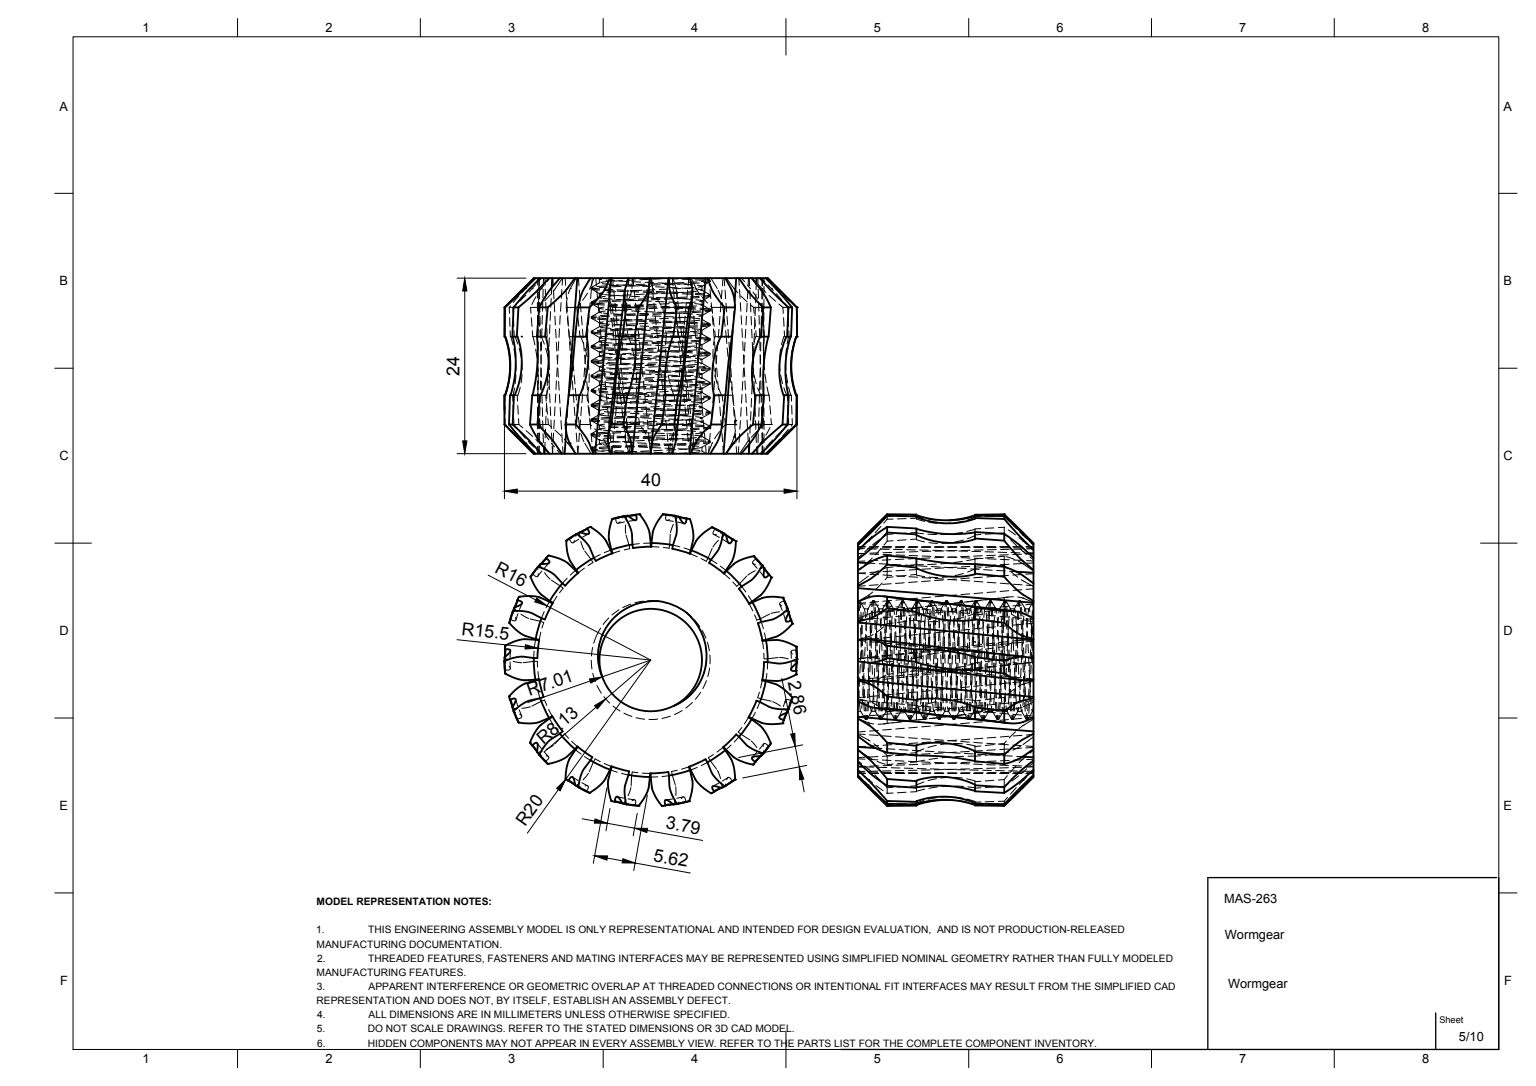
ISO-10303-21;
HEADER;
/* Generated by software containing ST-Developer
 * from STEP Tools, Inc. (www.steptools.com) 
 */

FILE_DESCRIPTION(
/* description */ (''),
/* implementation_level */ '2;1');

FILE_NAME(
/* name */ 'Wormgear.step',
/* time_stamp */ '2026-10-12T15:47:30-07:00',
/* author */ (''),
/* organization */ (''),
/* preprocessor_version */ 'ST-DEVELOPER v20.2',
/* originating_system */ 'Autodesk Translation Framework v15.15.0.0',
/* authorisation */ '');

FILE_SCHEMA (('AUTOMOTIVE_DESIGN { 1 0 10303 214 3 1 1 }'));
ENDSEC;

DATA;
#10=MECHANICAL_DESIGN_GEOMETRIC_PRESENTATION_REPRESENTATION('',(#82),#88483);
#64=SHAPE_REPRESENTATION_RELATIONSHIP('SRR','None',#88520,#73);
#73=ADVANCED_BREP_SHAPE_REPRESENTATION('',(#117),#88474);
#82=STYLED_ITEM('',(#88574),#117);
#117=MANIFOLD_SOLID_BREP('Body1',#12992);
#152=TOROIDAL_SURFACE('',#13586,31.2524414898979,12.0232331490224);
#153=TOROIDAL_SURFACE('',#13587,31.2524414898979,12.0232331490224);
#154=TOROIDAL_SURFACE('',#13588,31.2524414898979,12.0232331490224);
#155=TOROIDAL_SURFACE('',#13589,31.2524414898979,12.0232331490224);
#156=TOROIDAL_SURFACE('',#13590,31.2524414898979,12.0232331490224);
#157=TOROIDAL_SURFACE('',#13591,31.2524414898979,12.0232331490224);
#158=TOROIDAL_SURFACE('',#13592,31.2524414898979,12.0232331490224);
#159=TOROIDAL_SURFACE('',#13593,31.2524414898979,12.0232331490224);
#160=TOROIDAL_SURFACE('',#13594,31.2524414898979,12.0232331490224);
#161=TOROIDAL_SURFACE('',#13595,31.2524414898979,12.0232331490224);
#162=TOROIDAL_SURFACE('',#13596,31.2524414898979,12.0232331490224);
#163=TOROIDAL_SURFACE('',#13597,31.2524414898979,12.0232331490224);
#164=TOROIDAL_SURFACE('',#13598,31.2524414898979,12.0232331490224);
#165=TOROIDAL_SURFACE('',#13599,31.2524414898979,12.0232331490224);
#166=TOROIDAL_SURFACE('',#13600,31.2524414898979,12.0232331490224);
#167=TOROIDAL_SURFACE('',#13601,31.2524414898979,12.0232331490224);
#168=TOROIDAL_SURFACE('',#13602,31.2524414898979,12.0232331490224);
#169=TOROIDAL_SURFACE('',#13603,31.2524414898979,12.0232331490224);
#190=ELLIPSE('',#13431,4.95617711892471,2.63133228090511);
#191=ELLIPSE('',#13435,4.75668688712327,2.27225375309584);
#192=ELLIPSE('',#13437,4.75863627530638,2.27415348140964);
#193=ELLIPSE('',#13440,4.95728877126817,2.63371397588203);
#194=ELLIPSE('',#13442,4.75866828260205,2.27425851275333);
#195=ELLIPSE('',#13445,4.75676106745748,2.27242229825786);
#196=ELLIPSE('',#13449,4.95667352087062,2.63240829794641);
#197=ELLIPSE('',#13451,4.7584190628443,2.27363285019894);
#198=ELLIPSE('',#13454,4.95667835669603,2.63239579497757);
#199=ELLIPSE('',#13456,4.75854812753772,2.27394108049538);
#200=ELLIPSE('',#13459,4.75677100793017,2.27242870543475);
#201=ELLIPSE('',#13461,4.75867193464204,2.27425380136302);
#202=ELLIPSE('',#13464,4.95726759568865,2.6336926662635);
#203=ELLIPSE('',#13468,4.95701438814411,2.63313504607068);
#204=ELLIPSE('',#13470,4.75854681981732,2.2739502765965);
#205=ELLIPSE('',#13473,4.95618501228156,2.63134042899261);
#206=ELLIPSE('',#13475,4.7584142614767,2.27361309014758);
#207=ELLIPSE('',#13478,4.75669159480521,2.2722579746974);
#208=ELLIPSE('',#13480,4.75864115660623,2.27415786894356);
#209=ELLIPSE('',#13483,4.95728232466036,2.63370732110983);
#210=ELLIPSE('',#13487,4.75677068526519,2.27243087287144);
#211=ELLIPSE('',#13489,4.7586448406126,2.27416728394003);
#212=ELLIPSE('',#13492,4.95668328813391,2.63241837237374);
#213=ELLIPSE('',#13494,4.75842436294074,2.27363759998898);
#214=ELLIPSE('',#13497,4.95667013101771,2.63238731158809);
#215=ELLIPSE('',#13499,4.75854743391675,2.27394045782711);
#216=ELLIPSE('',#13502,4.75676675579442,2.2724249104892);
#217=ELLIPSE('',#13504,4.75867738441917,2.27425870334034);
#218=ELLIPSE('',#13507,4.95726880833492,2.63369391317148);
#219=ELLIPSE('',#13511,4.75669596930896,2.27226683434943);
#220=ELLIPSE('',#13516,4.95643307274524,2.6318762393004);
#221=ELLIPSE('',#13520,4.75673549365485,2.27235394216187);
#222=ELLIPSE('',#13524,4.75679029012967,2.27247967692196);
#223=ELLIPSE('',#13528,4.7567393782921,2.272363575723);
#224=ELLIPSE('',#13532,4.75651933654551,2.27183321728508);
#225=ELLIPSE('',#13536,4.75664142700045,2.27213579341419);
#226=ELLIPSE('',#13540,4.75678866048944,2.27247015627199);
#227=ELLIPSE('',#13544,4.75677929568429,2.27246401653084);
#228=ELLIPSE('',#13548,4.7566467644084,2.27215101059843);
#229=ELLIPSE('',#13552,4.75649416981517,2.27179513573923);
#230=ELLIPSE('',#13556,4.75673834040189,2.27235649175302);
#231=ELLIPSE('',#13560,4.7567849310581,2.27247488275134);
#232=ELLIPSE('',#13564,4.75674169310957,2.27236560062855);
#233=ELLIPSE('',#13568,4.75650474573201,2.27182012088408);
#234=ELLIPSE('',#13572,4.75664401077444,2.27213811276921);
#235=ELLIPSE('',#13576,4.75677759115208,2.27246023178278);
#236=ELLIPSE('',#13580,4.95724426884637,2.63364727447111);
#237=ELLIPSE('',#13584,4.95686686267409,2.63282116312156);
#290=CONICAL_SURFACE('',#13250,17.9979895488606,0.785398163397448);
#291=CONICAL_SURFACE('',#13253,17.9979895488606,0.785398163397448);
#292=CONICAL_SURFACE('',#13256,17.9979895488606,0.785398163397448);
#293=CONICAL_SURFACE('',#13259,17.9979895488606,0.785398163397448);
#294=CONICAL_SURFACE('',#13262,17.9979895488606,0.785398163397448);
#295=CONICAL_SURFACE('',#13265,17.9979895488606,0.785398163397448);
#296=CONICAL_SURFACE('',#13268,17.9979895488606,0.785398163397448);
#297=CONICAL_SURFACE('',#13271,17.9979895488606,0.785398163397448);
#298=CONICAL_SURFACE('',#13274,17.9979895488606,0.785398163397448);
#299=CONICAL_SURFACE('',#13277,17.9979895488606,0.785398163397448);
#300=CONICAL_SURFACE('',#13280,17.9979895488606,0.785398163397448);
#301=CONICAL_SURFACE('',#13283,17.9979895488606,0.785398163397448);
#302=CONICAL_SURFACE('',#13286,17.9979895488606,0.785398163397448);
#303=CONICAL_SURFACE('',#13289,17.9979895488606,0.785398163397448);
#304=CONICAL_SURFACE('',#13292,17.9979895488606,0.785398163397448);
#305=CONICAL_SURFACE('',#13295,17.9979895488606,0.785398163397448);
#306=CONICAL_SURFACE('',#13298,17.9979895488606,0.785398163397448);
#307=CONICAL_SURFACE('',#13301,17.9979895488606,0.785398163397448);
#308=CONICAL_SURFACE('',#13304,17.9979895488606,0.785398163397448);
#309=CONICAL_SURFACE('',#13309,17.9979895488606,0.785398163397448);
#310=CONICAL_SURFACE('',#13314,17.9979895488606,0.785398163397448);
#311=CONICAL_SURFACE('',#13319,17.9979895488606,0.785398163397448);
#312=CONICAL_SURFACE('',#13324,17.9979895488606,0.785398163397448);
#313=CONICAL_SURFACE('',#13329,17.9979895488606,0.785398163397448);
#314=CONICAL_SURFACE('',#13334,17.9979895488606,0.785398163397448);
#315=CONICAL_SURFACE('',#13339,17.9979895488606,0.785398163397448);
#316=CONICAL_SURFACE('',#13344,17.9979895488606,0.785398163397448);
#317=CONICAL_SURFACE('',#13349,17.9979895488606,0.785398163397448);
#318=CONICAL_SURFACE('',#13354,17.9979895488606,0.785398163397448);
#319=CONICAL_SURFACE('',#13359,17.9979895488606,0.785398163397448);
#320=CONICAL_SURFACE('',#13364,17.9979895488606,0.785398163397448);
#321=CONICAL_SURFACE('',#13369,17.9979895488606,0.785398163397448);
#322=CONICAL_SURFACE('',#13374,17.9979895488606,0.785398163397448);
#323=CONICAL_SURFACE('',#13379,17.9979895488606,0.785398163397448);
#324=CONICAL_SURFACE('',#13384,17.9979895488606,0.785398163397448);
#325=CONICAL_SURFACE('',#13389,17.9979895488606,0.785398163397448);
#347=FACE_BOUND('',#1491,.T.);
#348=FACE_BOUND('',#1720,.T.);
#440=PLANE('',#13159);
#441=PLANE('',#13196);
#442=PLANE('',#13199);
#443=PLANE('',#13202);
#444=PLANE('',#13205);
#445=PLANE('',#13208);
#446=PLANE('',#13211);
#447=PLANE('',#13214);
#448=PLANE('',#13217);
#449=PLANE('',#13220);
#450=PLANE('',#13223);
#451=PLANE('',#13226);
#452=PLANE('',#13229);
#453=PLANE('',#13232);
#454=PLANE('',#13235);
#455=PLANE('',#13238);
#456=PLANE('',#13241);
#457=PLANE('',#13244);
#458=PLANE('',#13247);
#459=PLANE('',#13394);
#460=PLANE('',#13396);
#461=PLANE('',#13398);
#462=PLANE('',#13400);
#463=PLANE('',#13402);
#464=PLANE('',#13404);
#465=PLANE('',#13406);
#466=PLANE('',#13408);
#467=PLANE('',#13410);
#468=PLANE('',#13412);
#469=PLANE('',#13414);
#470=PLANE('',#13416);
#471=PLANE('',#13418);
#472=PLANE('',#13420);
#473=PLANE('',#13422);
#474=PLANE('',#13424);
#475=PLANE('',#13426);
#476=PLANE('',#13428);
#477=PLANE('',#13430);
#478=PLANE('',#13434);
#479=PLANE('',#13439);
#480=PLANE('',#13444);
#481=PLANE('',#13448);
#482=PLANE('',#13453);
#483=PLANE('',#13458);
#484=PLANE('',#13463);
#485=PLANE('',#13467);
#486=PLANE('',#13472);
#487=PLANE('',#13477);
#488=PLANE('',#13482);
#489=PLANE('',#13486);
#490=PLANE('',#13491);
#491=PLANE('',#13496);
#492=PLANE('',#13501);
#493=PLANE('',#13506);
#494=PLANE('',#13510);
#495=PLANE('',#13514);
#496=PLANE('',#13518);
#497=PLANE('',#13522);
#498=PLANE('',#13526);
#499=PLANE('',#13530);
#500=PLANE('',#13534);
#501=PLANE('',#13538);
#502=PLANE('',#13542);
#503=PLANE('',#13546);
#504=PLANE('',#13550);
#505=PLANE('',#13554);
#506=PLANE('',#13558);
#507=PLANE('',#13562);
#508=PLANE('',#13566);
#509=PLANE('',#13570);
#510=PLANE('',#13574);
#511=PLANE('',#13578);
#512=PLANE('',#13582);
#513=PLANE('',#13680);
#610=B_SPLINE_SURFACE_WITH_KNOTS('',3,3,((#25169,#25170,#25171,#25172,#25173,
#25174,#25175,#25176,#25177,#25178,#25179,#25180,#25181,#25182,#25183,#25184,
#25185,#25186,#25187,#25188,#25189,#25190,#25191,#25192,#25193,#25194,#25195,
#25196,#25197,#25198,#25199,#25200,#25201,#25202,#25203,#25204,#25205,#25206,
#25207,#25208,#25209,#25210,#25211,#25212,#25213,#25214,#25215,#25216,#25217,
#25218,#25219,#25220,#25221,#25222,#25223,#25224,#25225,#25226,#25227,#25228,
#25229,#25230,#25231,#25232,#25233,#25234,#25235,#25236,#25237,#25238,#25239,
#25240,#25241,#25242,#25243,#25244,#25245,#25246,#25247,#25248,#25249,#25250,
#25251,#25252,#25253,#25254,#25255,#25256,#25257,#25258,#25259,#25260,#25261,
#25262,#25263,#25264,#25265,#25266,#25267,#25268,#25269,#25270,#25271,#25272,
#25273,#25274,#25275,#25276,#25277,#25278,#25279,#25280,#25281,#25282,#25283,
#25284,#25285,#25286,#25287,#25288,#25289,#25290,#25291,#25292,#25293,#25294,
#25295,#25296,#25297,#25298,#25299,#25300,#25301,#25302,#25303,#25304,#25305,
#25306,#25307,#25308,#25309,#25310,#25311,#25312,#25313,#25314,#25315,#25316,
#25317,#25318,#25319,#25320,#25321,#25322,#25323,#25324,#25325,#25326,#25327),
(#25328,#25329,#25330,#25331,#25332,#25333,#25334,#25335,#25336,#25337,
#25338,#25339,#25340,#25341,#25342,#25343,#25344,#25345,#25346,#25347,#25348,
#25349,#25350,#25351,#25352,#25353,#25354,#25355,#25356,#25357,#25358,#25359,
#25360,#25361,#25362,#25363,#25364,#25365,#25366,#25367,#25368,#25369,#25370,
#25371,#25372,#25373,#25374,#25375,#25376,#25377,#25378,#25379,#25380,#25381,
#25382,#25383,#25384,#25385,#25386,#25387,#25388,#25389,#25390,#25391,#25392,
#25393,#25394,#25395,#25396,#25397,#25398,#25399,#25400,#25401,#25402,#25403,
#25404,#25405,#25406,#25407,#25408,#25409,#25410,#25411,#25412,#25413,#25414,
#25415,#25416,#25417,#25418,#25419,#25420,#25421,#25422,#25423,#25424,#25425,
#25426,#25427,#25428,#25429,#25430,#25431,#25432,#25433,#25434,#25435,#25436,
#25437,#25438,#25439,#25440,#25441,#25442,#25443,#25444,#25445,#25446,#25447,
#25448,#25449,#25450,#25451,#25452,#25453,#25454,#25455,#25456,#25457,#25458,
#25459,#25460,#25461,#25462,#25463,#25464,#25465,#25466,#25467,#25468,#25469,
#25470,#25471,#25472,#25473,#25474,#25475,#25476,#25477,#25478,#25479,#25480,
#25481,#25482,#25483,#25484,#25485,#25486),(#25487,#25488,#25489,#25490,
#25491,#25492,#25493,#25494,#25495,#25496,#25497,#25498,#25499,#25500,#25501,
#25502,#25503,#25504,#25505,#25506,#25507,#25508,#25509,#25510,#25511,#25512,
#25513,#25514,#25515,#25516,#25517,#25518,#25519,#25520,#25521,#25522,#25523,
#25524,#25525,#25526,#25527,#25528,#25529,#25530,#25531,#25532,#25533,#25534,
#25535,#25536,#25537,#25538,#25539,#25540,#25541,#25542,#25543,#25544,#25545,
#25546,#25547,#25548,#25549,#25550,#25551,#25552,#25553,#25554,#25555,#25556,
#25557,#25558,#25559,#25560,#25561,#25562,#25563,#25564,#25565,#25566,#25567,
#25568,#25569,#25570,#25571,#25572,#25573,#25574,#25575,#25576,#25577,#25578,
#25579,#25580,#25581,#25582,#25583,#25584,#25585,#25586,#25587,#25588,#25589,
#25590,#25591,#25592,#25593,#25594,#25595,#25596,#25597,#25598,#25599,#25600,
#25601,#25602,#25603,#25604,#25605,#25606,#25607,#25608,#25609,#25610,#25611,
#25612,#25613,#25614,#25615,#25616,#25617,#25618,#25619,#25620,#25621,#25622,
#25623,#25624,#25625,#25626,#25627,#25628,#25629,#25630,#25631,#25632,#25633,
#25634,#25635,#25636,#25637,#25638,#25639,#25640,#25641,#25642,#25643,#25644,
#25645),(#25646,#25647,#25648,#25649,#25650,#25651,#25652,#25653,#25654,
#25655,#25656,#25657,#25658,#25659,#25660,#25661,#25662,#25663,#25664,#25665,
#25666,#25667,#25668,#25669,#25670,#25671,#25672,#25673,#25674,#25675,#25676,
#25677,#25678,#25679,#25680,#25681,#25682,#25683,#25684,#25685,#25686,#25687,
#25688,#25689,#25690,#25691,#25692,#25693,#25694,#25695,#25696,#25697,#25698,
#25699,#25700,#25701,#25702,#25703,#25704,#25705,#25706,#25707,#25708,#25709,
#25710,#25711,#25712,#25713,#25714,#25715,#25716,#25717,#25718,#25719,#25720,
#25721,#25722,#25723,#25724,#25725,#25726,#25727,#25728,#25729,#25730,#25731,
#25732,#25733,#25734,#25735,#25736,#25737,#25738,#25739,#25740,#25741,#25742,
#25743,#25744,#25745,#25746,#25747,#25748,#25749,#25750,#25751,#25752,#25753,
#25754,#25755,#25756,#25757,#25758,#25759,#25760,#25761,#25762,#25763,#25764,
#25765,#25766,#25767,#25768,#25769,#25770,#25771,#25772,#25773,#25774,#25775,
#25776,#25777,#25778,#25779,#25780,#25781,#25782,#25783,#25784,#25785,#25786,
#25787,#25788,#25789,#25790,#25791,#25792,#25793,#25794,#25795,#25796,#25797,
#25798,#25799,#25800,#25801,#25802,#25803,#25804)),.UNSPECIFIED.,.F.,.F.,
 .F.,(4,4),(4,1,1,1,1,1,1,1,1,1,1,1,1,1,1,1,1,1,1,1,1,1,1,1,1,1,1,1,1,1,
1,1,1,1,1,1,1,1,1,1,1,1,1,1,1,1,1,1,1,1,1,1,1,1,1,1,1,1,1,1,1,1,1,1,1,1,
1,1,1,1,1,1,1,1,1,1,1,1,1,1,1,1,1,1,1,1,1,1,1,1,1,1,1,1,1,1,1,1,1,1,1,1,
1,1,1,1,1,1,1,1,1,1,1,1,1,1,1,1,1,1,1,1,1,1,1,1,1,1,1,1,1,1,1,1,1,1,1,1,
1,1,1,1,1,1,1,1,1,1,1,1,1,1,1,1,1,1,4),(-8.30696747198589E-5,0.128693006748574),
(11.8548247440635,12.351182148212,12.8474564826858,13.3437308171596,13.8400051516334,
14.3362794861072,14.832553820581,15.3288281550548,15.8251024895286,16.3213768240024,
16.8176511584762,17.31392549295,17.8101998274238,18.3064741618976,18.8027484963714,
19.2990228308452,19.7952971653189,20.2915714997927,20.7878458342665,21.2841201687403,
21.7803945032141,22.2766688376879,22.7729431721617,23.2692175066355,23.7654918411093,
24.2617661755831,24.7580405100569,25.2543148445307,25.7505891790045,26.2468635134783,
26.7431378479521,27.2394121824259,27.7356865168997,28.2319608513735,28.7282351858473,
29.224509520321,29.7207838547948,30.2170581892686,30.7133325237424,31.2096068582162,
31.70588119269,32.2021555271638,32.6984298616376,33.1947041961114,33.6909785305852,
34.187252865059,34.6835271995328,35.1798015340066,35.6760758684804,36.1723502029542,
36.668624537428,37.1648988719018,37.6611732063756,38.1574475408493,38.6537218753231,
39.1499962097969,39.6462705442707,40.1425448787445,40.6388192132183,41.1350935476921,
41.6313678821659,42.1276422166397,42.6239165511135,43.1201908855873,43.6164652200611,
44.1127395545349,44.6090138890087,45.1052882234825,45.6015625579563,46.0978368924301,
46.5941112269039,47.0903855613777,47.5866598958514,48.0829342303252,48.579208564799,
49.0754828992728,49.5717572337466,50.0680315682204,50.5643059026942,51.060580237168,
51.5568545716418,52.0531289061156,52.5494032405894,53.0456775750632,53.541951909537,
54.0382262440108,54.5345005784846,55.0307749129584,55.5270492474322,56.023323581906,
56.5195979163798,57.0158722508535,57.5121465853273,58.0084209198011,58.5046952542749,
59.0009695887487,59.4972439232225,59.9935182576963,60.4897925921701,60.9860669266439,
61.4823412611177,61.9786155955915,62.4748899300653,62.9711642645391,63.4674385990129,
63.9637129334867,64.4599872679605,64.9562616024343,65.452535936908,65.9488102713818,
66.4450846058556,66.9413589403294,67.4376332748032,67.933907609277,68.4301819437508,
68.9264562782246,69.4227306126984,69.9190049471722,70.415279281646,70.9115536161198,
71.4078279505936,71.9041022850674,72.4003766195412,72.896650954015,73.3929252884888,
73.8891996229626,74.3854739574363,74.8817482919101,75.3780226263839,75.8742969608577,
76.3705712953315,76.8668456298053,77.3631199642791,77.8593942987529,78.3556686332267,
78.8519429677005,79.3482173021743,79.8444916366481,80.3407659711219,80.8370403055957,
81.3333146400695,81.8295889745433,82.3258633090171,82.8221376434909,83.3184119779647,
83.8146863124385,84.3109606469122,84.807234981386,85.3035093158598,85.7997836503336,
86.2960579848074,86.7923323192812,87.288606653755,87.7848809882288,88.2811553227026,
88.7774296571764,89.2737039916502),.UNSPECIFIED.);
#611=B_SPLINE_SURFACE_WITH_KNOTS('',3,3,((#26032,#26033,#26034,#26035,#26036,
#26037,#26038,#26039,#26040,#26041,#26042,#26043,#26044,#26045,#26046,#26047,
#26048,#26049,#26050,#26051,#26052,#26053,#26054,#26055,#26056,#26057,#26058,
#26059,#26060,#26061,#26062,#26063,#26064,#26065,#26066,#26067,#26068,#26069,
#26070,#26071,#26072,#26073,#26074,#26075,#26076,#26077,#26078,#26079,#26080,
#26081,#26082,#26083,#26084,#26085,#26086,#26087,#26088,#26089,#26090,#26091,
#26092,#26093,#26094,#26095,#26096,#26097,#26098,#26099,#26100,#26101,#26102,
#26103,#26104,#26105,#26106,#26107,#26108,#26109,#26110,#26111,#26112,#26113,
#26114,#26115,#26116,#26117,#26118,#26119,#26120,#26121,#26122,#26123,#26124,
#26125,#26126,#26127,#26128,#26129,#26130,#26131,#26132,#26133,#26134,#26135,
#26136,#26137,#26138,#26139,#26140,#26141,#26142,#26143,#26144,#26145,#26146,
#26147,#26148,#26149,#26150,#26151,#26152,#26153,#26154,#26155,#26156,#26157,
#26158,#26159,#26160,#26161,#26162,#26163,#26164,#26165,#26166,#26167,#26168,
#26169,#26170,#26171,#26172,#26173,#26174,#26175,#26176,#26177,#26178,#26179,
#26180,#26181,#26182,#26183,#26184,#26185,#26186,#26187,#26188,#26189,#26190),
(#26191,#26192,#26193,#26194,#26195,#26196,#26197,#26198,#26199,#26200,
#26201,#26202,#26203,#26204,#26205,#26206,#26207,#26208,#26209,#26210,#26211,
#26212,#26213,#26214,#26215,#26216,#26217,#26218,#26219,#26220,#26221,#26222,
#26223,#26224,#26225,#26226,#26227,#26228,#26229,#26230,#26231,#26232,#26233,
#26234,#26235,#26236,#26237,#26238,#26239,#26240,#26241,#26242,#26243,#26244,
#26245,#26246,#26247,#26248,#26249,#26250,#26251,#26252,#26253,#26254,#26255,
#26256,#26257,#26258,#26259,#26260,#26261,#26262,#26263,#26264,#26265,#26266,
#26267,#26268,#26269,#26270,#26271,#26272,#26273,#26274,#26275,#26276,#26277,
#26278,#26279,#26280,#26281,#26282,#26283,#26284,#26285,#26286,#26287,#26288,
#26289,#26290,#26291,#26292,#26293,#26294,#26295,#26296,#26297,#26298,#26299,
#26300,#26301,#26302,#26303,#26304,#26305,#26306,#26307,#26308,#26309,#26310,
#26311,#26312,#26313,#26314,#26315,#26316,#26317,#26318,#26319,#26320,#26321,
#26322,#26323,#26324,#26325,#26326,#26327,#26328,#26329,#26330,#26331,#26332,
#26333,#26334,#26335,#26336,#26337,#26338,#26339,#26340,#26341,#26342,#26343,
#26344,#26345,#26346,#26347,#26348,#26349),(#26350,#26351,#26352,#26353,
#26354,#26355,#26356,#26357,#26358,#26359,#26360,#26361,#26362,#26363,#26364,
#26365,#26366,#26367,#26368,#26369,#26370,#26371,#26372,#26373,#26374,#26375,
#26376,#26377,#26378,#26379,#26380,#26381,#26382,#26383,#26384,#26385,#26386,
#26387,#26388,#26389,#26390,#26391,#26392,#26393,#26394,#26395,#26396,#26397,
#26398,#26399,#26400,#26401,#26402,#26403,#26404,#26405,#26406,#26407,#26408,
#26409,#26410,#26411,#26412,#26413,#26414,#26415,#26416,#26417,#26418,#26419,
#26420,#26421,#26422,#26423,#26424,#26425,#26426,#26427,#26428,#26429,#26430,
#26431,#26432,#26433,#26434,#26435,#26436,#26437,#26438,#26439,#26440,#26441,
#26442,#26443,#26444,#26445,#26446,#26447,#26448,#26449,#26450,#26451,#26452,
#26453,#26454,#26455,#26456,#26457,#26458,#26459,#26460,#26461,#26462,#26463,
#26464,#26465,#26466,#26467,#26468,#26469,#26470,#26471,#26472,#26473,#26474,
#26475,#26476,#26477,#26478,#26479,#26480,#26481,#26482,#26483,#26484,#26485,
#26486,#26487,#26488,#26489,#26490,#26491,#26492,#26493,#26494,#26495,#26496,
#26497,#26498,#26499,#26500,#26501,#26502,#26503,#26504,#26505,#26506,#26507,
#26508),(#26509,#26510,#26511,#26512,#26513,#26514,#26515,#26516,#26517,
#26518,#26519,#26520,#26521,#26522,#26523,#26524,#26525,#26526,#26527,#26528,
#26529,#26530,#26531,#26532,#26533,#26534,#26535,#26536,#26537,#26538,#26539,
#26540,#26541,#26542,#26543,#26544,#26545,#26546,#26547,#26548,#26549,#26550,
#26551,#26552,#26553,#26554,#26555,#26556,#26557,#26558,#26559,#26560,#26561,
#26562,#26563,#26564,#26565,#26566,#26567,#26568,#26569,#26570,#26571,#26572,
#26573,#26574,#26575,#26576,#26577,#26578,#26579,#26580,#26581,#26582,#26583,
#26584,#26585,#26586,#26587,#26588,#26589,#26590,#26591,#26592,#26593,#26594,
#26595,#26596,#26597,#26598,#26599,#26600,#26601,#26602,#26603,#26604,#26605,
#26606,#26607,#26608,#26609,#26610,#26611,#26612,#26613,#26614,#26615,#26616,
#26617,#26618,#26619,#26620,#26621,#26622,#26623,#26624,#26625,#26626,#26627,
#26628,#26629,#26630,#26631,#26632,#26633,#26634,#26635,#26636,#26637,#26638,
#26639,#26640,#26641,#26642,#26643,#26644,#26645,#26646,#26647,#26648,#26649,
#26650,#26651,#26652,#26653,#26654,#26655,#26656,#26657,#26658,#26659,#26660,
#26661,#26662,#26663,#26664,#26665,#26666,#26667)),.UNSPECIFIED.,.F.,.F.,
 .F.,(4,4),(4,1,1,1,1,1,1,1,1,1,1,1,1,1,1,1,1,1,1,1,1,1,1,1,1,1,1,1,1,1,
1,1,1,1,1,1,1,1,1,1,1,1,1,1,1,1,1,1,1,1,1,1,1,1,1,1,1,1,1,1,1,1,1,1,1,1,
1,1,1,1,1,1,1,1,1,1,1,1,1,1,1,1,1,1,1,1,1,1,1,1,1,1,1,1,1,1,1,1,1,1,1,1,
1,1,1,1,1,1,1,1,1,1,1,1,1,1,1,1,1,1,1,1,1,1,1,1,1,1,1,1,1,1,1,1,1,1,1,1,
1,1,1,1,1,1,1,1,1,1,1,1,1,1,1,1,1,1,4),(-5.91850316919151E-5,0.128716709650167),
(14.3988535768129,14.8951279112866,15.3914022457604,15.8876765802342,16.383950914708,
16.8802252491818,17.3764995836556,17.8727739181294,18.3690482526032,18.865322587077,
19.3615969215508,19.8578712560246,20.3541455904984,20.8504199249722,21.346694259446,
21.8429685939198,22.3392429283936,22.8355172628674,23.3317915973412,23.828065931815,
24.3243402662887,24.8206146007625,25.3168889352363,25.8131632697101,26.3094376041839,
26.8057119386577,27.3019862731315,27.7982606076053,28.2945349420791,28.7908092765529,
29.2870836110267,29.7833579455005,30.2796322799743,30.7759066144481,31.2721809489219,
31.7684552833957,32.2647296178695,32.7610039523433,33.2572782868171,33.7535526212909,
34.2498269557646,34.7461012902384,35.2423756247122,35.738649959186,36.2349242936598,
36.7311986281336,37.2274729626074,37.7237472970812,38.220021631555,38.7162959660288,
39.2125703005026,39.7088446349764,40.2051189694502,40.701393303924,41.1976676383978,
41.6939419728716,42.1902163073454,42.6864906418191,43.1827649762929,43.6790393107667,
44.1753136452405,44.6715879797143,45.1678623141881,45.6641366486619,46.1604109831357,
46.6566853176095,47.1529596520833,47.6492339865571,48.1455083210309,48.6417826555047,
49.1380569899785,49.6343313244523,50.1306056589261,50.6268799933999,51.1231543278737,
51.6194286623475,52.1157029968213,52.6119773312951,53.1082516657688,53.6045260002426,
54.1008003347164,54.5970746691902,55.093349003664,55.5896233381378,56.0858976726116,
56.5821720070854,57.0784463415592,57.574720676033,58.0709950105068,58.5672693449806,
59.0635436794544,59.5598180139282,60.056092348402,60.5523666828758,61.0486410173496,
61.5449153518233,62.0411896862971,62.5374640207709,63.0337383552447,63.5300126897185,
64.0262870241923,64.5225613586661,65.0188356931399,65.5151100276137,66.0113843620875,
66.5076586965613,67.0039330310351,67.5002073655089,67.9964816999827,68.4927560344565,
68.9890303689303,69.4853047034041,69.9815790378779,70.4778533723517,70.9741277068254,
71.4704020412992,71.966676375773,72.4629507102468,72.9592250447206,73.4554993791944,
73.9517737136682,74.448048048142,74.9443223826158,75.4405967170896,75.9368710515634,
76.4331453860372,76.929419720511,77.4256940549848,77.9219683894586,78.4182427239324,
78.9145170584062,79.41079139288,79.9070657273538,80.4033400618275,80.8996143963013,
81.3958887307751,81.8921630652489,82.3884373997227,82.8847117341965,83.3809860686703,
83.8772604031441,84.3735347376179,84.8698090720917,85.3660834065655,85.8623577410393,
86.3586320755131,86.8549064099869,87.3511807444607,87.8474550789345,88.3437294134083,
88.8400037478821,89.3362780823559,89.8325524168297,90.3288267513034,90.8251010857772,
91.321375420251,91.8177328243995),.UNSPECIFIED.);
#612=B_SPLINE_SURFACE_WITH_KNOTS('',3,3,((#29359,#29360,#29361,#29362),
(#29363,#29364,#29365,#29366),(#29367,#29368,#29369,#29370),(#29371,#29372,
#29373,#29374)),.UNSPECIFIED.,.F.,.F.,.F.,(4,4),(4,4),(-1.00000000738492,
6.33181493099193E-12),(-0.228566601102733,0.828566601102733),
 .UNSPECIFIED.);
#613=B_SPLINE_SURFACE_WITH_KNOTS('',3,3,((#29383,#29384,#29385,#29386),
(#29387,#29388,#29389,#29390),(#29391,#29392,#29393,#29394),(#29395,#29396,
#29397,#29398)),.UNSPECIFIED.,.F.,.F.,.F.,(4,4),(4,4),(-1.00000000738848,
7.85174896767267E-12),(-0.228566601102733,0.828566601102734),
 .UNSPECIFIED.);
#614=B_SPLINE_SURFACE_WITH_KNOTS('',3,3,((#29407,#29408,#29409,#29410),
(#29411,#29412,#29413,#29414),(#29415,#29416,#29417,#29418),(#29419,#29420,
#29421,#29422)),.UNSPECIFIED.,.F.,.F.,.F.,(4,4),(4,4),(-1.00000000739146,
1.55845144401953E-11),(-0.228566601102734,0.828566601102734),
 .UNSPECIFIED.);
#615=B_SPLINE_SURFACE_WITH_KNOTS('',3,3,((#29431,#29432,#29433,#29434),
(#29435,#29436,#29437,#29438),(#29439,#29440,#29441,#29442),(#29443,#29444,
#29445,#29446)),.UNSPECIFIED.,.F.,.F.,.F.,(4,4),(4,4),(-1.00000000737499,
1.10248632487242E-11),(-0.228566601102733,0.828566601102734),
 .UNSPECIFIED.);
#616=B_SPLINE_SURFACE_WITH_KNOTS('',3,3,((#29455,#29456,#29457,#29458),
(#29459,#29460,#29461,#29462),(#29463,#29464,#29465,#29466),(#29467,#29468,
#29469,#29470)),.UNSPECIFIED.,.F.,.F.,.F.,(4,4),(4,4),(-1.00000000737555,
8.62684039186831E-12),(-0.228566601102733,0.828566601102733),
 .UNSPECIFIED.);
#617=B_SPLINE_SURFACE_WITH_KNOTS('',3,3,((#29479,#29480,#29481,#29482),
(#29483,#29484,#29485,#29486),(#29487,#29488,#29489,#29490),(#29491,#29492,
#29493,#29494)),.UNSPECIFIED.,.F.,.F.,.F.,(4,4),(4,4),(-1.00000000738693,
5.72012097454778E-12),(-0.228566601102733,0.828566601102734),
 .UNSPECIFIED.);
#618=B_SPLINE_SURFACE_WITH_KNOTS('',3,3,((#29503,#29504,#29505,#29506),
(#29507,#29508,#29509,#29510),(#29511,#29512,#29513,#29514),(#29515,#29516,
#29517,#29518)),.UNSPECIFIED.,.F.,.F.,.F.,(4,4),(4,4),(-1.00000000738919,
5.62379169111571E-12),(-0.228566601102733,0.828566601102734),
 .UNSPECIFIED.);
#619=B_SPLINE_SURFACE_WITH_KNOTS('',3,3,((#29527,#29528,#29529,#29530),
(#29531,#29532,#29533,#29534),(#29535,#29536,#29537,#29538),(#29539,#29540,
#29541,#29542)),.UNSPECIFIED.,.F.,.F.,.F.,(4,4),(4,4),(-1.00000000739289,
6.50467340161261E-12),(-0.228566601102733,0.828566601102733),
 .UNSPECIFIED.);
#620=B_SPLINE_SURFACE_WITH_KNOTS('',3,3,((#29551,#29552,#29553,#29554),
(#29555,#29556,#29557,#29558),(#29559,#29560,#29561,#29562),(#29563,#29564,
#29565,#29566)),.UNSPECIFIED.,.F.,.F.,.F.,(4,4),(4,4),(-1.00000000739148,
1.40793838710229E-11),(-0.228566601102733,0.828566601102734),
 .UNSPECIFIED.);
#621=B_SPLINE_SURFACE_WITH_KNOTS('',3,3,((#29575,#29576,#29577,#29578),
(#29579,#29580,#29581,#29582),(#29583,#29584,#29585,#29586),(#29587,#29588,
#29589,#29590)),.UNSPECIFIED.,.F.,.F.,.F.,(4,4),(4,4),(-1.00000000738262,
1.82838412051694E-11),(-0.228566601102733,0.828566601102734),
 .UNSPECIFIED.);
#622=B_SPLINE_SURFACE_WITH_KNOTS('',3,3,((#29599,#29600,#29601,#29602),
(#29603,#29604,#29605,#29606),(#29607,#29608,#29609,#29610),(#29611,#29612,
#29613,#29614)),.UNSPECIFIED.,.F.,.F.,.F.,(4,4),(4,4),(-1.00000000737784,
1.02973089179534E-11),(-0.228566601102733,0.828566601102734),
 .UNSPECIFIED.);
#623=B_SPLINE_SURFACE_WITH_KNOTS('',3,3,((#29623,#29624,#29625,#29626),
(#29627,#29628,#29629,#29630),(#29631,#29632,#29633,#29634),(#29635,#29636,
#29637,#29638)),.UNSPECIFIED.,.F.,.F.,.F.,(4,4),(4,4),(-1.00000000738658,
8.03237988227756E-12),(-0.228566601102733,0.828566601102733),
 .UNSPECIFIED.);
#624=B_SPLINE_SURFACE_WITH_KNOTS('',3,3,((#29647,#29648,#29649,#29650),
(#29651,#29652,#29653,#29654),(#29655,#29656,#29657,#29658),(#29659,#29660,
#29661,#29662)),.UNSPECIFIED.,.F.,.F.,.F.,(4,4),(4,4),(-1.00000000738646,
1.53840942326398E-11),(-0.228566601102734,0.828566601102734),
 .UNSPECIFIED.);
#625=B_SPLINE_SURFACE_WITH_KNOTS('',3,3,((#29671,#29672,#29673,#29674),
(#29675,#29676,#29677,#29678),(#29679,#29680,#29681,#29682),(#29683,#29684,
#29685,#29686)),.UNSPECIFIED.,.F.,.F.,.F.,(4,4),(4,4),(-1.00000000737555,
1.43664760969259E-11),(-0.228566601102733,0.828566601102734),
 .UNSPECIFIED.);
#626=B_SPLINE_SURFACE_WITH_KNOTS('',3,3,((#29695,#29696,#29697,#29698),
(#29699,#29700,#29701,#29702),(#29703,#29704,#29705,#29706),(#29707,#29708,
#29709,#29710)),.UNSPECIFIED.,.F.,.F.,.F.,(4,4),(4,4),(-1.00000000738601,
1.73046711715086E-14),(-0.228566601102733,0.828566601102733),
 .UNSPECIFIED.);
#627=B_SPLINE_SURFACE_WITH_KNOTS('',3,3,((#29719,#29720,#29721,#29722),
(#29723,#29724,#29725,#29726),(#29727,#29728,#29729,#29730),(#29731,#29732,
#29733,#29734)),.UNSPECIFIED.,.F.,.F.,.F.,(4,4),(4,4),(-1.00000000738919,
1.07500378715111E-11),(-0.228566601102733,0.828566601102734),
 .UNSPECIFIED.);
#628=B_SPLINE_SURFACE_WITH_KNOTS('',3,3,((#29743,#29744,#29745,#29746),
(#29747,#29748,#29749,#29750),(#29751,#29752,#29753,#29754),(#29755,#29756,
#29757,#29758)),.UNSPECIFIED.,.F.,.F.,.F.,(4,4),(4,4),(-1.00000000739238,
1.18069447204771E-11),(-0.228566601102733,0.828566601102734),
 .UNSPECIFIED.);
#629=B_SPLINE_SURFACE_WITH_KNOTS('',3,3,((#29767,#29768,#29769,#29770),
(#29771,#29772,#29773,#29774),(#29775,#29776,#29777,#29778),(#29779,#29780,
#29781,#29782)),.UNSPECIFIED.,.F.,.F.,.F.,(4,4),(4,4),(-1.00000000739217,
1.4414592214071E-11),(-0.228566601102733,0.828566601102734),
 .UNSPECIFIED.);
#630=B_SPLINE_SURFACE_WITH_KNOTS('',3,3,((#29791,#29792,#29793,#29794),
(#29795,#29796,#29797,#29798),(#29799,#29800,#29801,#29802),(#29803,#29804,
#29805,#29806),(#29807,#29808,#29809,#29810),(#29811,#29812,#29813,#29814),
(#29815,#29816,#29817,#29818)),.UNSPECIFIED.,.F.,.F.,.F.,(4,1,1,1,4),(4,
4),(-5.05014469441185E-14,0.1428571428571,0.28571428571425,0.571428571428551,
1.00000036560903),(-0.228509057368286,0.828509057368286),.UNSPECIFIED.);
#631=B_SPLINE_SURFACE_WITH_KNOTS('',3,3,((#29825,#29826,#29827,#29828),
(#29829,#29830,#29831,#29832),(#29833,#29834,#29835,#29836),(#29837,#29838,
#29839,#29840),(#29841,#29842,#29843,#29844),(#29845,#29846,#29847,#29848)),
 .UNSPECIFIED.,.F.,.F.,.F.,(4,1,1,4),(4,4),(-1.00000000000001,-0.42857142857138,
-0.214285714285645,9.03251141877686E-14),(-0.228509057368286,0.828509057368286),
 .UNSPECIFIED.);
#632=B_SPLINE_SURFACE_WITH_KNOTS('',3,3,((#29851,#29852,#29853,#29854),
(#29855,#29856,#29857,#29858),(#29859,#29860,#29861,#29862),(#29863,#29864,
#29865,#29866)),.UNSPECIFIED.,.F.,.F.,.F.,(4,4),(4,4),(-1.25904053593043E-16,
0.0850880881510745),(-0.100000001340248,0.1),.UNSPECIFIED.);
#633=B_SPLINE_SURFACE_WITH_KNOTS('',3,3,((#29867,#29868,#29869,#29870),
(#29871,#29872,#29873,#29874),(#29875,#29876,#29877,#29878),(#29879,#29880,
#29881,#29882)),.UNSPECIFIED.,.F.,.F.,.F.,(4,4),(4,4),(-1.25904053593043E-16,
0.0850880881510745),(0.5,0.700000001340097),.UNSPECIFIED.);
#634=B_SPLINE_SURFACE_WITH_KNOTS('',3,3,((#29883,#29884,#29885,#29886),
(#29887,#29888,#29889,#29890),(#29891,#29892,#29893,#29894),(#29895,#29896,
#29897,#29898),(#29899,#29900,#29901,#29902),(#29903,#29904,#29905,#29906)),
 .UNSPECIFIED.,.F.,.F.,.F.,(4,1,1,4),(4,4),(-5.14134515353765E-14,0.214285714285675,
0.4285714285714,1.),(-0.228509057368286,0.828509057368286),
 .UNSPECIFIED.);
#635=B_SPLINE_SURFACE_WITH_KNOTS('',3,3,((#29913,#29914,#29915,#29916),
(#29917,#29918,#29919,#29920),(#29921,#29922,#29923,#29924),(#29925,#29926,
#29927,#29928),(#29929,#29930,#29931,#29932),(#29933,#29934,#29935,#29936)),
 .UNSPECIFIED.,.F.,.F.,.F.,(4,1,1,4),(4,4),(-1.00000000000001,-0.428571428571412,
-0.214285714285689,3.45222547669068E-14),(-0.228509057368286,0.828509057368286),
 .UNSPECIFIED.);
#636=B_SPLINE_SURFACE_WITH_KNOTS('',3,3,((#29939,#29940,#29941,#29942),
(#29943,#29944,#29945,#29946),(#29947,#29948,#29949,#29950),(#29951,#29952,
#29953,#29954)),.UNSPECIFIED.,.F.,.F.,.F.,(4,4),(4,4),(-6.55275566865934E-17,
0.0850880881510748),(-0.100000001340248,0.1),.UNSPECIFIED.);
#637=B_SPLINE_SURFACE_WITH_KNOTS('',3,3,((#29955,#29956,#29957,#29958),
(#29959,#29960,#29961,#29962),(#29963,#29964,#29965,#29966),(#29967,#29968,
#29969,#29970)),.UNSPECIFIED.,.F.,.F.,.F.,(4,4),(4,4),(-6.55275566865934E-17,
0.0850880881510748),(0.5,0.700000001340096),.UNSPECIFIED.);
#638=B_SPLINE_SURFACE_WITH_KNOTS('',3,3,((#29971,#29972,#29973,#29974),
(#29975,#29976,#29977,#29978),(#29979,#29980,#29981,#29982),(#29983,#29984,
#29985,#29986),(#29987,#29988,#29989,#29990),(#29991,#29992,#29993,#29994),
(#29995,#29996,#29997,#29998)),.UNSPECIFIED.,.F.,.F.,.F.,(4,1,1,1,4),(4,
4),(-1.49004572061584E-13,0.142857142857015,0.28571428571418,0.571428571428509,
1.),(-0.228509057368286,0.828509057368286),.UNSPECIFIED.);
#639=B_SPLINE_SURFACE_WITH_KNOTS('',3,3,((#30005,#30006,#30007,#30008),
(#30009,#30010,#30011,#30012),(#30013,#30014,#30015,#30016),(#30017,#30018,
#30019,#30020),(#30021,#30022,#30023,#30024),(#30025,#30026,#30027,#30028),
(#30029,#30030,#30031,#30032)),.UNSPECIFIED.,.F.,.F.,.F.,(4,1,1,1,4),(4,
4),(-1.00000000194169,-0.571428572538049,-0.285714286268955,-0.142857143134408,
1.38482423202144E-13),(-0.228509057368286,0.828509057368287),
 .UNSPECIFIED.);
#640=B_SPLINE_SURFACE_WITH_KNOTS('',3,3,((#30035,#30036,#30037,#30038),
(#30039,#30040,#30041,#30042),(#30043,#30044,#30045,#30046),(#30047,#30048,
#30049,#30050)),.UNSPECIFIED.,.F.,.F.,.F.,(4,4),(4,4),(-8.47096787732307E-17,
0.0850880881510746),(-0.100000001340248,0.1),.UNSPECIFIED.);
#641=B_SPLINE_SURFACE_WITH_KNOTS('',3,3,((#30051,#30052,#30053,#30054),
(#30055,#30056,#30057,#30058),(#30059,#30060,#30061,#30062),(#30063,#30064,
#30065,#30066)),.UNSPECIFIED.,.F.,.F.,.F.,(4,4),(4,4),(-8.47096787732307E-17,
0.0850880881510746),(0.5,0.700000001340097),.UNSPECIFIED.);
#642=B_SPLINE_SURFACE_WITH_KNOTS('',3,3,((#30067,#30068,#30069,#30070),
(#30071,#30072,#30073,#30074),(#30075,#30076,#30077,#30078),(#30079,#30080,
#30081,#30082),(#30083,#30084,#30085,#30086),(#30087,#30088,#30089,#30090)),
 .UNSPECIFIED.,.F.,.F.,.F.,(4,1,1,4),(4,4),(-5.51374837743005E-14,0.214285714285672,
0.428571428571398,1.),(-0.228509057368286,0.828509057368286),
 .UNSPECIFIED.);
#643=B_SPLINE_SURFACE_WITH_KNOTS('',3,3,((#30097,#30098,#30099,#30100),
(#30101,#30102,#30103,#30104),(#30105,#30106,#30107,#30108),(#30109,#30110,
#30111,#30112),(#30113,#30114,#30115,#30116),(#30117,#30118,#30119,#30120),
(#30121,#30122,#30123,#30124)),.UNSPECIFIED.,.F.,.F.,.F.,(4,1,1,1,4),(4,
4),(-1.00000000194169,-0.571428572538072,-0.285714286268993,-0.142857143134453,
8.6647533219349E-14),(-0.228509057368286,0.828509057368286),
 .UNSPECIFIED.);
#644=B_SPLINE_SURFACE_WITH_KNOTS('',3,3,((#30127,#30128,#30129,#30130),
(#30131,#30132,#30133,#30134),(#30135,#30136,#30137,#30138),(#30139,#30140,
#30141,#30142)),.UNSPECIFIED.,.F.,.F.,.F.,(4,4),(4,4),(-7.29201002821673E-17,
0.0850880881510746),(-0.100000001340248,0.1),.UNSPECIFIED.);
#645=B_SPLINE_SURFACE_WITH_KNOTS('',3,3,((#30143,#30144,#30145,#30146),
(#30147,#30148,#30149,#30150),(#30151,#30152,#30153,#30154),(#30155,#30156,
#30157,#30158)),.UNSPECIFIED.,.F.,.F.,.F.,(4,4),(4,4),(-7.29201002821673E-17,
0.0850880881510746),(0.5,0.700000001340097),.UNSPECIFIED.);
#646=B_SPLINE_SURFACE_WITH_KNOTS('',3,3,((#30159,#30160,#30161,#30162),
(#30163,#30164,#30165,#30166),(#30167,#30168,#30169,#30170),(#30171,#30172,
#30173,#30174),(#30175,#30176,#30177,#30178),(#30179,#30180,#30181,#30182)),
 .UNSPECIFIED.,.F.,.F.,.F.,(4,1,1,4),(4,4),(-8.88579894424611E-14,0.214285714285645,
0.428571428571379,1.00000036560548),(-0.228509057368286,0.828509057368286),
 .UNSPECIFIED.);
#647=B_SPLINE_SURFACE_WITH_KNOTS('',3,3,((#30189,#30190,#30191,#30192),
(#30193,#30194,#30195,#30196),(#30197,#30198,#30199,#30200),(#30201,#30202,
#30203,#30204),(#30205,#30206,#30207,#30208),(#30209,#30210,#30211,#30212),
(#30213,#30214,#30215,#30216)),.UNSPECIFIED.,.F.,.F.,.F.,(4,1,1,1,4),(4,
4),(-1.00000000194169,-0.571428572538067,-0.285714286268987,-0.142857143134447,
9.29481593602791E-14),(-0.228509057368286,0.828509057368287),
 .UNSPECIFIED.);
#648=B_SPLINE_SURFACE_WITH_KNOTS('',3,3,((#30219,#30220,#30221,#30222),
(#30223,#30224,#30225,#30226),(#30227,#30228,#30229,#30230),(#30231,#30232,
#30233,#30234)),.UNSPECIFIED.,.F.,.F.,.F.,(4,4),(4,4),(-4.15613902556478E-17,
0.0850880881510746),(-0.100000001340247,0.1),.UNSPECIFIED.);
#649=B_SPLINE_SURFACE_WITH_KNOTS('',3,3,((#30235,#30236,#30237,#30238),
(#30239,#30240,#30241,#30242),(#30243,#30244,#30245,#30246),(#30247,#30248,
#30249,#30250)),.UNSPECIFIED.,.F.,.F.,.F.,(4,4),(4,4),(-4.15613902556478E-17,
0.0850880881510746),(0.5,0.700000001340097),.UNSPECIFIED.);
#650=B_SPLINE_SURFACE_WITH_KNOTS('',3,3,((#30251,#30252,#30253,#30254),
(#30255,#30256,#30257,#30258),(#30259,#30260,#30261,#30262),(#30263,#30264,
#30265,#30266),(#30267,#30268,#30269,#30270),(#30271,#30272,#30273,#30274),
(#30275,#30276,#30277,#30278)),.UNSPECIFIED.,.F.,.F.,.F.,(4,1,1,1,4),(4,
4),(-1.61169275568063E-13,0.142857142857005,0.285714285714171,0.571428571428504,
1.00000036560902),(-0.228509057368287,0.828509057368287),.UNSPECIFIED.);
#651=B_SPLINE_SURFACE_WITH_KNOTS('',3,3,((#30285,#30286,#30287,#30288),
(#30289,#30290,#30291,#30292),(#30293,#30294,#30295,#30296),(#30297,#30298,
#30299,#30300),(#30301,#30302,#30303,#30304),(#30305,#30306,#30307,#30308),
(#30309,#30310,#30311,#30312)),.UNSPECIFIED.,.F.,.F.,.F.,(4,1,1,1,4),(4,
4),(-1.00000000194169,-0.571428572538077,-0.285714286269001,-0.142857143134464,
7.42392258779034E-14),(-0.228509057368286,0.828509057368287),
 .UNSPECIFIED.);
#652=B_SPLINE_SURFACE_WITH_KNOTS('',3,3,((#30315,#30316,#30317,#30318),
(#30319,#30320,#30321,#30322),(#30323,#30324,#30325,#30326),(#30327,#30328,
#30329,#30330)),.UNSPECIFIED.,.F.,.F.,.F.,(4,4),(4,4),(-2.07473905953491E-17,
0.0850880881510745),(-0.100000001340248,0.1),.UNSPECIFIED.);
#653=B_SPLINE_SURFACE_WITH_KNOTS('',3,3,((#30331,#30332,#30333,#30334),
(#30335,#30336,#30337,#30338),(#30339,#30340,#30341,#30342),(#30343,#30344,
#30345,#30346)),.UNSPECIFIED.,.F.,.F.,.F.,(4,4),(4,4),(-2.07473905953491E-17,
0.0850880881510745),(0.5,0.700000001340097),.UNSPECIFIED.);
#654=B_SPLINE_SURFACE_WITH_KNOTS('',3,3,((#30347,#30348,#30349,#30350),
(#30351,#30352,#30353,#30354),(#30355,#30356,#30357,#30358),(#30359,#30360,
#30361,#30362),(#30363,#30364,#30365,#30366),(#30367,#30368,#30369,#30370)),
 .UNSPECIFIED.,.F.,.F.,.F.,(4,1,1,4),(4,4),(-5.7507029460608E-14,0.214285714285669,
0.428571428571396,1.),(-0.228509057368286,0.828509057368286),
 .UNSPECIFIED.);
#655=B_SPLINE_SURFACE_WITH_KNOTS('',3,3,((#30377,#30378,#30379,#30380),
(#30381,#30382,#30383,#30384),(#30385,#30386,#30387,#30388),(#30389,#30390,
#30391,#30392),(#30393,#30394,#30395,#30396),(#30397,#30398,#30399,#30400),
(#30401,#30402,#30403,#30404)),.UNSPECIFIED.,.F.,.F.,.F.,(4,1,1,1,4),(4,
4),(-1.00000036560901,-0.571428571428521,-0.285714285714198,-0.142857142857037,
1.24679780388881E-13),(-0.228509057368286,0.828509057368287),
 .UNSPECIFIED.);
#656=B_SPLINE_SURFACE_WITH_KNOTS('',3,3,((#30407,#30408,#30409,#30410),
(#30411,#30412,#30413,#30414),(#30415,#30416,#30417,#30418),(#30419,#30420,
#30421,#30422)),.UNSPECIFIED.,.F.,.F.,.F.,(4,4),(4,4),(-1.07135358020602E-16,
0.0850880881510746),(-0.100000001340247,0.1),.UNSPECIFIED.);
#657=B_SPLINE_SURFACE_WITH_KNOTS('',3,3,((#30423,#30424,#30425,#30426),
(#30427,#30428,#30429,#30430),(#30431,#30432,#30433,#30434),(#30435,#30436,
#30437,#30438)),.UNSPECIFIED.,.F.,.F.,.F.,(4,4),(4,4),(-1.07135358020602E-16,
0.0850880881510746),(0.5,0.700000001340097),.UNSPECIFIED.);
#658=B_SPLINE_SURFACE_WITH_KNOTS('',3,3,((#30439,#30440,#30441,#30442),
(#30443,#30444,#30445,#30446),(#30447,#30448,#30449,#30450),(#30451,#30452,
#30453,#30454),(#30455,#30456,#30457,#30458),(#30459,#30460,#30461,#30462),
(#30463,#30464,#30465,#30466)),.UNSPECIFIED.,.F.,.F.,.F.,(4,1,1,1,4),(4,
4),(-1.32140165738655E-13,0.14285714285703,0.285714285714192,0.571428571428516,
1.),(-0.228509057368287,0.828509057368286),.UNSPECIFIED.);
#659=B_SPLINE_SURFACE_WITH_KNOTS('',3,3,((#30473,#30474,#30475,#30476),
(#30477,#30478,#30479,#30480),(#30481,#30482,#30483,#30484),(#30485,#30486,
#30487,#30488),(#30489,#30490,#30491,#30492),(#30493,#30494,#30495,#30496),
(#30497,#30498,#30499,#30500)),.UNSPECIFIED.,.F.,.F.,.F.,(4,1,1,1,4),(4,
4),(-1.00000000194169,-0.571428572538052,-0.285714286268958,-0.142857143134411,
1.35967626047062E-13),(-0.228509057368286,0.828509057368287),
 .UNSPECIFIED.);
#660=B_SPLINE_SURFACE_WITH_KNOTS('',3,3,((#30503,#30504,#30505,#30506),
(#30507,#30508,#30509,#30510),(#30511,#30512,#30513,#30514),(#30515,#30516,
#30517,#30518)),.UNSPECIFIED.,.F.,.F.,.F.,(4,4),(4,4),(-8.26060906882159E-17,
0.0850880881510746),(-0.100000001340248,0.1),.UNSPECIFIED.);
#661=B_SPLINE_SURFACE_WITH_KNOTS('',3,3,((#30519,#30520,#30521,#30522),
(#30523,#30524,#30525,#30526),(#30527,#30528,#30529,#30530),(#30531,#30532,
#30533,#30534)),.UNSPECIFIED.,.F.,.F.,.F.,(4,4),(4,4),(-8.26060906882159E-17,
0.0850880881510746),(0.5,0.700000001340097),.UNSPECIFIED.);
#662=B_SPLINE_SURFACE_WITH_KNOTS('',3,3,((#30535,#30536,#30537,#30538),
(#30539,#30540,#30541,#30542),(#30543,#30544,#30545,#30546),(#30547,#30548,
#30549,#30550),(#30551,#30552,#30553,#30554),(#30555,#30556,#30557,#30558)),
 .UNSPECIFIED.,.F.,.F.,.F.,(4,1,1,4),(4,4),(-4.84798868997719E-14,0.214285714285676,
0.428571428571401,1.),(-0.228509057368286,0.828509057368286),
 .UNSPECIFIED.);
#663=B_SPLINE_SURFACE_WITH_KNOTS('',3,3,((#30565,#30566,#30567,#30568),
(#30569,#30570,#30571,#30572),(#30573,#30574,#30575,#30576),(#30577,#30578,
#30579,#30580),(#30581,#30582,#30583,#30584),(#30585,#30586,#30587,#30588),
(#30589,#30590,#30591,#30592)),.UNSPECIFIED.,.F.,.F.,.F.,(4,1,1,1,4),(4,
4),(-1.00000000194169,-0.571428572538047,-0.285714286268952,-0.142857143134404,
1.43590337818802E-13),(-0.228509057368286,0.828509057368287),
 .UNSPECIFIED.);
#664=B_SPLINE_SURFACE_WITH_KNOTS('',3,3,((#30595,#30596,#30597,#30598),
(#30599,#30600,#30601,#30602),(#30603,#30604,#30605,#30606),(#30607,#30608,
#30609,#30610)),.UNSPECIFIED.,.F.,.F.,.F.,(4,4),(4,4),(-2.90655708167386E-17,
0.0850880881510745),(-0.100000001340248,0.1),.UNSPECIFIED.);
#665=B_SPLINE_SURFACE_WITH_KNOTS('',3,3,((#30611,#30612,#30613,#30614),
(#30615,#30616,#30617,#30618),(#30619,#30620,#30621,#30622),(#30623,#30624,
#30625,#30626)),.UNSPECIFIED.,.F.,.F.,.F.,(4,4),(4,4),(-2.90655708167386E-17,
0.0850880881510745),(0.5,0.700000001340097),.UNSPECIFIED.);
#666=B_SPLINE_SURFACE_WITH_KNOTS('',3,3,((#30627,#30628,#30629,#30630),
(#30631,#30632,#30633,#30634),(#30635,#30636,#30637,#30638),(#30639,#30640,
#30641,#30642),(#30643,#30644,#30645,#30646),(#30647,#30648,#30649,#30650)),
 .UNSPECIFIED.,.F.,.F.,.F.,(4,1,1,4),(4,4),(-1.28256780196345E-13,0.214285714285614,
0.428571428571356,1.00000036560545),(-0.228509057368286,0.828509057368287),
 .UNSPECIFIED.);
#667=B_SPLINE_SURFACE_WITH_KNOTS('',3,3,((#30657,#30658,#30659,#30660),
(#30661,#30662,#30663,#30664),(#30665,#30666,#30667,#30668),(#30669,#30670,
#30671,#30672),(#30673,#30674,#30675,#30676),(#30677,#30678,#30679,#30680),
(#30681,#30682,#30683,#30684)),.UNSPECIFIED.,.F.,.F.,.F.,(4,1,1,1,4),(4,
4),(-1.00000000194169,-0.571428572538048,-0.285714286268956,-0.142857143134409,
1.3670329409697E-13),(-0.228509057368286,0.828509057368286),
 .UNSPECIFIED.);
#668=B_SPLINE_SURFACE_WITH_KNOTS('',3,3,((#30687,#30688,#30689,#30690),
(#30691,#30692,#30693,#30694),(#30695,#30696,#30697,#30698),(#30699,#30700,
#30701,#30702)),.UNSPECIFIED.,.F.,.F.,.F.,(4,4),(4,4),(-8.38546438727493E-17,
0.0850880881510746),(-0.100000001340248,0.1),.UNSPECIFIED.);
#669=B_SPLINE_SURFACE_WITH_KNOTS('',3,3,((#30703,#30704,#30705,#30706),
(#30707,#30708,#30709,#30710),(#30711,#30712,#30713,#30714),(#30715,#30716,
#30717,#30718)),.UNSPECIFIED.,.F.,.F.,.F.,(4,4),(4,4),(-8.38546438727493E-17,
0.0850880881510746),(0.5,0.700000001340096),.UNSPECIFIED.);
#670=B_SPLINE_SURFACE_WITH_KNOTS('',3,3,((#30719,#30720,#30721,#30722),
(#30723,#30724,#30725,#30726),(#30727,#30728,#30729,#30730),(#30731,#30732,
#30733,#30734),(#30735,#30736,#30737,#30738),(#30739,#30740,#30741,#30742)),
 .UNSPECIFIED.,.F.,.F.,.F.,(4,1,1,4),(4,4),(-8.42716484967992E-14,0.214285714285649,
0.428571428571382,1.),(-0.228509057368286,0.828509057368286),
 .UNSPECIFIED.);
#671=B_SPLINE_SURFACE_WITH_KNOTS('',3,3,((#30749,#30750,#30751,#30752),
(#30753,#30754,#30755,#30756),(#30757,#30758,#30759,#30760),(#30761,#30762,
#30763,#30764),(#30765,#30766,#30767,#30768),(#30769,#30770,#30771,#30772),
(#30773,#30774,#30775,#30776)),.UNSPECIFIED.,.F.,.F.,.F.,(4,1,1,1,4),(4,
4),(-1.00000000000001,-0.571428571428515,-0.285714285714187,-0.142857142857022,
1.42032265556368E-13),(-0.228509057368286,0.828509057368287),
 .UNSPECIFIED.);
#672=B_SPLINE_SURFACE_WITH_KNOTS('',3,3,((#30779,#30780,#30781,#30782),
(#30783,#30784,#30785,#30786),(#30787,#30788,#30789,#30790),(#30791,#30792,
#30793,#30794)),.UNSPECIFIED.,.F.,.F.,.F.,(4,4),(4,4),(-2.97741345382747E-17,
0.0850880881510747),(-0.100000001340248,0.1),.UNSPECIFIED.);
#673=B_SPLINE_SURFACE_WITH_KNOTS('',3,3,((#30795,#30796,#30797,#30798),
(#30799,#30800,#30801,#30802),(#30803,#30804,#30805,#30806),(#30807,#30808,
#30809,#30810)),.UNSPECIFIED.,.F.,.F.,.F.,(4,4),(4,4),(-2.97741345382747E-17,
0.0850880881510747),(0.5,0.700000001340097),.UNSPECIFIED.);
#674=B_SPLINE_SURFACE_WITH_KNOTS('',3,3,((#30811,#30812,#30813,#30814),
(#30815,#30816,#30817,#30818),(#30819,#30820,#30821,#30822),(#30823,#30824,
#30825,#30826),(#30827,#30828,#30829,#30830),(#30831,#30832,#30833,#30834),
(#30835,#30836,#30837,#30838)),.UNSPECIFIED.,.F.,.F.,.F.,(4,1,1,1,4),(4,
4),(-2.83059630199531E-14,0.142857142857119,0.285714285714266,0.57142857142856,
1.),(-0.228509057368285,0.828509057368286),.UNSPECIFIED.);
#675=B_SPLINE_SURFACE_WITH_KNOTS('',3,3,((#30845,#30846,#30847,#30848),
(#30849,#30850,#30851,#30852),(#30853,#30854,#30855,#30856),(#30857,#30858,
#30859,#30860),(#30861,#30862,#30863,#30864),(#30865,#30866,#30867,#30868),
(#30869,#30870,#30871,#30872)),.UNSPECIFIED.,.F.,.F.,.F.,(4,1,1,1,4),(4,
4),(-1.00000000194169,-0.571428572538095,-0.285714286269031,-0.1428571431345,
3.20438120482436E-14),(-0.228509057368286,0.828509057368286),
 .UNSPECIFIED.);
#676=B_SPLINE_SURFACE_WITH_KNOTS('',3,3,((#30875,#30876,#30877,#30878),
(#30879,#30880,#30881,#30882),(#30883,#30884,#30885,#30886),(#30887,#30888,
#30889,#30890)),.UNSPECIFIED.,.F.,.F.,.F.,(4,4),(4,4),(-5.63046512512485E-17,
0.0850880881510746),(-0.100000001340247,0.1),.UNSPECIFIED.);
#677=B_SPLINE_SURFACE_WITH_KNOTS('',3,3,((#30891,#30892,#30893,#30894),
(#30895,#30896,#30897,#30898),(#30899,#30900,#30901,#30902),(#30903,#30904,
#30905,#30906)),.UNSPECIFIED.,.F.,.F.,.F.,(4,4),(4,4),(-5.63046512512485E-17,
0.0850880881510746),(0.5,0.700000001340097),.UNSPECIFIED.);
#678=B_SPLINE_SURFACE_WITH_KNOTS('',3,3,((#30907,#30908,#30909,#30910),
(#30911,#30912,#30913,#30914),(#30915,#30916,#30917,#30918),(#30919,#30920,
#30921,#30922),(#30923,#30924,#30925,#30926),(#30927,#30928,#30929,#30930)),
 .UNSPECIFIED.,.F.,.F.,.F.,(4,1,1,4),(4,4),(-7.28930804605454E-14,0.214285714285657,
0.428571428571387,1.),(-0.228509057368286,0.828509057368286),
 .UNSPECIFIED.);
#679=B_SPLINE_SURFACE_WITH_KNOTS('',3,3,((#30937,#30938,#30939,#30940),
(#30941,#30942,#30943,#30944),(#30945,#30946,#30947,#30948),(#30949,#30950,
#30951,#30952),(#30953,#30954,#30955,#30956),(#30957,#30958,#30959,#30960),
(#30961,#30962,#30963,#30964)),.UNSPECIFIED.,.F.,.F.,.F.,(4,1,1,1,4),(4,
4),(-1.00000000194169,-0.571428572538071,-0.285714286268993,-0.142857143134454,
8.48557335508815E-14),(-0.228509057368286,0.828509057368286),
 .UNSPECIFIED.);
#680=B_SPLINE_SURFACE_WITH_KNOTS('',3,3,((#30967,#30968,#30969,#30970),
(#30971,#30972,#30973,#30974),(#30975,#30976,#30977,#30978),(#30979,#30980,
#30981,#30982)),.UNSPECIFIED.,.F.,.F.,.F.,(4,4),(4,4),(-2.55704448513501E-18,
0.0850880881510746),(-0.100000001340247,0.1),.UNSPECIFIED.);
#681=B_SPLINE_SURFACE_WITH_KNOTS('',3,3,((#30983,#30984,#30985,#30986),
(#30987,#30988,#30989,#30990),(#30991,#30992,#30993,#30994),(#30995,#30996,
#30997,#30998)),.UNSPECIFIED.,.F.,.F.,.F.,(4,4),(4,4),(-2.55704448513501E-18,
0.0850880881510746),(0.5,0.700000001340097),.UNSPECIFIED.);
#682=B_SPLINE_SURFACE_WITH_KNOTS('',3,3,((#30999,#31000,#31001,#31002),
(#31003,#31004,#31005,#31006),(#31007,#31008,#31009,#31010),(#31011,#31012,
#31013,#31014),(#31015,#31016,#31017,#31018),(#31019,#31020,#31021,#31022)),
 .UNSPECIFIED.,.F.,.F.,.F.,(4,1,1,4),(4,4),(-7.99234215486585E-14,0.214285714285652,
0.428571428571384,1.00000036560556),(-0.228509057368286,0.828509057368286),
 .UNSPECIFIED.);
#683=B_SPLINE_SURFACE_WITH_KNOTS('',3,3,((#31029,#31030,#31031,#31032),
(#31033,#31034,#31035,#31036),(#31037,#31038,#31039,#31040),(#31041,#31042,
#31043,#31044),(#31045,#31046,#31047,#31048),(#31049,#31050,#31051,#31052),
(#31053,#31054,#31055,#31056)),.UNSPECIFIED.,.F.,.F.,.F.,(4,1,1,1,4),(4,
4),(-1.00000000194169,-0.571428572538088,-0.28571428626902,-0.142857143134486,
4.79429694563687E-14),(-0.228509057368286,0.828509057368286),
 .UNSPECIFIED.);
#684=B_SPLINE_SURFACE_WITH_KNOTS('',3,3,((#31059,#31060,#31061,#31062),
(#31063,#31064,#31065,#31066),(#31067,#31068,#31069,#31070),(#31071,#31072,
#31073,#31074)),.UNSPECIFIED.,.F.,.F.,.F.,(4,4),(4,4),(-3.9786331981339E-17,
0.0850880881510746),(-0.100000001340247,0.1),.UNSPECIFIED.);
#685=B_SPLINE_SURFACE_WITH_KNOTS('',3,3,((#31075,#31076,#31077,#31078),
(#31079,#31080,#31081,#31082),(#31083,#31084,#31085,#31086),(#31087,#31088,
#31089,#31090)),.UNSPECIFIED.,.F.,.F.,.F.,(4,4),(4,4),(-3.9786331981339E-17,
0.0850880881510746),(0.5,0.700000001340097),.UNSPECIFIED.);
#686=B_SPLINE_SURFACE_WITH_KNOTS('',3,3,((#31091,#31092,#31093,#31094),
(#31095,#31096,#31097,#31098),(#31099,#31100,#31101,#31102),(#31103,#31104,
#31105,#31106),(#31107,#31108,#31109,#31110),(#31111,#31112,#31113,#31114),
(#31115,#31116,#31117,#31118)),.UNSPECIFIED.,.F.,.F.,.F.,(4,1,1,1,4),(4,
4),(-4.11753964257855E-14,0.142857142857108,0.285714285714257,0.571428571428555,
1.00000036560902),(-0.228509057368286,0.828509057368286),.UNSPECIFIED.);
#687=B_SPLINE_SURFACE_WITH_KNOTS('',3,3,((#31125,#31126,#31127,#31128),
(#31129,#31130,#31131,#31132),(#31133,#31134,#31135,#31136),(#31137,#31138,
#31139,#31140),(#31141,#31142,#31143,#31144),(#31145,#31146,#31147,#31148),
(#31149,#31150,#31151,#31152)),.UNSPECIFIED.,.F.,.F.,.F.,(4,1,1,1,4),(4,
4),(-1.00000000000001,-0.571428571428513,-0.285714285714184,-0.14285714285702,
1.44717038445973E-13),(-0.228509057368286,0.828509057368287),
 .UNSPECIFIED.);
#688=B_SPLINE_SURFACE_WITH_KNOTS('',3,3,((#31155,#31156,#31157,#31158),
(#31159,#31160,#31161,#31162),(#31163,#31164,#31165,#31166),(#31167,#31168,
#31169,#31170)),.UNSPECIFIED.,.F.,.F.,.F.,(4,4),(4,4),(-5.86293617278695E-17,
0.0850880881510746),(-0.100000001340248,0.1),.UNSPECIFIED.);
#689=B_SPLINE_SURFACE_WITH_KNOTS('',3,3,((#31171,#31172,#31173,#31174),
(#31175,#31176,#31177,#31178),(#31179,#31180,#31181,#31182),(#31183,#31184,
#31185,#31186)),.UNSPECIFIED.,.F.,.F.,.F.,(4,4),(4,4),(-5.86293617278695E-17,
0.0850880881510746),(0.5,0.700000001340097),.UNSPECIFIED.);
#690=B_SPLINE_SURFACE_WITH_KNOTS('',3,3,((#31187,#31188,#31189,#31190),
(#31191,#31192,#31193,#31194),(#31195,#31196,#31197,#31198),(#31199,#31200,
#31201,#31202),(#31203,#31204,#31205,#31206),(#31207,#31208,#31209,#31210)),
 .UNSPECIFIED.,.F.,.F.,.F.,(4,1,1,4),(4,4),(-9.25699570363353E-14,0.214285714285642,
0.428571428571376,1.),(-0.228509057368286,0.828509057368287),
 .UNSPECIFIED.);
#691=B_SPLINE_SURFACE_WITH_KNOTS('',3,3,((#31217,#31218,#31219,#31220),
(#31221,#31222,#31223,#31224),(#31225,#31226,#31227,#31228),(#31229,#31230,
#31231,#31232),(#31233,#31234,#31235,#31236),(#31237,#31238,#31239,#31240),
(#31241,#31242,#31243,#31244)),.UNSPECIFIED.,.F.,.F.,.F.,(4,1,1,1,4),(4,
4),(-1.00000000194169,-0.571428572538053,-0.285714286268962,-0.142857143134417,
1.28531982146453E-13),(-0.228509057368285,0.828509057368287),
 .UNSPECIFIED.);
#692=B_SPLINE_SURFACE_WITH_KNOTS('',3,3,((#31247,#31248,#31249,#31250),
(#31251,#31252,#31253,#31254),(#31255,#31256,#31257,#31258),(#31259,#31260,
#31261,#31262)),.UNSPECIFIED.,.F.,.F.,.F.,(4,4),(4,4),(-1.09019546950253E-16,
0.0850880881510746),(-0.100000001340248,0.1),.UNSPECIFIED.);
#693=B_SPLINE_SURFACE_WITH_KNOTS('',3,3,((#31263,#31264,#31265,#31266),
(#31267,#31268,#31269,#31270),(#31271,#31272,#31273,#31274),(#31275,#31276,
#31277,#31278)),.UNSPECIFIED.,.F.,.F.,.F.,(4,4),(4,4),(-1.09019546950253E-16,
0.0850880881510746),(0.5,0.700000001340097),.UNSPECIFIED.);
#694=B_SPLINE_SURFACE_WITH_KNOTS('',3,3,((#31279,#31280,#31281,#31282),
(#31283,#31284,#31285,#31286),(#31287,#31288,#31289,#31290),(#31291,#31292,
#31293,#31294),(#31295,#31296,#31297,#31298),(#31299,#31300,#31301,#31302),
(#31303,#31304,#31305,#31306)),.UNSPECIFIED.,.F.,.F.,.F.,(4,1,1,1,4),(4,
4),(-8.76619728054132E-14,0.142857142857068,0.285714285714223,0.571428571428534,
1.),(-0.228509057368286,0.828509057368286),.UNSPECIFIED.);
#695=B_SPLINE_SURFACE_WITH_KNOTS('',3,3,((#31313,#31314,#31315,#31316),
(#31317,#31318,#31319,#31320),(#31321,#31322,#31323,#31324),(#31325,#31326,
#31327,#31328),(#31329,#31330,#31331,#31332),(#31333,#31334,#31335,#31336),
(#31337,#31338,#31339,#31340)),.UNSPECIFIED.,.F.,.F.,.F.,(4,1,1,1,4),(4,
4),(-1.00000000194169,-0.571428572538084,-0.285714286269015,-0.14285714313448,
5.42037452861625E-14),(-0.228509057368285,0.828509057368286),
 .UNSPECIFIED.);
#696=B_SPLINE_SURFACE_WITH_KNOTS('',3,3,((#31343,#31344,#31345,#31346),
(#31347,#31348,#31349,#31350),(#31351,#31352,#31353,#31354),(#31355,#31356,
#31357,#31358)),.UNSPECIFIED.,.F.,.F.,.F.,(4,4),(4,4),(-7.28779245561565E-17,
0.0850880881510746),(-0.100000001340248,0.1),.UNSPECIFIED.);
#697=B_SPLINE_SURFACE_WITH_KNOTS('',3,3,((#31359,#31360,#31361,#31362),
(#31363,#31364,#31365,#31366),(#31367,#31368,#31369,#31370),(#31371,#31372,
#31373,#31374)),.UNSPECIFIED.,.F.,.F.,.F.,(4,4),(4,4),(-7.28779245561565E-17,
0.0850880881510746),(0.5,0.700000001340097),.UNSPECIFIED.);
#698=B_SPLINE_SURFACE_WITH_KNOTS('',3,3,((#31375,#31376,#31377,#31378),
(#31379,#31380,#31381,#31382),(#31383,#31384,#31385,#31386),(#31387,#31388,
#31389,#31390),(#31391,#31392,#31393,#31394),(#31395,#31396,#31397,#31398)),
 .UNSPECIFIED.,.F.,.F.,.F.,(4,1,1,4),(4,4),(-4.97324904964964E-14,0.214285714285675,
0.4285714285714,1.),(-0.228509057368285,0.828509057368286),
 .UNSPECIFIED.);
#699=B_SPLINE_SURFACE_WITH_KNOTS('',3,3,((#31405,#31406,#31407,#31408),
(#31409,#31410,#31411,#31412),(#31413,#31414,#31415,#31416),(#31417,#31418,
#31419,#31420),(#31421,#31422,#31423,#31424),(#31425,#31426,#31427,#31428)),
 .UNSPECIFIED.,.F.,.F.,.F.,(4,1,1,4),(4,4),(-1.0000003656055,-0.428571428571403,
-0.214285714285677,4.91672674796106E-14),(-0.228509057368286,0.828509057368286),
 .UNSPECIFIED.);
#700=B_SPLINE_SURFACE_WITH_KNOTS('',3,3,((#31431,#31432,#31433,#31434),
(#31435,#31436,#31437,#31438),(#31439,#31440,#31441,#31442),(#31443,#31444,
#31445,#31446)),.UNSPECIFIED.,.F.,.F.,.F.,(4,4),(4,4),(-2.90655708167386E-17,
0.0850880881510745),(-0.100000001340247,0.1),.UNSPECIFIED.);
#701=B_SPLINE_SURFACE_WITH_KNOTS('',3,3,((#31447,#31448,#31449,#31450),
(#31451,#31452,#31453,#31454),(#31455,#31456,#31457,#31458),(#31459,#31460,
#31461,#31462)),.UNSPECIFIED.,.F.,.F.,.F.,(4,4),(4,4),(-2.90655708167386E-17,
0.0850880881510745),(0.5,0.700000001340097),.UNSPECIFIED.);
#702=B_SPLINE_SURFACE_WITH_KNOTS('',3,3,((#31463,#31464,#31465,#31466),
(#31467,#31468,#31469,#31470),(#31471,#31472,#31473,#31474),(#31475,#31476,
#31477,#31478)),.UNSPECIFIED.,.F.,.F.,.F.,(4,4),(4,4),(-0.871332876340297,
-0.774999998579001),(-0.3,0.9),.UNSPECIFIED.);
#703=B_SPLINE_SURFACE_WITH_KNOTS('',3,3,((#31494,#31495,#31496,#31497),
(#31498,#31499,#31500,#31501),(#31502,#31503,#31504,#31505),(#31506,#31507,
#31508,#31509)),.UNSPECIFIED.,.F.,.F.,.F.,(4,4),(4,4),(-5.14197626699797E-6,
1.00000003476692),(-0.228566601398621,0.828566601398622),.UNSPECIFIED.);
#704=B_SPLINE_SURFACE_WITH_KNOTS('',3,3,((#31514,#31515,#31516,#31517),
(#31518,#31519,#31520,#31521),(#31522,#31523,#31524,#31525),(#31526,#31527,
#31528,#31529)),.UNSPECIFIED.,.F.,.F.,.F.,(4,4),(4,4),(0.774999998579001,
0.871332876340297),(-0.3,0.9),.UNSPECIFIED.);
#705=B_SPLINE_SURFACE_WITH_KNOTS('',3,3,((#31577,#31578,#31579,#31580),
(#31581,#31582,#31583,#31584),(#31585,#31586,#31587,#31588),(#31589,#31590,
#31591,#31592)),.UNSPECIFIED.,.F.,.F.,.F.,(4,4),(4,4),(0.774999998579001,
0.871332876340298),(-0.3,0.9),.UNSPECIFIED.);
#706=B_SPLINE_SURFACE_WITH_KNOTS('',3,3,((#31612,#31613,#31614,#31615),
(#31616,#31617,#31618,#31619),(#31620,#31621,#31622,#31623),(#31624,#31625,
#31626,#31627)),.UNSPECIFIED.,.F.,.F.,.F.,(4,4),(4,4),(-0.871332876340297,
-0.774999998579),(-0.3,0.9),.UNSPECIFIED.);
#707=B_SPLINE_SURFACE_WITH_KNOTS('',3,3,((#31629,#31630,#31631,#31632),
(#31633,#31634,#31635,#31636),(#31637,#31638,#31639,#31640),(#31641,#31642,
#31643,#31644)),.UNSPECIFIED.,.F.,.F.,.F.,(4,4),(4,4),(-5.14198768541974E-6,
1.00000001443829),(-0.228566601398622,0.828566601398622),.UNSPECIFIED.);
#708=B_SPLINE_SURFACE_WITH_KNOTS('',3,3,((#31645,#31646,#31647,#31648),
(#31649,#31650,#31651,#31652),(#31653,#31654,#31655,#31656),(#31657,#31658,
#31659,#31660)),.UNSPECIFIED.,.F.,.F.,.F.,(4,4),(4,4),(-0.871332876340297,
-0.774999998579),(-0.3,0.9),.UNSPECIFIED.);
#709=B_SPLINE_SURFACE_WITH_KNOTS('',3,3,((#31676,#31677,#31678,#31679),
(#31680,#31681,#31682,#31683),(#31684,#31685,#31686,#31687),(#31688,#31689,
#31690,#31691)),.UNSPECIFIED.,.F.,.F.,.F.,(4,4),(4,4),(0.774999998579,0.871332876340298),
(-0.3,0.9),.UNSPECIFIED.);
#710=B_SPLINE_SURFACE_WITH_KNOTS('',3,3,((#31711,#31712,#31713,#31714),
(#31715,#31716,#31717,#31718),(#31719,#31720,#31721,#31722),(#31723,#31724,
#31725,#31726)),.UNSPECIFIED.,.F.,.F.,.F.,(4,4),(4,4),(-5.14198403323007E-6,
1.00000003476684),(-0.228566601398622,0.828566601398622),.UNSPECIFIED.);
#711=B_SPLINE_SURFACE_WITH_KNOTS('',3,3,((#31817,#31818,#31819,#31820),
(#31821,#31822,#31823,#31824),(#31825,#31826,#31827,#31828),(#31829,#31830,
#31831,#31832)),.UNSPECIFIED.,.F.,.F.,.F.,(4,4),(4,4),(-0.871332876340297,
-0.774999998579),(-0.3,0.9),.UNSPECIFIED.);
#712=B_SPLINE_SURFACE_WITH_KNOTS('',3,3,((#31833,#31834,#31835,#31836),
(#31837,#31838,#31839,#31840),(#31841,#31842,#31843,#31844),(#31845,#31846,
#31847,#31848)),.UNSPECIFIED.,.F.,.F.,.F.,(4,4),(4,4),(-5.14197252954318E-6,
1.00000003476695),(-0.228566601398621,0.828566601398621),.UNSPECIFIED.);
#713=B_SPLINE_SURFACE_WITH_KNOTS('',3,3,((#31853,#31854,#31855,#31856),
(#31857,#31858,#31859,#31860),(#31861,#31862,#31863,#31864),(#31865,#31866,
#31867,#31868)),.UNSPECIFIED.,.F.,.F.,.F.,(4,4),(4,4),(0.774999998579001,
0.871332876340297),(-0.3,0.9),.UNSPECIFIED.);
#714=B_SPLINE_SURFACE_WITH_KNOTS('',3,3,((#31897,#31898,#31899,#31900),
(#31901,#31902,#31903,#31904),(#31905,#31906,#31907,#31908),(#31909,#31910,
#31911,#31912)),.UNSPECIFIED.,.F.,.F.,.F.,(4,4),(4,4),(0.774999998579,0.871332876340298),
(-0.3,0.9),.UNSPECIFIED.);
#715=B_SPLINE_SURFACE_WITH_KNOTS('',3,3,((#31930,#31931,#31932,#31933),
(#31934,#31935,#31936,#31937),(#31938,#31939,#31940,#31941),(#31942,#31943,
#31944,#31945)),.UNSPECIFIED.,.F.,.F.,.F.,(4,4),(4,4),(-0.871332876340297,
-0.774999998579),(-0.3,0.9),.UNSPECIFIED.);
#716=B_SPLINE_SURFACE_WITH_KNOTS('',3,3,((#31946,#31947,#31948,#31949),
(#31950,#31951,#31952,#31953),(#31954,#31955,#31956,#31957),(#31958,#31959,
#31960,#31961)),.UNSPECIFIED.,.F.,.F.,.F.,(4,4),(4,4),(-5.14197203926869E-6,
1.00000003476844),(-0.228566601398621,0.828566601398622),.UNSPECIFIED.);
#717=B_SPLINE_SURFACE_WITH_KNOTS('',3,3,((#31962,#31963,#31964,#31965),
(#31966,#31967,#31968,#31969),(#31970,#31971,#31972,#31973),(#31974,#31975,
#31976,#31977)),.UNSPECIFIED.,.F.,.F.,.F.,(4,4),(4,4),(-0.871332876340297,
-0.774999998579),(-0.3,0.9),.UNSPECIFIED.);
#718=B_SPLINE_SURFACE_WITH_KNOTS('',3,3,((#31991,#31992,#31993,#31994),
(#31995,#31996,#31997,#31998),(#31999,#32000,#32001,#32002),(#32003,#32004,
#32005,#32006)),.UNSPECIFIED.,.F.,.F.,.F.,(4,4),(4,4),(0.774999998579,0.871332876340298),
(-0.3,0.9),.UNSPECIFIED.);
#719=B_SPLINE_SURFACE_WITH_KNOTS('',3,3,((#32024,#32025,#32026,#32027),
(#32028,#32029,#32030,#32031),(#32032,#32033,#32034,#32035),(#32036,#32037,
#32038,#32039)),.UNSPECIFIED.,.F.,.F.,.F.,(4,4),(4,4),(-5.14197986944964E-6,
1.00000003476884),(-0.228566601398622,0.828566601398622),.UNSPECIFIED.);
#720=B_SPLINE_SURFACE_WITH_KNOTS('',3,3,((#32054,#32055,#32056,#32057),
(#32058,#32059,#32060,#32061),(#32062,#32063,#32064,#32065),(#32066,#32067,
#32068,#32069)),.UNSPECIFIED.,.F.,.F.,.F.,(4,4),(4,4),(-0.871332876340297,
-0.774999998579),(-0.3,0.9),.UNSPECIFIED.);
#721=B_SPLINE_SURFACE_WITH_KNOTS('',3,3,((#32070,#32071,#32072,#32073),
(#32074,#32075,#32076,#32077),(#32078,#32079,#32080,#32081),(#32082,#32083,
#32084,#32085)),.UNSPECIFIED.,.F.,.F.,.F.,(4,4),(4,4),(-5.14196888445895E-6,
1.0000000144377),(-0.228566601398621,0.828566601398621),.UNSPECIFIED.);
#722=B_SPLINE_SURFACE_WITH_KNOTS('',3,3,((#32090,#32091,#32092,#32093),
(#32094,#32095,#32096,#32097),(#32098,#32099,#32100,#32101),(#32102,#32103,
#32104,#32105)),.UNSPECIFIED.,.F.,.F.,.F.,(4,4),(4,4),(0.774999998579,0.871332876340297),
(-0.3,0.9),.UNSPECIFIED.);
#723=B_SPLINE_SURFACE_WITH_KNOTS('',3,3,((#32134,#32135,#32136,#32137),
(#32138,#32139,#32140,#32141),(#32142,#32143,#32144,#32145),(#32146,#32147,
#32148,#32149)),.UNSPECIFIED.,.F.,.F.,.F.,(4,4),(4,4),(0.774999998579,0.871332876340298),
(-0.3,0.9),.UNSPECIFIED.);
#724=B_SPLINE_SURFACE_WITH_KNOTS('',3,3,((#32167,#32168,#32169,#32170),
(#32171,#32172,#32173,#32174),(#32175,#32176,#32177,#32178),(#32179,#32180,
#32181,#32182)),.UNSPECIFIED.,.F.,.F.,.F.,(4,4),(4,4),(-0.871332876340297,
-0.774999998579),(-0.3,0.9),.UNSPECIFIED.);
#725=B_SPLINE_SURFACE_WITH_KNOTS('',3,3,((#32183,#32184,#32185,#32186),
(#32187,#32188,#32189,#32190),(#32191,#32192,#32193,#32194),(#32195,#32196,
#32197,#32198)),.UNSPECIFIED.,.F.,.F.,.F.,(4,4),(4,4),(-5.14198304557567E-6,
1.00000001443821),(-0.228566601398622,0.828566601398623),.UNSPECIFIED.);
#726=B_SPLINE_SURFACE_WITH_KNOTS('',3,3,((#32199,#32200,#32201,#32202),
(#32203,#32204,#32205,#32206),(#32207,#32208,#32209,#32210),(#32211,#32212,
#32213,#32214)),.UNSPECIFIED.,.F.,.F.,.F.,(4,4),(4,4),(-0.871332876340297,
-0.774999998579),(-0.3,0.9),.UNSPECIFIED.);
#727=B_SPLINE_SURFACE_WITH_KNOTS('',3,3,((#32228,#32229,#32230,#32231),
(#32232,#32233,#32234,#32235),(#32236,#32237,#32238,#32239),(#32240,#32241,
#32242,#32243)),.UNSPECIFIED.,.F.,.F.,.F.,(4,4),(4,4),(0.774999998579,0.871332876340297),
(-0.3,0.9),.UNSPECIFIED.);
#728=B_SPLINE_SURFACE_WITH_KNOTS('',3,3,((#32261,#32262,#32263,#32264),
(#32265,#32266,#32267,#32268),(#32269,#32270,#32271,#32272),(#32273,#32274,
#32275,#32276)),.UNSPECIFIED.,.F.,.F.,.F.,(4,4),(4,4),(-5.14198393375409E-6,
1.0000000347646),(-0.228566601398622,0.828566601398623),.UNSPECIFIED.);
#729=B_SPLINE_SURFACE_WITH_KNOTS('',3,3,((#32291,#32292,#32293,#32294),
(#32295,#32296,#32297,#32298),(#32299,#32300,#32301,#32302),(#32303,#32304,
#32305,#32306)),.UNSPECIFIED.,.F.,.F.,.F.,(4,4),(4,4),(-0.871332876340297,
-0.774999998579),(-0.3,0.9),.UNSPECIFIED.);
#730=B_SPLINE_SURFACE_WITH_KNOTS('',3,3,((#32307,#32308,#32309,#32310),
(#32311,#32312,#32313,#32314),(#32315,#32316,#32317,#32318),(#32319,#32320,
#32321,#32322)),.UNSPECIFIED.,.F.,.F.,.F.,(4,4),(4,4),(-5.14198745804606E-6,
1.00000001443741),(-0.228566601398622,0.828566601398622),.UNSPECIFIED.);
#731=B_SPLINE_SURFACE_WITH_KNOTS('',3,3,((#32327,#32328,#32329,#32330),
(#32331,#32332,#32333,#32334),(#32335,#32336,#32337,#32338),(#32339,#32340,
#32341,#32342)),.UNSPECIFIED.,.F.,.F.,.F.,(4,4),(4,4),(0.774999998579001,
0.871332876340298),(-0.3,0.900000000000001),.UNSPECIFIED.);
#732=B_SPLINE_SURFACE_WITH_KNOTS('',3,3,((#32371,#32372,#32373,#32374),
(#32375,#32376,#32377,#32378),(#32379,#32380,#32381,#32382),(#32383,#32384,
#32385,#32386)),.UNSPECIFIED.,.F.,.F.,.F.,(4,4),(4,4),(0.774999998579001,
0.871332876340297),(-0.3,0.9),.UNSPECIFIED.);
#733=B_SPLINE_SURFACE_WITH_KNOTS('',3,3,((#32404,#32405,#32406,#32407),
(#32408,#32409,#32410,#32411),(#32412,#32413,#32414,#32415),(#32416,#32417,
#32418,#32419)),.UNSPECIFIED.,.F.,.F.,.F.,(4,4),(4,4),(-0.871332876340297,
-0.774999998579),(-0.3,0.9),.UNSPECIFIED.);
#734=B_SPLINE_SURFACE_WITH_KNOTS('',3,3,((#32420,#32421,#32422,#32423),
(#32424,#32425,#32426,#32427),(#32428,#32429,#32430,#32431),(#32432,#32433,
#32434,#32435)),.UNSPECIFIED.,.F.,.F.,.F.,(4,4),(4,4),(-5.14199177104047E-6,
1.0000000347666),(-0.228566601398622,0.828566601398623),.UNSPECIFIED.);
#735=B_SPLINE_SURFACE_WITH_KNOTS('',3,3,((#32436,#32437,#32438,#32439),
(#32440,#32441,#32442,#32443),(#32444,#32445,#32446,#32447),(#32448,#32449,
#32450,#32451)),.UNSPECIFIED.,.F.,.F.,.F.,(4,4),(4,4),(-0.871332876340297,
-0.774999998579),(-0.3,0.9),.UNSPECIFIED.);
#736=B_SPLINE_SURFACE_WITH_KNOTS('',3,3,((#32465,#32466,#32467,#32468),
(#32469,#32470,#32471,#32472),(#32473,#32474,#32475,#32476),(#32477,#32478,
#32479,#32480)),.UNSPECIFIED.,.F.,.F.,.F.,(4,4),(4,4),(0.774999998579,0.871332876340298),
(-0.3,0.9),.UNSPECIFIED.);
#737=B_SPLINE_SURFACE_WITH_KNOTS('',3,3,((#32498,#32499,#32500,#32501),
(#32502,#32503,#32504,#32505),(#32506,#32507,#32508,#32509),(#32510,#32511,
#32512,#32513)),.UNSPECIFIED.,.F.,.F.,.F.,(4,4),(4,4),(-5.14197888179524E-6,
1.00000003476801),(-0.228566601398622,0.828566601398622),.UNSPECIFIED.);
#738=B_SPLINE_SURFACE_WITH_KNOTS('',3,3,((#32528,#32529,#32530,#32531),
(#32532,#32533,#32534,#32535),(#32536,#32537,#32538,#32539),(#32540,#32541,
#32542,#32543)),.UNSPECIFIED.,.F.,.F.,.F.,(4,4),(4,4),(-0.871332876340297,
-0.774999998579),(-0.3,0.9),.UNSPECIFIED.);
#739=B_SPLINE_SURFACE_WITH_KNOTS('',3,3,((#32544,#32545,#32546,#32547),
(#32548,#32549,#32550,#32551),(#32552,#32553,#32554,#32555),(#32556,#32557,
#32558,#32559)),.UNSPECIFIED.,.F.,.F.,.F.,(4,4),(4,4),(-5.1419737019387E-6,
1.00000001443723),(-0.228566601398621,0.828566601398621),.UNSPECIFIED.);
#740=B_SPLINE_SURFACE_WITH_KNOTS('',3,3,((#32564,#32565,#32566,#32567),
(#32568,#32569,#32570,#32571),(#32572,#32573,#32574,#32575),(#32576,#32577,
#32578,#32579)),.UNSPECIFIED.,.F.,.F.,.F.,(4,4),(4,4),(0.774999998579,0.871332876340297),
(-0.3,0.9),.UNSPECIFIED.);
#741=B_SPLINE_SURFACE_WITH_KNOTS('',3,3,((#32608,#32609,#32610,#32611),
(#32612,#32613,#32614,#32615),(#32616,#32617,#32618,#32619),(#32620,#32621,
#32622,#32623)),.UNSPECIFIED.,.F.,.F.,.F.,(4,4),(4,4),(0.774999998579,0.871332876340297),
(-0.3,0.9),.UNSPECIFIED.);
#742=B_SPLINE_SURFACE_WITH_KNOTS('',3,3,((#32641,#32642,#32643,#32644),
(#32645,#32646,#32647,#32648),(#32649,#32650,#32651,#32652),(#32653,#32654,
#32655,#32656)),.UNSPECIFIED.,.F.,.F.,.F.,(4,4),(4,4),(-0.871332876340297,
-0.774999998579),(-0.3,0.9),.UNSPECIFIED.);
#743=B_SPLINE_SURFACE_WITH_KNOTS('',3,3,((#32657,#32658,#32659,#32660),
(#32661,#32662,#32663,#32664),(#32665,#32666,#32667,#32668),(#32669,#32670,
#32671,#32672)),.UNSPECIFIED.,.F.,.F.,.F.,(4,4),(4,4),(-5.1419868967173E-6,
1.00000003476766),(-0.228566601398622,0.828566601398622),.UNSPECIFIED.);
#744=B_SPLINE_SURFACE_WITH_KNOTS('',3,3,((#32673,#32674,#32675,#32676),
(#32677,#32678,#32679,#32680),(#32681,#32682,#32683,#32684),(#32685,#32686,
#32687,#32688)),.UNSPECIFIED.,.F.,.F.,.F.,(4,4),(4,4),(-0.871332876340297,
-0.774999998579),(-0.3,0.9),.UNSPECIFIED.);
#745=B_SPLINE_SURFACE_WITH_KNOTS('',3,3,((#32702,#32703,#32704,#32705),
(#32706,#32707,#32708,#32709),(#32710,#32711,#32712,#32713),(#32714,#32715,
#32716,#32717)),.UNSPECIFIED.,.F.,.F.,.F.,(4,4),(4,4),(0.774999998579001,
0.871332876340297),(-0.3,0.9),.UNSPECIFIED.);
#746=B_SPLINE_SURFACE_WITH_KNOTS('',3,3,((#32735,#32736,#32737,#32738),
(#32739,#32740,#32741,#32742),(#32743,#32744,#32745,#32746),(#32747,#32748,
#32749,#32750)),.UNSPECIFIED.,.F.,.F.,.F.,(4,4),(4,4),(-5.14197624568169E-6,
1.00000001444045),(-0.228566601398621,0.828566601398622),.UNSPECIFIED.);
#747=B_SPLINE_SURFACE_WITH_KNOTS('',3,3,((#32765,#32766,#32767,#32768),
(#32769,#32770,#32771,#32772),(#32773,#32774,#32775,#32776),(#32777,#32778,
#32779,#32780)),.UNSPECIFIED.,.F.,.F.,.F.,(4,4),(4,4),(-0.871332876340297,
-0.774999998579),(-0.3,0.9),.UNSPECIFIED.);
#748=B_SPLINE_SURFACE_WITH_KNOTS('',3,3,((#32781,#32782,#32783,#32784),
(#32785,#32786,#32787,#32788),(#32789,#32790,#32791,#32792),(#32793,#32794,
#32795,#32796)),.UNSPECIFIED.,.F.,.F.,.F.,(4,4),(4,4),(-5.14197358114643E-6,
1.00000003476771),(-0.228566601398621,0.828566601398622),.UNSPECIFIED.);
#749=B_SPLINE_SURFACE_WITH_KNOTS('',3,3,((#32801,#32802,#32803,#32804),
(#32805,#32806,#32807,#32808),(#32809,#32810,#32811,#32812),(#32813,#32814,
#32815,#32816)),.UNSPECIFIED.,.F.,.F.,.F.,(4,4),(4,4),(0.774999998579,0.871332876340297),
(-0.3,0.9),.UNSPECIFIED.);
#750=B_SPLINE_SURFACE_WITH_KNOTS('',3,3,((#32845,#32846,#32847,#32848),
(#32849,#32850,#32851,#32852),(#32853,#32854,#32855,#32856),(#32857,#32858,
#32859,#32860)),.UNSPECIFIED.,.F.,.F.,.F.,(4,4),(4,4),(0.774999998579,0.871332876340298),
(-0.3,0.9),.UNSPECIFIED.);
#751=B_SPLINE_SURFACE_WITH_KNOTS('',3,3,((#32878,#32879,#32880,#32881),
(#32882,#32883,#32884,#32885),(#32886,#32887,#32888,#32889),(#32890,#32891,
#32892,#32893)),.UNSPECIFIED.,.F.,.F.,.F.,(4,4),(4,4),(-0.871332876340297,
-0.774999998579001),(-0.3,0.9),.UNSPECIFIED.);
#752=B_SPLINE_SURFACE_WITH_KNOTS('',3,3,((#32894,#32895,#32896,#32897),
(#32898,#32899,#32900,#32901),(#32902,#32903,#32904,#32905),(#32906,#32907,
#32908,#32909)),.UNSPECIFIED.,.F.,.F.,.F.,(4,4),(4,4),(-5.14197949286199E-6,
1.00000003476611),(-0.228566601398621,0.828566601398622),.UNSPECIFIED.);
#753=B_SPLINE_SURFACE_WITH_KNOTS('',3,3,((#32910,#32911,#32912,#32913),
(#32914,#32915,#32916,#32917),(#32918,#32919,#32920,#32921),(#32922,#32923,
#32924,#32925)),.UNSPECIFIED.,.F.,.F.,.F.,(4,4),(4,4),(-0.871332876340297,
-0.774999998579),(-0.3,0.9),.UNSPECIFIED.);
#754=B_SPLINE_SURFACE_WITH_KNOTS('',3,3,((#32939,#32940,#32941,#32942),
(#32943,#32944,#32945,#32946),(#32947,#32948,#32949,#32950),(#32951,#32952,
#32953,#32954)),.UNSPECIFIED.,.F.,.F.,.F.,(4,4),(4,4),(0.774999998579,0.871332876340297),
(-0.3,0.9),.UNSPECIFIED.);
#755=B_SPLINE_SURFACE_WITH_KNOTS('',3,3,((#32959,#32960,#32961,#32962),
(#32963,#32964,#32965,#32966),(#32967,#32968,#32969,#32970),(#32971,#32972,
#32973,#32974)),.UNSPECIFIED.,.F.,.F.,.F.,(4,4),(4,4),(-5.14197984813336E-6,
1.00000003476548),(-0.228566601398621,0.828566601398622),.UNSPECIFIED.);
#796=FACE_OUTER_BOUND('',#1462,.T.);
#797=FACE_OUTER_BOUND('',#1463,.T.);
#798=FACE_OUTER_BOUND('',#1464,.T.);
#799=FACE_OUTER_BOUND('',#1465,.T.);
#800=FACE_OUTER_BOUND('',#1466,.T.);
#801=FACE_OUTER_BOUND('',#1467,.T.);
#802=FACE_OUTER_BOUND('',#1468,.T.);
#803=FACE_OUTER_BOUND('',#1469,.T.);
#804=FACE_OUTER_BOUND('',#1470,.T.);
#805=FACE_OUTER_BOUND('',#1471,.T.);
#806=FACE_OUTER_BOUND('',#1472,.T.);
#807=FACE_OUTER_BOUND('',#1473,.T.);
#808=FACE_OUTER_BOUND('',#1474,.T.);
#809=FACE_OUTER_BOUND('',#1475,.T.);
#810=FACE_OUTER_BOUND('',#1476,.T.);
#811=FACE_OUTER_BOUND('',#1477,.T.);
#812=FACE_OUTER_BOUND('',#1478,.T.);
#813=FACE_OUTER_BOUND('',#1479,.T.);
#814=FACE_OUTER_BOUND('',#1480,.T.);
#815=FACE_OUTER_BOUND('',#1481,.T.);
#816=FACE_OUTER_BOUND('',#1482,.T.);
#817=FACE_OUTER_BOUND('',#1483,.T.);
#818=FACE_OUTER_BOUND('',#1484,.T.);
#819=FACE_OUTER_BOUND('',#1485,.T.);
#820=FACE_OUTER_BOUND('',#1486,.T.);
#821=FACE_OUTER_BOUND('',#1487,.T.);
#822=FACE_OUTER_BOUND('',#1488,.T.);
#823=FACE_OUTER_BOUND('',#1489,.T.);
#824=FACE_OUTER_BOUND('',#1490,.T.);
#825=FACE_OUTER_BOUND('',#1492,.T.);
#826=FACE_OUTER_BOUND('',#1493,.T.);
#827=FACE_OUTER_BOUND('',#1494,.T.);
#828=FACE_OUTER_BOUND('',#1495,.T.);
#829=FACE_OUTER_BOUND('',#1496,.T.);
#830=FACE_OUTER_BOUND('',#1497,.T.);
#831=FACE_OUTER_BOUND('',#1498,.T.);
#832=FACE_OUTER_BOUND('',#1499,.T.);
#833=FACE_OUTER_BOUND('',#1500,.T.);
#834=FACE_OUTER_BOUND('',#1501,.T.);
#835=FACE_OUTER_BOUND('',#1502,.T.);
#836=FACE_OUTER_BOUND('',#1503,.T.);
#837=FACE_OUTER_BOUND('',#1504,.T.);
#838=FACE_OUTER_BOUND('',#1505,.T.);
#839=FACE_OUTER_BOUND('',#1506,.T.);
#840=FACE_OUTER_BOUND('',#1507,.T.);
#841=FACE_OUTER_BOUND('',#1508,.T.);
#842=FACE_OUTER_BOUND('',#1509,.T.);
#843=FACE_OUTER_BOUND('',#1510,.T.);
#844=FACE_OUTER_BOUND('',#1511,.T.);
#845=FACE_OUTER_BOUND('',#1512,.T.);
#846=FACE_OUTER_BOUND('',#1513,.T.);
#847=FACE_OUTER_BOUND('',#1514,.T.);
#848=FACE_OUTER_BOUND('',#1515,.T.);
#849=FACE_OUTER_BOUND('',#1516,.T.);
#850=FACE_OUTER_BOUND('',#1517,.T.);
#851=FACE_OUTER_BOUND('',#1518,.T.);
#852=FACE_OUTER_BOUND('',#1519,.T.);
#853=FACE_OUTER_BOUND('',#1520,.T.);
#854=FACE_OUTER_BOUND('',#1521,.T.);
#855=FACE_OUTER_BOUND('',#1522,.T.);
#856=FACE_OUTER_BOUND('',#1523,.T.);
#857=FACE_OUTER_BOUND('',#1524,.T.);
#858=FACE_OUTER_BOUND('',#1525,.T.);
#859=FACE_OUTER_BOUND('',#1526,.T.);
#860=FACE_OUTER_BOUND('',#1527,.T.);
#861=FACE_OUTER_BOUND('',#1528,.T.);
#862=FACE_OUTER_BOUND('',#1529,.T.);
#863=FACE_OUTER_BOUND('',#1530,.T.);
#864=FACE_OUTER_BOUND('',#1531,.T.);
#865=FACE_OUTER_BOUND('',#1532,.T.);
#866=FACE_OUTER_BOUND('',#1533,.T.);
#867=FACE_OUTER_BOUND('',#1534,.T.);
#868=FACE_OUTER_BOUND('',#1535,.T.);
#869=FACE_OUTER_BOUND('',#1536,.T.);
#870=FACE_OUTER_BOUND('',#1537,.T.);
#871=FACE_OUTER_BOUND('',#1538,.T.);
#872=FACE_OUTER_BOUND('',#1539,.T.);
#873=FACE_OUTER_BOUND('',#1540,.T.);
#874=FACE_OUTER_BOUND('',#1541,.T.);
#875=FACE_OUTER_BOUND('',#1542,.T.);
#876=FACE_OUTER_BOUND('',#1543,.T.);
#877=FACE_OUTER_BOUND('',#1544,.T.);
#878=FACE_OUTER_BOUND('',#1545,.T.);
#879=FACE_OUTER_BOUND('',#1546,.T.);
#880=FACE_OUTER_BOUND('',#1547,.T.);
#881=FACE_OUTER_BOUND('',#1548,.T.);
#882=FACE_OUTER_BOUND('',#1549,.T.);
#883=FACE_OUTER_BOUND('',#1550,.T.);
#884=FACE_OUTER_BOUND('',#1551,.T.);
#885=FACE_OUTER_BOUND('',#1552,.T.);
#886=FACE_OUTER_BOUND('',#1553,.T.);
#887=FACE_OUTER_BOUND('',#1554,.T.);
#888=FACE_OUTER_BOUND('',#1555,.T.);
#889=FACE_OUTER_BOUND('',#1556,.T.);
#890=FACE_OUTER_BOUND('',#1557,.T.);
#891=FACE_OUTER_BOUND('',#1558,.T.);
#892=FACE_OUTER_BOUND('',#1559,.T.);
#893=FACE_OUTER_BOUND('',#1560,.T.);
#894=FACE_OUTER_BOUND('',#1561,.T.);
#895=FACE_OUTER_BOUND('',#1562,.T.);
#896=FACE_OUTER_BOUND('',#1563,.T.);
#897=FACE_OUTER_BOUND('',#1564,.T.);
#898=FACE_OUTER_BOUND('',#1565,.T.);
#899=FACE_OUTER_BOUND('',#1566,.T.);
#900=FACE_OUTER_BOUND('',#1567,.T.);
#901=FACE_OUTER_BOUND('',#1568,.T.);
#902=FACE_OUTER_BOUND('',#1569,.T.);
#903=FACE_OUTER_BOUND('',#1570,.T.);
#904=FACE_OUTER_BOUND('',#1571,.T.);
#905=FACE_OUTER_BOUND('',#1572,.T.);
#906=FACE_OUTER_BOUND('',#1573,.T.);
#907=FACE_OUTER_BOUND('',#1574,.T.);
#908=FACE_OUTER_BOUND('',#1575,.T.);
#909=FACE_OUTER_BOUND('',#1576,.T.);
#910=FACE_OUTER_BOUND('',#1577,.T.);
#911=FACE_OUTER_BOUND('',#1578,.T.);
#912=FACE_OUTER_BOUND('',#1579,.T.);
#913=FACE_OUTER_BOUND('',#1580,.T.);
#914=FACE_OUTER_BOUND('',#1581,.T.);
#915=FACE_OUTER_BOUND('',#1582,.T.);
#916=FACE_OUTER_BOUND('',#1583,.T.);
#917=FACE_OUTER_BOUND('',#1584,.T.);
#918=FACE_OUTER_BOUND('',#1585,.T.);
#919=FACE_OUTER_BOUND('',#1586,.T.);
#920=FACE_OUTER_BOUND('',#1587,.T.);
#921=FACE_OUTER_BOUND('',#1588,.T.);
#922=FACE_OUTER_BOUND('',#1589,.T.);
#923=FACE_OUTER_BOUND('',#1590,.T.);
#924=FACE_OUTER_BOUND('',#1591,.T.);
#925=FACE_OUTER_BOUND('',#1592,.T.);
#926=FACE_OUTER_BOUND('',#1593,.T.);
#927=FACE_OUTER_BOUND('',#1594,.T.);
#928=FACE_OUTER_BOUND('',#1595,.T.);
#929=FACE_OUTER_BOUND('',#1596,.T.);
#930=FACE_OUTER_BOUND('',#1597,.T.);
#931=FACE_OUTER_BOUND('',#1598,.T.);
#932=FACE_OUTER_BOUND('',#1599,.T.);
#933=FACE_OUTER_BOUND('',#1600,.T.);
#934=FACE_OUTER_BOUND('',#1601,.T.);
#935=FACE_OUTER_BOUND('',#1602,.T.);
#936=FACE_OUTER_BOUND('',#1603,.T.);
#937=FACE_OUTER_BOUND('',#1604,.T.);
#938=FACE_OUTER_BOUND('',#1605,.T.);
#939=FACE_OUTER_BOUND('',#1606,.T.);
#940=FACE_OUTER_BOUND('',#1607,.T.);
#941=FACE_OUTER_BOUND('',#1608,.T.);
#942=FACE_OUTER_BOUND('',#1609,.T.);
#943=FACE_OUTER_BOUND('',#1610,.T.);
#944=FACE_OUTER_BOUND('',#1611,.T.);
#945=FACE_OUTER_BOUND('',#1612,.T.);
#946=FACE_OUTER_BOUND('',#1613,.T.);
#947=FACE_OUTER_BOUND('',#1614,.T.);
#948=FACE_OUTER_BOUND('',#1615,.T.);
#949=FACE_OUTER_BOUND('',#1616,.T.);
#950=FACE_OUTER_BOUND('',#1617,.T.);
#951=FACE_OUTER_BOUND('',#1618,.T.);
#952=FACE_OUTER_BOUND('',#1619,.T.);
#953=FACE_OUTER_BOUND('',#1620,.T.);
#954=FACE_OUTER_BOUND('',#1621,.T.);
#955=FACE_OUTER_BOUND('',#1622,.T.);
#956=FACE_OUTER_BOUND('',#1623,.T.);
#957=FACE_OUTER_BOUND('',#1624,.T.);
#958=FACE_OUTER_BOUND('',#1625,.T.);
#959=FACE_OUTER_BOUND('',#1626,.T.);
#960=FACE_OUTER_BOUND('',#1627,.T.);
#961=FACE_OUTER_BOUND('',#1628,.T.);
#962=FACE_OUTER_BOUND('',#1629,.T.);
#963=FACE_OUTER_BOUND('',#1630,.T.);
#964=FACE_OUTER_BOUND('',#1631,.T.);
#965=FACE_OUTER_BOUND('',#1632,.T.);
#966=FACE_OUTER_BOUND('',#1633,.T.);
#967=FACE_OUTER_BOUND('',#1634,.T.);
#968=FACE_OUTER_BOUND('',#1635,.T.);
#969=FACE_OUTER_BOUND('',#1636,.T.);
#970=FACE_OUTER_BOUND('',#1637,.T.);
#971=FACE_OUTER_BOUND('',#1638,.T.);
#972=FACE_OUTER_BOUND('',#1639,.T.);
#973=FACE_OUTER_BOUND('',#1640,.T.);
#974=FACE_OUTER_BOUND('',#1641,.T.);
#975=FACE_OUTER_BOUND('',#1642,.T.);
#976=FACE_OUTER_BOUND('',#1643,.T.);
#977=FACE_OUTER_BOUND('',#1644,.T.);
#978=FACE_OUTER_BOUND('',#1645,.T.);
#979=FACE_OUTER_BOUND('',#1646,.T.);
#980=FACE_OUTER_BOUND('',#1647,.T.);
#981=FACE_OUTER_BOUND('',#1648,.T.);
#982=FACE_OUTER_BOUND('',#1649,.T.);
#983=FACE_OUTER_BOUND('',#1650,.T.);
#984=FACE_OUTER_BOUND('',#1651,.T.);
#985=FACE_OUTER_BOUND('',#1652,.T.);
#986=FACE_OUTER_BOUND('',#1653,.T.);
#987=FACE_OUTER_BOUND('',#1654,.T.);
#988=FACE_OUTER_BOUND('',#1655,.T.);
#989=FACE_OUTER_BOUND('',#1656,.T.);
#990=FACE_OUTER_BOUND('',#1657,.T.);
#991=FACE_OUTER_BOUND('',#1658,.T.);
#992=FACE_OUTER_BOUND('',#1659,.T.);
#993=FACE_OUTER_BOUND('',#1660,.T.);
#994=FACE_OUTER_BOUND('',#1661,.T.);
#995=FACE_OUTER_BOUND('',#1662,.T.);
#996=FACE_OUTER_BOUND('',#1663,.T.);
#997=FACE_OUTER_BOUND('',#1664,.T.);
#998=FACE_OUTER_BOUND('',#1665,.T.);
#999=FACE_OUTER_BOUND('',#1666,.T.);
#1000=FACE_OUTER_BOUND('',#1667,.T.);
#1001=FACE_OUTER_BOUND('',#1668,.T.);
#1002=FACE_OUTER_BOUND('',#1669,.T.);
#1003=FACE_OUTER_BOUND('',#1670,.T.);
#1004=FACE_OUTER_BOUND('',#1671,.T.);
#1005=FACE_OUTER_BOUND('',#1672,.T.);
#1006=FACE_OUTER_BOUND('',#1673,.T.);
#1007=FACE_OUTER_BOUND('',#1674,.T.);
#1008=FACE_OUTER_BOUND('',#1675,.T.);
#1009=FACE_OUTER_BOUND('',#1676,.T.);
#1010=FACE_OUTER_BOUND('',#1677,.T.);
#1011=FACE_OUTER_BOUND('',#1678,.T.);
#1012=FACE_OUTER_BOUND('',#1679,.T.);
#1013=FACE_OUTER_BOUND('',#1680,.T.);
#1014=FACE_OUTER_BOUND('',#1681,.T.);
#1015=FACE_OUTER_BOUND('',#1682,.T.);
#1016=FACE_OUTER_BOUND('',#1683,.T.);
#1017=FACE_OUTER_BOUND('',#1684,.T.);
#1018=FACE_OUTER_BOUND('',#1685,.T.);
#1019=FACE_OUTER_BOUND('',#1686,.T.);
#1020=FACE_OUTER_BOUND('',#1687,.T.);
#1021=FACE_OUTER_BOUND('',#1688,.T.);
#1022=FACE_OUTER_BOUND('',#1689,.T.);
#1023=FACE_OUTER_BOUND('',#1690,.T.);
#1024=FACE_OUTER_BOUND('',#1691,.T.);
#1025=FACE_OUTER_BOUND('',#1692,.T.);
#1026=FACE_OUTER_BOUND('',#1693,.T.);
#1027=FACE_OUTER_BOUND('',#1694,.T.);
#1028=FACE_OUTER_BOUND('',#1695,.T.);
#1029=FACE_OUTER_BOUND('',#1696,.T.);
#1030=FACE_OUTER_BOUND('',#1697,.T.);
#1031=FACE_OUTER_BOUND('',#1698,.T.);
#1032=FACE_OUTER_BOUND('',#1699,.T.);
#1033=FACE_OUTER_BOUND('',#1700,.T.);
#1034=FACE_OUTER_BOUND('',#1701,.T.);
#1035=FACE_OUTER_BOUND('',#1702,.T.);
#1036=FACE_OUTER_BOUND('',#1703,.T.);
#1037=FACE_OUTER_BOUND('',#1704,.T.);
#1038=FACE_OUTER_BOUND('',#1705,.T.);
#1039=FACE_OUTER_BOUND('',#1706,.T.);
#1040=FACE_OUTER_BOUND('',#1707,.T.);
#1041=FACE_OUTER_BOUND('',#1708,.T.);
#1042=FACE_OUTER_BOUND('',#1709,.T.);
#1043=FACE_OUTER_BOUND('',#1710,.T.);
#1044=FACE_OUTER_BOUND('',#1711,.T.);
#1045=FACE_OUTER_BOUND('',#1712,.T.);
#1046=FACE_OUTER_BOUND('',#1713,.T.);
#1047=FACE_OUTER_BOUND('',#1714,.T.);
#1048=FACE_OUTER_BOUND('',#1715,.T.);
#1049=FACE_OUTER_BOUND('',#1716,.T.);
#1050=FACE_OUTER_BOUND('',#1717,.T.);
#1051=FACE_OUTER_BOUND('',#1718,.T.);
#1052=FACE_OUTER_BOUND('',#1719,.T.);
#1053=FACE_OUTER_BOUND('',#1721,.T.);
#1054=FACE_OUTER_BOUND('',#1722,.T.);
#1055=FACE_OUTER_BOUND('',#1723,.T.);
#1056=FACE_OUTER_BOUND('',#1724,.T.);
#1057=FACE_OUTER_BOUND('',#1725,.T.);
#1058=FACE_OUTER_BOUND('',#1726,.T.);
#1059=FACE_OUTER_BOUND('',#1727,.T.);
#1060=FACE_OUTER_BOUND('',#1728,.T.);
#1061=FACE_OUTER_BOUND('',#1729,.T.);
#1062=FACE_OUTER_BOUND('',#1730,.T.);
#1063=FACE_OUTER_BOUND('',#1731,.T.);
#1064=FACE_OUTER_BOUND('',#1732,.T.);
#1065=FACE_OUTER_BOUND('',#1733,.T.);
#1066=FACE_OUTER_BOUND('',#1734,.T.);
#1067=FACE_OUTER_BOUND('',#1735,.T.);
#1068=FACE_OUTER_BOUND('',#1736,.T.);
#1069=FACE_OUTER_BOUND('',#1737,.T.);
#1070=FACE_OUTER_BOUND('',#1738,.T.);
#1071=FACE_OUTER_BOUND('',#1739,.T.);
#1072=FACE_OUTER_BOUND('',#1740,.T.);
#1073=FACE_OUTER_BOUND('',#1741,.T.);
#1074=FACE_OUTER_BOUND('',#1742,.T.);
#1075=FACE_OUTER_BOUND('',#1743,.T.);
#1076=FACE_OUTER_BOUND('',#1744,.T.);
#1077=FACE_OUTER_BOUND('',#1745,.T.);
#1078=FACE_OUTER_BOUND('',#1746,.T.);
#1079=FACE_OUTER_BOUND('',#1747,.T.);
#1080=FACE_OUTER_BOUND('',#1748,.T.);
#1081=FACE_OUTER_BOUND('',#1749,.T.);
#1082=FACE_OUTER_BOUND('',#1750,.T.);
#1083=FACE_OUTER_BOUND('',#1751,.T.);
#1084=FACE_OUTER_BOUND('',#1752,.T.);
#1085=FACE_OUTER_BOUND('',#1753,.T.);
#1086=FACE_OUTER_BOUND('',#1754,.T.);
#1087=FACE_OUTER_BOUND('',#1755,.T.);
#1088=FACE_OUTER_BOUND('',#1756,.T.);
#1089=FACE_OUTER_BOUND('',#1757,.T.);
#1090=FACE_OUTER_BOUND('',#1758,.T.);
#1091=FACE_OUTER_BOUND('',#1759,.T.);
#1092=FACE_OUTER_BOUND('',#1760,.T.);
#1093=FACE_OUTER_BOUND('',#1761,.T.);
#1094=FACE_OUTER_BOUND('',#1762,.T.);
#1095=FACE_OUTER_BOUND('',#1763,.T.);
#1096=FACE_OUTER_BOUND('',#1764,.T.);
#1097=FACE_OUTER_BOUND('',#1765,.T.);
#1098=FACE_OUTER_BOUND('',#1766,.T.);
#1099=FACE_OUTER_BOUND('',#1767,.T.);
#1100=FACE_OUTER_BOUND('',#1768,.T.);
#1101=FACE_OUTER_BOUND('',#1769,.T.);
#1102=FACE_OUTER_BOUND('',#1770,.T.);
#1103=FACE_OUTER_BOUND('',#1771,.T.);
#1104=FACE_OUTER_BOUND('',#1772,.T.);
#1105=FACE_OUTER_BOUND('',#1773,.T.);
#1106=FACE_OUTER_BOUND('',#1774,.T.);
#1107=FACE_OUTER_BOUND('',#1775,.T.);
#1108=FACE_OUTER_BOUND('',#1776,.T.);
#1109=FACE_OUTER_BOUND('',#1777,.T.);
#1110=FACE_OUTER_BOUND('',#1778,.T.);
#1111=FACE_OUTER_BOUND('',#1779,.T.);
#1112=FACE_OUTER_BOUND('',#1780,.T.);
#1113=FACE_OUTER_BOUND('',#1781,.T.);
#1462=EDGE_LOOP('',(#8072,#8073,#8074,#8075));
#1463=EDGE_LOOP('',(#8076,#8077,#8078,#8079,#8080,#8081));
#1464=EDGE_LOOP('',(#8082,#8083,#8084,#8085,#8086,#8087));
#1465=EDGE_LOOP('',(#8088,#8089,#8090,#8091,#8092,#8093));
#1466=EDGE_LOOP('',(#8094,#8095,#8096,#8097,#8098,#8099));
#1467=EDGE_LOOP('',(#8100,#8101,#8102,#8103,#8104,#8105));
#1468=EDGE_LOOP('',(#8106,#8107,#8108,#8109,#8110,#8111));
#1469=EDGE_LOOP('',(#8112,#8113,#8114,#8115,#8116,#8117));
#1470=EDGE_LOOP('',(#8118,#8119,#8120,#8121,#8122,#8123));
#1471=EDGE_LOOP('',(#8124,#8125,#8126,#8127,#8128,#8129));
#1472=EDGE_LOOP('',(#8130,#8131,#8132,#8133,#8134,#8135));
#1473=EDGE_LOOP('',(#8136,#8137,#8138,#8139,#8140,#8141));
#1474=EDGE_LOOP('',(#8142,#8143,#8144,#8145));
#1475=EDGE_LOOP('',(#8146,#8147,#8148,#8149,#8150));
#1476=EDGE_LOOP('',(#8151,#8152,#8153,#8154,#8155,#8156));
#1477=EDGE_LOOP('',(#8157,#8158,#8159,#8160,#8161,#8162));
#1478=EDGE_LOOP('',(#8163,#8164,#8165,#8166,#8167,#8168));
#1479=EDGE_LOOP('',(#8169,#8170,#8171,#8172,#8173,#8174));
#1480=EDGE_LOOP('',(#8175,#8176,#8177,#8178,#8179,#8180));
#1481=EDGE_LOOP('',(#8181,#8182,#8183,#8184,#8185));
#1482=EDGE_LOOP('',(#8186,#8187,#8188,#8189,#8190,#8191));
#1483=EDGE_LOOP('',(#8192,#8193,#8194,#8195,#8196));
#1484=EDGE_LOOP('',(#8197,#8198,#8199,#8200,#8201));
#1485=EDGE_LOOP('',(#8202,#8203,#8204,#8205,#8206));
#1486=EDGE_LOOP('',(#8207,#8208,#8209,#8210,#8211,#8212));
#1487=EDGE_LOOP('',(#8213,#8214,#8215,#8216,#8217,#8218));
#1488=EDGE_LOOP('',(#8219,#8220,#8221,#8222,#8223,#8224,#8225,#8226,#8227,
#8228,#8229,#8230,#8231,#8232,#8233,#8234,#8235,#8236,#8237,#8238,#8239,
#8240,#8241,#8242,#8243,#8244,#8245,#8246,#8247,#8248,#8249,#8250,#8251,
#8252,#8253,#8254,#8255,#8256,#8257,#8258,#8259,#8260,#8261,#8262,#8263,
#8264,#8265,#8266,#8267,#8268,#8269));
#1489=EDGE_LOOP('',(#8270,#8271,#8272,#8273,#8274,#8275,#8276,#8277,#8278,
#8279,#8280,#8281,#8282,#8283,#8284,#8285,#8286,#8287,#8288,#8289,#8290,
#8291,#8292,#8293,#8294,#8295,#8296,#8297,#8298,#8299,#8300,#8301,#8302,
#8303,#8304,#8305,#8306,#8307,#8308,#8309,#8310,#8311,#8312,#8313,#8314,
#8315,#8316,#8317,#8318));
#1490=EDGE_LOOP('',(#8319,#8320,#8321,#8322,#8323,#8324,#8325,#8326,#8327,
#8328,#8329,#8330,#8331,#8332,#8333,#8334,#8335,#8336,#8337,#8338,#8339,
#8340,#8341,#8342,#8343,#8344,#8345,#8346,#8347,#8348,#8349,#8350,#8351,
#8352,#8353,#8354,#8355,#8356,#8357,#8358,#8359,#8360,#8361,#8362,#8363,
#8364,#8365,#8366,#8367,#8368,#8369,#8370,#8371,#8372,#8373,#8374,#8375,
#8376,#8377,#8378,#8379,#8380,#8381,#8382,#8383,#8384,#8385,#8386,#8387,
#8388,#8389,#8390));
#1491=EDGE_LOOP('',(#8391,#8392,#8393,#8394));
#1492=EDGE_LOOP('',(#8395,#8396,#8397,#8398));
#1493=EDGE_LOOP('',(#8399,#8400,#8401,#8402));
#1494=EDGE_LOOP('',(#8403,#8404,#8405,#8406));
#1495=EDGE_LOOP('',(#8407,#8408,#8409,#8410));
#1496=EDGE_LOOP('',(#8411,#8412,#8413,#8414));
#1497=EDGE_LOOP('',(#8415,#8416,#8417,#8418));
#1498=EDGE_LOOP('',(#8419,#8420,#8421,#8422));
#1499=EDGE_LOOP('',(#8423,#8424,#8425,#8426));
#1500=EDGE_LOOP('',(#8427,#8428,#8429,#8430));
#1501=EDGE_LOOP('',(#8431,#8432,#8433,#8434));
#1502=EDGE_LOOP('',(#8435,#8436,#8437,#8438));
#1503=EDGE_LOOP('',(#8439,#8440,#8441,#8442));
#1504=EDGE_LOOP('',(#8443,#8444,#8445,#8446));
#1505=EDGE_LOOP('',(#8447,#8448,#8449,#8450));
#1506=EDGE_LOOP('',(#8451,#8452,#8453,#8454));
#1507=EDGE_LOOP('',(#8455,#8456,#8457,#8458));
#1508=EDGE_LOOP('',(#8459,#8460,#8461,#8462));
#1509=EDGE_LOOP('',(#8463,#8464,#8465,#8466));
#1510=EDGE_LOOP('',(#8467,#8468,#8469,#8470,#8471,#8472,#8473,#8474));
#1511=EDGE_LOOP('',(#8475,#8476,#8477,#8478,#8479,#8480,#8481,#8482));
#1512=EDGE_LOOP('',(#8483,#8484,#8485,#8486,#8487,#8488,#8489,#8490));
#1513=EDGE_LOOP('',(#8491,#8492,#8493,#8494,#8495,#8496,#8497,#8498));
#1514=EDGE_LOOP('',(#8499,#8500,#8501,#8502,#8503,#8504,#8505,#8506));
#1515=EDGE_LOOP('',(#8507,#8508,#8509,#8510,#8511,#8512,#8513,#8514));
#1516=EDGE_LOOP('',(#8515,#8516,#8517,#8518,#8519,#8520,#8521,#8522));
#1517=EDGE_LOOP('',(#8523,#8524,#8525,#8526,#8527,#8528,#8529,#8530));
#1518=EDGE_LOOP('',(#8531,#8532,#8533,#8534,#8535,#8536,#8537,#8538));
#1519=EDGE_LOOP('',(#8539,#8540,#8541,#8542,#8543,#8544,#8545,#8546));
#1520=EDGE_LOOP('',(#8547,#8548,#8549,#8550,#8551,#8552,#8553,#8554));
#1521=EDGE_LOOP('',(#8555,#8556,#8557,#8558,#8559,#8560,#8561,#8562));
#1522=EDGE_LOOP('',(#8563,#8564,#8565,#8566,#8567,#8568,#8569,#8570));
#1523=EDGE_LOOP('',(#8571,#8572,#8573,#8574,#8575,#8576,#8577,#8578));
#1524=EDGE_LOOP('',(#8579,#8580,#8581,#8582,#8583,#8584,#8585,#8586));
#1525=EDGE_LOOP('',(#8587,#8588,#8589,#8590,#8591,#8592,#8593,#8594));
#1526=EDGE_LOOP('',(#8595,#8596,#8597,#8598,#8599,#8600,#8601,#8602));
#1527=EDGE_LOOP('',(#8603,#8604,#8605,#8606,#8607,#8608,#8609,#8610));
#1528=EDGE_LOOP('',(#8611,#8612,#8613,#8614,#8615,#8616,#8617,#8618));
#1529=EDGE_LOOP('',(#8619,#8620,#8621,#8622,#8623,#8624,#8625,#8626));
#1530=EDGE_LOOP('',(#8627,#8628,#8629,#8630,#8631,#8632,#8633,#8634));
#1531=EDGE_LOOP('',(#8635,#8636,#8637,#8638,#8639,#8640,#8641,#8642));
#1532=EDGE_LOOP('',(#8643,#8644,#8645,#8646,#8647,#8648,#8649,#8650));
#1533=EDGE_LOOP('',(#8651,#8652,#8653,#8654,#8655,#8656,#8657,#8658));
#1534=EDGE_LOOP('',(#8659,#8660,#8661,#8662,#8663,#8664,#8665,#8666));
#1535=EDGE_LOOP('',(#8667,#8668,#8669,#8670,#8671,#8672,#8673,#8674));
#1536=EDGE_LOOP('',(#8675,#8676,#8677,#8678,#8679,#8680,#8681,#8682));
#1537=EDGE_LOOP('',(#8683,#8684,#8685,#8686,#8687,#8688,#8689,#8690));
#1538=EDGE_LOOP('',(#8691,#8692,#8693,#8694,#8695,#8696,#8697,#8698));
#1539=EDGE_LOOP('',(#8699,#8700,#8701,#8702,#8703,#8704,#8705,#8706));
#1540=EDGE_LOOP('',(#8707,#8708,#8709,#8710,#8711,#8712,#8713,#8714));
#1541=EDGE_LOOP('',(#8715,#8716,#8717,#8718,#8719,#8720,#8721,#8722));
#1542=EDGE_LOOP('',(#8723,#8724,#8725,#8726,#8727,#8728,#8729,#8730));
#1543=EDGE_LOOP('',(#8731,#8732,#8733,#8734,#8735,#8736,#8737,#8738));
#1544=EDGE_LOOP('',(#8739,#8740,#8741,#8742,#8743,#8744,#8745,#8746));
#1545=EDGE_LOOP('',(#8747,#8748,#8749,#8750,#8751,#8752,#8753,#8754));
#1546=EDGE_LOOP('',(#8755,#8756,#8757,#8758));
#1547=EDGE_LOOP('',(#8759,#8760,#8761,#8762));
#1548=EDGE_LOOP('',(#8763,#8764,#8765,#8766));
#1549=EDGE_LOOP('',(#8767,#8768,#8769,#8770));
#1550=EDGE_LOOP('',(#8771,#8772,#8773,#8774));
#1551=EDGE_LOOP('',(#8775,#8776,#8777,#8778));
#1552=EDGE_LOOP('',(#8779,#8780,#8781,#8782));
#1553=EDGE_LOOP('',(#8783,#8784,#8785,#8786));
#1554=EDGE_LOOP('',(#8787,#8788,#8789,#8790));
#1555=EDGE_LOOP('',(#8791,#8792,#8793,#8794));
#1556=EDGE_LOOP('',(#8795,#8796,#8797,#8798));
#1557=EDGE_LOOP('',(#8799,#8800,#8801,#8802));
#1558=EDGE_LOOP('',(#8803,#8804,#8805,#8806));
#1559=EDGE_LOOP('',(#8807,#8808,#8809,#8810));
#1560=EDGE_LOOP('',(#8811,#8812,#8813,#8814));
#1561=EDGE_LOOP('',(#8815,#8816,#8817,#8818));
#1562=EDGE_LOOP('',(#8819,#8820,#8821,#8822));
#1563=EDGE_LOOP('',(#8823,#8824,#8825,#8826));
#1564=EDGE_LOOP('',(#8827,#8828,#8829,#8830));
#1565=EDGE_LOOP('',(#8831,#8832,#8833,#8834));
#1566=EDGE_LOOP('',(#8835,#8836,#8837,#8838));
#1567=EDGE_LOOP('',(#8839,#8840,#8841,#8842));
#1568=EDGE_LOOP('',(#8843,#8844,#8845,#8846));
#1569=EDGE_LOOP('',(#8847,#8848,#8849,#8850));
#1570=EDGE_LOOP('',(#8851,#8852,#8853,#8854));
#1571=EDGE_LOOP('',(#8855,#8856,#8857,#8858));
#1572=EDGE_LOOP('',(#8859,#8860,#8861,#8862));
#1573=EDGE_LOOP('',(#8863,#8864,#8865,#8866));
#1574=EDGE_LOOP('',(#8867,#8868,#8869,#8870));
#1575=EDGE_LOOP('',(#8871,#8872,#8873,#8874));
#1576=EDGE_LOOP('',(#8875,#8876,#8877,#8878));
#1577=EDGE_LOOP('',(#8879,#8880,#8881,#8882));
#1578=EDGE_LOOP('',(#8883,#8884,#8885,#8886));
#1579=EDGE_LOOP('',(#8887,#8888,#8889,#8890));
#1580=EDGE_LOOP('',(#8891,#8892,#8893,#8894));
#1581=EDGE_LOOP('',(#8895,#8896,#8897,#8898));
#1582=EDGE_LOOP('',(#8899,#8900,#8901,#8902));
#1583=EDGE_LOOP('',(#8903,#8904,#8905,#8906));
#1584=EDGE_LOOP('',(#8907,#8908,#8909,#8910));
#1585=EDGE_LOOP('',(#8911,#8912,#8913,#8914));
#1586=EDGE_LOOP('',(#8915,#8916,#8917,#8918));
#1587=EDGE_LOOP('',(#8919,#8920,#8921,#8922));
#1588=EDGE_LOOP('',(#8923,#8924,#8925,#8926));
#1589=EDGE_LOOP('',(#8927,#8928,#8929,#8930));
#1590=EDGE_LOOP('',(#8931,#8932,#8933,#8934));
#1591=EDGE_LOOP('',(#8935,#8936,#8937,#8938));
#1592=EDGE_LOOP('',(#8939,#8940,#8941,#8942));
#1593=EDGE_LOOP('',(#8943,#8944,#8945,#8946));
#1594=EDGE_LOOP('',(#8947,#8948,#8949,#8950));
#1595=EDGE_LOOP('',(#8951,#8952,#8953,#8954));
#1596=EDGE_LOOP('',(#8955,#8956,#8957,#8958));
#1597=EDGE_LOOP('',(#8959,#8960,#8961,#8962));
#1598=EDGE_LOOP('',(#8963,#8964,#8965,#8966));
#1599=EDGE_LOOP('',(#8967,#8968,#8969,#8970));
#1600=EDGE_LOOP('',(#8971,#8972,#8973,#8974));
#1601=EDGE_LOOP('',(#8975,#8976,#8977,#8978));
#1602=EDGE_LOOP('',(#8979,#8980,#8981,#8982));
#1603=EDGE_LOOP('',(#8983,#8984,#8985,#8986));
#1604=EDGE_LOOP('',(#8987,#8988,#8989,#8990));
#1605=EDGE_LOOP('',(#8991,#8992,#8993,#8994));
#1606=EDGE_LOOP('',(#8995,#8996,#8997,#8998));
#1607=EDGE_LOOP('',(#8999,#9000,#9001,#9002));
#1608=EDGE_LOOP('',(#9003,#9004,#9005,#9006));
#1609=EDGE_LOOP('',(#9007,#9008,#9009,#9010));
#1610=EDGE_LOOP('',(#9011,#9012,#9013,#9014));
#1611=EDGE_LOOP('',(#9015,#9016,#9017,#9018));
#1612=EDGE_LOOP('',(#9019,#9020,#9021,#9022));
#1613=EDGE_LOOP('',(#9023,#9024,#9025,#9026));
#1614=EDGE_LOOP('',(#9027,#9028,#9029,#9030));
#1615=EDGE_LOOP('',(#9031,#9032,#9033,#9034));
#1616=EDGE_LOOP('',(#9035,#9036,#9037,#9038));
#1617=EDGE_LOOP('',(#9039,#9040,#9041,#9042));
#1618=EDGE_LOOP('',(#9043,#9044,#9045,#9046));
#1619=EDGE_LOOP('',(#9047,#9048,#9049,#9050));
#1620=EDGE_LOOP('',(#9051,#9052,#9053,#9054));
#1621=EDGE_LOOP('',(#9055,#9056,#9057,#9058));
#1622=EDGE_LOOP('',(#9059,#9060,#9061,#9062));
#1623=EDGE_LOOP('',(#9063,#9064,#9065,#9066));
#1624=EDGE_LOOP('',(#9067,#9068,#9069,#9070));
#1625=EDGE_LOOP('',(#9071,#9072,#9073,#9074));
#1626=EDGE_LOOP('',(#9075,#9076,#9077,#9078));
#1627=EDGE_LOOP('',(#9079,#9080,#9081,#9082));
#1628=EDGE_LOOP('',(#9083,#9084,#9085,#9086));
#1629=EDGE_LOOP('',(#9087,#9088,#9089,#9090));
#1630=EDGE_LOOP('',(#9091,#9092,#9093,#9094));
#1631=EDGE_LOOP('',(#9095,#9096,#9097,#9098));
#1632=EDGE_LOOP('',(#9099,#9100,#9101,#9102));
#1633=EDGE_LOOP('',(#9103,#9104,#9105,#9106));
#1634=EDGE_LOOP('',(#9107,#9108,#9109,#9110));
#1635=EDGE_LOOP('',(#9111,#9112,#9113,#9114));
#1636=EDGE_LOOP('',(#9115,#9116,#9117,#9118,#9119,#9120,#9121,#9122,#9123,
#9124));
#1637=EDGE_LOOP('',(#9125,#9126,#9127,#9128,#9129,#9130,#9131,#9132,#9133,
#9134));
#1638=EDGE_LOOP('',(#9135,#9136,#9137,#9138));
#1639=EDGE_LOOP('',(#9139,#9140,#9141,#9142));
#1640=EDGE_LOOP('',(#9143,#9144,#9145,#9146,#9147,#9148,#9149,#9150,#9151,
#9152));
#1641=EDGE_LOOP('',(#9153,#9154,#9155,#9156,#9157,#9158,#9159,#9160,#9161,
#9162));
#1642=EDGE_LOOP('',(#9163,#9164,#9165,#9166));
#1643=EDGE_LOOP('',(#9167,#9168,#9169,#9170));
#1644=EDGE_LOOP('',(#9171,#9172,#9173,#9174,#9175,#9176,#9177,#9178,#9179,
#9180));
#1645=EDGE_LOOP('',(#9181,#9182,#9183,#9184,#9185,#9186,#9187,#9188,#9189,
#9190));
#1646=EDGE_LOOP('',(#9191,#9192,#9193,#9194));
#1647=EDGE_LOOP('',(#9195,#9196,#9197,#9198));
#1648=EDGE_LOOP('',(#9199,#9200,#9201,#9202,#9203,#9204,#9205,#9206,#9207,
#9208));
#1649=EDGE_LOOP('',(#9209,#9210,#9211,#9212,#9213,#9214,#9215,#9216,#9217,
#9218));
#1650=EDGE_LOOP('',(#9219,#9220,#9221,#9222));
#1651=EDGE_LOOP('',(#9223,#9224,#9225,#9226));
#1652=EDGE_LOOP('',(#9227,#9228,#9229,#9230,#9231,#9232,#9233,#9234,#9235,
#9236));
#1653=EDGE_LOOP('',(#9237,#9238,#9239,#9240,#9241,#9242,#9243,#9244,#9245,
#9246));
#1654=EDGE_LOOP('',(#9247,#9248,#9249,#9250));
#1655=EDGE_LOOP('',(#9251,#9252,#9253,#9254));
#1656=EDGE_LOOP('',(#9255,#9256,#9257,#9258,#9259,#9260,#9261,#9262,#9263,
#9264));
#1657=EDGE_LOOP('',(#9265,#9266,#9267,#9268,#9269,#9270,#9271,#9272,#9273,
#9274));
#1658=EDGE_LOOP('',(#9275,#9276,#9277,#9278));
#1659=EDGE_LOOP('',(#9279,#9280,#9281,#9282));
#1660=EDGE_LOOP('',(#9283,#9284,#9285,#9286,#9287,#9288,#9289,#9290,#9291,
#9292));
#1661=EDGE_LOOP('',(#9293,#9294,#9295,#9296,#9297,#9298,#9299,#9300,#9301,
#9302));
#1662=EDGE_LOOP('',(#9303,#9304,#9305,#9306));
#1663=EDGE_LOOP('',(#9307,#9308,#9309,#9310));
#1664=EDGE_LOOP('',(#9311,#9312,#9313,#9314,#9315,#9316,#9317,#9318,#9319,
#9320));
#1665=EDGE_LOOP('',(#9321,#9322,#9323,#9324,#9325,#9326,#9327,#9328,#9329,
#9330));
#1666=EDGE_LOOP('',(#9331,#9332,#9333,#9334));
#1667=EDGE_LOOP('',(#9335,#9336,#9337,#9338));
#1668=EDGE_LOOP('',(#9339,#9340,#9341,#9342,#9343,#9344,#9345,#9346,#9347,
#9348));
#1669=EDGE_LOOP('',(#9349,#9350,#9351,#9352,#9353,#9354,#9355,#9356,#9357,
#9358));
#1670=EDGE_LOOP('',(#9359,#9360,#9361,#9362));
#1671=EDGE_LOOP('',(#9363,#9364,#9365,#9366));
#1672=EDGE_LOOP('',(#9367,#9368,#9369,#9370,#9371,#9372,#9373,#9374,#9375,
#9376));
#1673=EDGE_LOOP('',(#9377,#9378,#9379,#9380,#9381,#9382,#9383,#9384,#9385,
#9386));
#1674=EDGE_LOOP('',(#9387,#9388,#9389,#9390));
#1675=EDGE_LOOP('',(#9391,#9392,#9393,#9394));
#1676=EDGE_LOOP('',(#9395,#9396,#9397,#9398,#9399,#9400,#9401,#9402,#9403,
#9404));
#1677=EDGE_LOOP('',(#9405,#9406,#9407,#9408,#9409,#9410,#9411,#9412,#9413,
#9414));
#1678=EDGE_LOOP('',(#9415,#9416,#9417,#9418));
#1679=EDGE_LOOP('',(#9419,#9420,#9421,#9422));
#1680=EDGE_LOOP('',(#9423,#9424,#9425,#9426,#9427,#9428,#9429,#9430,#9431,
#9432));
#1681=EDGE_LOOP('',(#9433,#9434,#9435,#9436,#9437,#9438,#9439,#9440,#9441,
#9442));
#1682=EDGE_LOOP('',(#9443,#9444,#9445,#9446));
#1683=EDGE_LOOP('',(#9447,#9448,#9449,#9450));
#1684=EDGE_LOOP('',(#9451,#9452,#9453,#9454,#9455,#9456,#9457,#9458,#9459,
#9460));
#1685=EDGE_LOOP('',(#9461,#9462,#9463,#9464,#9465,#9466,#9467,#9468,#9469,
#9470));
#1686=EDGE_LOOP('',(#9471,#9472,#9473,#9474));
#1687=EDGE_LOOP('',(#9475,#9476,#9477,#9478));
#1688=EDGE_LOOP('',(#9479,#9480,#9481,#9482,#9483,#9484,#9485,#9486,#9487,
#9488));
#1689=EDGE_LOOP('',(#9489,#9490,#9491,#9492,#9493,#9494,#9495,#9496,#9497,
#9498));
#1690=EDGE_LOOP('',(#9499,#9500,#9501,#9502));
#1691=EDGE_LOOP('',(#9503,#9504,#9505,#9506));
#1692=EDGE_LOOP('',(#9507,#9508,#9509,#9510,#9511,#9512,#9513,#9514,#9515,
#9516));
#1693=EDGE_LOOP('',(#9517,#9518,#9519,#9520,#9521,#9522,#9523,#9524,#9525,
#9526));
#1694=EDGE_LOOP('',(#9527,#9528,#9529,#9530));
#1695=EDGE_LOOP('',(#9531,#9532,#9533,#9534));
#1696=EDGE_LOOP('',(#9535,#9536,#9537,#9538,#9539,#9540,#9541,#9542,#9543,
#9544));
#1697=EDGE_LOOP('',(#9545,#9546,#9547,#9548,#9549,#9550,#9551,#9552,#9553,
#9554));
#1698=EDGE_LOOP('',(#9555,#9556,#9557,#9558));
#1699=EDGE_LOOP('',(#9559,#9560,#9561,#9562));
#1700=EDGE_LOOP('',(#9563,#9564,#9565,#9566,#9567,#9568,#9569,#9570,#9571,
#9572));
#1701=EDGE_LOOP('',(#9573,#9574,#9575,#9576,#9577,#9578,#9579,#9580,#9581,
#9582));
#1702=EDGE_LOOP('',(#9583,#9584,#9585,#9586));
#1703=EDGE_LOOP('',(#9587,#9588,#9589,#9590));
#1704=EDGE_LOOP('',(#9591,#9592,#9593,#9594,#9595,#9596,#9597,#9598,#9599,
#9600));
#1705=EDGE_LOOP('',(#9601,#9602,#9603,#9604,#9605,#9606,#9607,#9608,#9609,
#9610));
#1706=EDGE_LOOP('',(#9611,#9612,#9613,#9614));
#1707=EDGE_LOOP('',(#9615,#9616,#9617,#9618));
#1708=EDGE_LOOP('',(#9619,#9620,#9621,#9622,#9623,#9624));
#1709=EDGE_LOOP('',(#9625,#9626,#9627,#9628));
#1710=EDGE_LOOP('',(#9629,#9630,#9631,#9632,#9633,#9634));
#1711=EDGE_LOOP('',(#9635,#9636,#9637,#9638));
#1712=EDGE_LOOP('',(#9639,#9640,#9641,#9642));
#1713=EDGE_LOOP('',(#9643,#9644,#9645,#9646,#9647,#9648));
#1714=EDGE_LOOP('',(#9649,#9650,#9651,#9652,#9653,#9654));
#1715=EDGE_LOOP('',(#9655,#9656,#9657,#9658));
#1716=EDGE_LOOP('',(#9659,#9660,#9661,#9662,#9663,#9664));
#1717=EDGE_LOOP('',(#9665,#9666,#9667,#9668,#9669,#9670));
#1718=EDGE_LOOP('',(#9671,#9672,#9673,#9674));
#1719=EDGE_LOOP('',(#9675,#9676,#9677,#9678,#9679,#9680,#9681,#9682,#9683,
#9684,#9685,#9686,#9687,#9688,#9689,#9690,#9691,#9692,#9693,#9694,#9695,
#9696,#9697,#9698,#9699,#9700,#9701,#9702,#9703,#9704,#9705,#9706,#9707,
#9708,#9709,#9710,#9711,#9712,#9713,#9714,#9715,#9716,#9717,#9718,#9719,
#9720,#9721,#9722,#9723,#9724,#9725,#9726,#9727,#9728,#9729,#9730,#9731,
#9732,#9733,#9734,#9735,#9736,#9737,#9738,#9739,#9740,#9741,#9742,#9743,
#9744,#9745,#9746));
#1720=EDGE_LOOP('',(#9747,#9748,#9749,#9750,#9751));
#1721=EDGE_LOOP('',(#9752,#9753,#9754,#9755));
#1722=EDGE_LOOP('',(#9756,#9757,#9758,#9759,#9760,#9761));
#1723=EDGE_LOOP('',(#9762,#9763,#9764,#9765));
#1724=EDGE_LOOP('',(#9766,#9767,#9768,#9769,#9770,#9771));
#1725=EDGE_LOOP('',(#9772,#9773,#9774,#9775));
#1726=EDGE_LOOP('',(#9776,#9777,#9778,#9779));
#1727=EDGE_LOOP('',(#9780,#9781,#9782,#9783,#9784,#9785));
#1728=EDGE_LOOP('',(#9786,#9787,#9788,#9789,#9790,#9791));
#1729=EDGE_LOOP('',(#9792,#9793,#9794,#9795));
#1730=EDGE_LOOP('',(#9796,#9797,#9798,#9799,#9800,#9801));
#1731=EDGE_LOOP('',(#9802,#9803,#9804,#9805,#9806,#9807));
#1732=EDGE_LOOP('',(#9808,#9809,#9810,#9811));
#1733=EDGE_LOOP('',(#9812,#9813,#9814,#9815));
#1734=EDGE_LOOP('',(#9816,#9817,#9818,#9819,#9820,#9821));
#1735=EDGE_LOOP('',(#9822,#9823,#9824,#9825));
#1736=EDGE_LOOP('',(#9826,#9827,#9828,#9829,#9830,#9831));
#1737=EDGE_LOOP('',(#9832,#9833,#9834,#9835));
#1738=EDGE_LOOP('',(#9836,#9837,#9838,#9839));
#1739=EDGE_LOOP('',(#9840,#9841,#9842,#9843,#9844,#9845));
#1740=EDGE_LOOP('',(#9846,#9847,#9848,#9849,#9850,#9851));
#1741=EDGE_LOOP('',(#9852,#9853,#9854,#9855));
#1742=EDGE_LOOP('',(#9856,#9857,#9858,#9859,#9860,#9861));
#1743=EDGE_LOOP('',(#9862,#9863,#9864,#9865,#9866,#9867));
#1744=EDGE_LOOP('',(#9868,#9869,#9870,#9871));
#1745=EDGE_LOOP('',(#9872,#9873,#9874,#9875));
#1746=EDGE_LOOP('',(#9876,#9877,#9878,#9879,#9880,#9881));
#1747=EDGE_LOOP('',(#9882,#9883,#9884,#9885));
#1748=EDGE_LOOP('',(#9886,#9887,#9888,#9889,#9890,#9891));
#1749=EDGE_LOOP('',(#9892,#9893,#9894,#9895));
#1750=EDGE_LOOP('',(#9896,#9897,#9898,#9899));
#1751=EDGE_LOOP('',(#9900,#9901,#9902,#9903,#9904,#9905));
#1752=EDGE_LOOP('',(#9906,#9907,#9908,#9909,#9910,#9911));
#1753=EDGE_LOOP('',(#9912,#9913,#9914,#9915));
#1754=EDGE_LOOP('',(#9916,#9917,#9918,#9919,#9920,#9921));
#1755=EDGE_LOOP('',(#9922,#9923,#9924,#9925,#9926,#9927));
#1756=EDGE_LOOP('',(#9928,#9929,#9930,#9931));
#1757=EDGE_LOOP('',(#9932,#9933,#9934,#9935));
#1758=EDGE_LOOP('',(#9936,#9937,#9938,#9939,#9940,#9941));
#1759=EDGE_LOOP('',(#9942,#9943,#9944,#9945));
#1760=EDGE_LOOP('',(#9946,#9947,#9948,#9949,#9950,#9951));
#1761=EDGE_LOOP('',(#9952,#9953,#9954,#9955));
#1762=EDGE_LOOP('',(#9956,#9957,#9958,#9959));
#1763=EDGE_LOOP('',(#9960,#9961,#9962,#9963,#9964,#9965));
#1764=EDGE_LOOP('',(#9966,#9967,#9968,#9969,#9970,#9971));
#1765=EDGE_LOOP('',(#9972,#9973,#9974,#9975));
#1766=EDGE_LOOP('',(#9976,#9977,#9978,#9979,#9980,#9981));
#1767=EDGE_LOOP('',(#9982,#9983,#9984,#9985,#9986,#9987));
#1768=EDGE_LOOP('',(#9988,#9989,#9990,#9991));
#1769=EDGE_LOOP('',(#9992,#9993,#9994,#9995));
#1770=EDGE_LOOP('',(#9996,#9997,#9998,#9999,#10000,#10001));
#1771=EDGE_LOOP('',(#10002,#10003,#10004,#10005));
#1772=EDGE_LOOP('',(#10006,#10007,#10008,#10009,#10010,#10011));
#1773=EDGE_LOOP('',(#10012,#10013,#10014,#10015));
#1774=EDGE_LOOP('',(#10016,#10017,#10018,#10019));
#1775=EDGE_LOOP('',(#10020,#10021,#10022,#10023,#10024,#10025));
#1776=EDGE_LOOP('',(#10026,#10027,#10028,#10029,#10030,#10031));
#1777=EDGE_LOOP('',(#10032,#10033,#10034,#10035));
#1778=EDGE_LOOP('',(#10036,#10037,#10038,#10039,#10040,#10041));
#1779=EDGE_LOOP('',(#10042,#10043,#10044,#10045,#10046,#10047));
#1780=EDGE_LOOP('',(#10048,#10049,#10050,#10051));
#1781=EDGE_LOOP('',(#10052,#10053,#10054,#10055));
#2221=CIRCLE('',#13130,8.12525);
#2222=CIRCLE('',#13142,8.12525);
#2223=CIRCLE('',#13144,7.01125);
#2224=CIRCLE('',#13156,7.01125);
#2225=CIRCLE('',#13160,15.9979895488606);
#2226=CIRCLE('',#13161,15.5);
#2227=CIRCLE('',#13162,15.9979895488606);
#2228=CIRCLE('',#13163,15.5);
#2229=CIRCLE('',#13164,15.9979895488606);
#2230=CIRCLE('',#13165,15.5);
#2231=CIRCLE('',#13166,15.9979895488606);
#2232=CIRCLE('',#13167,15.5);
#2233=CIRCLE('',#13168,15.9979895488606);
#2234=CIRCLE('',#13169,15.5);
#2235=CIRCLE('',#13170,15.9979895488606);
#2236=CIRCLE('',#13171,15.5);
#2237=CIRCLE('',#13172,15.9979895488606);
#2238=CIRCLE('',#13173,15.5);
#2239=CIRCLE('',#13174,15.9979895488606);
#2240=CIRCLE('',#13175,15.5);
#2241=CIRCLE('',#13176,15.9979895488606);
#2242=CIRCLE('',#13177,15.5);
#2243=CIRCLE('',#13178,15.9979895488606);
#2244=CIRCLE('',#13179,15.5);
#2245=CIRCLE('',#13180,15.9979895488606);
#2246=CIRCLE('',#13181,15.5);
#2247=CIRCLE('',#13182,15.9979895488606);
#2248=CIRCLE('',#13183,15.5);
#2249=CIRCLE('',#13184,15.9979895488606);
#2250=CIRCLE('',#13185,15.5);
#2251=CIRCLE('',#13186,15.9979895488606);
#2252=CIRCLE('',#13187,15.5);
#2253=CIRCLE('',#13188,15.9979895488606);
#2254=CIRCLE('',#13189,15.5);
#2255=CIRCLE('',#13190,15.9979895488606);
#2256=CIRCLE('',#13191,15.5);
#2257=CIRCLE('',#13192,15.9979895488606);
#2258=CIRCLE('',#13193,15.5);
#2259=CIRCLE('',#13194,15.9979895488606);
#2260=CIRCLE('',#13195,15.5);
#2261=CIRCLE('',#13197,19.9979895488606);
#2262=CIRCLE('',#13198,20.0030144756463);
#2263=CIRCLE('',#13200,19.9979895488606);
#2264=CIRCLE('',#13201,20.0030144756504);
#2265=CIRCLE('',#13203,19.9979895488606);
#2266=CIRCLE('',#13204,20.0030144756628);
#2267=CIRCLE('',#13206,19.9979895488606);
#2268=CIRCLE('',#13207,20.0030144756547);
#2269=CIRCLE('',#13209,19.9979895488606);
#2270=CIRCLE('',#13210,20.0030144756757);
#2271=CIRCLE('',#13212,19.9979895488606);
#2272=CIRCLE('',#13213,20.003014475647);
#2273=CIRCLE('',#13215,19.9979895488606);
#2274=CIRCLE('',#13216,20.0030144756693);
#2275=CIRCLE('',#13218,19.9979895488606);
#2276=CIRCLE('',#13219,20.0030144756498);
#2277=CIRCLE('',#13221,19.9979895488606);
#2278=CIRCLE('',#13222,20.0030144756644);
#2279=CIRCLE('',#13224,19.9979895488606);
#2280=CIRCLE('',#13225,20.0030144756482);
#2281=CIRCLE('',#13227,19.9979895488606);
#2282=CIRCLE('',#13228,20.0030144756504);
#2283=CIRCLE('',#13230,19.9979895488606);
#2284=CIRCLE('',#13231,20.0030144756643);
#2285=CIRCLE('',#13233,19.9979895488606);
#2286=CIRCLE('',#13234,20.0030144756551);
#2287=CIRCLE('',#13236,19.9979895488606);
#2288=CIRCLE('',#13237,20.003014475638);
#2289=CIRCLE('',#13239,19.9979895488606);
#2290=CIRCLE('',#13240,20.0030144756176);
#2291=CIRCLE('',#13242,19.9979895488606);
#2292=CIRCLE('',#13243,20.0030144756693);
#2293=CIRCLE('',#13245,19.9979895488606);
#2294=CIRCLE('',#13246,20.0030144756499);
#2295=CIRCLE('',#13248,19.9979895488606);
#2296=CIRCLE('',#13249,20.0030144756645);
#2297=CIRCLE('',#13251,153.58770900085);
#2298=CIRCLE('',#13252,153.587709001305);
#2299=CIRCLE('',#13254,153.587709000006);
#2300=CIRCLE('',#13255,153.587709000986);
#2301=CIRCLE('',#13257,153.587709000895);
#2302=CIRCLE('',#13258,153.587709000364);
#2303=CIRCLE('',#13260,153.587709000872);
#2304=CIRCLE('',#13261,153.587709001053);
#2305=CIRCLE('',#13263,153.587709000643);
#2306=CIRCLE('',#13264,153.587709000849);
#2307=CIRCLE('',#13266,153.587709004083);
#2308=CIRCLE('',#13267,153.587709001836);
#2309=CIRCLE('',#13269,153.5877090017);
#2310=CIRCLE('',#13270,153.587709001977);
#2311=CIRCLE('',#13272,153.587709000674);
#2312=CIRCLE('',#13273,153.587709000286);
#2313=CIRCLE('',#13275,153.58770900064);
#2314=CIRCLE('',#13276,153.587709001091);
#2315=CIRCLE('',#13278,153.587709000099);
#2316=CIRCLE('',#13279,153.587709001243);
#2317=CIRCLE('',#13281,153.587709001448);
#2318=CIRCLE('',#13282,153.587709000446);
#2319=CIRCLE('',#13284,153.587709000445);
#2320=CIRCLE('',#13285,153.587709000972);
#2321=CIRCLE('',#13287,153.587709000937);
#2322=CIRCLE('',#13288,153.587709001348);
#2323=CIRCLE('',#13290,153.587709001259);
#2324=CIRCLE('',#13291,153.587709000715);
#2325=CIRCLE('',#13293,153.587709001696);
#2326=CIRCLE('',#13294,153.587709001411);
#2327=CIRCLE('',#13296,153.587709001257);
#2328=CIRCLE('',#13297,153.587709000945);
#2329=CIRCLE('',#13299,153.587709001131);
#2330=CIRCLE('',#13300,153.58770900096);
#2331=CIRCLE('',#13302,153.587709000845);
#2332=CIRCLE('',#13303,153.587709000983);
#2333=CIRCLE('',#13305,153.587709001349);
#2334=CIRCLE('',#13306,15.9979895488606);
#2335=CIRCLE('',#13307,153.587709000931);
#2336=CIRCLE('',#13308,19.9979895488606);
#2337=CIRCLE('',#13310,153.587709001089);
#2338=CIRCLE('',#13311,15.9979895488606);
#2339=CIRCLE('',#13312,153.587709001593);
#2340=CIRCLE('',#13313,19.9979895488606);
#2341=CIRCLE('',#13315,153.587709000602);
#2342=CIRCLE('',#13316,15.9979895488606);
#2343=CIRCLE('',#13317,153.587709000574);
#2344=CIRCLE('',#13318,19.9979895488606);
#2345=CIRCLE('',#13320,153.587709001501);
#2346=CIRCLE('',#13321,15.9979895488606);
#2347=CIRCLE('',#13322,153.587709000733);
#2348=CIRCLE('',#13323,19.9979895488606);
#2349=CIRCLE('',#13325,153.587709001334);
#2350=CIRCLE('',#13326,15.9979895488606);
#2351=CIRCLE('',#13327,153.587709000931);
#2352=CIRCLE('',#13328,19.9979895488606);
#2353=CIRCLE('',#13330,153.587709000819);
#2354=CIRCLE('',#13331,15.9979895488606);
#2355=CIRCLE('',#13332,153.587709001092);
#2356=CIRCLE('',#13333,19.9979895488606);
#2357=CIRCLE('',#13335,153.587709000441);
#2358=CIRCLE('',#13336,15.9979895488606);
#2359=CIRCLE('',#13337,153.587709000835);
#2360=CIRCLE('',#13338,19.9979895488606);
#2361=CIRCLE('',#13340,153.587708999976);
#2362=CIRCLE('',#13341,15.9979895488606);
#2363=CIRCLE('',#13342,153.587709002011);
#2364=CIRCLE('',#13343,19.9979895488606);
#2365=CIRCLE('',#13345,153.587709000862);
#2366=CIRCLE('',#13346,15.9979895488606);
#2367=CIRCLE('',#13347,153.587709000429);
#2368=CIRCLE('',#13348,19.9979895488606);
#2369=CIRCLE('',#13350,153.587709000768);
#2370=CIRCLE('',#13351,15.9979895488606);
#2371=CIRCLE('',#13352,153.587709000924);
#2372=CIRCLE('',#13353,19.9979895488606);
#2373=CIRCLE('',#13355,153.587709001594);
#2374=CIRCLE('',#13356,15.9979895488606);
#2375=CIRCLE('',#13357,153.587709001193);
#2376=CIRCLE('',#13358,19.9979895488606);
#2377=CIRCLE('',#13360,153.587708999931);
#2378=CIRCLE('',#13361,15.9979895488606);
#2379=CIRCLE('',#13362,153.587709001467);
#2380=CIRCLE('',#13363,19.9979895488606);
#2381=CIRCLE('',#13365,153.587709001247);
#2382=CIRCLE('',#13366,15.9979895488606);
#2383=CIRCLE('',#13367,153.587709000706);
#2384=CIRCLE('',#13368,19.9979895488606);
#2385=CIRCLE('',#13370,153.587709001118);
#2386=CIRCLE('',#13371,15.9979895488606);
#2387=CIRCLE('',#13372,153.587709000915);
#2388=CIRCLE('',#13373,19.9979895488606);
#2389=CIRCLE('',#13375,153.587709000848);
#2390=CIRCLE('',#13376,15.9979895488606);
#2391=CIRCLE('',#13377,153.587709000911);
#2392=CIRCLE('',#13378,19.9979895488606);
#2393=CIRCLE('',#13380,153.587709000116);
#2394=CIRCLE('',#13381,15.9979895488606);
#2395=CIRCLE('',#13382,153.587709000787);
#2396=CIRCLE('',#13383,19.9979895488606);
#2397=CIRCLE('',#13385,153.587709000229);
#2398=CIRCLE('',#13386,15.9979895488606);
#2399=CIRCLE('',#13387,153.587709001888);
#2400=CIRCLE('',#13388,19.9979895488606);
#2401=CIRCLE('',#13390,153.587709000873);
#2402=CIRCLE('',#13391,15.9979895488606);
#2403=CIRCLE('',#13392,153.587709000422);
#2404=CIRCLE('',#13393,19.9979895488606);
#2405=CIRCLE('',#13395,20.0030144756182);
#2406=CIRCLE('',#13397,20.0030144756451);
#2407=CIRCLE('',#13399,20.0030144756147);
#2408=CIRCLE('',#13401,20.0030144756611);
#2409=CIRCLE('',#13403,20.0030144756232);
#2410=CIRCLE('',#13405,20.0030144756284);
#2411=CIRCLE('',#13407,20.0030144756652);
#2412=CIRCLE('',#13409,20.0030144756486);
#2413=CIRCLE('',#13411,20.0030144756281);
#2414=CIRCLE('',#13413,20.0030144756182);
#2415=CIRCLE('',#13415,20.0030144756466);
#2416=CIRCLE('',#13417,20.003014475679);
#2417=CIRCLE('',#13419,20.0030144756625);
#2418=CIRCLE('',#13421,20.0030144756237);
#2419=CIRCLE('',#13423,20.003014475629);
#2420=CIRCLE('',#13425,20.0030144756642);
#2421=CIRCLE('',#13427,20.0030144756486);
#2422=CIRCLE('',#13429,20.0030144756277);
#2423=CIRCLE('',#13432,20.0030144756662);
#2424=CIRCLE('',#13433,19.9140934904867);
#2425=CIRCLE('',#13436,20.0030144756255);
#2426=CIRCLE('',#13438,19.9140934904867);
#2427=CIRCLE('',#13441,20.0030144756289);
#2428=CIRCLE('',#13443,19.9140934904867);
#2429=CIRCLE('',#13446,20.0030144756142);
#2430=CIRCLE('',#13447,19.9140934904867);
#2431=CIRCLE('',#13450,20.0030144756439);
#2432=CIRCLE('',#13452,19.9140934904867);
#2433=CIRCLE('',#13455,20.0030144756117);
#2434=CIRCLE('',#13457,19.9140934904867);
#2435=CIRCLE('',#13460,20.0030144756195);
#2436=CIRCLE('',#13462,19.9140934904867);
#2437=CIRCLE('',#13465,20.003014475617);
#2438=CIRCLE('',#13466,19.9140934904867);
#2439=CIRCLE('',#13469,20.0030144756512);
#2440=CIRCLE('',#13471,19.9140934904867);
#2441=CIRCLE('',#13474,20.0030144756233);
#2442=CIRCLE('',#13476,19.9140934904867);
#2443=CIRCLE('',#13479,20.0030144756255);
#2444=CIRCLE('',#13481,19.9140934904867);
#2445=CIRCLE('',#13484,20.0030144756289);
#2446=CIRCLE('',#13485,19.9140934904867);
#2447=CIRCLE('',#13488,20.0030144756141);
#2448=CIRCLE('',#13490,19.9140934904867);
#2449=CIRCLE('',#13493,20.0030144756447);
#2450=CIRCLE('',#13495,19.9140934904867);
#2451=CIRCLE('',#13498,20.003014475657);
#2452=CIRCLE('',#13500,19.9140934904867);
#2453=CIRCLE('',#13503,20.0030144756171);
#2454=CIRCLE('',#13505,19.9140934904867);
#2455=CIRCLE('',#13508,20.0030144756463);
#2456=CIRCLE('',#13509,19.9140934904867);
#2457=CIRCLE('',#13512,20.003014475691);
#2458=CIRCLE('',#13513,19.9140934904867);
#2459=CIRCLE('',#13515,19.9140934904867);
#2460=CIRCLE('',#13517,20.0030144756501);
#2461=CIRCLE('',#13519,19.9140934904867);
#2462=CIRCLE('',#13521,20.0030144756426);
#2463=CIRCLE('',#13523,19.9140934904867);
#2464=CIRCLE('',#13525,20.0030144756575);
#2465=CIRCLE('',#13527,19.9140934904867);
#2466=CIRCLE('',#13529,20.0030144756947);
#2467=CIRCLE('',#13531,19.9140934904867);
#2468=CIRCLE('',#13533,20.0030144756567);
#2469=CIRCLE('',#13535,19.9140934904867);
#2470=CIRCLE('',#13537,20.0030144756689);
#2471=CIRCLE('',#13539,19.9140934904867);
#2472=CIRCLE('',#13541,20.0030144756252);
#2473=CIRCLE('',#13543,19.9140934904867);
#2474=CIRCLE('',#13545,20.0030144756634);
#2475=CIRCLE('',#13547,19.9140934904867);
#2476=CIRCLE('',#13549,20.0030144756389);
#2477=CIRCLE('',#13551,19.9140934904867);
#2478=CIRCLE('',#13553,20.0030144756501);
#2479=CIRCLE('',#13555,19.9140934904867);
#2480=CIRCLE('',#13557,20.003014475641);
#2481=CIRCLE('',#13559,19.9140934904867);
#2482=CIRCLE('',#13561,20.0030144756575);
#2483=CIRCLE('',#13563,19.9140934904867);
#2484=CIRCLE('',#13565,20.0030144756939);
#2485=CIRCLE('',#13567,19.9140934904867);
#2486=CIRCLE('',#13569,20.0030144756567);
#2487=CIRCLE('',#13571,19.9140934904867);
#2488=CIRCLE('',#13573,20.00301447567);
#2489=CIRCLE('',#13575,19.9140934904867);
#2490=CIRCLE('',#13577,20.0030144756496);
#2491=CIRCLE('',#13579,19.9140934904867);
#2492=CIRCLE('',#13581,20.0030144756634);
#2493=CIRCLE('',#13583,19.9140934904867);
#2494=CIRCLE('',#13585,20.0030144756377);
#2495=CIRCLE('',#13604,1187.25159941003);
#2496=CIRCLE('',#13605,1187.25159940698);
#2497=CIRCLE('',#13606,1187.25159941794);
#2498=CIRCLE('',#13607,1187.25159940193);
#2499=CIRCLE('',#13608,1187.25159944622);
#2500=CIRCLE('',#13609,1187.2515994077);
#2501=CIRCLE('',#13610,1187.25159945662);
#2502=CIRCLE('',#13611,1187.2515994434);
#2503=CIRCLE('',#13612,1187.25159941087);
#2504=CIRCLE('',#13613,1187.2515994045);
#2505=CIRCLE('',#13614,1187.25365514628);
#2506=CIRCLE('',#13615,1187.25431298417);
#2507=CIRCLE('',#13616,1187.25159941029);
#2508=CIRCLE('',#13617,1187.2515994038);
#2509=CIRCLE('',#13618,1187.25365511458);
#2510=CIRCLE('',#13619,1187.25431295325);
#2511=CIRCLE('',#13620,1187.25159942133);
#2512=CIRCLE('',#13621,1187.25159939926);
#2513=CIRCLE('',#13622,1187.25365512903);
#2514=CIRCLE('',#13623,1187.2543129837);
#2515=CIRCLE('',#13624,1187.2515994291);
#2516=CIRCLE('',#13625,1187.25159943443);
#2517=CIRCLE('',#13626,1187.25365512723);
#2518=CIRCLE('',#13627,1187.25431299336);
#2519=CIRCLE('',#13628,1187.25159941435);
#2520=CIRCLE('',#13629,1187.25159942688);
#2521=CIRCLE('',#13630,1187.25159941979);
#2522=CIRCLE('',#13631,1187.25159941986);
#2523=CIRCLE('',#13632,1187.25159943305);
#2524=CIRCLE('',#13633,1187.2515994192);
#2525=CIRCLE('',#13634,1187.25365512172);
#2526=CIRCLE('',#13635,1187.25431297033);
#2527=CIRCLE('',#13636,1187.2515994132);
#2528=CIRCLE('',#13637,1187.25159939511);
#2529=CIRCLE('',#13638,1187.25365511663);
#2530=CIRCLE('',#13639,1187.25431293833);
#2531=CIRCLE('',#13640,1187.25159941033);
#2532=CIRCLE('',#13641,1187.25159940711);
#2533=CIRCLE('',#13642,1187.25365511087);
#2534=CIRCLE('',#13643,1187.25431299739);
#2535=CIRCLE('',#13644,1187.25159944517);
#2536=CIRCLE('',#13645,1187.25159940862);
#2537=CIRCLE('',#13646,1187.25159943111);
#2538=CIRCLE('',#13647,1187.25159944031);
#2539=CIRCLE('',#13648,1187.25159941049);
#2540=CIRCLE('',#13649,1187.25159940449);
#2541=CIRCLE('',#13650,1187.25365511182);
#2542=CIRCLE('',#13651,1187.25431298523);
#2543=CIRCLE('',#13652,1187.25159941186);
#2544=CIRCLE('',#13653,1187.2515994023);
#2545=CIRCLE('',#13654,1187.2536551145);
#2546=CIRCLE('',#13655,1187.25431297681);
#2547=CIRCLE('',#13656,1187.25159942333);
#2548=CIRCLE('',#13657,1187.25159939856);
#2549=CIRCLE('',#13658,1187.25365512919);
#2550=CIRCLE('',#13659,1187.25431298215);
#2551=CIRCLE('',#13660,1187.2515994291);
#2552=CIRCLE('',#13661,1187.25159943443);
#2553=CIRCLE('',#13662,1187.25159944835);
#2554=CIRCLE('',#13663,1187.25159943896);
#2555=CIRCLE('',#13664,1187.25159941435);
#2556=CIRCLE('',#13665,1187.25159942352);
#2557=CIRCLE('',#13666,1187.25365510695);
#2558=CIRCLE('',#13667,1187.25431298853);
#2559=CIRCLE('',#13668,1187.25159940573);
#2560=CIRCLE('',#13669,1187.25159941578);
#2561=CIRCLE('',#13670,1187.25365512172);
#2562=CIRCLE('',#13671,1187.25431296975);
#2563=CIRCLE('',#13672,1187.25159941323);
#2564=CIRCLE('',#13673,1187.25159939663);
#2565=CIRCLE('',#13674,1187.25159940667);
#2566=CIRCLE('',#13675,1187.25159943706);
#2567=CIRCLE('',#13677,15.5);
#2568=CIRCLE('',#13679,15.5);
#2569=CIRCLE('',#13681,15.5);
#2570=CIRCLE('',#13682,15.5);
#2571=CIRCLE('',#13683,15.5);
#2572=CIRCLE('',#13684,15.5);
#2573=CIRCLE('',#13685,15.5);
#2574=CIRCLE('',#13686,15.5);
#2575=CIRCLE('',#13687,15.5);
#2576=CIRCLE('',#13688,15.5);
#2577=CIRCLE('',#13689,15.5);
#2578=CIRCLE('',#13690,15.5);
#2579=CIRCLE('',#13691,15.5);
#2580=CIRCLE('',#13692,15.5);
#2581=CIRCLE('',#13693,15.5);
#2582=CIRCLE('',#13694,15.5);
#2583=CIRCLE('',#13695,15.5);
#2584=CIRCLE('',#13696,15.5);
#2872=B_SPLINE_CURVE_WITH_KNOTS('',3,(#17360,#17361,#17362,#17363,#17364,
#17365,#17366,#17367),.UNSPECIFIED.,.F.,.F.,(4,1,1,1,1,4),(87.0483584551456,
87.288606653755,87.7848809882288,88.2811553227026,88.7774296571764,89.2737039916502),
 .UNSPECIFIED.);
#2873=B_SPLINE_CURVE_WITH_KNOTS('',3,(#17370,#17371,#17372,#17373,#17374,
#17375,#17376,#17377,#17378),.UNSPECIFIED.,.F.,.F.,(4,1,1,1,1,1,4),(87.0483757384693,
87.3511807444607,87.8474550789345,88.3437294134083,88.8400037478821,89.3362780823559,
89.7970772629679),.UNSPECIFIED.);
#2874=B_SPLINE_CURVE_WITH_KNOTS('',3,(#17384,#17385,#17386,#17387,#17388,
#17389,#17390,#17391,#17392,#17393,#17394,#17395,#17396,#17397,#17398,#17399,
#17400,#17401,#17402,#17403,#17404,#17405,#17406,#17407,#17408,#17409,#17410,
#17411,#17412,#17413,#17414,#17415,#17416,#17417,#17418,#17419,#17420,#17421,
#17422,#17423,#17424,#17425,#17426,#17427,#17428,#17429,#17430,#17431,#17432,
#17433,#17434,#17435,#17436,#17437,#17438,#17439,#17440,#17441,#17442,#17443,
#17444,#17445,#17446,#17447,#17448,#17449,#17450,#17451,#17452,#17453,#17454,
#17455,#17456,#17457,#17458,#17459,#17460,#17461,#17462,#17463,#17464,#17465,
#17466,#17467,#17468,#17469,#17470,#17471,#17472,#17473,#17474,#17475,#17476,
#17477,#17478,#17479,#17480,#17481,#17482,#17483,#17484,#17485,#17486,#17487,
#17488,#17489,#17490,#17491,#17492,#17493,#17494,#17495,#17496,#17497,#17498,
#17499,#17500,#17501,#17502,#17503,#17504,#17505,#17506,#17507,#17508,#17509,
#17510,#17511,#17512,#17513,#17514,#17515,#17516,#17517,#17518,#17519,#17520,
#17521,#17522,#17523,#17524,#17525,#17526,#17527,#17528,#17529,#17530,#17531,
#17532,#17533,#17534,#17535,#17536,#17537,#17538,#17539,#17540,#17541,#17542,
#17543,#17544,#17545,#17546,#17547,#17548,#17549,#17550,#17551,#17552,#17553,
#17554,#17555,#17556,#17557,#17558),.UNSPECIFIED.,.F.,.F.,(4,3,3,3,3,3,
3,3,3,3,3,3,3,3,3,3,3,3,3,3,3,3,3,3,3,3,3,3,3,3,3,3,3,3,3,3,3,3,3,3,3,3,
3,3,3,3,3,3,3,3,3,3,3,3,3,3,3,3,4),(80.7651597880717,80.8370403055957,80.914545344832,
80.9920362923502,81.0695186842698,81.1470072216587,81.2244955439902,81.3020000212182,
81.3333146400695,81.4108196470028,81.4883105620921,81.5657929215612,81.6432814267086,
81.7207697169786,81.7982741626174,81.8295889745433,81.9070940470507,81.9845850279213,
82.0620674531671,82.1395560235961,82.2170443787414,82.2945488882385,82.3258633090171,
82.4033682793892,82.4808591578936,82.5583414808702,82.6358299499321,82.7133182044183,
82.790822614948,82.8221376434909,82.8996427153748,82.9771336953985,83.0546161195796,
83.1321046886325,83.2095930422246,83.2870975499181,83.3184119779647,83.3959170883937,
83.4734081078065,83.5508905720845,83.6283791819793,83.7058675767654,83.7833721259062,
83.8146863124385,83.8921909082518,83.9696814101362,84.0471633556579,84.1246514488292,
84.2021393290257,84.2796433700398,84.3109606469122,84.3884668552791,84.4659589764845,
84.5434425428528,84.6209322471122,84.6984217297766,84.7759273502229,84.807234981386,
84.8230016469244),.UNSPECIFIED.);
#2875=B_SPLINE_CURVE_WITH_KNOTS('',3,(#17559,#17560,#17561,#17562,#17563,
#17564,#17565,#17566),.UNSPECIFIED.,.F.,.F.,(4,1,1,1,1,4),(84.8230016659403,
85.3035093158598,85.7997836503336,86.2960579848074,86.7923323192812,87.0483584551456),
 .UNSPECIFIED.);
#2876=B_SPLINE_CURVE_WITH_KNOTS('',3,(#17568,#17569,#17570,#17571,#17572,
#17573,#17574,#17575,#17576),.UNSPECIFIED.,.F.,.F.,(4,1,1,1,1,1,4),(84.8230016469244,
84.8698090720917,85.3660834065655,85.8623577410393,86.3586320755131,86.8549064099869,
87.0483757384693),.UNSPECIFIED.);
#2877=B_SPLINE_CURVE_WITH_KNOTS('',3,(#17577,#17578,#17579,#17580,#17581,
#17582,#17583,#17584,#17585,#17586,#17587,#17588,#17589,#17590,#17591,#17592,
#17593,#17594,#17595,#17596,#17597,#17598,#17599,#17600,#17601,#17602,#17603,
#17604,#17605,#17606,#17607,#17608,#17609,#17610,#17611,#17612,#17613,#17614,
#17615,#17616,#17617,#17618,#17619,#17620,#17621,#17622,#17623,#17624,#17625,
#17626,#17627,#17628,#17629,#17630,#17631,#17632,#17633,#17634,#17635,#17636,
#17637,#17638,#17639,#17640,#17641,#17642,#17643,#17644,#17645,#17646,#17647,
#17648,#17649,#17650,#17651,#17652,#17653,#17654,#17655,#17656,#17657,#17658,
#17659,#17660,#17661,#17662,#17663,#17664,#17665,#17666,#17667,#17668,#17669,
#17670,#17671,#17672,#17673,#17674,#17675,#17676,#17677,#17678,#17679,#17680,
#17681,#17682,#17683,#17684,#17685,#17686,#17687,#17688,#17689,#17690,#17691,
#17692,#17693,#17694,#17695,#17696,#17697,#17698,#17699,#17700,#17701,#17702,
#17703,#17704,#17705,#17706,#17707,#17708,#17709,#17710,#17711,#17712,#17713,
#17714,#17715,#17716,#17717,#17718,#17719,#17720,#17721,#17722,#17723,#17724,
#17725,#17726,#17727,#17728,#17729,#17730,#17731,#17732,#17733,#17734,#17735,
#17736,#17737,#17738,#17739,#17740,#17741,#17742,#17743,#17744,#17745,#17746,
#17747,#17748),.UNSPECIFIED.,.F.,.F.,(4,3,3,3,3,3,3,3,3,3,3,3,3,3,3,3,3,
3,3,3,3,3,3,3,3,3,3,3,3,3,3,3,3,3,3,3,3,3,3,3,3,3,3,3,3,3,3,3,3,3,3,3,3,
3,3,3,3,4),(80.7651593553048,80.8426649664577,80.8996143963013,80.9771194265575,
81.0546103650544,81.1320927479402,81.2095812763449,81.2870695897373,81.3645740581496,
81.3958887307751,81.4733937598586,81.5508846971797,81.6283670788907,81.7058556061292,
81.7833439183629,81.860848385635,81.8921630652489,81.9696680959697,82.0471590349305,
82.1246414182788,82.2021299471396,82.2796182609839,82.3571227298382,82.3884373997227,
82.4659424292746,82.5434333670696,82.6209157492587,82.6984042769776,82.7758925896912,
82.8533970574419,82.8847117341965,82.962216761565,83.0397076971565,83.1171900771288,
83.1946786026281,83.2721669131255,83.3496713786775,83.3809860686703,83.4584911079066,
83.5359820554258,83.6134644473447,83.6909529847341,83.7684413070656,83.8459457842936,
83.8772604031441,83.9547654100771,84.0322563251666,84.1097386846358,84.1872271897834,
84.2647154800541,84.3422199256925,84.3735347376179,84.4507891948756,84.5280287669538,
84.6052689644067,84.6825047195202,84.7597573289946,84.8230016469244),
 .UNSPECIFIED.);
#2878=B_SPLINE_CURVE_WITH_KNOTS('',3,(#17754,#17755,#17756,#17757,#17758,
#17759,#17760,#17761,#17762,#17763,#17764,#17765),.UNSPECIFIED.,.F.,.F.,
(4,1,1,1,1,1,1,1,1,4),(74.4820139112556,74.8817482919101,75.3780226263839,
75.8742969608577,76.3705712953315,76.8668456298053,77.3631199642791,77.8593942987529,
78.3556686332267,78.5398163045171),.UNSPECIFIED.);
#2879=B_SPLINE_CURVE_WITH_KNOTS('',3,(#17766,#17767,#17768,#17769,#17770,
#17771,#17772,#17773,#17774,#17775,#17776,#17777,#17778,#17779,#17780,#17781,
#17782,#17783,#17784,#17785,#17786,#17787,#17788,#17789,#17790,#17791,#17792,
#17793,#17794,#17795,#17796,#17797,#17798,#17799,#17800,#17801,#17802,#17803,
#17804,#17805,#17806,#17807,#17808,#17809,#17810,#17811,#17812,#17813,#17814,
#17815,#17816,#17817,#17818,#17819,#17820,#17821,#17822,#17823,#17824,#17825,
#17826,#17827,#17828,#17829,#17830,#17831,#17832,#17833,#17834,#17835,#17836,
#17837,#17838,#17839,#17840,#17841,#17842,#17843,#17844,#17845,#17846,#17847,
#17848,#17849,#17850,#17851,#17852,#17853,#17854,#17855,#17856,#17857,#17858,
#17859),.UNSPECIFIED.,.F.,.F.,(4,3,3,3,3,3,3,3,3,3,3,3,3,3,3,3,3,3,3,3,
3,3,3,3,3,3,3,3,3,3,3,4),(78.5398163397448,78.6178479967337,78.6954897638523,
78.7737163657764,78.8519429677005,78.9294479967842,79.0069389341053,79.084421315816,
79.1619098430544,79.2393981552877,79.3169026225599,79.3482173021743,79.4257223328949,
79.5032132718561,79.5806956552048,79.6581841840654,79.735672497909,79.8131769667635,
79.8444916366481,79.9219966662,79.9994876039955,80.0769699861842,80.1544585139031,
80.2319468266171,80.3094512943681,80.3407659711219,80.4182703729319,80.495760433696,
80.5732483850591,80.6507311082695,80.7282234409962,80.7651597880717),
 .UNSPECIFIED.);
#2880=B_SPLINE_CURVE_WITH_KNOTS('',3,(#17861,#17862,#17863,#17864,#17865,
#17866,#17867,#17868,#17869,#17870,#17871,#17872,#17873,#17874,#17875,#17876,
#17877,#17878,#17879,#17880,#17881,#17882,#17883,#17884,#17885,#17886,#17887,
#17888,#17889,#17890,#17891,#17892,#17893,#17894,#17895,#17896,#17897,#17898,
#17899,#17900,#17901,#17902,#17903,#17904,#17905,#17906,#17907,#17908,#17909,
#17910,#17911,#17912,#17913,#17914,#17915,#17916,#17917,#17918,#17919,#17920,
#17921,#17922,#17923,#17924,#17925,#17926,#17927,#17928,#17929,#17930,#17931,
#17932,#17933,#17934,#17935,#17936,#17937,#17938,#17939,#17940,#17941,#17942,
#17943,#17944,#17945,#17946,#17947,#17948,#17949,#17950,#17951,#17952,#17953,
#17954),.UNSPECIFIED.,.F.,.F.,(4,3,3,3,3,3,3,3,3,3,3,3,3,3,3,3,3,3,3,3,
3,3,3,3,3,3,3,3,3,3,3,4),(78.5398163397448,78.6170621768428,78.6943109079355,
78.7715563124194,78.8488208011277,78.9145170584062,78.9920220882176,79.0695130262683,
79.1469954087081,79.2244839366697,79.3019722496216,79.3794767176006,79.41079139288,
79.4882964226991,79.5657873607574,79.6432697432046,79.7207582711736,79.7982465841325,
79.8757510521183,79.9070657273538,79.9845707572399,80.0620616953655,80.139544077881,
80.2170326059175,80.2945209189436,80.3720253869959,80.4033400618275,80.4808443139909,
80.5583386268419,80.6358226274582,80.713310678145,80.7651593553048),
 .UNSPECIFIED.);
#2881=B_SPLINE_CURVE_WITH_KNOTS('',3,(#17955,#17956,#17957,#17958,#17959,
#17960,#17961,#17962,#17963,#17964,#17965,#17966,#17967,#17968,#17969,#17970,
#17971,#17972,#17973,#17974,#17975,#17976,#17977,#17978,#17979,#17980,#17981,
#17982,#17983,#17984,#17985,#17986,#17987,#17988,#17989,#17990,#17991,#17992,
#17993,#17994,#17995,#17996,#17997,#17998,#17999,#18000,#18001,#18002,#18003,
#18004,#18005,#18006,#18007,#18008,#18009,#18010,#18011,#18012,#18013,#18014,
#18015,#18016,#18017,#18018,#18019,#18020,#18021,#18022,#18023,#18024,#18025,
#18026,#18027,#18028,#18029,#18030,#18031,#18032,#18033,#18034,#18035,#18036,
#18037,#18038,#18039,#18040,#18041,#18042,#18043,#18044,#18045,#18046,#18047,
#18048,#18049,#18050,#18051,#18052,#18053,#18054,#18055,#18056,#18057,#18058,
#18059,#18060,#18061,#18062,#18063,#18064,#18065,#18066,#18067,#18068,#18069,
#18070,#18071,#18072,#18073,#18074,#18075,#18076,#18077,#18078,#18079,#18080,
#18081,#18082,#18083,#18084,#18085,#18086,#18087,#18088,#18089,#18090,#18091,
#18092,#18093,#18094,#18095,#18096,#18097,#18098,#18099,#18100,#18101,#18102,
#18103,#18104,#18105,#18106,#18107,#18108,#18109,#18110,#18111,#18112,#18113,
#18114,#18115,#18116,#18117,#18118,#18119,#18120,#18121,#18122,#18123,#18124,
#18125,#18126),.UNSPECIFIED.,.F.,.F.,(4,3,3,3,3,3,3,3,3,3,3,3,3,3,3,3,3,
3,3,3,3,3,3,3,3,3,3,3,3,3,3,3,3,3,3,3,3,3,3,3,3,3,3,3,3,3,3,3,3,3,3,3,3,
3,3,3,3,4),(74.4819991062224,74.5594972817628,74.6369837912023,74.7144748782765,
74.7919626281567,74.8694696203011,74.9443223826158,75.0218274124397,75.0993183505029,
75.1768007329554,75.2542892609294,75.3317775738933,75.4092820418842,75.4405967170896,
75.5181017469132,75.5955926849761,75.6730750674282,75.7505635954018,75.8280519083655,
75.9055563763561,75.9368710515634,76.0143760813873,76.0918670194505,76.1693494019029,
76.2468379298769,76.3243262428409,76.4018307108318,76.4331453860372,76.5106504158612,
76.5881413539246,76.6656237363772,76.7431122643514,76.8206005773155,76.8981050453065,
76.929419720511,77.0069247503333,77.0844156883949,77.1618980708456,77.239386598818,
77.3168749117803,77.3943793797696,77.4256940549848,77.5031990848125,77.5806900228796,
77.658172405336,77.7356609333137,77.8131492462817,77.8906537142763,77.9219683894586,
77.9994734192743,78.0769643573295,78.1544467397738,78.2319352677398,78.3094235806959,
78.3869280486788,78.4182427239324,78.4997461276738,78.5398163396564),
 .UNSPECIFIED.);
#2882=B_SPLINE_CURVE_WITH_KNOTS('',3,(#18132,#18133,#18134,#18135,#18136,
#18137,#18138,#18139,#18140,#18141,#18142,#18143,#18144,#18145,#18146,#18147,
#18148,#18149,#18150,#18151,#18152,#18153,#18154,#18155,#18156,#18157,#18158,
#18159,#18160,#18161,#18162,#18163,#18164,#18165,#18166,#18167,#18168,#18169,
#18170,#18171,#18172,#18173,#18174,#18175,#18176,#18177,#18178,#18179,#18180,
#18181,#18182,#18183,#18184,#18185,#18186,#18187,#18188,#18189,#18190,#18191,
#18192,#18193,#18194,#18195,#18196,#18197,#18198,#18199,#18200,#18201,#18202,
#18203,#18204,#18205,#18206,#18207,#18208,#18209,#18210,#18211,#18212,#18213,
#18214,#18215,#18216,#18217,#18218,#18219,#18220,#18221,#18222,#18223,#18224,
#18225,#18226,#18227,#18228,#18229,#18230,#18231,#18232,#18233,#18234,#18235,
#18236,#18237,#18238,#18239,#18240,#18241,#18242,#18243,#18244,#18245,#18246,
#18247,#18248,#18249,#18250,#18251,#18252,#18253,#18254,#18255,#18256,#18257,
#18258,#18259,#18260,#18261,#18262,#18263,#18264,#18265,#18266,#18267,#18268,
#18269,#18270,#18271,#18272,#18273,#18274,#18275,#18276,#18277,#18278,#18279,
#18280,#18281,#18282,#18283,#18284,#18285,#18286,#18287,#18288,#18289,#18290,
#18291,#18292,#18293,#18294,#18295,#18296,#18297,#18298,#18299,#18300,#18301,
#18302,#18303),.UNSPECIFIED.,.F.,.F.,(4,3,3,3,3,3,3,3,3,3,3,3,3,3,3,3,3,
3,3,3,3,3,3,3,3,3,3,3,3,3,3,3,3,3,3,3,3,3,3,3,3,3,3,3,3,3,3,3,3,3,3,3,3,
3,3,3,3,4),(68.198801431243,68.2762891932681,68.3537963258945,68.4301819437508,
68.5076869735746,68.5851779116379,68.6626602940891,68.740148822063,68.8176371350266,
68.8951416030175,68.9264562782246,69.0039613080483,69.0814522461114,69.1589346285636,
69.2364231565373,69.3139114695007,69.3914159374917,69.4227306126984,69.500235642522,
69.5777265805855,69.6552089630386,69.7326974910125,69.8101858039759,69.8876902719668,
69.9190049471722,69.9965099769959,70.0740009150587,70.1514832975117,70.2289718254855,
70.306460138449,70.38396460644,70.415279281646,70.4927843114698,70.5702752495332,
70.6477576319852,70.7252461599591,70.8027344729236,70.8802389409149,70.9115536161198,
70.9890586459435,71.0665495840061,71.1440319664588,71.2215204944324,71.2990088073963,
71.3765132753868,71.4078279505936,71.4853329804172,71.5628239184807,71.6403063009341,
71.7177948289081,71.7952831418719,71.872787609863,71.9041022850674,71.9814641664295,
72.0588148259056,72.1361550941926,72.213498904701,72.2566310325652),
 .UNSPECIFIED.);
#2883=B_SPLINE_CURVE_WITH_KNOTS('',3,(#18304,#18305,#18306,#18307,#18308,
#18309,#18310,#18311,#18312),.UNSPECIFIED.,.F.,.F.,(4,1,1,1,1,1,4),(72.2566310562343,
72.4003766195412,72.896650954015,73.3929252884888,73.8891996229626,74.3854739574363,
74.4820139112556),.UNSPECIFIED.);
#2884=B_SPLINE_CURVE_WITH_KNOTS('',3,(#18314,#18315,#18316,#18317,#18318,
#18319,#18320,#18321,#18322,#18323,#18324,#18325,#18326,#18327,#18328,#18329,
#18330,#18331,#18332,#18333,#18334,#18335,#18336,#18337,#18338,#18339,#18340,
#18341,#18342,#18343,#18344,#18345,#18346,#18347,#18348,#18349,#18350,#18351,
#18352,#18353,#18354,#18355,#18356,#18357,#18358,#18359,#18360,#18361,#18362,
#18363,#18364,#18365,#18366,#18367,#18368,#18369,#18370,#18371,#18372,#18373,
#18374,#18375,#18376,#18377,#18378,#18379,#18380,#18381,#18382,#18383,#18384,
#18385,#18386,#18387,#18388,#18389,#18390,#18391,#18392,#18393,#18394,#18395,
#18396,#18397,#18398,#18399,#18400,#18401,#18402,#18403,#18404,#18405,#18406,
#18407,#18408,#18409,#18410),.UNSPECIFIED.,.F.,.F.,(4,3,3,3,3,3,3,3,3,3,
3,3,3,3,3,3,3,3,3,3,3,3,3,3,3,3,3,3,3,3,3,3,4),(72.2566310326268,72.3358367452908,
72.4150680313353,72.4629507102468,72.5404557400706,72.6179466781338,72.695429060586,
72.7729175885598,72.8504059015235,72.927910369514,72.9592250447206,73.0367300745445,
73.1142210126076,73.1917033950602,73.269191923034,73.3466802359978,73.4241847039887,
73.4554993791944,73.5330044090182,73.6104953470813,73.6879777295337,73.7654662575075,
73.8429545704714,73.9204590384622,73.9517737136682,74.029278743492,74.1067696815552,
74.1842520640075,74.2617405919814,74.3392289049453,74.4167333729361,74.448048048142,
74.4819991062224),.UNSPECIFIED.);
#2885=B_SPLINE_CURVE_WITH_KNOTS('',3,(#18411,#18412,#18413,#18414,#18415,
#18416,#18417,#18418,#18419,#18420,#18421,#18422,#18423,#18424,#18425,#18426,
#18427,#18428,#18429,#18430,#18431,#18432,#18433,#18434,#18435,#18436,#18437,
#18438,#18439,#18440,#18441,#18442,#18443,#18444,#18445,#18446,#18447,#18448,
#18449,#18450,#18451,#18452,#18453,#18454,#18455,#18456,#18457,#18458,#18459,
#18460,#18461,#18462,#18463,#18464,#18465,#18466,#18467,#18468,#18469,#18470,
#18471,#18472,#18473,#18474,#18475,#18476,#18477,#18478,#18479,#18480,#18481,
#18482,#18483,#18484,#18485,#18486,#18487,#18488,#18489,#18490,#18491,#18492,
#18493,#18494,#18495,#18496,#18497,#18498,#18499,#18500,#18501,#18502,#18503,
#18504,#18505,#18506,#18507,#18508,#18509,#18510,#18511,#18512,#18513,#18514,
#18515,#18516,#18517,#18518,#18519,#18520,#18521,#18522,#18523,#18524,#18525,
#18526,#18527,#18528,#18529,#18530,#18531,#18532,#18533,#18534,#18535,#18536,
#18537,#18538,#18539,#18540,#18541,#18542,#18543,#18544,#18545,#18546,#18547,
#18548,#18549,#18550,#18551,#18552,#18553,#18554,#18555,#18556,#18557,#18558,
#18559,#18560,#18561,#18562,#18563,#18564,#18565,#18566,#18567,#18568,#18569,
#18570,#18571,#18572,#18573,#18574,#18575,#18576,#18577,#18578,#18579,#18580,
#18581,#18582),.UNSPECIFIED.,.F.,.F.,(4,3,3,3,3,3,3,3,3,3,3,3,3,3,3,3,3,
3,3,3,3,3,3,3,3,3,3,3,3,3,3,3,3,3,3,3,3,3,3,3,3,3,3,3,3,3,3,3,3,3,3,3,3,
3,3,3,3,4),(68.198812002236,68.2763021152483,68.3537898515224,68.4312957656329,
68.4927560344565,68.5702610642803,68.6477520023434,68.7252343847957,68.8027229127696,
68.8802112257334,68.9577156937242,68.9890303689303,69.0665353987541,69.1440263368171,
69.2215087192695,69.2989972472433,69.3764855602071,69.4539900281979,69.4853047034041,
69.5628097332279,69.640300671291,69.7177830537434,69.7952715817172,69.8727598946811,
69.9502643626719,69.9815790378779,70.0590840677017,70.1365750057647,70.214057388217,
70.2915459161909,70.3690342291547,70.4465386971454,70.4778533723517,70.5553584021755,
70.6328493402385,70.7103317226907,70.7878202506645,70.8653085636282,70.942813031619,
70.9741277068254,71.0516327366491,71.1291236747122,71.2066060571644,71.2840945851382,
71.361582898102,71.4390873660927,71.4704020412992,71.547907071123,71.6253980091863,
71.7028803916382,71.780368919612,71.8578572325758,71.9353617005666,71.966676375773,
72.0445687492081,72.122444909863,72.2003138435325,72.2566310325652),
 .UNSPECIFIED.);
#2886=B_SPLINE_CURVE_WITH_KNOTS('',3,(#18588,#18589,#18590,#18591,#18592,
#18593,#18594,#18595,#18596,#18597,#18598,#18599,#18600,#18601,#18602,#18603,
#18604,#18605,#18606,#18607,#18608,#18609,#18610,#18611,#18612,#18613,#18614,
#18615,#18616,#18617,#18618,#18619,#18620,#18621,#18622,#18623,#18624,#18625,
#18626,#18627,#18628,#18629,#18630,#18631,#18632,#18633,#18634,#18635,#18636,
#18637,#18638,#18639,#18640,#18641,#18642,#18643,#18644,#18645,#18646,#18647,
#18648,#18649,#18650,#18651,#18652,#18653,#18654,#18655,#18656,#18657,#18658,
#18659,#18660,#18661,#18662,#18663,#18664,#18665,#18666,#18667,#18668,#18669,
#18670,#18671,#18672,#18673,#18674,#18675,#18676,#18677,#18678,#18679,#18680,
#18681,#18682,#18683,#18684,#18685,#18686,#18687,#18688,#18689,#18690,#18691,
#18692,#18693,#18694,#18695,#18696,#18697,#18698,#18699,#18700,#18701,#18702,
#18703,#18704,#18705,#18706,#18707,#18708,#18709,#18710,#18711,#18712,#18713,
#18714,#18715,#18716,#18717,#18718,#18719,#18720,#18721,#18722,#18723,#18724,
#18725,#18726,#18727,#18728,#18729,#18730,#18731,#18732,#18733,#18734,#18735,
#18736,#18737,#18738,#18739,#18740,#18741,#18742,#18743,#18744,#18745,#18746,
#18747,#18748,#18749,#18750,#18751,#18752,#18753,#18754,#18755,#18756,#18757,
#18758,#18759,#18760,#18761,#18762),.UNSPECIFIED.,.F.,.F.,(4,3,3,3,3,3,
3,3,3,3,3,3,3,3,3,3,3,3,3,3,3,3,3,3,3,3,3,3,3,3,3,3,3,3,3,3,3,3,3,3,3,3,
3,3,3,3,3,3,3,3,3,3,3,3,3,3,3,3,4),(61.9156047763896,61.9786155955915,62.0561206254154,
62.1336115634786,62.2110939459307,62.2885824739047,62.3660707868687,62.4435752548594,
62.4748899300653,62.552394959889,62.6298858979524,62.7073682804045,62.7848568083784,
62.862345121342,62.9398495893327,62.9711642645391,63.0486692943629,63.126160232426,
63.2036426148776,63.2811311428513,63.3586194558156,63.4361239238064,63.4674385990129,
63.5449436288367,63.6224345668995,63.6999169493516,63.7774054773254,63.8548937902894,
63.9323982582801,63.9637129334867,64.0412179633103,64.1187089013731,64.1961912838254,
64.2736798117994,64.3511681247633,64.4286725927539,64.4599872679605,64.5374922977843,
64.614983235847,64.6924656183003,64.7699541462741,64.8474424592383,64.924946927229,
64.9562616024343,65.0337666322583,65.1112575703216,65.188739952774,65.266228480748,
65.3437167937126,65.4212212617037,65.452535936908,65.5300409667316,65.6075319047948,
65.6850142872465,65.7625028152201,65.8399911281846,65.9174955961746,65.9488102713818,
65.9734457253856),.UNSPECIFIED.);
#2887=B_SPLINE_CURVE_WITH_KNOTS('',3,(#18763,#18764,#18765,#18766,#18767,
#18768,#18769,#18770,#18771,#18772,#18773,#18774,#18775,#18776,#18777,#18778,
#18779,#18780,#18781,#18782,#18783,#18784,#18785,#18786,#18787,#18788,#18789,
#18790,#18791,#18792,#18793,#18794,#18795,#18796,#18797,#18798,#18799,#18800,
#18801,#18802,#18803,#18804,#18805,#18806,#18807,#18808,#18809,#18810,#18811,
#18812,#18813,#18814,#18815,#18816,#18817,#18818,#18819,#18820,#18821,#18822,
#18823,#18824,#18825,#18826,#18827,#18828,#18829,#18830,#18831,#18832,#18833,
#18834,#18835,#18836,#18837,#18838,#18839,#18840,#18841,#18842,#18843,#18844,
#18845,#18846,#18847,#18848,#18849,#18850,#18851,#18852,#18853,#18854,#18855,
#18856),.UNSPECIFIED.,.F.,.F.,(4,3,3,3,3,3,3,3,3,3,3,3,3,3,3,3,3,3,3,3,
3,3,3,3,3,3,3,3,3,3,3,4),(65.9734457254986,66.0507928770444,66.1281258638911,
66.2073655493822,66.2846965630064,66.364890584431,66.4450846058556,66.5225896356792,
66.6000805737422,66.6775629561948,66.7550514841686,66.8325397971324,66.910044265123,
66.9413589403294,67.0188639701531,67.0963549082163,67.173837290669,67.2513258186429,
67.3288141316065,67.4063185995973,67.4376332748032,67.5151383046269,67.5926292426899,
67.6701116251421,67.7476001531158,67.8250884660794,67.9025929340702,67.933907609277,
68.0114130956238,68.0889034409014,68.1663881412969,68.198801431243),
 .UNSPECIFIED.);
#2888=B_SPLINE_CURVE_WITH_KNOTS('',3,(#18858,#18859,#18860,#18861,#18862,
#18863,#18864,#18865,#18866,#18867,#18868,#18869,#18870,#18871,#18872,#18873,
#18874,#18875,#18876,#18877,#18878,#18879,#18880,#18881,#18882,#18883,#18884,
#18885,#18886,#18887,#18888,#18889,#18890,#18891,#18892,#18893,#18894,#18895,
#18896,#18897,#18898,#18899,#18900,#18901,#18902,#18903,#18904,#18905,#18906,
#18907,#18908,#18909,#18910,#18911,#18912,#18913,#18914,#18915,#18916,#18917,
#18918,#18919,#18920,#18921,#18922,#18923,#18924,#18925,#18926,#18927,#18928,
#18929,#18930,#18931,#18932,#18933,#18934,#18935,#18936,#18937,#18938,#18939,
#18940,#18941,#18942,#18943,#18944,#18945,#18946,#18947,#18948,#18949,#18950,
#18951,#18952,#18953,#18954),.UNSPECIFIED.,.F.,.F.,(4,3,3,3,3,3,3,3,3,3,
3,3,3,3,3,3,3,3,3,3,3,3,3,3,3,3,3,3,3,3,3,3,4),(65.9734457253856,66.0113843620875,
66.0888893919113,66.1663803299744,66.2438627124269,66.3213512404007,66.3988395533646,
66.4763440213554,66.5076586965613,66.5851637263852,66.6626546644483,66.7401370469007,
66.8176255748745,66.8951138878385,66.9726183558293,67.0039330310351,67.0814380608589,
67.1589289989221,67.2364113813744,67.3138999093482,67.3913882223121,67.4688926903028,
67.5002073655089,67.5777123953327,67.6552033333958,67.7326857158482,67.810174243822,
67.8876625567858,67.9651670247766,67.9964816999827,68.0739860168883,68.1514785081145,
68.198812002236),.UNSPECIFIED.);
#2889=B_SPLINE_CURVE_WITH_KNOTS('',3,(#18955,#18956,#18957,#18958,#18959,
#18960,#18961,#18962,#18963,#18964,#18965,#18966),.UNSPECIFIED.,.F.,.F.,
(4,1,1,1,1,1,1,1,1,4),(61.915593798429,62.0411896862971,62.5374640207709,
63.0337383552447,63.5300126897185,64.0262870241923,64.5225613586661,65.0188356931399,
65.5151100276137,65.973445690953),.UNSPECIFIED.);
#2890=B_SPLINE_CURVE_WITH_KNOTS('',3,(#18972,#18973,#18974,#18975,#18976,
#18977,#18978,#18979,#18980,#18981,#18982,#18983,#18984,#18985,#18986,#18987,
#18988,#18989,#18990,#18991,#18992,#18993,#18994,#18995,#18996,#18997,#18998,
#18999,#19000,#19001,#19002,#19003,#19004,#19005,#19006,#19007,#19008,#19009,
#19010,#19011,#19012,#19013,#19014,#19015,#19016,#19017,#19018,#19019,#19020,
#19021,#19022,#19023,#19024,#19025,#19026,#19027,#19028,#19029,#19030,#19031,
#19032,#19033,#19034,#19035,#19036,#19037,#19038,#19039,#19040,#19041,#19042,
#19043,#19044,#19045,#19046,#19047,#19048,#19049,#19050,#19051,#19052,#19053,
#19054,#19055,#19056,#19057,#19058,#19059,#19060,#19061,#19062,#19063,#19064,
#19065,#19066,#19067,#19068,#19069,#19070,#19071,#19072,#19073,#19074,#19075,
#19076,#19077,#19078,#19079,#19080,#19081,#19082,#19083,#19084,#19085,#19086,
#19087,#19088,#19089,#19090,#19091,#19092,#19093,#19094,#19095,#19096,#19097,
#19098,#19099,#19100,#19101,#19102,#19103,#19104,#19105,#19106,#19107,#19108,
#19109,#19110,#19111,#19112,#19113,#19114,#19115,#19116,#19117,#19118,#19119,
#19120,#19121,#19122,#19123,#19124,#19125,#19126,#19127,#19128,#19129,#19130,
#19131,#19132,#19133,#19134,#19135,#19136,#19137,#19138,#19139,#19140,#19141,
#19142,#19143),.UNSPECIFIED.,.F.,.F.,(4,3,3,3,3,3,3,3,3,3,3,3,3,3,3,3,3,
3,3,3,3,3,3,3,3,3,3,3,3,3,3,3,3,3,3,3,3,3,3,3,3,3,3,3,3,3,3,3,3,3,3,3,3,
3,3,3,3,4),(55.6324502817996,55.7099375026088,55.7882840224331,55.8657718222351,
55.9445477020706,56.023323581906,56.1008286117298,56.1783195497928,56.2558019322451,
56.3332904602189,56.4107787731827,56.4882832411734,56.5195979163798,56.5971029462036,
56.6745938842667,56.752076266719,56.8295647946928,56.9070531076567,56.9845575756474,
57.0158722508535,57.0933772806773,57.1708682187403,57.2483506011926,57.3258391291664,
57.4033274421302,57.4808319101209,57.5121465853273,57.5896516151511,57.6671425532142,
57.7446249356666,57.8221134636404,57.8996017766043,57.9771062445951,58.0084209198011,
58.0859259496249,58.1634168876881,58.2408992701405,58.3183877981143,58.3958761110781,
58.4733805790688,58.5046952542749,58.5822002840987,58.6596912221618,58.7371736046139,
58.8146621325877,58.8921504455517,58.9696549135425,59.0009695887487,59.0784746185724,
59.1559655566355,59.2334479390883,59.3109364670621,59.3884247800259,59.4659292480167,
59.4972439232225,59.5767649286567,59.6562642201875,59.6902604181339),
 .UNSPECIFIED.);
#2891=B_SPLINE_CURVE_WITH_KNOTS('',3,(#19144,#19145,#19146,#19147,#19148,
#19149,#19150,#19151,#19152,#19153,#19154,#19155,#19156,#19157,#19158,#19159,
#19160,#19161,#19162,#19163,#19164,#19165,#19166,#19167,#19168,#19169,#19170,
#19171,#19172,#19173,#19174,#19175,#19176,#19177,#19178,#19179,#19180,#19181,
#19182,#19183,#19184,#19185,#19186,#19187,#19188,#19189,#19190,#19191,#19192,
#19193,#19194,#19195,#19196,#19197,#19198,#19199,#19200,#19201,#19202,#19203,
#19204,#19205,#19206,#19207,#19208,#19209,#19210,#19211,#19212,#19213,#19214,
#19215,#19216,#19217,#19218,#19219,#19220,#19221,#19222,#19223,#19224,#19225,
#19226,#19227,#19228,#19229,#19230,#19231,#19232,#19233,#19234,#19235,#19236,
#19237),.UNSPECIFIED.,.F.,.F.,(4,3,3,3,3,3,3,3,3,3,3,3,3,3,3,3,3,3,3,3,
3,3,3,3,3,3,3,3,3,3,3,4),(59.690260418206,59.7679892440258,59.8457171883824,
59.9234656380215,59.9935182576963,60.0710232875201,60.1485142255832,60.2259966080357,
60.3034851360095,60.3809734489736,60.4584779169643,60.4897925921701,60.5672976219939,
60.6447885600572,60.7222709425095,60.7997594704833,60.8772477834472,60.954752251438,
60.9860669266439,61.0635719564677,61.1410628945307,61.2185452769831,61.296033804957,
61.3735221179207,61.4510265859116,61.4823412611177,61.5598457164873,61.6373358615963,
61.714824493991,61.7923078312911,61.8698020429645,61.9156047763896),
 .UNSPECIFIED.);
#2892=B_SPLINE_CURVE_WITH_KNOTS('',3,(#19239,#19240,#19241,#19242,#19243,
#19244,#19245,#19246),.UNSPECIFIED.,.F.,.F.,(4,1,1,1,1,4),(59.690260418206,
60.056092348402,60.5523666828758,61.0486410173496,61.5449153518233,61.915593798429),
 .UNSPECIFIED.);
#2893=B_SPLINE_CURVE_WITH_KNOTS('',3,(#19247,#19248,#19249,#19250,#19251,
#19252,#19253,#19254,#19255,#19256,#19257,#19258,#19259,#19260,#19261,#19262,
#19263,#19264,#19265,#19266,#19267,#19268,#19269,#19270,#19271,#19272,#19273,
#19274,#19275,#19276,#19277,#19278,#19279,#19280,#19281,#19282,#19283,#19284,
#19285,#19286,#19287,#19288,#19289,#19290,#19291,#19292,#19293,#19294,#19295,
#19296,#19297,#19298,#19299,#19300,#19301,#19302,#19303,#19304,#19305,#19306,
#19307,#19308,#19309,#19310,#19311,#19312,#19313,#19314,#19315,#19316,#19317,
#19318,#19319,#19320,#19321,#19322,#19323,#19324,#19325,#19326,#19327,#19328,
#19329,#19330,#19331,#19332,#19333,#19334,#19335,#19336,#19337,#19338,#19339,
#19340,#19341,#19342,#19343,#19344,#19345,#19346,#19347,#19348,#19349,#19350,
#19351,#19352,#19353,#19354,#19355,#19356,#19357,#19358,#19359,#19360,#19361,
#19362,#19363,#19364,#19365,#19366,#19367,#19368,#19369,#19370,#19371,#19372,
#19373,#19374,#19375,#19376,#19377,#19378,#19379,#19380,#19381,#19382,#19383,
#19384,#19385,#19386,#19387,#19388,#19389,#19390,#19391,#19392,#19393,#19394,
#19395,#19396,#19397,#19398,#19399,#19400,#19401,#19402,#19403,#19404,#19405,
#19406,#19407,#19408,#19409,#19410,#19411,#19412,#19413,#19414,#19415,#19416,
#19417,#19418),.UNSPECIFIED.,.F.,.F.,(4,3,3,3,3,3,3,3,3,3,3,3,3,3,3,3,3,
3,3,3,3,3,3,3,3,3,3,3,3,3,3,3,3,3,3,3,3,3,3,3,3,3,3,3,3,3,3,3,3,3,3,3,3,
3,3,3,3,4),(55.6324449452842,55.7099415050222,55.7874270322703,55.8649174558887,
55.9424051781908,56.0199114266392,56.0858976726116,56.1634027024354,56.2408936404985,
56.3183760229507,56.3958645509246,56.4733528638884,56.5508573318792,56.5821720070854,
56.6596770369092,56.7371679749723,56.8146503574246,56.8921388853984,56.9696271983623,
57.0471316663531,57.0784463415592,57.155951371383,57.2334423094461,57.3109246918983,
57.3884132198722,57.465901532836,57.5434060008268,57.574720676033,57.6522257058568,
57.7297166439199,57.8071990263723,57.8846875543461,57.96217586731,58.0396803353008,
58.0709950105068,58.1485000403306,58.2259909783937,58.3034733608458,58.3809618888196,
58.4584502017835,58.5359546697743,58.5672693449806,58.6447743748043,58.7222653128674,
58.7997476953199,58.8772362232938,58.9547245362576,59.0322290042483,59.0635436794544,
59.1410487092782,59.2185396473415,59.2960220297936,59.3735105577675,59.4509988707312,
59.528503338722,59.5598180139282,59.6410306749168,59.6902604165018),
 .UNSPECIFIED.);
#2894=B_SPLINE_CURVE_WITH_KNOTS('',3,(#19424,#19425,#19426,#19427,#19428,
#19429,#19430,#19431,#19432,#19433,#19434,#19435),.UNSPECIFIED.,.F.,.F.,
(4,1,1,1,1,1,1,1,1,4),(49.3492407452519,49.5717572337466,50.0680315682204,
50.5643059026942,51.060580237168,51.5568545716418,52.0531289061156,52.5494032405894,
53.0456775750632,53.4070751110264),.UNSPECIFIED.);
#2895=B_SPLINE_CURVE_WITH_KNOTS('',3,(#19436,#19437,#19438,#19439,#19440,
#19441,#19442,#19443,#19444,#19445,#19446,#19447,#19448,#19449,#19450,#19451,
#19452,#19453,#19454,#19455,#19456,#19457,#19458,#19459,#19460,#19461,#19462,
#19463,#19464,#19465,#19466,#19467,#19468,#19469,#19470,#19471,#19472,#19473,
#19474,#19475,#19476,#19477,#19478,#19479,#19480,#19481,#19482,#19483,#19484,
#19485,#19486,#19487,#19488,#19489,#19490,#19491,#19492,#19493,#19494,#19495,
#19496,#19497,#19498,#19499,#19500,#19501,#19502,#19503,#19504,#19505,#19506,
#19507,#19508,#19509,#19510,#19511,#19512,#19513,#19514,#19515,#19516,#19517,
#19518,#19519,#19520,#19521,#19522,#19523,#19524,#19525,#19526,#19527,#19528,
#19529,#19530,#19531,#19532),.UNSPECIFIED.,.F.,.F.,(4,3,3,3,3,3,3,3,3,3,
3,3,3,3,3,3,3,3,3,3,3,3,3,3,3,3,3,3,3,3,3,3,4),(53.40707511313,53.488147551321,
53.541951909537,53.6194569393608,53.6969478774239,53.7744302598764,53.8519187878503,
53.929407100814,54.0069115688048,54.0382262440108,54.1157312738346,54.1932222118976,
54.2707045943503,54.348193122324,54.425681435288,54.5031859032787,54.5345005784846,
54.6120056083084,54.6894965463715,54.7669789288238,54.8444674567977,54.9219557697616,
54.9994602377522,55.0307749129584,55.1082799427822,55.1857708808453,55.2632532632976,
55.3407417912714,55.4182301042351,55.4957345722259,55.5270492474322,55.6045536371399,
55.6324502817996),.UNSPECIFIED.);
#2896=B_SPLINE_CURVE_WITH_KNOTS('',3,(#19534,#19535,#19536,#19537,#19538,
#19539,#19540,#19541,#19542,#19543,#19544,#19545,#19546,#19547,#19548,#19549,
#19550,#19551,#19552,#19553,#19554,#19555,#19556,#19557,#19558,#19559,#19560,
#19561,#19562,#19563,#19564,#19565,#19566,#19567,#19568,#19569,#19570,#19571,
#19572,#19573,#19574,#19575,#19576,#19577,#19578,#19579,#19580,#19581,#19582,
#19583,#19584,#19585,#19586,#19587,#19588,#19589,#19590,#19591,#19592,#19593,
#19594,#19595,#19596,#19597,#19598,#19599,#19600,#19601,#19602,#19603,#19604,
#19605,#19606,#19607,#19608,#19609,#19610,#19611,#19612,#19613,#19614,#19615,
#19616,#19617,#19618,#19619,#19620,#19621,#19622,#19623,#19624,#19625,#19626,
#19627,#19628,#19629,#19630),.UNSPECIFIED.,.F.,.F.,(4,3,3,3,3,3,3,3,3,3,
3,3,3,3,3,3,3,3,3,3,3,3,3,3,3,3,3,3,3,3,3,3,4),(53.4070751110957,53.4864712424076,
53.5658927786533,53.6045260002426,53.6820310300664,53.7595219681295,53.8370043505816,
53.9144928785553,53.9919811915191,54.0694856595099,54.1008003347164,54.1783053645402,
54.2557963026032,54.3332786850558,54.4107672130297,54.4882555259938,54.5657599939845,
54.5970746691902,54.6745796990139,54.7520706370771,54.8295530195294,54.9070415475032,
54.9845298604671,55.0620343284579,55.093349003664,55.1708540334878,55.2483449715509,
55.3258273540031,55.403315881977,55.4808041949409,55.5583086629317,55.5896233381378,
55.6324449452842),.UNSPECIFIED.);
#2897=B_SPLINE_CURVE_WITH_KNOTS('',3,(#19631,#19632,#19633,#19634,#19635,
#19636,#19637,#19638,#19639,#19640,#19641,#19642,#19643,#19644,#19645,#19646,
#19647,#19648,#19649,#19650,#19651,#19652,#19653,#19654,#19655,#19656,#19657,
#19658,#19659,#19660,#19661,#19662,#19663,#19664,#19665,#19666,#19667,#19668,
#19669,#19670,#19671,#19672,#19673,#19674,#19675,#19676,#19677,#19678,#19679,
#19680,#19681,#19682,#19683,#19684,#19685,#19686,#19687,#19688,#19689,#19690,
#19691,#19692,#19693,#19694,#19695,#19696,#19697,#19698,#19699,#19700,#19701,
#19702,#19703,#19704,#19705,#19706,#19707,#19708,#19709,#19710,#19711,#19712,
#19713,#19714,#19715,#19716,#19717,#19718,#19719,#19720,#19721,#19722,#19723,
#19724,#19725,#19726,#19727,#19728,#19729,#19730,#19731,#19732,#19733,#19734,
#19735,#19736,#19737,#19738,#19739,#19740,#19741,#19742,#19743,#19744,#19745,
#19746,#19747,#19748,#19749,#19750,#19751,#19752,#19753,#19754,#19755,#19756,
#19757,#19758,#19759,#19760,#19761,#19762,#19763,#19764,#19765,#19766,#19767,
#19768,#19769,#19770,#19771,#19772,#19773,#19774,#19775,#19776,#19777,#19778,
#19779,#19780,#19781,#19782,#19783,#19784,#19785,#19786,#19787,#19788,#19789,
#19790,#19791,#19792,#19793,#19794,#19795,#19796,#19797,#19798,#19799,#19800,
#19801,#19802),.UNSPECIFIED.,.F.,.F.,(4,3,3,3,3,3,3,3,3,3,3,3,3,3,3,3,3,
3,3,3,3,3,3,3,3,3,3,3,3,3,3,3,3,3,3,3,3,3,3,3,3,3,3,3,3,3,3,3,3,3,3,3,3,
3,3,3,3,4),(49.3492546709687,49.4267442304708,49.5042320490615,49.581737396915,
49.6343313244523,49.7118363542761,49.7893272923391,49.8668096747915,49.9442982027653,
50.0217865157291,50.0992909837199,50.1306056589261,50.2081106887499,50.285601626813,
50.3630840092653,50.4405725372391,50.5180608502029,50.5955653181937,50.6268799933999,
50.7043850232237,50.7818759612868,50.8593583437391,50.9368468717129,51.0143351846768,
51.0918396526675,51.1231543278737,51.2006593576975,51.2781502957606,51.3556326782129,
51.4331212061867,51.5106095191505,51.5881139871414,51.6194286623475,51.6969336921713,
51.7744246302345,51.8519070126868,51.9293955406606,52.0068838536244,52.0843883216152,
52.1157029968213,52.1932080266451,52.2706989647081,52.3481813471605,52.4256698751343,
52.5031581880983,52.580662656089,52.6119773312951,52.6894823611189,52.7669732991819,
52.8444556816342,52.9219442096081,52.9994325225718,53.0769369905626,53.1082516657688,
53.1860463074653,53.2638247514645,53.3415977600619,53.4070751110264),
 .UNSPECIFIED.);
#2898=B_SPLINE_CURVE_WITH_KNOTS('',3,(#19808,#19809,#19810,#19811,#19812,
#19813,#19814,#19815,#19816,#19817,#19818,#19819,#19820,#19821,#19822,#19823,
#19824,#19825,#19826,#19827,#19828,#19829,#19830,#19831,#19832,#19833,#19834,
#19835,#19836,#19837,#19838,#19839,#19840,#19841,#19842,#19843,#19844,#19845,
#19846,#19847,#19848,#19849,#19850,#19851,#19852,#19853,#19854,#19855,#19856,
#19857,#19858,#19859,#19860,#19861,#19862,#19863,#19864,#19865,#19866,#19867,
#19868,#19869,#19870,#19871,#19872,#19873,#19874,#19875,#19876,#19877,#19878,
#19879,#19880,#19881,#19882,#19883,#19884,#19885,#19886,#19887,#19888,#19889,
#19890,#19891,#19892,#19893,#19894,#19895,#19896,#19897,#19898,#19899,#19900,
#19901,#19902,#19903,#19904,#19905,#19906,#19907,#19908,#19909,#19910,#19911,
#19912,#19913,#19914,#19915,#19916,#19917,#19918,#19919,#19920,#19921,#19922,
#19923,#19924,#19925,#19926,#19927,#19928,#19929,#19930,#19931,#19932,#19933,
#19934,#19935,#19936,#19937,#19938,#19939,#19940,#19941,#19942,#19943,#19944,
#19945,#19946,#19947,#19948,#19949,#19950,#19951,#19952,#19953,#19954,#19955,
#19956,#19957,#19958,#19959,#19960,#19961,#19962,#19963,#19964,#19965,#19966,
#19967,#19968,#19969,#19970,#19971,#19972,#19973,#19974,#19975,#19976,#19977,
#19978,#19979,#19980,#19981,#19982),.UNSPECIFIED.,.F.,.F.,(4,3,3,3,3,3,
3,3,3,3,3,3,3,3,3,3,3,3,3,3,3,3,3,3,3,3,3,3,3,3,3,3,3,3,3,3,3,3,3,3,3,3,
3,3,3,3,3,3,3,3,3,3,3,3,3,3,3,3,4),(43.0660500108131,43.1201908855873,43.1976959154111,
43.2751868534745,43.3526692359268,43.4301577639007,43.5076460768648,43.5851505448554,
43.6164652200611,43.6939702498849,43.7714611879481,43.8489435704003,43.9264320983741,
44.0039204113377,44.0814248793284,44.1127395545349,44.1902445843586,44.2677355224217,
44.3452179048738,44.4227064328476,44.5001947458119,44.5776992138026,44.6090138890087,
44.6865189188325,44.7640098568957,44.841492239348,44.9189807673218,44.9964690802853,
45.0739735482761,45.1052882234825,45.1827932533063,45.2602841913696,45.337766573823,
45.4152551017967,45.4927434147604,45.5702478827512,45.6015625579563,45.6790675877801,
45.7565585258428,45.8340409082948,45.9115294362686,45.9890177492321,46.0665222172227,
46.0978368924301,46.175341922254,46.252832860317,46.3303152427694,46.4078037707431,
46.4852920837064,46.5627965516972,46.5941112269039,46.6716162567278,46.7491071947912,
46.8265895772435,46.9040781052176,46.9815664181814,47.0590708861724,47.0903855613777,
47.1238898038468),.UNSPECIFIED.);
#2899=B_SPLINE_CURVE_WITH_KNOTS('',3,(#19983,#19984,#19985,#19986,#19987,
#19988,#19989,#19990),.UNSPECIFIED.,.F.,.F.,(4,1,1,1,1,4),(47.1238898363668,
47.5866598958514,48.0829342303252,48.579208564799,49.0754828992728,49.3492407452519),
 .UNSPECIFIED.);
#2900=B_SPLINE_CURVE_WITH_KNOTS('',3,(#19992,#19993,#19994,#19995,#19996,
#19997,#19998,#19999,#20000,#20001,#20002,#20003,#20004,#20005,#20006,#20007,
#20008,#20009,#20010,#20011,#20012,#20013,#20014,#20015,#20016,#20017,#20018,
#20019,#20020,#20021,#20022,#20023,#20024,#20025,#20026,#20027,#20028,#20029,
#20030,#20031,#20032,#20033,#20034,#20035,#20036,#20037,#20038,#20039,#20040,
#20041,#20042,#20043,#20044,#20045,#20046,#20047,#20048,#20049,#20050,#20051,
#20052,#20053,#20054,#20055,#20056,#20057,#20058,#20059,#20060,#20061,#20062,
#20063,#20064,#20065,#20066,#20067,#20068,#20069,#20070,#20071,#20072,#20073,
#20074,#20075,#20076,#20077,#20078,#20079,#20080,#20081,#20082,#20083,#20084,
#20085,#20086,#20087,#20088),.UNSPECIFIED.,.F.,.F.,(4,3,3,3,3,3,3,3,3,3,
3,3,3,3,3,3,3,3,3,3,3,3,3,3,3,3,3,3,3,3,3,3,4),(47.1238898038468,47.1529596520833,
47.2304646819071,47.3079556199699,47.3854380024221,47.462926530396,47.5404148433597,
47.6179193113505,47.6492339865571,47.7267390163809,47.8042299544441,47.8817123368962,
47.95920086487,48.0366891778341,48.1141936458248,48.1455083210309,48.2230133508547,
48.3005042889178,48.3779866713703,48.4554751993441,48.5329635123081,48.6104679802988,
48.6417826555047,48.7192876853285,48.7967786233916,48.8742610058439,48.9517495338177,
49.0292378467816,49.1067423147723,49.1380569899785,49.2155613837407,49.2930547509972,
49.3492546709687),.UNSPECIFIED.);
#2901=B_SPLINE_CURVE_WITH_KNOTS('',3,(#20089,#20090,#20091,#20092,#20093,
#20094,#20095,#20096,#20097,#20098,#20099,#20100),.UNSPECIFIED.,.F.,.F.,
(4,1,1,1,1,1,1,1,1,4),(43.0660378051096,43.1827649762929,43.6790393107667,
44.1753136452405,44.6715879797143,45.1678623141881,45.6641366486619,46.1604109831357,
46.6566853176095,47.1238897738335),.UNSPECIFIED.);
#2902=B_SPLINE_CURVE_WITH_KNOTS('',3,(#20106,#20107,#20108,#20109,#20110,
#20111,#20112,#20113,#20114,#20115,#20116,#20117),.UNSPECIFIED.,.F.,.F.,
(4,1,1,1,1,1,1,1,1,4),(36.7829030456445,37.1648988719018,37.6611732063756,
38.1574475408493,38.6537218753231,39.1499962097969,39.6462705442707,40.1425448787445,
40.6388192132183,40.8407044662609),.UNSPECIFIED.);
#2903=B_SPLINE_CURVE_WITH_KNOTS('',3,(#20118,#20119,#20120,#20121,#20122,
#20123,#20124,#20125,#20126,#20127,#20128,#20129,#20130,#20131,#20132,#20133,
#20134,#20135,#20136,#20137,#20138,#20139,#20140,#20141,#20142,#20143,#20144,
#20145,#20146,#20147,#20148,#20149,#20150,#20151,#20152,#20153,#20154,#20155,
#20156,#20157,#20158,#20159,#20160,#20161,#20162,#20163,#20164,#20165,#20166,
#20167,#20168,#20169,#20170,#20171,#20172,#20173,#20174,#20175,#20176,#20177,
#20178,#20179,#20180,#20181,#20182,#20183,#20184,#20185,#20186,#20187,#20188,
#20189,#20190,#20191,#20192,#20193,#20194,#20195,#20196,#20197,#20198,#20199,
#20200,#20201,#20202,#20203,#20204,#20205,#20206,#20207,#20208,#20209,#20210,
#20211),.UNSPECIFIED.,.F.,.F.,(4,3,3,3,3,3,3,3,3,3,3,3,3,3,3,3,3,3,3,3,
3,3,3,3,3,3,3,3,3,3,3,4),(40.8407044966673,40.9185261972124,40.9963482049705,
41.0741901903445,41.1350935476921,41.212598577516,41.2900895155792,41.3675718980314,
41.4450604260052,41.5225487389693,41.6000532069602,41.6313678821659,41.7088729119896,
41.7863638500527,41.8638462325043,41.9413347604782,42.0188230734419,42.0963275414328,
42.1276422166397,42.2051472464636,42.2826381845264,42.3601205669791,42.4376090949529,
42.5150974079168,42.5926018759076,42.6239165511135,42.701421064934,42.7789112992601,
42.8564006396014,42.9338846178947,43.0113808235583,43.0660500108131),
 .UNSPECIFIED.);
#2904=B_SPLINE_CURVE_WITH_KNOTS('',3,(#20213,#20214,#20215,#20216,#20217,
#20218,#20219,#20220),.UNSPECIFIED.,.F.,.F.,(4,1,1,1,1,4),(40.8407044966673,
41.1976676383978,41.6939419728716,42.1902163073454,42.6864906418191,43.0660378051096),
 .UNSPECIFIED.);
#2905=B_SPLINE_CURVE_WITH_KNOTS('',3,(#20221,#20222,#20223,#20224,#20225,
#20226,#20227,#20228,#20229,#20230,#20231,#20232,#20233,#20234,#20235,#20236,
#20237,#20238,#20239,#20240,#20241,#20242,#20243,#20244,#20245,#20246,#20247,
#20248,#20249,#20250,#20251,#20252,#20253,#20254,#20255,#20256,#20257,#20258,
#20259,#20260,#20261,#20262,#20263,#20264,#20265,#20266,#20267,#20268,#20269,
#20270,#20271,#20272,#20273,#20274,#20275,#20276,#20277,#20278,#20279,#20280,
#20281,#20282,#20283,#20284,#20285,#20286,#20287,#20288,#20289,#20290,#20291,
#20292,#20293,#20294,#20295,#20296,#20297,#20298,#20299,#20300,#20301,#20302,
#20303,#20304,#20305,#20306,#20307,#20308,#20309,#20310,#20311,#20312,#20313,
#20314,#20315,#20316,#20317,#20318,#20319,#20320,#20321,#20322,#20323,#20324,
#20325,#20326,#20327,#20328,#20329,#20330,#20331,#20332,#20333,#20334,#20335,
#20336,#20337,#20338,#20339,#20340,#20341,#20342,#20343,#20344,#20345,#20346,
#20347,#20348,#20349,#20350,#20351,#20352,#20353,#20354,#20355,#20356,#20357,
#20358,#20359,#20360,#20361,#20362,#20363,#20364,#20365,#20366,#20367,#20368,
#20369,#20370,#20371,#20372,#20373,#20374,#20375,#20376,#20377,#20378,#20379,
#20380,#20381,#20382,#20383,#20384,#20385,#20386,#20387,#20388,#20389,#20390,
#20391,#20392),.UNSPECIFIED.,.F.,.F.,(4,3,3,3,3,3,3,3,3,3,3,3,3,3,3,3,3,
3,3,3,3,3,3,3,3,3,3,3,3,3,3,3,3,3,3,3,3,3,3,3,3,3,3,3,3,3,3,3,3,3,3,3,3,
3,3,3,3,4),(36.7828905111531,36.8603855276508,36.9378701451936,37.0153599781323,
37.0928477456159,37.1703533678302,37.2274729626074,37.3049779924312,37.3824689304943,
37.4599513129466,37.5374398409205,37.6149281538843,37.6924326218751,37.7237472970812,
37.801252326905,37.8787432649681,37.9562256474204,38.0337141753942,38.111202488358,
38.1887069563488,38.220021631555,38.2975266613788,38.3750175994419,38.4524999818942,
38.529988509868,38.6074768228319,38.6849812908227,38.7162959660288,38.7938009958526,
38.8712919339157,38.9487743163681,39.0262628443419,39.1037511573058,39.1812556252966,
39.2125703005026,39.2900753303264,39.3675662683894,39.4450486508418,39.5225371788156,
39.6000254917794,39.6775299597702,39.7088446349764,39.7863496648002,39.8638406028632,
39.9413229853155,40.0188115132893,40.0962998262532,40.173804294244,40.2051189694502,
40.282623999274,40.3601149373372,40.4375973197892,40.5150858477629,40.592574160727,
40.6700786287177,40.701393303924,40.7823288599563,40.8407044942733),
 .UNSPECIFIED.);
#2906=B_SPLINE_CURVE_WITH_KNOTS('',3,(#20398,#20399,#20400,#20401,#20402,
#20403,#20404,#20405,#20406,#20407,#20408,#20409,#20410,#20411,#20412,#20413,
#20414,#20415,#20416,#20417,#20418,#20419,#20420,#20421,#20422,#20423,#20424,
#20425,#20426,#20427,#20428,#20429,#20430,#20431,#20432,#20433,#20434,#20435,
#20436,#20437,#20438,#20439,#20440,#20441,#20442,#20443,#20444,#20445,#20446,
#20447,#20448,#20449,#20450,#20451,#20452,#20453,#20454,#20455,#20456,#20457,
#20458,#20459,#20460,#20461,#20462,#20463,#20464,#20465,#20466,#20467,#20468,
#20469,#20470,#20471,#20472,#20473,#20474,#20475,#20476,#20477,#20478,#20479,
#20480,#20481,#20482,#20483,#20484,#20485,#20486,#20487,#20488,#20489,#20490,
#20491,#20492,#20493,#20494,#20495,#20496,#20497,#20498,#20499,#20500,#20501,
#20502,#20503,#20504,#20505,#20506,#20507,#20508,#20509,#20510,#20511,#20512,
#20513,#20514,#20515,#20516,#20517,#20518,#20519,#20520,#20521,#20522,#20523,
#20524,#20525,#20526,#20527,#20528,#20529,#20530,#20531,#20532,#20533,#20534,
#20535,#20536,#20537,#20538,#20539,#20540,#20541,#20542,#20543,#20544,#20545,
#20546,#20547,#20548,#20549,#20550,#20551,#20552,#20553,#20554,#20555,#20556,
#20557,#20558,#20559,#20560,#20561,#20562,#20563,#20564,#20565,#20566,#20567,
#20568,#20569),.UNSPECIFIED.,.F.,.F.,(4,3,3,3,3,3,3,3,3,3,3,3,3,3,3,3,3,
3,3,3,3,3,3,3,3,3,3,3,3,3,3,3,3,3,3,3,3,3,3,3,3,3,3,3,3,3,3,3,3,3,3,3,3,
3,3,3,3,4),(30.4996866134875,30.5771743679583,30.6546800900358,30.7133325237424,
30.7908375535663,30.8683284916292,30.9458108740808,31.0232994020546,31.1007877150188,
31.1782921830093,31.2096068582162,31.2871118880399,31.364602826103,31.4420852085554,
31.5195737365294,31.5970620494926,31.6745665174833,31.70588119269,31.7833862225136,
31.8608771605768,31.9383595430285,32.0158480710025,32.0933363839657,32.1708408519566,
32.2021555271638,32.2796605569876,32.3571514950511,32.4346338775035,32.5121224054774,
32.589610718441,32.6671151864316,32.6984298616376,32.7759348914614,32.8534258295247,
32.9309082119769,33.0083967399509,33.0858850529152,33.1633895209059,33.1947041961114,
33.2722092259351,33.3497001639985,33.4271825464495,33.5046710744235,33.5821593873876,
33.6596638553783,33.6909785305852,33.7684835604093,33.8459744984727,33.9234568809248,
34.0009454088985,34.078433721862,34.155938189853,34.187252865059,34.2645317736749,
34.341800711369,34.4190593754722,34.4963250242707,34.5575191894877),
 .UNSPECIFIED.);
#2907=B_SPLINE_CURVE_WITH_KNOTS('',3,(#20570,#20571,#20572,#20573,#20574,
#20575,#20576,#20577,#20578),.UNSPECIFIED.,.F.,.F.,(4,1,1,1,1,1,4),(34.5575191995802,
34.6835271995328,35.1798015340066,35.6760758684804,36.1723502029542,36.668624537428,
36.7829030456445),.UNSPECIFIED.);
#2908=B_SPLINE_CURVE_WITH_KNOTS('',3,(#20580,#20581,#20582,#20583,#20584,
#20585,#20586,#20587,#20588,#20589,#20590,#20591,#20592,#20593,#20594,#20595,
#20596,#20597,#20598,#20599,#20600,#20601,#20602,#20603,#20604,#20605,#20606,
#20607,#20608,#20609,#20610,#20611,#20612,#20613,#20614,#20615,#20616,#20617,
#20618,#20619,#20620,#20621,#20622,#20623,#20624,#20625,#20626,#20627,#20628,
#20629,#20630,#20631,#20632,#20633,#20634,#20635,#20636,#20637,#20638,#20639,
#20640,#20641,#20642,#20643,#20644,#20645,#20646,#20647,#20648,#20649,#20650,
#20651,#20652,#20653,#20654,#20655,#20656,#20657,#20658,#20659,#20660,#20661,
#20662,#20663,#20664,#20665,#20666,#20667,#20668,#20669,#20670,#20671,#20672,
#20673,#20674,#20675,#20676),.UNSPECIFIED.,.F.,.F.,(4,3,3,3,3,3,3,3,3,3,
3,3,3,3,3,3,3,3,3,3,3,3,3,3,3,3,3,3,3,3,3,3,4),(34.5575191941331,34.6371161377194,
34.7167383160435,34.7461012902384,34.8236063200621,34.9010972581253,34.9785796405779,
35.0560681685518,35.1335564815155,35.2110609495063,35.2423756247122,35.319880654536,
35.3973715925991,35.4748539750512,35.5523425030251,35.6298308159892,35.7073352839799,
35.738649959186,35.8161549890098,35.8936459270729,35.9711283095253,36.0486168374991,
36.1261051504629,36.2036096184536,36.2349242936598,36.3124293234836,36.3899202615467,
36.4674026439991,36.5448911719729,36.6223794849368,36.6998839529276,36.7311986281336,
36.7828905111531),.UNSPECIFIED.);
#2909=B_SPLINE_CURVE_WITH_KNOTS('',3,(#20677,#20678,#20679,#20680,#20681,
#20682,#20683,#20684,#20685,#20686,#20687,#20688),.UNSPECIFIED.,.F.,.F.,
(4,1,1,1,1,1,1,1,1,4),(30.4997008468882,30.7759066144481,31.2721809489219,
31.7684552833957,32.2647296178695,32.7610039523433,33.2572782868171,33.7535526212909,
34.2498269557646,34.5575191894877),.UNSPECIFIED.);
#2910=B_SPLINE_CURVE_WITH_KNOTS('',3,(#20694,#20695,#20696,#20697,#20698,
#20699,#20700,#20701,#20702,#20703,#20704,#20705,#20706),.UNSPECIFIED.,
 .F.,.F.,(4,1,1,1,1,1,1,1,1,1,4),(24.2164925491897,24.2617661755831,24.7580405100569,
25.2543148445307,25.7505891790045,26.2468635134783,26.7431378479521,27.2394121824259,
27.7356865168997,28.2319608513735,28.2743338823081),.UNSPECIFIED.);
#2911=B_SPLINE_CURVE_WITH_KNOTS('',3,(#20707,#20708,#20709,#20710,#20711,
#20712,#20713,#20714,#20715,#20716,#20717,#20718,#20719,#20720,#20721,#20722,
#20723,#20724,#20725,#20726,#20727,#20728,#20729,#20730,#20731,#20732,#20733,
#20734,#20735,#20736,#20737,#20738,#20739,#20740,#20741,#20742,#20743,#20744,
#20745,#20746,#20747,#20748,#20749,#20750,#20751,#20752,#20753,#20754,#20755,
#20756,#20757,#20758,#20759,#20760,#20761,#20762,#20763,#20764,#20765,#20766,
#20767,#20768,#20769,#20770,#20771,#20772,#20773,#20774,#20775,#20776,#20777,
#20778,#20779,#20780,#20781,#20782,#20783,#20784,#20785,#20786,#20787,#20788,
#20789,#20790,#20791,#20792,#20793,#20794,#20795,#20796,#20797,#20798,#20799,
#20800),.UNSPECIFIED.,.F.,.F.,(4,3,3,3,3,3,3,3,3,3,3,3,3,3,3,3,3,3,3,3,
3,3,3,3,3,3,3,3,3,3,3,4),(28.2743338823081,28.3516005304913,28.4288535310633,
28.5061092838686,28.5833615214816,28.6606328802227,28.7282351858473,28.805740215671,
28.8832311537342,28.9607135361864,29.0382020641603,29.1156903771241,29.1931948451148,
29.224509520321,29.3020145501449,29.379505488208,29.4569878706601,29.5344763986339,
29.6119647115976,29.6894691795883,29.7207838547948,29.7982888846186,29.8757798226816,
29.9532622051341,30.0307507331081,30.1082390460719,30.1857435140626,30.2170581892686,
30.2945642729969,30.3720550819576,30.4495420149547,30.4996866134875),
 .UNSPECIFIED.);
#2912=B_SPLINE_CURVE_WITH_KNOTS('',3,(#20802,#20803,#20804,#20805,#20806,
#20807,#20808,#20809,#20810),.UNSPECIFIED.,.F.,.F.,(4,1,1,1,1,1,4),(28.2743338823081,
28.2945349420791,28.7908092765529,29.2870836110267,29.7833579455005,30.2796322799743,
30.4997008468882),.UNSPECIFIED.);
#2913=B_SPLINE_CURVE_WITH_KNOTS('',3,(#20811,#20812,#20813,#20814,#20815,
#20816,#20817,#20818,#20819,#20820,#20821,#20822,#20823,#20824,#20825,#20826,
#20827,#20828,#20829,#20830,#20831,#20832,#20833,#20834,#20835,#20836,#20837,
#20838,#20839,#20840,#20841,#20842,#20843,#20844,#20845,#20846,#20847,#20848,
#20849,#20850,#20851,#20852,#20853,#20854,#20855,#20856,#20857,#20858,#20859,
#20860,#20861,#20862,#20863,#20864,#20865,#20866,#20867,#20868,#20869,#20870,
#20871,#20872,#20873,#20874,#20875,#20876,#20877,#20878,#20879,#20880,#20881,
#20882,#20883,#20884,#20885,#20886,#20887,#20888,#20889,#20890,#20891,#20892,
#20893,#20894,#20895,#20896,#20897,#20898,#20899,#20900,#20901,#20902,#20903,
#20904,#20905,#20906,#20907,#20908,#20909,#20910,#20911,#20912,#20913,#20914,
#20915,#20916,#20917,#20918,#20919,#20920,#20921,#20922,#20923,#20924,#20925,
#20926,#20927,#20928,#20929,#20930,#20931,#20932,#20933,#20934,#20935,#20936,
#20937,#20938,#20939,#20940,#20941,#20942,#20943,#20944,#20945,#20946,#20947,
#20948,#20949,#20950,#20951,#20952,#20953,#20954,#20955,#20956,#20957,#20958,
#20959,#20960,#20961,#20962,#20963,#20964,#20965,#20966,#20967,#20968,#20969,
#20970,#20971,#20972,#20973,#20974,#20975,#20976,#20977,#20978,#20979,#20980,
#20981,#20982,#20983,#20984,#20985),.UNSPECIFIED.,.F.,.F.,(4,3,3,3,3,3,
3,3,3,3,3,3,3,3,3,3,3,3,3,3,3,3,3,3,3,3,3,3,3,3,3,3,3,3,3,3,3,3,3,3,3,3,
3,3,3,3,3,3,3,3,3,3,3,3,3,3,3,3,4),(24.2164906146016,24.293995059513,24.3243402662887,
24.4018452953929,24.4793362327265,24.5568186144429,24.6343071416759,24.7117954538968,
24.7892999211475,24.8206146007625,24.8981196310086,24.9756105694992,25.0530929523823,
25.1305814807896,25.2080697941879,25.285574262611,25.3168889352363,25.3943939648685,
25.4718849027378,25.5493672849951,25.6268558127727,25.7043441255404,25.7818485933357,
25.8131632697101,25.8906682995953,25.9681592377207,26.0456416202358,26.1231301482722,
26.2006184612982,26.2781229293511,26.3094376041839,26.3869426340027,26.4644335720607,
26.5419159545076,26.6194044824769,26.6968927954367,26.7743972634227,26.8057119386577,
26.8832169684698,26.9607079065205,27.0381902889601,27.1156788169219,27.1931671298729,
27.2706715978511,27.3019862731315,27.3794913029673,27.4569822410422,27.5344646235078,
27.6119531514941,27.6894414644704,27.7669459324735,27.7982606076053,27.8756329726693,
27.952990826376,28.033326590359,28.1106815343842,28.1880375066588,28.2654085791595,
28.2743338823081),.UNSPECIFIED.);
#2914=B_SPLINE_CURVE_WITH_KNOTS('',3,(#20991,#20992,#20993,#20994,#20995,
#20996,#20997,#20998,#20999),.UNSPECIFIED.,.F.,.F.,(4,1,1,1,1,1,4),(15.7079632679489,
15.8876765802342,16.383950914708,16.8802252491818,17.3764995836556,17.8727739181294,
17.9333400728794),.UNSPECIFIED.);
#2915=B_SPLINE_CURVE_WITH_KNOTS('',3,(#21001,#21002,#21003,#21004,#21005,
#21006),.UNSPECIFIED.,.F.,.F.,(4,1,1,4),(14.3988535768129,14.8951279112866,
15.3914022457604,15.7079632679489),.UNSPECIFIED.);
#2916=B_SPLINE_CURVE_WITH_KNOTS('',3,(#21010,#21011,#21012,#21013,#21014,
#21015,#21016,#21017,#21018,#21019,#21020,#21021,#21022,#21023,#21024,#21025,
#21026,#21027,#21028,#21029,#21030,#21031,#21032,#21033,#21034,#21035,#21036,
#21037,#21038,#21039,#21040,#21041,#21042,#21043,#21044,#21045,#21046,#21047,
#21048,#21049,#21050,#21051,#21052,#21053,#21054,#21055,#21056,#21057,#21058,
#21059,#21060,#21061,#21062,#21063,#21064,#21065,#21066,#21067,#21068,#21069,
#21070,#21071,#21072,#21073,#21074,#21075,#21076,#21077,#21078,#21079,#21080,
#21081,#21082,#21083,#21084,#21085),.UNSPECIFIED.,.F.,.F.,(4,3,3,3,3,3,
3,3,3,3,3,3,3,3,3,3,3,3,3,3,3,3,3,3,3,4),(13.8754803054952,13.9527915991825,
14.0300891179163,14.1073893679387,14.1846856665792,14.2620014441097,14.3362794861072,
14.4137829478898,14.4912723246912,14.5687531577414,14.6462401656036,14.7237269782611,
14.801229985091,14.832553820581,14.9100553301433,14.987542692496,15.0650214555568,
15.142506326132,15.2199909664686,15.2974917626711,15.3288281550548,15.4060793552377,
15.4833212986073,15.5605530255635,15.6377935536614,15.7079632679489),
 .UNSPECIFIED.);
#2917=B_SPLINE_CURVE_WITH_KNOTS('',3,(#21086,#21087,#21088,#21089,#21090,
#21091,#21092,#21093,#21094,#21095,#21096,#21097,#21098,#21099,#21100,#21101,
#21102,#21103,#21104,#21105,#21106,#21107,#21108,#21109,#21110,#21111,#21112,
#21113,#21114,#21115,#21116,#21117,#21118,#21119,#21120,#21121,#21122,#21123,
#21124,#21125,#21126,#21127,#21128,#21129,#21130,#21131,#21132,#21133,#21134,
#21135,#21136,#21137,#21138,#21139,#21140,#21141,#21142,#21143,#21144,#21145,
#21146,#21147,#21148,#21149,#21150,#21151,#21152,#21153,#21154,#21155,#21156,
#21157,#21158,#21159,#21160,#21161,#21162,#21163,#21164,#21165,#21166,#21167,
#21168,#21169,#21170,#21171,#21172,#21173,#21174,#21175,#21176,#21177,#21178,
#21179,#21180,#21181,#21182),.UNSPECIFIED.,.F.,.F.,(4,3,3,3,3,3,3,3,3,3,
3,3,3,3,3,3,3,3,3,3,3,3,3,3,3,3,3,3,3,3,3,3,4),(15.7079632680288,15.7896238438224,
15.8251024895286,15.9026051904092,15.9800937703955,16.0575737733851,16.1350599078411,
16.2125458235925,16.2900479042311,16.3213768240024,16.3988830078092,16.4763751134108,
16.5538586731209,16.6313483840178,16.7088378809863,16.7863435270014,16.8176511584762,
16.895155760811,16.9726462668389,17.0501282141283,17.1276163055372,17.2051041819359,
17.2826082161604,17.31392549295,17.3914306039829,17.4689216237793,17.5464040882215,
17.6238926979533,17.7013810923885,17.7788856409009,17.8101998274238,17.8877048528018,
17.9333380487234),.UNSPECIFIED.);
#2918=B_SPLINE_CURVE_WITH_KNOTS('',3,(#21188,#21189,#21190,#21191,#21192,
#21193,#21194,#21195),.UNSPECIFIED.,.F.,.F.,(4,2,2,4),(-0.24984933934325,
-0.173343887030935,-0.120986450366014,-5.83022767437317E-5),
 .UNSPECIFIED.);
#2919=B_SPLINE_CURVE_WITH_KNOTS('',3,(#21198,#21199,#21200,#21201,#21202,
#21203,#21204,#21205,#21206,#21207,#21208,#21209,#21210,#21211,#21212,#21213,
#21214,#21215,#21216,#21217,#21218,#21219,#21220,#21221,#21222,#21223,#21224,
#21225,#21226,#21227,#21228,#21229,#21230,#21231,#21232,#21233,#21234,#21235,
#21236,#21237,#21238,#21239,#21240,#21241,#21242,#21243,#21244,#21245,#21246,
#21247,#21248,#21249,#21250,#21251,#21252,#21253,#21254,#21255,#21256,#21257,
#21258,#21259,#21260,#21261,#21262,#21263,#21264,#21265,#21266,#21267,#21268,
#21269,#21270,#21271,#21272,#21273,#21274,#21275,#21276,#21277,#21278,#21279,
#21280,#21281,#21282,#21283,#21284,#21285),.UNSPECIFIED.,.F.,.F.,(4,3,3,
3,3,3,3,3,3,3,3,3,3,3,3,3,3,3,3,3,3,3,3,3,3,3,3,3,3,4),(-75.398223608073,
-75.318009037967,-75.2378091726219,-75.1576065863558,-75.0774076436808,
-74.9971894012001,-74.937424505543,-74.8570105508218,-74.7766116468169,
-74.69274627788,-74.6123498096441,-74.5319524963766,-74.4515392340459,-74.4411501710692,
-74.3607382418802,-74.2803414302624,-74.1964750318456,-74.1160807873363,
-74.0356857342678,-73.9552747701957,-73.9448758365954,-73.8644565163834,
-73.7840522023662,-73.700189527305,-73.6197876282239,-73.539384899434,-73.4589662739223,
-73.4486015021216,-73.3682988747528,-73.3238177496334),.UNSPECIFIED.);
#2920=B_SPLINE_CURVE_WITH_KNOTS('',3,(#21290,#21291,#21292,#21293,#21294,
#21295,#21296,#21297,#21298,#21299,#21300,#21301,#21302,#21303,#21304,#21305,
#21306,#21307,#21308,#21309,#21310,#21311,#21312,#21313,#21314,#21315,#21316,
#21317,#21318,#21319,#21320,#21321,#21322,#21323,#21324,#21325,#21326,#21327,
#21328,#21329,#21330,#21331,#21332,#21333,#21334,#21335,#21336,#21337,#21338,
#21339,#21340,#21341,#21342,#21343,#21344,#21345,#21346,#21347,#21348,#21349,
#21350,#21351,#21352,#21353,#21354,#21355,#21356,#21357,#21358,#21359,#21360,
#21361,#21362,#21363,#21364,#21365,#21366,#21367,#21368,#21369,#21370,#21371,
#21372,#21373,#21374,#21375,#21376,#21377,#21378,#21379,#21380,#21381,#21382,
#21383,#21384,#21385,#21386,#21387,#21388,#21389,#21390,#21391,#21392,#21393,
#21394,#21395,#21396,#21397,#21398,#21399,#21400,#21401,#21402,#21403,#21404,
#21405,#21406,#21407,#21408,#21409,#21410,#21411,#21412,#21413,#21414,#21415,
#21416,#21417,#21418,#21419,#21420,#21421,#21422,#21423,#21424,#21425,#21426,
#21427,#21428,#21429,#21430,#21431,#21432,#21433,#21434,#21435,#21436,#21437,
#21438,#21439,#21440,#21441,#21442,#21443),.UNSPECIFIED.,.F.,.F.,(4,2,2,
2,2,2,2,2,2,2,2,2,2,2,2,2,2,2,2,2,2,2,2,2,2,2,2,2,2,2,2,2,2,2,2,2,2,2,2,
2,2,2,2,2,2,2,2,2,2,2,2,2,2,2,2,2,2,2,2,2,2,2,2,2,2,2,2,2,2,2,2,2,2,2,2,
2,4),(-4.6604807148913,-4.61334475694576,-4.55984181574834,-4.53242377612221,
-4.5107875949951,-4.42356313296582,-4.35683282385191,-4.29437188688845,
-4.20601588083401,-4.17280892017205,-4.11426280773656,-4.04896992918726,
-3.99267617112123,-3.91273796752958,-3.86163756290624,-3.82680962834829,
-3.77698350095406,-3.70606384614301,-3.64832213371534,-3.53312480790826,
-3.50975322979048,-3.4763685978861,-3.41697863169213,-3.351940989318,-3.29570890247222,
-3.21866506262813,-3.16591823667992,-3.13061402538623,-3.06420103444955,
-3.02019411022275,-2.95843573977559,-2.83467487239128,-2.78861356788968,
-2.7491478137684,-2.668206714305,-2.60791226229094,-2.49096078734472,-2.45512420992431,
-2.42379811483375,-2.40623558811782,-2.34983856552957,-2.27766018523853,
-2.22111731642953,-2.15489946542858,-2.09929972861543,-2.06675245307284,
-1.98003559810137,-1.91589221954151,-1.85163962848125,-1.76974127329886,
-1.73549093138055,-1.67210578483828,-1.57986492237622,-1.52261465929151,
-1.45413293650151,-1.39911962377229,-1.36454975712187,-1.31406964444337,
-1.23315151866149,-1.17747412332377,-1.11354560615875,-1.05123048084556,
-1.01671421042371,-0.966982982709164,-0.883978144907126,-0.826699521657825,
-0.758975125168801,-0.704205029792625,-0.670313095416478,-0.646154031014603,
-0.534877130256036,-0.483215096994178,-0.419123134283916,-0.357410058846901,
-0.328069350014561,-0.290289649212232,-0.24984933934325),.UNSPECIFIED.);
#2921=B_SPLINE_CURVE_WITH_KNOTS('',3,(#21445,#21446,#21447,#21448,#21449,
#21450,#21451,#21452,#21453,#21454,#21455,#21456,#21457,#21458,#21459,#21460),
 .UNSPECIFIED.,.F.,.F.,(4,3,3,3,3,4),(-73.3238177496334,-73.2435365115161,
-73.1632507410983,-73.0829664079746,-73.0026647607017,-72.9680938357794),
 .UNSPECIFIED.);
#2922=B_SPLINE_CURVE_WITH_KNOTS('',3,(#21461,#21462,#21463,#21464,#21465,
#21466,#21467,#21468,#21469,#21470,#21471,#21472,#21473,#21474,#21475,#21476,
#21477),.UNSPECIFIED.,.F.,.F.,(4,2,1,1,1,1,1,1,1,1,1,1,1,4),(-72.9680938331862,
-72.9523271676478,-72.456052833174,-71.9597784987002,-71.4635041642264,
-70.9672298297526,-70.4709554952788,-69.974681160805,-69.4784068263312,
-68.9821324918575,-68.4858581573837,-67.9895838229099,-67.4933094884361,
-67.0406615200402),.UNSPECIFIED.);
#2923=B_SPLINE_CURVE_WITH_KNOTS('',3,(#21483,#21484,#21485,#21486,#21487,
#21488,#21489,#21490,#21491,#21492,#21493,#21494,#21495,#21496,#21497,#21498),
 .UNSPECIFIED.,.F.,.F.,(4,1,1,1,1,1,1,1,1,1,1,1,1,4),(64.4966950710674,
64.5156634815933,65.0119378160671,65.5082121505409,66.0044864850147,66.5007608194885,
66.9970351539623,67.4933094884361,67.9895838229099,68.4858581573837,68.9821324918575,
69.4784068263313,69.9746811608051,70.4241480285323),.UNSPECIFIED.);
#2924=B_SPLINE_CURVE_WITH_KNOTS('',3,(#21499,#21500,#21501,#21502,#21503,
#21504,#21505,#21506,#21507,#21508,#21509,#21510),.UNSPECIFIED.,.F.,.F.,
(4,2,2,2,2,4),(-4.91020706723789,-4.88001929369499,-4.84959643912597,-4.74176696137822,
-4.68911415734267,-4.6604807148913),.UNSPECIFIED.);
#2925=B_SPLINE_CURVE_WITH_KNOTS('',3,(#21512,#21513,#21514,#21515,#21516),
 .UNSPECIFIED.,.F.,.F.,(4,1,4),(-67.0406615200402,-66.9970351539623,-66.6849085260066),
 .UNSPECIFIED.);
#2926=B_SPLINE_CURVE_WITH_KNOTS('',3,(#21517,#21518,#21519,#21520,#21521,
#21522,#21523,#21524,#21525,#21526,#21527,#21528,#21529,#21530,#21531,#21532,
#21533,#21534,#21535,#21536,#21537,#21538,#21539,#21540,#21541,#21542,#21543,
#21544,#21545,#21546,#21547,#21548,#21549,#21550,#21551,#21552,#21553,#21554,
#21555,#21556,#21557,#21558,#21559,#21560,#21561,#21562,#21563,#21564,#21565,
#21566,#21567,#21568,#21569,#21570,#21571,#21572,#21573,#21574,#21575,#21576,
#21577,#21578,#21579,#21580,#21581,#21582,#21583,#21584,#21585,#21586,#21587,
#21588,#21589,#21590,#21591,#21592,#21593,#21594,#21595,#21596,#21597,#21598,
#21599,#21600,#21601,#21602,#21603,#21604,#21605,#21606,#21607,#21608,#21609,
#21610,#21611,#21612,#21613,#21614,#21615,#21616,#21617,#21618,#21619,#21620,
#21621,#21622,#21623,#21624,#21625,#21626,#21627,#21628,#21629,#21630,#21631,
#21632,#21633,#21634,#21635,#21636,#21637,#21638,#21639,#21640,#21641,#21642,
#21643,#21644,#21645,#21646,#21647,#21648,#21649,#21650,#21651,#21652,#21653,
#21654,#21655,#21656,#21657,#21658,#21659,#21660,#21661,#21662,#21663,#21664,
#21665,#21666,#21667,#21668,#21669,#21670,#21671,#21672,#21673,#21674,#21675,
#21676,#21677,#21678,#21679,#21680,#21681,#21682,#21683,#21684,#21685,#21686,
#21687,#21688,#21689,#21690,#21691,#21692,#21693,#21694,#21695,#21696,#21697,
#21698,#21699,#21700,#21701,#21702,#21703,#21704,#21705,#21706,#21707,#21708,
#21709,#21710,#21711,#21712,#21713,#21714,#21715,#21716,#21717,#21718,#21719,
#21720,#21721,#21722,#21723,#21724,#21725,#21726,#21727,#21728,#21729,#21730,
#21731,#21732,#21733,#21734,#21735,#21736,#21737,#21738,#21739,#21740,#21741,
#21742,#21743,#21744,#21745,#21746,#21747,#21748,#21749,#21750,#21751,#21752,
#21753,#21754,#21755,#21756,#21757,#21758,#21759,#21760,#21761,#21762,#21763,
#21764,#21765,#21766,#21767,#21768,#21769),.UNSPECIFIED.,.F.,.F.,(4,3,3,
3,3,3,3,3,3,3,3,3,3,3,3,3,3,3,3,3,3,3,3,3,3,3,3,3,3,3,3,3,3,3,3,3,3,3,3,
3,3,3,3,3,3,3,3,3,3,3,3,3,3,3,3,3,3,3,3,3,3,3,3,3,3,3,3,3,3,3,3,3,3,3,3,
3,3,3,3,3,3,3,3,3,4),(-66.6849085260066,-66.6022141450956,-66.5194935653768,
-66.5007608194885,-66.4203452380402,-66.3399447147115,-66.2560801572873,
-66.175682114948,-66.0952832498526,-66.0148684756778,-66.0044864850147,
-65.9240709033037,-65.8436703797093,-65.7598058224172,-65.6794077798094,
-65.599008914445,-65.5185941400035,-65.5082121505409,-65.4277965688989,
-65.3473960453742,-65.2635314880474,-65.1831334455096,-65.1027345802153,
-65.0223198058429,-65.0119378160671,-64.9315222344323,-64.8511217109148,
-64.7672571535845,-64.6868591110544,-64.6064602457679,-64.5260454714036,
-64.5156634815933,-64.4352478999337,-64.3548473763912,-64.2709828190733,
-64.1905847765176,-64.1101859112055,-64.0297711368156,-64.0193891471195,
-63.9389735654804,-63.8585730419587,-63.7747084846305,-63.6943104420959,
-63.6139115768051,-63.5334968024362,-63.5231148126457,-63.4426992309946,
-63.3622987074607,-63.2784341501385,-63.1980361075916,-63.1176372422883,
-63.0372224679071,-63.0268404781719,-62.9464248965263,-62.8660243729978,
-62.7821598156729,-62.7017617731316,-62.6213629078341,-62.5409481334585,
-62.5305661436981,-62.4501505620507,-62.3697500385205,-62.2858854811964,
-62.2054874386533,-62.125088573354,-62.0446737989765,-62.0342918092243,
-61.953876227577,-61.873475704047,-61.7896111467229,-61.7092131041798,-61.6288142388805,
-61.5483994645032,-61.5380174747505,-61.4576018931038,-61.3772013695742,
-61.2933368122498,-61.2129387697073,-61.1325399044087,-61.0521251300321,
-61.0417431402768,-60.9613264014195,-60.8809260071003,-60.8005299808948,
-60.7574681838464),.UNSPECIFIED.);
#2927=B_SPLINE_CURVE_WITH_KNOTS('',3,(#21775,#21776,#21777,#21778,#21779,
#21780,#21781,#21782,#21783,#21784,#21785,#21786,#21787,#21788,#21789,#21790,
#21791,#21792,#21793,#21794,#21795,#21796,#21797,#21798,#21799,#21800,#21801,
#21802,#21803,#21804,#21805,#21806,#21807,#21808,#21809,#21810,#21811,#21812,
#21813,#21814,#21815,#21816,#21817,#21818,#21819,#21820,#21821,#21822,#21823,
#21824,#21825,#21826,#21827,#21828,#21829,#21830,#21831,#21832,#21833,#21834,
#21835,#21836,#21837,#21838,#21839,#21840,#21841,#21842,#21843,#21844,#21845,
#21846,#21847,#21848,#21849,#21850,#21851,#21852,#21853,#21854,#21855,#21856,
#21857,#21858,#21859,#21860,#21861,#21862,#21863,#21864,#21865,#21866,#21867,
#21868,#21869,#21870,#21871,#21872,#21873,#21874,#21875,#21876,#21877,#21878,
#21879,#21880,#21881,#21882,#21883,#21884,#21885,#21886,#21887,#21888,#21889,
#21890,#21891,#21892,#21893,#21894,#21895,#21896,#21897,#21898,#21899,#21900,
#21901,#21902,#21903,#21904,#21905,#21906,#21907,#21908,#21909,#21910,#21911,
#21912,#21913,#21914,#21915,#21916,#21917,#21918,#21919,#21920,#21921,#21922,
#21923,#21924,#21925,#21926,#21927,#21928,#21929,#21930,#21931,#21932,#21933,
#21934,#21935,#21936,#21937,#21938,#21939,#21940,#21941,#21942,#21943,#21944,
#21945,#21946,#21947,#21948,#21949,#21950,#21951,#21952,#21953,#21954,#21955,
#21956,#21957,#21958,#21959,#21960,#21961,#21962,#21963,#21964,#21965,#21966,
#21967,#21968,#21969,#21970,#21971,#21972,#21973,#21974,#21975,#21976,#21977,
#21978,#21979,#21980,#21981,#21982,#21983,#21984,#21985,#21986,#21987,#21988,
#21989,#21990,#21991,#21992,#21993,#21994,#21995,#21996,#21997,#21998,#21999,
#22000,#22001,#22002,#22003,#22004,#22005,#22006,#22007,#22008,#22009,#22010,
#22011,#22012,#22013,#22014,#22015,#22016,#22017,#22018,#22019,#22020,#22021,
#22022,#22023,#22024,#22025,#22026,#22027),.UNSPECIFIED.,.F.,.F.,(4,3,3,
3,3,3,3,3,3,3,3,3,3,3,3,3,3,3,3,3,3,3,3,3,3,3,3,3,3,3,3,3,3,3,3,3,3,3,3,
3,3,3,3,3,3,3,3,3,3,3,3,3,3,3,3,3,3,3,3,3,3,3,3,3,3,3,3,3,3,3,3,3,3,3,3,
3,3,3,3,3,3,3,3,3,4),(58.2135306995125,58.2939232292864,58.3743217990603,
58.4547200449574,58.5351349677853,58.5603714679078,58.6407870495549,58.7211875730847,
58.8050521304089,58.8854501729518,58.9658490382507,59.0462638126277,59.0566458023816,
59.1370613840286,59.2174619075586,59.3013264648828,59.3817245074256,59.4621233727246,
59.5425381471016,59.5529201368554,59.6333357185025,59.7137362420324,59.7976007993566,
59.8779988418995,59.9583977071986,60.0388124815757,60.0491944713292,60.1296100529762,
60.210010576506,60.2938751338303,60.374273176373,60.4546720416721,60.5350868160491,
60.545468805803,60.6258843874502,60.7062849109802,60.7901494683044,60.8705475108473,
60.9509463761467,61.0313611505239,61.0417431402768,61.1221587219237,61.2025592454535,
61.2864238027778,61.3668218453204,61.4472207106195,61.5276354849965,61.5380174747506,
61.6184330563977,61.6988335799276,61.7826981372518,61.8630961797946,61.9434950450938,
62.023909819471,62.0342918092243,62.1147073908717,62.195107914402,62.278972471726,
62.3593705142691,62.4397693795688,62.5201841539462,62.5305661436981,62.6109817253437,
62.6913822488721,62.7752468061971,62.8556448487385,62.9360437140362,63.0164584884119,
63.0268404781719,63.107256059823,63.187656583357,63.2715211406792,63.351919183226,
63.4323180485291,63.5127328229102,63.5231148126457,63.6035303942844,63.683930917806,
63.7677954751344,63.8481935176689,63.9285923829598,64.0090071573289,64.0193891471195,
64.1039532538953,64.1409627629319),.UNSPECIFIED.);
#2928=B_SPLINE_CURVE_WITH_KNOTS('',3,(#22028,#22029,#22030,#22031),
 .UNSPECIFIED.,.F.,.F.,(4,4),(64.1409627629319,64.4966950710674),
 .UNSPECIFIED.);
#2929=B_SPLINE_CURVE_WITH_KNOTS('',3,(#22033,#22034,#22035,#22036,#22037,
#22038,#22039,#22040,#22041,#22042,#22043,#22044,#22045,#22046,#22047,#22048),
 .UNSPECIFIED.,.F.,.F.,(4,3,3,3,3,4),(-60.7574681838464,-60.6770705117027,
-60.5966545091061,-60.545468805803,-60.4616324956271,-60.401723218827),
 .UNSPECIFIED.);
#2930=B_SPLINE_CURVE_WITH_KNOTS('',3,(#22049,#22050,#22051,#22052,#22053,
#22054,#22055,#22056,#22057,#22058,#22059,#22060,#22061,#22062,#22063,#22064),
 .UNSPECIFIED.,.F.,.F.,(4,1,1,1,1,1,1,1,1,1,1,1,1,4),(-60.401723218827,
-60.0491944713291,-59.5529201368554,-59.0566458023816,-58.5603714679078,
-58.064097133434,-57.5678227989602,-57.0715484644864,-56.5752741300126,
-56.0789997955388,-55.582725461065,-55.0864511265912,-54.5901767921174,
-54.4742514652626),.UNSPECIFIED.);
#2931=B_SPLINE_CURVE_WITH_KNOTS('',3,(#22070,#22071,#22072,#22073,#22074,
#22075,#22076,#22077,#22078,#22079,#22080,#22081,#22082,#22083,#22084,#22085),
 .UNSPECIFIED.,.F.,.F.,(4,1,1,1,1,1,1,1,1,1,1,1,1,4),(51.9303121562591,
52.1088051197484,52.6050794542222,53.101353788696,53.5976281231698,54.0939024576436,
54.5901767921174,55.0864511265912,55.582725461065,56.0789997955388,56.5752741300126,
57.0715484644864,57.5678227989602,57.8577774557523),.UNSPECIFIED.);
#2932=B_SPLINE_CURVE_WITH_KNOTS('',3,(#22086,#22087,#22088,#22089,#22090,
#22091,#22092,#22093,#22094,#22095,#22096,#22097,#22098,#22099,#22100,#22101),
 .UNSPECIFIED.,.F.,.F.,(4,3,3,3,3,4),(57.8577774557523,57.9399575861014,
58.0221642585411,58.064097133434,58.1445144829838,58.2135306995125),
 .UNSPECIFIED.);
#2933=B_SPLINE_CURVE_WITH_KNOTS('',3,(#22103,#22104,#22105,#22106),
 .UNSPECIFIED.,.F.,.F.,(4,4),(-54.4742514652626,-54.118537942137),
 .UNSPECIFIED.);
#2934=B_SPLINE_CURVE_WITH_KNOTS('',3,(#22107,#22108,#22109,#22110,#22111,
#22112,#22113,#22114,#22115,#22116,#22117,#22118,#22119,#22120,#22121,#22122,
#22123,#22124,#22125,#22126,#22127,#22128,#22129,#22130,#22131,#22132,#22133,
#22134,#22135,#22136,#22137,#22138,#22139,#22140,#22141,#22142,#22143,#22144,
#22145,#22146,#22147,#22148,#22149,#22150,#22151,#22152,#22153,#22154,#22155,
#22156,#22157,#22158,#22159,#22160,#22161,#22162,#22163,#22164,#22165,#22166,
#22167,#22168,#22169,#22170,#22171,#22172,#22173,#22174,#22175,#22176,#22177,
#22178,#22179,#22180,#22181,#22182,#22183,#22184,#22185,#22186,#22187,#22188,
#22189,#22190,#22191,#22192,#22193,#22194,#22195,#22196,#22197,#22198,#22199,
#22200,#22201,#22202,#22203,#22204,#22205,#22206,#22207,#22208,#22209,#22210,
#22211,#22212,#22213,#22214,#22215,#22216,#22217,#22218,#22219,#22220,#22221,
#22222,#22223,#22224,#22225,#22226,#22227,#22228,#22229,#22230,#22231,#22232,
#22233,#22234,#22235,#22236,#22237,#22238,#22239,#22240,#22241,#22242,#22243,
#22244,#22245,#22246,#22247,#22248,#22249,#22250,#22251,#22252,#22253,#22254,
#22255,#22256,#22257,#22258,#22259,#22260,#22261,#22262,#22263,#22264,#22265,
#22266,#22267,#22268,#22269,#22270,#22271,#22272,#22273,#22274,#22275,#22276,
#22277,#22278,#22279,#22280,#22281,#22282,#22283,#22284,#22285,#22286,#22287,
#22288,#22289,#22290,#22291,#22292,#22293,#22294,#22295,#22296,#22297,#22298,
#22299,#22300,#22301,#22302,#22303,#22304,#22305,#22306,#22307,#22308,#22309,
#22310,#22311,#22312,#22313,#22314,#22315,#22316,#22317,#22318,#22319,#22320,
#22321,#22322,#22323,#22324,#22325,#22326,#22327,#22328,#22329,#22330,#22331,
#22332,#22333,#22334,#22335,#22336,#22337,#22338,#22339,#22340,#22341,#22342,
#22343,#22344,#22345,#22346,#22347,#22348,#22349,#22350,#22351,#22352,#22353,
#22354,#22355,#22356,#22357,#22358,#22359),.UNSPECIFIED.,.F.,.F.,(4,3,3,
3,3,3,3,3,3,3,3,3,3,3,3,3,3,3,3,3,3,3,3,3,3,3,3,3,3,3,3,3,3,3,3,3,3,3,3,
3,3,3,3,3,3,3,3,3,3,3,3,3,3,3,3,3,3,3,3,3,3,3,3,3,3,3,3,3,3,3,3,3,3,3,3,
3,3,3,3,3,3,3,3,3,4),(-54.1185379116474,-54.0939024576436,-54.0134868759983,
-53.9330863524702,-53.8492217951451,-53.768823752604,-53.6884248873065,
-53.6080101129313,-53.5976281231698,-53.517212541522,-53.4368120179915,
-53.3529474606676,-53.2725494181242,-53.1921505528245,-53.1117357784469,
-53.101353788696,-53.0209382070492,-52.9405376835194,-52.8566731261951,
-52.7762750836525,-52.6958762183537,-52.6154614439767,-52.6050794542222,
-52.5246638725751,-52.4442633490453,-52.3603987917211,-52.2800007491782,
-52.199601883879,-52.1191871095019,-52.1088051197484,-52.0283895381012,
-51.9479890145712,-51.864124457247,-51.7837264147041,-51.7033275494047,
-51.6229127750274,-51.6125307852746,-51.5321152036277,-51.451714680098,
-51.3678501227737,-51.2874520802311,-51.2070532149321,-51.1266384405552,
-51.1162564508009,-51.0358408691537,-50.9554403456238,-50.8715757882996,
-50.7911777457567,-50.7107788804575,-50.6303641060803,-50.6199821163271,
-50.53956653468,-50.45916601115,-50.3753014538258,-50.294903411283,-50.2145045459838,
-50.1340897716066,-50.1237077818533,-50.0432922002063,-49.9628916766764,
-49.8790271193522,-49.7986290768094,-49.7182302115103,-49.6378154371333,
-49.6274334473795,-49.5470178657324,-49.4666173422025,-49.3827527848783,
-49.3023547423355,-49.2219558770364,-49.1415411026592,-49.1311591129057,
-49.0507435312586,-48.9703430077288,-48.8864784504046,-48.8060804078618,
-48.7256815425627,-48.6452667681856,-48.6348847784319,-48.5544697200655,
-48.4740699157614,-48.3936710920797,-48.3132774925887,-48.232871672302,
-48.1911042754973),.UNSPECIFIED.);
#2935=B_SPLINE_CURVE_WITH_KNOTS('',3,(#22365,#22366,#22367,#22368,#22369,
#22370,#22371,#22372,#22373,#22374,#22375,#22376,#22377,#22378,#22379,#22380,
#22381,#22382,#22383,#22384,#22385,#22386,#22387,#22388,#22389,#22390,#22391,
#22392,#22393,#22394,#22395,#22396,#22397,#22398,#22399,#22400,#22401,#22402,
#22403,#22404,#22405,#22406,#22407,#22408,#22409,#22410,#22411,#22412,#22413,
#22414,#22415,#22416,#22417,#22418,#22419,#22420,#22421,#22422,#22423,#22424,
#22425,#22426,#22427,#22428,#22429,#22430,#22431,#22432,#22433,#22434,#22435,
#22436,#22437,#22438,#22439,#22440,#22441,#22442,#22443,#22444,#22445,#22446,
#22447,#22448,#22449,#22450,#22451,#22452,#22453,#22454,#22455,#22456,#22457,
#22458,#22459,#22460,#22461,#22462,#22463,#22464,#22465,#22466,#22467,#22468,
#22469,#22470,#22471,#22472,#22473,#22474,#22475,#22476,#22477,#22478,#22479,
#22480,#22481,#22482,#22483,#22484,#22485,#22486,#22487,#22488,#22489,#22490,
#22491,#22492,#22493,#22494,#22495,#22496,#22497,#22498,#22499,#22500,#22501,
#22502,#22503,#22504,#22505,#22506,#22507,#22508,#22509,#22510,#22511,#22512,
#22513,#22514,#22515,#22516,#22517,#22518,#22519,#22520,#22521,#22522,#22523,
#22524,#22525,#22526,#22527,#22528,#22529,#22530,#22531,#22532,#22533,#22534,
#22535,#22536,#22537,#22538,#22539,#22540,#22541,#22542,#22543,#22544,#22545,
#22546,#22547,#22548,#22549,#22550,#22551,#22552,#22553,#22554,#22555,#22556,
#22557,#22558,#22559,#22560,#22561,#22562,#22563,#22564,#22565,#22566,#22567,
#22568,#22569,#22570,#22571,#22572,#22573,#22574,#22575,#22576,#22577,#22578,
#22579,#22580,#22581,#22582,#22583,#22584,#22585,#22586,#22587,#22588,#22589,
#22590,#22591,#22592,#22593,#22594,#22595,#22596,#22597,#22598,#22599,#22600,
#22601,#22602,#22603,#22604,#22605,#22606,#22607,#22608,#22609,#22610,#22611,
#22612,#22613,#22614,#22615,#22616,#22617),.UNSPECIFIED.,.F.,.F.,(4,3,3,
3,3,3,3,3,3,3,3,3,3,3,3,3,3,3,3,3,3,3,3,3,3,3,3,3,3,3,3,3,3,3,3,3,3,3,3,
3,3,3,3,3,3,3,3,3,3,3,3,3,3,3,3,3,3,3,3,3,3,3,3,3,3,3,3,3,3,3,3,3,3,3,3,
3,3,3,3,3,3,3,3,3,4),(45.647142400955,45.6572387715891,45.7376543532363,
45.8180548767661,45.9019194340903,45.9823174766332,46.0627163419325,46.1431311163099,
46.1535131060629,46.2339286877099,46.3143292112395,46.3981937685638,46.4785918111067,
46.5589906764063,46.6394054507831,46.6497874405367,46.7302030221839,46.8106035457137,
46.8944681030379,46.9748661455806,47.0552650108795,47.135679785257,47.1460617750105,
47.2264773566577,47.3068778801874,47.3907424375117,47.4711404800545,47.5515393453538,
47.6319541197311,47.6423361094843,47.7227516911314,47.8031522146613,47.8870167719855,
47.9674148145283,48.0478136798277,48.1282284542052,48.1386104439581,48.2190260256053,
48.2994265491352,48.3832911064594,48.4636891490023,48.5440880143019,48.6245027886792,
48.6348847784319,48.7153003600789,48.7957008836091,48.8795654409332,48.959963483476,
49.0403623487745,49.1207771231514,49.1311591129057,49.2115746945528,49.2919752180826,
49.3758397754068,49.4562378179496,49.5366366832484,49.6170514576258,49.6274334473795,
49.7078490290264,49.7882495525564,49.8721141098806,49.9525121524234,50.0329110177216,
50.113325792099,50.1237077818533,50.2041233635004,50.2845238870303,50.3683884443545,
50.4487864868975,50.5291853521968,50.6096001265737,50.6199821163271,50.7003976979744,
50.7807982215041,50.8646627788283,50.9450608213712,51.0254596866705,51.1058744610481,
51.1162564508009,51.1964454262238,51.2766186167369,51.3567929105404,51.4369628388392,
51.5171506432341,51.5745921433062),.UNSPECIFIED.);
#2936=B_SPLINE_CURVE_WITH_KNOTS('',3,(#22618,#22619,#22620,#22621,#22622),
 .UNSPECIFIED.,.F.,.F.,(4,1,4),(51.5745921485727,51.6125307852747,51.9303121562591),
 .UNSPECIFIED.);
#2937=B_SPLINE_CURVE_WITH_KNOTS('',3,(#22624,#22625,#22626,#22627,#22628,
#22629,#22630,#22631,#22632,#22633,#22634,#22635,#22636,#22637,#22638,#22639),
 .UNSPECIFIED.,.F.,.F.,(4,3,3,3,3,4),(-48.1911042754973,-48.1386104439581,
-48.0579420042558,-47.9772908992282,-47.8966451486634,-47.8353526044678),
 .UNSPECIFIED.);
#2938=B_SPLINE_CURVE_WITH_KNOTS('',3,(#22640,#22641,#22642,#22643,#22644,
#22645,#22646,#22647,#22648,#22649,#22650,#22651,#22652,#22653,#22654,#22655),
 .UNSPECIFIED.,.F.,.F.,(4,1,1,1,1,1,1,1,1,1,1,1,1,4),(-47.8353525749775,
-47.6423361094843,-47.1460617750105,-46.6497874405367,-46.1535131060629,
-45.6572387715891,-45.1609644371153,-44.6646901026415,-44.1684157681677,
-43.6721414336939,-43.1758670992201,-42.6795927647463,-42.1833184302725,
-41.9079142575377),.UNSPECIFIED.);
#2939=B_SPLINE_CURVE_WITH_KNOTS('',3,(#22661,#22662,#22663,#22664,#22665,
#22666,#22667,#22668,#22669,#22670,#22671,#22672,#22673,#22674,#22675,#22676,
#22677,#22678,#22679,#22680,#22681,#22682,#22683,#22684,#22685,#22686,#22687,
#22688,#22689,#22690,#22691,#22692,#22693,#22694,#22695,#22696,#22697,#22698,
#22699,#22700,#22701,#22702,#22703,#22704,#22705,#22706,#22707,#22708,#22709,
#22710,#22711,#22712,#22713,#22714,#22715,#22716,#22717,#22718,#22719,#22720,
#22721,#22722,#22723,#22724,#22725,#22726,#22727,#22728,#22729,#22730,#22731,
#22732,#22733,#22734,#22735,#22736,#22737,#22738,#22739,#22740,#22741,#22742,
#22743,#22744,#22745,#22746,#22747,#22748,#22749,#22750,#22751,#22752,#22753,
#22754,#22755,#22756,#22757,#22758,#22759,#22760,#22761,#22762,#22763,#22764,
#22765,#22766,#22767,#22768,#22769,#22770,#22771,#22772,#22773,#22774,#22775,
#22776,#22777,#22778,#22779,#22780,#22781,#22782,#22783,#22784,#22785,#22786,
#22787,#22788,#22789,#22790,#22791,#22792,#22793,#22794,#22795,#22796),
 .UNSPECIFIED.,.F.,.F.,(4,2,2,2,2,2,2,2,2,2,2,2,2,2,2,2,2,2,2,2,2,2,2,2,
2,2,2,2,2,2,2,2,2,2,2,2,2,2,2,2,2,2,2,2,2,2,2,2,2,2,2,2,2,2,2,2,2,2,2,2,
2,2,2,2,2,2,2,4),(-4.16125843062839,-4.1108086605335,-4.05416447052261,
-3.98749224892683,-3.93335266536444,-3.90089760007793,-3.81396261840104,
-3.75034504100606,-3.68650609084296,-3.60473171151153,-3.57003366441495,
-3.50441512059131,-3.41364754281864,-3.35686392893218,-3.28964848409738,
-3.23537623700149,-3.20235008820308,-3.17963213204777,-3.05593950076319,
-2.99418126756799,-2.95018762802497,-2.88372166014699,-2.84839584138017,
-2.79557554860951,-2.71865311166099,-2.66243250284885,-2.59742866299811,
-2.53793459965514,-2.50453156308288,-2.48112530574869,-2.36122344306523,
-2.30092403435905,-2.21995596297141,-2.18052956626483,-2.13434766972314,
-2.01080383157267,-1.94908345957558,-1.83812709929393,-1.80245275651468,
-1.74842312898728,-1.67350706895093,-1.6173100370115,-1.55240221556747,
-1.49258544298174,-1.45911175717965,-1.43557908690942,-1.31490300923238,
-1.25386188550675,-1.16989048405493,-1.13360923308017,-1.08140683606103,
-0.96871936538971,-0.909129093310782,-0.831008023402229,-0.791565263964351,
-0.75438182047145,-0.695006080529864,-0.621258347948833,-0.56218228778284,
-0.486096455137806,-0.442681649268167,-0.404944314135633,-0.343370842314088,
-0.277218096883528,-0.225297486579145,-0.119533728146101,-0.0878835127706171,
-0.000106117481471679),.UNSPECIFIED.);
#2940=B_SPLINE_CURVE_WITH_KNOTS('',3,(#22797,#22798,#22799,#22800,#22801,
#22802,#22803,#22804,#22805,#22806,#22807,#22808,#22809,#22810,#22811,#22812),
 .UNSPECIFIED.,.F.,.F.,(4,3,3,3,3,4),(45.2914068413931,45.3715871243321,
45.4517702421806,45.5319511477599,45.6121488851322,45.647142400955),
 .UNSPECIFIED.);
#2941=B_SPLINE_CURVE_WITH_KNOTS('',3,(#22814,#22815,#22816,#22817,#22818),
 .UNSPECIFIED.,.F.,.F.,(4,1,4),(-41.9079142575377,-41.6870440957988,-41.5521673127012),
 .UNSPECIFIED.);
#2942=B_SPLINE_CURVE_WITH_KNOTS('',3,(#22819,#22820,#22821,#22822,#22823,
#22824,#22825,#22826,#22827,#22828,#22829,#22830,#22831,#22832,#22833,#22834,
#22835,#22836,#22837,#22838,#22839,#22840,#22841,#22842,#22843,#22844,#22845,
#22846,#22847,#22848,#22849,#22850,#22851,#22852,#22853,#22854,#22855,#22856,
#22857,#22858,#22859,#22860,#22861,#22862,#22863,#22864,#22865,#22866,#22867,
#22868,#22869,#22870,#22871,#22872,#22873,#22874,#22875,#22876,#22877,#22878,
#22879,#22880,#22881,#22882,#22883,#22884,#22885,#22886,#22887,#22888,#22889,
#22890,#22891,#22892,#22893,#22894,#22895,#22896,#22897,#22898,#22899,#22900,
#22901,#22902,#22903,#22904,#22905,#22906,#22907,#22908,#22909,#22910,#22911,
#22912,#22913,#22914,#22915,#22916,#22917,#22918,#22919,#22920,#22921,#22922,
#22923,#22924,#22925,#22926,#22927,#22928,#22929,#22930,#22931,#22932,#22933,
#22934,#22935,#22936,#22937,#22938,#22939,#22940,#22941,#22942,#22943,#22944,
#22945,#22946,#22947,#22948,#22949,#22950,#22951,#22952,#22953,#22954,#22955,
#22956,#22957,#22958,#22959,#22960,#22961,#22962,#22963,#22964,#22965,#22966,
#22967,#22968,#22969,#22970,#22971,#22972,#22973,#22974,#22975,#22976,#22977,
#22978,#22979,#22980,#22981,#22982,#22983,#22984,#22985,#22986,#22987,#22988,
#22989,#22990,#22991,#22992,#22993,#22994,#22995,#22996,#22997,#22998,#22999,
#23000,#23001,#23002,#23003,#23004,#23005,#23006,#23007,#23008,#23009,#23010,
#23011,#23012,#23013,#23014,#23015,#23016,#23017,#23018,#23019,#23020,#23021,
#23022,#23023,#23024,#23025,#23026,#23027,#23028,#23029,#23030,#23031,#23032,
#23033,#23034,#23035,#23036,#23037,#23038,#23039,#23040,#23041,#23042,#23043,
#23044,#23045,#23046,#23047,#23048,#23049,#23050,#23051,#23052,#23053,#23054,
#23055,#23056,#23057,#23058,#23059,#23060,#23061,#23062,#23063,#23064,#23065,
#23066,#23067,#23068,#23069,#23070,#23071),.UNSPECIFIED.,.F.,.F.,(4,3,3,
3,3,3,3,3,3,3,3,3,3,3,3,3,3,3,3,3,3,3,3,3,3,3,3,3,3,3,3,3,3,3,3,3,3,3,3,
3,3,3,3,3,3,3,3,3,3,3,3,3,3,3,3,3,3,3,3,3,3,3,3,3,3,3,3,3,3,3,3,3,3,3,3,
3,3,3,3,3,3,3,3,3,4),(-41.5521672972882,-41.4719671688436,-41.3917628968607,
-41.3115604309128,-41.2313396225703,-41.190769761325,-41.1103541796779,
-41.0299536561481,-40.9460890988238,-40.865691056281,-40.7852921909818,
-40.7048774166049,-40.6944954268512,-40.6140798452041,-40.533679321674,
-40.4498147643498,-40.369416721807,-40.2890178565077,-40.2086030821303,
-40.1982210923774,-40.1178055107303,-40.0374049872004,-39.9535404298762,
-39.8731423873333,-39.7927435220346,-39.7123287476571,-39.7019467579036,
-39.6215311762567,-39.5411306527269,-39.4572660954026,-39.3768680528599,
-39.2964691875608,-39.2160544131837,-39.2056724234298,-39.1252568417827,
-39.0448563182525,-38.9609917609284,-38.8805937183855,-38.8001948530866,
-38.7197800787096,-38.709398088956,-38.6289825073088,-38.5485819837791,
-38.4647174264549,-38.3843193839121,-38.3039205186132,-38.2235057442359,
-38.2131237544822,-38.1327081728352,-38.0523076493057,-37.9684430919814,
-37.8880450494384,-37.8076461841394,-37.7272314097624,-37.7168494200084,
-37.6364338383614,-37.5560333148318,-37.4721687575075,-37.3917707149647,
-37.311371849666,-37.2309570752894,-37.2205750855346,-37.1401595038874,
-37.0597589803572,-36.9758944230331,-36.8954963804905,-36.815097515191,
-36.7346827408139,-36.7243007510608,-36.6438851694137,-36.5634846458835,
-36.4796200885594,-36.3992220460168,-36.3188231807168,-36.2384084063399,
-36.228026416587,-36.1476108349403,-36.0672103114103,-35.983345754086,-35.9029477115432,
-35.8225488462444,-35.7421340718673,-35.7317520821132,-35.6515438818655,
-35.6247062080056),.UNSPECIFIED.);
#2943=B_SPLINE_CURVE_WITH_KNOTS('',3,(#23076,#23077,#23078,#23079,#23080,
#23081,#23082,#23083,#23084,#23085,#23086,#23087,#23088,#23089,#23090,#23091,
#23092,#23093,#23094,#23095,#23096,#23097,#23098,#23099,#23100,#23101,#23102,
#23103,#23104,#23105,#23106,#23107,#23108,#23109,#23110,#23111,#23112,#23113,
#23114,#23115,#23116,#23117,#23118,#23119,#23120,#23121,#23122,#23123,#23124,
#23125,#23126,#23127,#23128,#23129,#23130,#23131,#23132,#23133,#23134,#23135,
#23136,#23137,#23138,#23139,#23140,#23141,#23142,#23143,#23144,#23145,#23146,
#23147,#23148,#23149,#23150,#23151,#23152,#23153,#23154,#23155,#23156,#23157,
#23158,#23159,#23160,#23161,#23162,#23163,#23164,#23165,#23166,#23167,#23168,
#23169,#23170,#23171,#23172,#23173,#23174,#23175,#23176,#23177,#23178,#23179,
#23180,#23181,#23182,#23183,#23184,#23185,#23186,#23187,#23188,#23189,#23190,
#23191,#23192,#23193,#23194,#23195,#23196,#23197,#23198,#23199,#23200,#23201,
#23202,#23203,#23204,#23205,#23206,#23207,#23208,#23209,#23210,#23211,#23212,
#23213,#23214,#23215,#23216,#23217,#23218,#23219,#23220,#23221,#23222,#23223,
#23224,#23225,#23226,#23227),.UNSPECIFIED.,.F.,.F.,(4,2,2,2,2,2,2,2,2,2,
2,2,2,2,2,2,2,2,2,2,2,2,2,2,2,2,2,2,2,2,2,2,2,2,2,2,2,2,2,2,2,2,2,2,2,2,
2,2,2,2,2,2,2,2,2,2,2,2,2,2,2,2,2,2,2,2,2,2,2,2,2,2,2,2,2,4),(-8.57214567350776,
-8.5266526945173,-8.47967990369863,-8.45352593416885,-8.41269080105662,
-8.32357750766793,-8.26675918760088,-8.17541753599182,-8.11128974902864,
-8.07734762921564,-7.99492171986943,-7.93051510561155,-7.867438884642,-7.78085350584145,
-7.74794241748207,-7.68271771847744,-7.62071885661382,-7.59482270420592,
-7.53820554178689,-7.41727315483455,-7.38527882315083,-7.30251478290774,
-7.23574075296484,-7.17329952166471,-7.08490414212474,-7.05168861272035,
-6.99309313453794,-6.92780991550629,-6.87151711115175,-6.79163488564728,
-6.74049863515228,-6.70565835006123,-6.65581906752867,-6.58489709551557,
-6.52715000382637,-6.41197745733838,-6.38859477706288,-6.35520388857515,
-6.29576392880009,-6.23073825351169,-6.17451102941036,-6.09734748834294,
-6.0446691883285,-6.00938343143802,-5.96661625394913,-5.89148028632875,
-5.8326462101903,-5.75898501190176,-5.69985734716562,-5.66274231957707,
-5.6232229887053,-5.54517646139644,-5.48560457797253,-5.37305407574671,
-5.32076994023303,-5.28450800708924,-5.20050925348284,-5.13946077987214,
-5.01875985988877,-4.99523565647675,-4.96176632701582,-4.90196426199717,
-4.83704884082245,-4.7808499002071,-4.70579620245074,-4.65185471080323,
-4.61620534622512,-4.56149675036933,-4.49267357885504,-4.46599248140042,
-4.41096987361156,-4.38049219746669,-4.29791625040967,-4.2646669972504,
-4.19899215883652,-4.16125843062839),.UNSPECIFIED.);
#2944=B_SPLINE_CURVE_WITH_KNOTS('',3,(#23229,#23230,#23231,#23232,#23233,
#23234,#23235,#23236,#23237,#23238,#23239,#23240,#23241,#23242,#23243,#23244),
 .UNSPECIFIED.,.F.,.F.,(4,3,3,3,3,4),(-35.6247062080056,-35.5445172087638,
-35.4643253594168,-35.3841357287812,-35.3039293308426,-35.2689819950581),
 .UNSPECIFIED.);
#2945=B_SPLINE_CURVE_WITH_KNOTS('',3,(#23245,#23246,#23247,#23248,#23249,
#23250,#23251,#23252,#23253,#23254,#23255,#23256,#23257,#23258,#23259,#23260),
 .UNSPECIFIED.,.F.,.F.,(4,1,1,1,1,1,1,1,1,1,1,1,1,4),(-35.2689819901086,
-35.2354777476394,-34.7392034131656,-34.2429290786918,-33.746654744218,
-33.2503804097442,-32.7541060752704,-32.2578317407966,-31.7615574063229,
-31.2652830718491,-30.7690087373753,-30.2727344029015,-29.7764600684277,
-29.3415541759224),.UNSPECIFIED.);
#2946=B_SPLINE_CURVE_WITH_KNOTS('',3,(#23266,#23267,#23268,#23269,#23270,
#23271,#23272,#23273,#23274,#23275,#23276,#23277,#23278,#23279,#23280,#23281,
#23282,#23283,#23284,#23285,#23286,#23287,#23288,#23289,#23290,#23291,#23292,
#23293,#23294,#23295,#23296,#23297,#23298,#23299,#23300,#23301,#23302,#23303,
#23304,#23305,#23306,#23307,#23308,#23309,#23310,#23311,#23312,#23313,#23314,
#23315,#23316,#23317,#23318,#23319,#23320,#23321,#23322,#23323,#23324,#23325,
#23326,#23327,#23328,#23329,#23330,#23331,#23332,#23333,#23334,#23335,#23336,
#23337,#23338,#23339,#23340,#23341,#23342,#23343,#23344,#23345,#23346,#23347,
#23348,#23349,#23350,#23351,#23352,#23353,#23354,#23355,#23356,#23357,#23358,
#23359,#23360,#23361,#23362,#23363,#23364,#23365,#23366,#23367,#23368,#23369,
#23370,#23371,#23372,#23373,#23374,#23375,#23376,#23377,#23378,#23379,#23380,
#23381,#23382,#23383,#23384,#23385,#23386,#23387,#23388,#23389,#23390,#23391,
#23392,#23393,#23394,#23395,#23396,#23397,#23398,#23399,#23400,#23401,#23402,
#23403,#23404,#23405,#23406,#23407,#23408,#23409,#23410,#23411,#23412,#23413,
#23414,#23415,#23416,#23417,#23418,#23419,#23420,#23421,#23422,#23423,#23424,
#23425,#23426,#23427,#23428,#23429,#23430,#23431,#23432,#23433,#23434,#23435,
#23436,#23437,#23438,#23439,#23440,#23441,#23442,#23443,#23444,#23445,#23446,
#23447,#23448,#23449,#23450,#23451,#23452,#23453,#23454,#23455,#23456,#23457,
#23458,#23459,#23460,#23461,#23462,#23463,#23464,#23465,#23466,#23467,#23468,
#23469,#23470,#23471,#23472,#23473,#23474,#23475,#23476,#23477,#23478,#23479,
#23480,#23481,#23482,#23483,#23484,#23485,#23486,#23487,#23488,#23489,#23490,
#23491,#23492,#23493,#23494,#23495,#23496,#23497,#23498,#23499,#23500,#23501,
#23502,#23503,#23504,#23505,#23506,#23507,#23508,#23509,#23510,#23511,#23512,
#23513,#23514,#23515,#23516,#23517,#23518),.UNSPECIFIED.,.F.,.F.,(4,3,3,
3,3,3,3,3,3,3,3,3,3,3,3,3,3,3,3,3,3,3,3,3,3,3,3,3,3,3,3,3,3,3,3,3,3,3,3,
3,3,3,3,3,3,3,3,3,3,3,3,3,3,3,3,3,3,3,3,3,3,3,3,3,3,3,3,3,3,3,3,3,3,3,3,
3,3,3,3,3,3,3,3,3,4),(26.7975893262247,26.7988140615849,26.8792296432319,
26.9596301667617,27.043494724086,27.1238927666289,27.2042916319276,27.2847064063046,
27.2950883960587,27.3755039777059,27.4559045012358,27.53976905856,27.6201671011028,
27.700565966402,27.7809807407789,27.7913627305325,27.8717783121796,27.9521788357092,
28.0360433930335,28.1164414355764,28.1968403008755,28.2772550752525,28.2876370650063,
28.3680526466533,28.448453170183,28.5323177275073,28.61271577005,28.6931146353489,
28.7735294097261,28.7839113994801,28.8643269811273,28.9447275046572,29.0285920619814,
29.1089901045244,29.1893889698233,29.2698037442009,29.2801857339539,29.360601315601,
29.4410018391309,29.5248663964551,29.6052644389978,29.6856633042968,29.7660780786739,
29.7764600684277,29.8568756500748,29.9372761736052,30.0211407309293,30.1015387734722,
30.1819376387715,30.262352413149,30.2727344029015,30.3531499845486,30.4335505080785,
30.5174150654027,30.5978131079454,30.6782119732445,30.7586267476212,30.7690087373753,
30.8494243190225,30.929824842553,31.013689399877,31.0940874424199,31.1744863077184,
31.2549010820954,31.2652830718491,31.3456986534964,31.4260991770262,31.5099637343504,
31.5903617768931,31.6707606421923,31.7511754165694,31.7615574063229,31.8419729879701,
31.9223735115007,32.0062380688247,32.0866361113677,32.1670349766674,32.2474497510447,
32.2578317407967,32.3380614960746,32.4182755973972,32.4984913520439,32.5787024990809,
32.6589326269847,32.72503622265),.UNSPECIFIED.);
#2947=B_SPLINE_CURVE_WITH_KNOTS('',3,(#23519,#23520,#23521,#23522,#23523,
#23524,#23525,#23526,#23527,#23528,#23529,#23530),.UNSPECIFIED.,.F.,.F.,
(4,2,2,2,2,4),(-8.82186319664549,-8.79141945747857,-8.74049362082466,-8.66687908944385,
-8.61461409729926,-8.57214567350776),.UNSPECIFIED.);
#2948=B_SPLINE_CURVE_WITH_KNOTS('',3,(#23532,#23533,#23534,#23535,#23536),
 .UNSPECIFIED.,.F.,.F.,(4,1,4),(-29.3415541759224,-29.2801857339539,-28.985796682929),
 .UNSPECIFIED.);
#2949=B_SPLINE_CURVE_WITH_KNOTS('',3,(#23537,#23538,#23539,#23540,#23541,
#23542,#23543,#23544,#23545,#23546,#23547,#23548,#23549,#23550,#23551,#23552,
#23553,#23554,#23555,#23556,#23557,#23558,#23559,#23560,#23561,#23562,#23563,
#23564,#23565,#23566,#23567,#23568,#23569,#23570,#23571,#23572,#23573,#23574,
#23575,#23576,#23577,#23578,#23579,#23580,#23581,#23582,#23583,#23584,#23585,
#23586,#23587,#23588,#23589,#23590,#23591,#23592,#23593,#23594,#23595,#23596,
#23597,#23598,#23599,#23600,#23601,#23602,#23603,#23604,#23605,#23606,#23607,
#23608,#23609,#23610,#23611,#23612,#23613,#23614,#23615,#23616,#23617,#23618,
#23619,#23620,#23621,#23622,#23623,#23624,#23625,#23626,#23627,#23628,#23629,
#23630,#23631,#23632,#23633,#23634,#23635,#23636,#23637,#23638,#23639,#23640,
#23641,#23642,#23643,#23644,#23645,#23646,#23647,#23648,#23649,#23650,#23651,
#23652,#23653,#23654,#23655,#23656,#23657,#23658,#23659,#23660,#23661,#23662,
#23663,#23664,#23665,#23666,#23667,#23668,#23669,#23670,#23671,#23672,#23673,
#23674),.UNSPECIFIED.,.F.,.F.,(4,2,2,2,2,2,2,2,2,2,2,2,2,2,2,2,2,2,2,2,
2,2,2,2,2,2,2,2,2,2,2,2,2,2,2,2,2,2,2,2,2,2,2,2,2,2,2,2,2,2,2,2,2,2,2,2,
2,2,2,2,2,2,2,2,2,2,2,2,4),(-8.82172059392306,-8.71505368676722,-8.68624371205641,
-8.65611514691957,-8.54557674370032,-8.49338883640374,-8.40158893096534,
-8.35665083111386,-8.32980663957806,-8.28691118496182,-8.21003328989268,
-8.15075738237388,-8.07570115263926,-8.01696196782507,-7.97995546412746,
-7.94025100202579,-7.86237138033921,-7.80284299793858,-7.73325471975515,
-7.6705356287488,-7.63244458781466,-7.58491672932839,-7.51108418160777,
-7.45258680549647,-7.37981951316885,-7.32053733326194,-7.28338074337444,
-7.2439083516446,-7.16581840375805,-7.10623786727216,-6.99361175932215,
-6.94138128277694,-6.90510911230878,-6.82112971419231,-6.76008840114547,
-6.63941157246137,-6.61588393384177,-6.58241383775098,-6.52780156363633,
-6.46035964173157,-6.40351868950041,-6.31168471996753,-6.24706609050832,
-6.2124428079742,-6.12588788695974,-6.06419368677298,-5.94075834738571,
-5.89452728609497,-5.85512965052663,-5.77413146740684,-5.71382525966102,
-5.59389389757059,-5.57049885079202,-5.53710218161794,-5.47763050823255,
-5.41261884996788,-5.35639726446858,-5.28316424821052,-5.22801481061597,
-5.19202016590582,-5.08111441265303,-5.01923283027586,-4.9515521806941,
-4.86795926594443,-4.85351588792323,-4.81890838662932,-4.7323315443045,
-4.6706319387406,-4.660704216232),.UNSPECIFIED.);
#2950=B_SPLINE_CURVE_WITH_KNOTS('',3,(#23680,#23681,#23682,#23683,#23684,
#23685,#23686,#23687,#23688,#23689,#23690,#23691,#23692,#23693,#23694,#23695,
#23696,#23697,#23698,#23699,#23700,#23701,#23702,#23703,#23704,#23705,#23706,
#23707,#23708,#23709,#23710,#23711,#23712,#23713,#23714,#23715,#23716,#23717,
#23718,#23719,#23720,#23721,#23722,#23723,#23724,#23725,#23726,#23727,#23728,
#23729,#23730,#23731,#23732,#23733,#23734,#23735,#23736,#23737,#23738,#23739,
#23740,#23741,#23742,#23743,#23744,#23745,#23746,#23747,#23748,#23749,#23750,
#23751,#23752,#23753,#23754,#23755,#23756,#23757,#23758,#23759,#23760,#23761,
#23762,#23763,#23764,#23765,#23766,#23767,#23768,#23769,#23770,#23771,#23772,
#23773,#23774,#23775,#23776,#23777,#23778,#23779,#23780,#23781,#23782,#23783,
#23784,#23785,#23786,#23787,#23788,#23789,#23790,#23791,#23792,#23793,#23794,
#23795,#23796,#23797,#23798,#23799,#23800,#23801,#23802,#23803,#23804,#23805,
#23806,#23807,#23808,#23809,#23810,#23811),.UNSPECIFIED.,.F.,.F.,(4,2,2,
2,2,2,2,2,2,2,2,2,2,2,2,2,2,2,2,2,2,2,2,2,2,2,2,2,2,2,2,2,2,2,2,2,2,2,2,
2,2,2,2,2,2,2,2,2,2,2,2,2,2,2,2,2,2,2,2,2,2,2,2,2,2,4),(-4.16138304547812,
-4.10880352144696,-4.04805008561075,-3.96523095703559,-3.92757479253391,
-3.87734452415319,-3.7613557865919,-3.70123826662044,-3.62100074986933,
-3.58082982128405,-3.53586596392477,-3.40982075028046,-3.34742356816844,
-3.23988682517842,-3.20580322670447,-3.15728421195415,-3.07244360287468,
-3.01596606526195,-2.94994473558394,-2.89376227702972,-2.8609918600829,
-2.83875677645363,-2.713177381296,-2.65091225920373,-2.54277365518383,-2.50846622597842,
-2.4591702484774,-2.37584352543414,-2.31943100330132,-2.25366876917332,
-2.1966509079333,-2.16373525390199,-2.07714140578139,-2.01407762942821,
-1.94966166227699,-1.86723904862984,-1.83330977350635,-1.76858209765694,
-1.67797231069848,-1.62119634461225,-1.55401342392953,-1.49980315704946,
-1.4668438961061,-1.44425152277379,-1.32007145222321,-1.25818624235187,
-1.14729443100237,-1.11131094387604,-1.05620309810477,-0.982935406714329,
-0.926724669947922,-0.861764380026687,-0.802118393454944,-0.768681882116029,
-0.745216402820036,-0.624295447520146,-0.563199493245989,-0.479013994167103,
-0.442911235281126,-0.415516240580332,-0.362141659965845,-0.286147608388949,
-0.233496139249837,-0.125746681025646,-0.0941040473628391,-0.000106119371468615),
 .UNSPECIFIED.);
#2951=B_SPLINE_CURVE_WITH_KNOTS('',3,(#23812,#23813,#23814,#23815,#23816,
#23817,#23818,#23819,#23820,#23821,#23822,#23823,#23824,#23825,#23826,#23827),
 .UNSPECIFIED.,.F.,.F.,(4,3,3,3,3,4),(26.4418509198543,26.522072587646,
26.6022987878389,26.6825236672068,26.7627664191034,26.7975893262247),
 .UNSPECIFIED.);
#2952=B_SPLINE_CURVE_WITH_KNOTS('',3,(#23828,#23829,#23830,#23831,#23832,
#23833,#23834,#23835,#23836,#23837,#23838,#23839,#23840,#23841,#23842,#23843,
#23844,#23845,#23846,#23847,#23848,#23849,#23850,#23851,#23852,#23853,#23854,
#23855,#23856,#23857,#23858,#23859,#23860,#23861,#23862,#23863,#23864,#23865,
#23866,#23867,#23868,#23869,#23870,#23871,#23872,#23873,#23874,#23875,#23876,
#23877,#23878,#23879,#23880,#23881,#23882,#23883,#23884,#23885,#23886,#23887,
#23888,#23889,#23890,#23891,#23892,#23893,#23894,#23895,#23896,#23897,#23898,
#23899,#23900,#23901,#23902,#23903,#23904,#23905,#23906,#23907,#23908,#23909,
#23910,#23911,#23912,#23913,#23914,#23915,#23916,#23917,#23918,#23919,#23920,
#23921,#23922,#23923,#23924,#23925,#23926,#23927,#23928,#23929,#23930,#23931,
#23932,#23933,#23934,#23935,#23936,#23937,#23938,#23939,#23940,#23941,#23942,
#23943,#23944,#23945,#23946,#23947,#23948,#23949,#23950,#23951,#23952,#23953,
#23954,#23955,#23956,#23957,#23958,#23959,#23960,#23961,#23962,#23963,#23964,
#23965,#23966,#23967,#23968,#23969,#23970,#23971,#23972,#23973,#23974,#23975),
 .UNSPECIFIED.,.F.,.F.,(4,2,2,2,2,2,2,2,2,2,2,2,2,2,2,2,2,2,2,2,2,2,2,2,
2,2,2,2,2,2,2,2,2,2,2,2,2,2,2,2,2,2,2,2,2,2,2,2,2,2,2,2,2,2,2,2,2,2,2,2,
2,2,2,2,2,2,2,2,2,2,2,2,2,4),(-4.660704216232,-4.54717480836569,-4.52439802262577,
-4.49134032769968,-4.41095770906608,-4.33846805041116,-4.28202925163412,
-4.21615621482939,-4.15950699887394,-4.12665741613199,-4.08257226621711,
-3.98859124966383,-3.931639734452,-3.8637717708191,-3.8088144078729,-3.77453866438938,
-3.72535087666706,-3.64181968159527,-3.58539993883686,-3.51960524249073,
-3.46269887573972,-3.42980362476136,-3.38554825092803,-3.29191886988205,
-3.23498348594814,-3.16718122252458,-3.11225612445079,-3.07810177585851,
-3.02933756822755,-2.94497659794237,-2.88851973318813,-2.82258247217076,
-2.76612709165884,-2.73330995681478,-2.66158730669186,-2.59494606351099,
-2.53791946566919,-2.46976809087832,-2.41473488817004,-2.37996583558301,
-2.32907305363151,-2.24874533318724,-2.1924410454408,-2.12710903943484,
-2.06868969505259,-2.0355088158653,-1.9472743563323,-1.88471530185778,-1.8181228971323,
-1.73537908631784,-1.70329384084289,-1.58051101535088,-1.52975767095848,
-1.44746322211503,-1.3730957337222,-1.34052211829442,-1.25387596864685,
-1.19030967730142,-1.12641693492717,-1.04155617290932,-1.00816851100997,
-0.875070668338063,-0.820273992003613,-0.793332950341518,-0.722356942616175,
-0.67273142763783,-0.637974179999183,-0.587120874394874,-0.506724252010099,
-0.453316858963204,-0.390466277726096,-0.328215731381091,-0.296710621679306,
-0.249923280266006),.UNSPECIFIED.);
#2953=B_SPLINE_CURVE_WITH_KNOTS('',3,(#23980,#23981,#23982,#23983,#23984,
#23985,#23986,#23987,#23988,#23989,#23990,#23991,#23992,#23993,#23994,#23995,
#23996,#23997,#23998,#23999,#24000,#24001,#24002,#24003,#24004,#24005,#24006,
#24007,#24008,#24009,#24010,#24011,#24012,#24013,#24014,#24015,#24016,#24017,
#24018,#24019,#24020,#24021,#24022,#24023,#24024,#24025,#24026,#24027,#24028,
#24029,#24030,#24031,#24032,#24033,#24034,#24035,#24036,#24037,#24038,#24039,
#24040,#24041,#24042,#24043,#24044,#24045,#24046,#24047,#24048,#24049,#24050,
#24051,#24052,#24053,#24054,#24055,#24056,#24057,#24058,#24059,#24060,#24061,
#24062,#24063,#24064,#24065,#24066,#24067,#24068,#24069,#24070,#24071,#24072,
#24073,#24074,#24075,#24076,#24077,#24078,#24079,#24080,#24081,#24082,#24083,
#24084,#24085,#24086,#24087,#24088,#24089,#24090,#24091,#24092,#24093,#24094,
#24095,#24096,#24097,#24098,#24099,#24100,#24101,#24102,#24103,#24104,#24105,
#24106,#24107,#24108,#24109,#24110,#24111,#24112,#24113,#24114,#24115,#24116,
#24117,#24118,#24119,#24120,#24121,#24122,#24123,#24124,#24125,#24126,#24127),
 .UNSPECIFIED.,.F.,.F.,(4,2,2,2,2,2,2,2,2,2,2,2,2,2,2,2,2,2,2,2,2,2,2,2,
2,2,2,2,2,2,2,2,2,2,2,2,2,2,2,2,2,2,2,2,2,2,2,2,2,2,2,2,2,2,2,2,2,2,2,2,
2,2,2,2,2,2,2,2,2,2,2,2,2,4),(-8.57207326543173,-8.52540157720413,-8.48258196231714,
-8.45354508349237,-8.40816043619921,-8.32814767430087,-8.27172870728119,
-8.18823972312311,-8.13903307648575,-8.104751464036,-7.99668303756801,-7.93440105020989,
-7.80876681606068,-7.78654819712475,-7.75378653899148,-7.69977967941424,
-7.63269438177325,-7.57594519780263,-7.48580263904452,-7.42151370133059,
-7.38811004137267,-7.30325416509756,-7.23938405597625,-7.17580111269242,
-7.08904419035894,-7.05652048815099,-7.00189634746641,-6.9353791069696,
-6.8787756658092,-6.79136222217601,-6.72539664972693,-6.69233904816397,
-6.60740205800124,-6.54309020535531,-6.47865734322217,-6.39324180946986,
-6.37786536766714,-6.34521886813112,-6.26251897439032,-6.19636468789063,
-6.13350594686396,-6.04579945998549,-6.01266771602776,-5.95830159661692,
-5.89103040409763,-5.83423267327737,-5.74321587174528,-5.68184083926186,
-5.64992581521011,-5.56715567188756,-5.50022934259423,-5.43789336089576,
-5.34936433787834,-5.31612168526708,-5.26166689922114,-5.19433972773177,
-5.13752754186971,-5.04624537886821,-4.98104132260954,-4.94632315303402,
-4.86456245237656,-4.80073608887504,-4.73710628141658,-4.65010069051738,
-4.61767551275871,-4.55556568905253,-4.49267278742941,-4.46668244678827,
-4.41110587693669,-4.34647792101919,-4.28573190276621,-4.25204675379642,
-4.22813653827197,-4.16138304547812),.UNSPECIFIED.);
#2954=B_SPLINE_CURVE_WITH_KNOTS('',3,(#24129,#24130,#24131,#24132,#24133,
#24134,#24135,#24136),.UNSPECIFIED.,.F.,.F.,(4,2,2,4),(-0.249923280266006,
-0.171457320855668,-0.119217469302637,-0.000106124780310168),
 .UNSPECIFIED.);
#2955=B_SPLINE_CURVE_WITH_KNOTS('',3,(#24137,#24138,#24139,#24140,#24141,
#24142,#24143,#24144,#24145,#24146,#24147,#24148,#24149,#24150,#24151,#24152,
#24153,#24154,#24155,#24156,#24157,#24158,#24159,#24160,#24161,#24162,#24163,
#24164,#24165,#24166,#24167,#24168,#24169,#24170,#24171,#24172,#24173,#24174,
#24175,#24176,#24177,#24178,#24179,#24180,#24181,#24182,#24183,#24184,#24185,
#24186,#24187,#24188,#24189,#24190,#24191,#24192,#24193,#24194,#24195,#24196,
#24197,#24198,#24199,#24200,#24201,#24202,#24203,#24204,#24205,#24206,#24207,
#24208,#24209,#24210,#24211,#24212,#24213,#24214,#24215,#24216,#24217,#24218,
#24219,#24220,#24221,#24222,#24223,#24224,#24225,#24226,#24227,#24228,#24229,
#24230,#24231,#24232,#24233,#24234,#24235,#24236,#24237,#24238,#24239,#24240,
#24241,#24242,#24243,#24244,#24245,#24246,#24247,#24248,#24249,#24250,#24251,
#24252,#24253,#24254,#24255,#24256,#24257,#24258,#24259,#24260,#24261,#24262,
#24263,#24264,#24265,#24266,#24267,#24268,#24269,#24270,#24271,#24272,#24273,
#24274,#24275,#24276,#24277,#24278,#24279,#24280,#24281,#24282,#24283,#24284,
#24285,#24286,#24287,#24288,#24289,#24290,#24291,#24292,#24293,#24294,#24295,
#24296,#24297,#24298,#24299,#24300,#24301,#24302,#24303,#24304,#24305,#24306,
#24307,#24308,#24309,#24310,#24311,#24312,#24313,#24314,#24315,#24316,#24317,
#24318,#24319,#24320,#24321,#24322,#24323,#24324,#24325,#24326,#24327,#24328,
#24329,#24330,#24331,#24332,#24333,#24334,#24335,#24336,#24337,#24338,#24339,
#24340,#24341,#24342,#24343,#24344,#24345,#24346,#24347,#24348,#24349,#24350,
#24351,#24352,#24353,#24354,#24355,#24356,#24357,#24358,#24359,#24360,#24361,
#24362,#24363,#24364,#24365,#24366,#24367,#24368,#24369,#24370,#24371,#24372,
#24373,#24374,#24375,#24376,#24377,#24378,#24379,#24380,#24381,#24382,#24383,
#24384,#24385,#24386,#24387,#24388,#24389),.UNSPECIFIED.,.F.,.F.,(4,3,3,
3,3,3,3,3,3,3,3,3,3,3,3,3,3,3,3,3,3,3,3,3,3,3,3,3,3,3,3,3,3,3,3,3,3,3,3,
3,3,3,3,3,3,3,3,3,3,3,3,3,3,3,3,3,3,3,3,3,3,3,3,3,3,3,3,3,3,3,3,3,3,3,3,
3,3,3,3,3,3,3,3,3,4),(-16.4194260685698,-16.3770530376352,-16.2966374559875,
-16.2162369324569,-16.132372375133,-16.0519743325897,-15.9715754672898,
-15.8911606929121,-15.8807787031614,-15.8003631215144,-15.7199625979849,
-15.6360980406606,-15.555699998118,-15.4753011328189,-15.394886358442,-15.3845043686876,
-15.3040887870402,-15.2236882635099,-15.1398237061858,-15.0594256636427,
-14.9790267983431,-14.8986120239656,-14.8882300342138,-14.8078144525681,
-14.7274139290397,-14.6435493717148,-14.5631513291734,-14.4827524638757,
-14.4023376895001,-14.39195569974,-14.311540118089,-14.2311395945552,-14.147275037233,
-14.0668769946863,-13.9864781293833,-13.9060633550023,-13.8956813652663,
-13.8152657836274,-13.7348652601058,-13.6510007027774,-13.5706026602428,
-13.4902037949517,-13.4097890205825,-13.3994070307925,-13.3189914491325,
-13.2385909255897,-13.154726368272,-13.0743283257164,-12.9939294604045,
-12.913514686015,-12.9031326963187,-12.8227171146844,-12.7423165911674,
-12.6584520338368,-12.5780539913066,-12.4976551260199,-12.417240351655,
-12.4068583618449,-12.3264427802026,-12.2460422566776,-12.162177699351,
-12.0817796568132,-12.0013807915192,-11.9209660171472,-11.9105840273711,
-11.8301684456594,-11.7497679220645,-11.6659033647727,-11.585505322165,
-11.5051064568015,-11.4246916823607,-11.4143096928973,-11.3338941114529,
-11.2534935881266,-11.1696290307009,-11.0892309883605,-11.0088321232625,
-10.9284173490835,-10.9180353584235,-10.8376204161101,-10.7572207940968,
-10.676823409421,-10.5964311048214,-10.5160291436,-10.4919945899008),
 .UNSPECIFIED.);
#2956=B_SPLINE_CURVE_WITH_KNOTS('',3,(#24395,#24396,#24397,#24398,#24399),
 .UNSPECIFIED.,.F.,.F.,(4,1,4),(-4.20879728873375,-3.97019467579036,-3.85305545639561),
 .UNSPECIFIED.);
#2957=B_SPLINE_CURVE_WITH_KNOTS('',3,(#24401,#24402,#24403,#24404,#24405,
#24406,#24407,#24408,#24409,#24410,#24411,#24412,#24413,#24414,#24415,#24416,
#24417,#24418,#24419,#24420,#24421,#24422,#24423,#24424,#24425,#24426,#24427,
#24428,#24429,#24430,#24431,#24432,#24433,#24434,#24435,#24436,#24437,#24438,
#24439,#24440,#24441,#24442,#24443,#24444,#24445,#24446,#24447,#24448,#24449,
#24450,#24451,#24452,#24453,#24454,#24455,#24456,#24457,#24458,#24459,#24460,
#24461,#24462,#24463,#24464,#24465,#24466,#24467,#24468,#24469,#24470,#24471,
#24472,#24473,#24474,#24475,#24476,#24477,#24478,#24479,#24480,#24481,#24482,
#24483,#24484,#24485,#24486,#24487,#24488,#24489,#24490,#24491,#24492,#24493,
#24494,#24495,#24496,#24497,#24498,#24499,#24500,#24501,#24502,#24503,#24504,
#24505,#24506,#24507,#24508,#24509,#24510,#24511,#24512,#24513,#24514,#24515,
#24516,#24517,#24518,#24519,#24520,#24521,#24522,#24523,#24524,#24525,#24526,
#24527,#24528,#24529,#24530,#24531,#24532,#24533,#24534,#24535,#24536,#24537,
#24538,#24539,#24540,#24541,#24542,#24543,#24544,#24545,#24546,#24547,#24548,
#24549,#24550,#24551,#24552,#24553,#24554,#24555,#24556,#24557,#24558,#24559,
#24560),.UNSPECIFIED.,.F.,.F.,(4,3,3,3,3,3,3,3,3,3,3,3,3,3,3,3,3,3,3,3,
3,3,3,3,3,3,3,3,3,3,3,3,3,3,3,3,3,3,3,3,3,3,3,3,3,3,3,3,3,3,3,3,3,4),(-3.85305545421067,
-3.77291964238566,-3.69278153984504,-3.61264712623592,-3.53249330145913,
-3.47392034131656,-3.39350856937354,-3.31311185551211,-3.22924539334477,
-3.14885109862192,-3.06845594440698,-2.98804480902414,-2.97764600684277,
-2.89723194483455,-2.81683297413262,-2.73296764869171,-2.65257121471742,
-2.5721739704636,-2.4917608250185,-2.48137167236897,-2.40093647695799,-2.32051622613262,
-2.23666150407326,-2.15624377821962,-2.07582532646403,-1.99539121234268,
-1.98509733789518,-1.90474324759607,-1.82440447274427,-1.74050910541355,
-1.66017244479229,-1.57983458393119,-1.4994799427304,-1.48882300342138,
-1.40826740291856,-1.32772640753817,-1.24393197289052,-1.16339467572715,
-1.08285756497712,-1.00230674301718,-0.99254866894759,-0.912388322686476,
-0.832243389392974,-0.748251125663179,-0.668105491870725,-0.587956937046544,
-0.507788147193865,-0.496274334473794,-0.415365456522927,-0.334472363569503,
-0.250854272677127,-0.169974037999006,-0.0849870189995029,0.),
 .UNSPECIFIED.);
#2958=B_SPLINE_CURVE_WITH_KNOTS('',3,(#24563,#24564,#24565,#24566,#24567,
#24568,#24569,#24570,#24571,#24572,#24573,#24574,#24575,#24576,#24577,#24578,
#24579,#24580,#24581,#24582,#24583,#24584,#24585,#24586,#24587,#24588,#24589,
#24590,#24591,#24592,#24593,#24594,#24595,#24596,#24597,#24598,#24599,#24600,
#24601,#24602,#24603,#24604,#24605,#24606,#24607,#24608,#24609,#24610,#24611,
#24612,#24613,#24614,#24615,#24616,#24617,#24618,#24619,#24620,#24621,#24622,
#24623,#24624,#24625,#24626,#24627,#24628,#24629,#24630,#24631,#24632,#24633,
#24634,#24635,#24636,#24637,#24638,#24639,#24640,#24641,#24642,#24643,#24644,
#24645,#24646,#24647,#24648,#24649,#24650,#24651,#24652,#24653,#24654,#24655,
#24656,#24657,#24658,#24659,#24660,#24661,#24662,#24663,#24664,#24665,#24666,
#24667,#24668,#24669,#24670,#24671,#24672,#24673,#24674,#24675,#24676,#24677,
#24678,#24679,#24680,#24681,#24682,#24683,#24684,#24685,#24686,#24687,#24688,
#24689,#24690,#24691,#24692,#24693,#24694,#24695,#24696,#24697,#24698,#24699,
#24700),.UNSPECIFIED.,.F.,.F.,(4,2,2,2,2,2,2,2,2,2,2,2,2,2,2,2,2,2,2,2,
2,2,2,2,2,2,2,2,2,2,2,2,2,2,2,2,2,2,2,2,2,2,2,2,2,2,2,2,2,2,2,2,2,2,2,2,
2,2,2,2,2,2,2,2,2,2,2,2,4),(-8.32193337931491,-8.19665781353201,-8.1427529639967,
-8.02220072731463,-7.99255198247967,-7.94385232850661,-7.87303717104052,
-7.82270695671389,-7.69679462639956,-7.67463489572474,-7.6419389575693,
-7.58786118762996,-7.52072419252838,-7.46394288169517,-7.37415689321913,
-7.30823185140564,-7.27385373582285,-7.19183114545146,-7.12772906426362,
-7.06306346937112,-6.97762663172909,-6.94495075490186,-6.88928089675609,
-6.8230946558089,-6.76657808334903,-6.69760602277879,-6.63903708717948,
-6.60207759364124,-6.56362835461421,-6.48500962592191,-6.42528878653741,
-6.35583897708348,-6.2928149402416,-6.25464003254163,-6.20734561495133,
-6.13334845796692,-6.07480848589869,-6.01432373401582,-5.9465127727114,
-5.90709862009578,-5.86436758857633,-5.77267610384581,-5.74681023095454,
-5.69007100024129,-5.56944863910889,-5.53738516985327,-5.45463390315573,
-5.38799611725067,-5.32546887649081,-5.23719453118219,-5.20400494179616,
-5.14958925729567,-5.08228560596609,-5.02547738868342,-4.9343210120028,
-4.87303275504826,-4.84110725070179,-4.7583339931184,-4.69142205281254,
-4.62907103673601,-4.54055340354179,-4.50731238809251,-4.44858947671009,
-4.38334647012783,-4.32706453012634,-4.24752462083681,-4.19620040999603,
-4.16130608063852,-4.16130056038158),.UNSPECIFIED.);
#2959=B_SPLINE_CURVE_WITH_KNOTS('',3,(#24703,#24704,#24705,#24706,#24707,
#24708,#24709,#24710,#24711,#24712,#24713,#24714,#24715,#24716,#24717,#24718,
#24719,#24720,#24721,#24722,#24723,#24724,#24725,#24726,#24727,#24728,#24729,
#24730,#24731,#24732,#24733,#24734,#24735,#24736,#24737,#24738,#24739,#24740,
#24741,#24742,#24743,#24744,#24745,#24746,#24747,#24748,#24749,#24750,#24751,
#24752,#24753,#24754,#24755,#24756,#24757,#24758,#24759,#24760,#24761,#24762,
#24763,#24764,#24765,#24766,#24767,#24768,#24769,#24770,#24771,#24772,#24773,
#24774,#24775,#24776,#24777,#24778,#24779,#24780,#24781,#24782,#24783,#24784,
#24785,#24786,#24787,#24788,#24789,#24790,#24791,#24792,#24793,#24794,#24795,
#24796,#24797,#24798,#24799,#24800,#24801,#24802,#24803,#24804,#24805,#24806,
#24807,#24808,#24809,#24810,#24811,#24812,#24813,#24814,#24815,#24816,#24817,
#24818,#24819,#24820,#24821,#24822,#24823,#24824,#24825,#24826,#24827,#24828,
#24829,#24830,#24831,#24832,#24833,#24834),.UNSPECIFIED.,.F.,.F.,(4,2,2,
2,2,2,2,2,2,2,2,2,2,2,2,2,2,2,2,2,2,2,2,2,2,2,2,2,2,2,2,2,2,2,2,2,2,2,2,
2,2,2,2,2,2,2,2,2,2,2,2,2,2,2,2,2,2,2,2,2,2,2,2,2,2,4),(-4.16130056038158,
-4.14695393791753,-4.06352973478219,-3.99548150715283,-3.93379535980784,
-3.84727841182617,-3.81262648858228,-3.74894939215065,-3.65595505377096,
-3.59905127916525,-3.53137331181627,-3.47652887803669,-3.44260623387991,
-3.41827850791444,-3.30037702990747,-3.23990795474275,-3.15825244353961,
-3.11950337566717,-3.07200793984769,-2.95226383378267,-2.89199586497062,
-2.81115409710204,-2.77160112118748,-2.72564150774563,-2.60165031294345,
-2.5398150447074,-2.44638631193077,-2.41429831063311,-2.35007478735879,
-2.26329695406303,-2.20672615451093,-2.14033861576261,-2.08531481131674,
-2.05272994009653,-1.96611697937537,-1.90191556761914,-1.83736857855361,
-1.75492110859993,-1.72110895505862,-1.70636375952528,-1.62121747498458,
-1.55519381364485,-1.49224145259603,-1.40074251949297,-1.36878041841618,
-1.30285834918699,-1.21855005778575,-1.162097566399,-1.0961716147161,-1.03968999970123,
-1.00686929024496,-0.962893811918559,-0.868682850224344,-0.811720046912751,
-0.743809316271993,-0.688833908848399,-0.654481905197044,-0.605029867622139,
-0.522007255792696,-0.469543740804877,-0.407196423362226,-0.343212260589455,
-0.312139103092669,-0.206243036740045,-0.149073400185228,-0.000110996093532989),
 .UNSPECIFIED.);
#2960=B_SPLINE_CURVE_WITH_KNOTS('',3,(#24835,#24836,#24837,#24838,#24839,
#24840,#24841,#24842,#24843,#24844,#24845,#24846),.UNSPECIFIED.,.F.,.F.,
(4,2,2,2,2,4),(-8.82178672303514,-8.79444566643878,-8.74517120012775,-8.67475029100605,
-8.62305989272208,-8.57207326543173),.UNSPECIFIED.);
#2961=B_SPLINE_CURVE_WITH_KNOTS('',3,(#24848,#24849,#24850,#24851,#24852,
#24853,#24854,#24855,#24856,#24857,#24858,#24859,#24860,#24861,#24862,#24863),
 .UNSPECIFIED.,.F.,.F.,(4,3,3,3,3,4),(-10.4919945899008,-10.4217610239497,
-10.3408897465942,-10.2600358481682,-10.1791909548845,-10.1362407613903),
 .UNSPECIFIED.);
#2962=B_SPLINE_CURVE_WITH_KNOTS('',3,(#24864,#24865,#24866,#24867,#24868,
#24869,#24870,#24871,#24872,#24873,#24874,#24875,#24876,#24877,#24878,#24879),
 .UNSPECIFIED.,.F.,.F.,(4,1,1,1,1,1,1,1,1,1,1,1,1,4),(-10.1362407381615,
-9.92548668947589,-9.4292123550021,-8.9329380205283,-8.43666368605451,-7.94038935158072,
-7.44411501710692,-6.94784068263312,-6.45156634815933,-5.95529201368554,
-5.45901767921174,-4.96274334473795,-4.46646901026415,-4.20879728873375),
 .UNSPECIFIED.);
#2963=B_SPLINE_CURVE_WITH_KNOTS('',3,(#24882,#24883,#24884,#24885,#24886,
#24887,#24888,#24889,#24890,#24891,#24892,#24893,#24894,#24895,#24896,#24897,
#24898,#24899,#24900,#24901,#24902,#24903,#24904,#24905,#24906,#24907,#24908,
#24909,#24910,#24911,#24912,#24913,#24914,#24915,#24916,#24917,#24918,#24919,
#24920,#24921,#24922,#24923,#24924,#24925,#24926,#24927,#24928,#24929,#24930,
#24931,#24932,#24933,#24934,#24935,#24936,#24937,#24938,#24939,#24940,#24941,
#24942,#24943,#24944,#24945,#24946,#24947,#24948,#24949,#24950,#24951,#24952,
#24953,#24954,#24955,#24956,#24957,#24958,#24959,#24960,#24961,#24962,#24963,
#24964,#24965,#24966,#24967,#24968,#24969,#24970,#24971,#24972,#24973,#24974,
#24975,#24976,#24977,#24978,#24979,#24980,#24981,#24982,#24983,#24984,#24985,
#24986,#24987,#24988,#24989,#24990,#24991,#24992,#24993,#24994,#24995,#24996,
#24997,#24998,#24999,#25000,#25001,#25002,#25003,#25004,#25005,#25006,#25007,
#25008,#25009,#25010,#25011,#25012,#25013,#25014,#25015,#25016,#25017,#25018,
#25019,#25020,#25021,#25022,#25023,#25024,#25025,#25026,#25027,#25028,#25029,
#25030,#25031,#25032,#25033,#25034,#25035,#25036,#25037,#25038,#25039,#25040,
#25041,#25042,#25043,#25044,#25045,#25046,#25047,#25048,#25049,#25050,#25051,
#25052,#25053),.UNSPECIFIED.,.F.,.F.,(4,3,3,3,3,3,3,3,3,3,3,3,3,3,3,3,3,
3,3,3,3,3,3,3,3,3,3,3,3,3,3,3,3,3,3,3,3,3,3,3,3,3,3,3,3,3,3,3,3,3,3,3,3,
3,3,3,3,4),(17.9333380487234,18.0108233197382,18.0883135892053,18.1658013598437,
18.2433074384587,18.3064741618976,18.3839791341702,18.4614700138817,18.538952337374,
18.6164408059227,18.6939290593022,18.7714334678537,18.8027484963714,18.8802535677613,
18.9577445479216,19.0352269728638,19.1127155435947,19.1902038993907,19.2677084100512,
19.2990228308452,19.3765278382868,19.454018753699,19.5315011133061,19.6089896183162,
19.6864779082904,19.7639823534002,19.7952971653189,19.8728022043913,19.9502931518055,
20.027775543681,20.1052640811144,20.1827524035413,20.2602568809398,20.2915714997927,
20.369076527175,20.4465674627749,20.5240498427505,20.6015383682459,20.6790266787349,
20.7565311442723,20.7878458342665,20.8653508638495,20.9428418016642,21.0203241838615,
21.097812711572,21.1753010242683,21.2528054919869,21.2841201687403,21.3616251994293,
21.4391161383701,21.51659852171,21.5940870505792,21.6715753644414,21.7490798333289,
21.7803945032141,21.8595346027181,21.9386551930325,21.9911485717322),
 .UNSPECIFIED.);
#2964=B_SPLINE_CURVE_WITH_KNOTS('',3,(#25054,#25055,#25056,#25057,#25058,
#25059,#25060,#25061),.UNSPECIFIED.,.F.,.F.,(4,1,1,1,1,4),(21.9911485751285,
22.2766688376879,22.7729431721617,23.2692175066355,23.7654918411093,24.2164925491897),
 .UNSPECIFIED.);
#2965=B_SPLINE_CURVE_WITH_KNOTS('',3,(#25063,#25064,#25065,#25066,#25067,
#25068,#25069,#25070,#25071,#25072,#25073,#25074,#25075,#25076,#25077,#25078,
#25079,#25080,#25081,#25082,#25083,#25084,#25085,#25086,#25087,#25088,#25089,
#25090,#25091,#25092,#25093,#25094,#25095,#25096,#25097,#25098,#25099,#25100,
#25101,#25102,#25103,#25104,#25105,#25106,#25107,#25108,#25109,#25110,#25111,
#25112,#25113,#25114,#25115,#25116,#25117,#25118,#25119,#25120,#25121,#25122,
#25123,#25124,#25125,#25126,#25127,#25128,#25129,#25130,#25131,#25132,#25133,
#25134,#25135,#25136,#25137,#25138,#25139,#25140,#25141,#25142,#25143,#25144,
#25145,#25146,#25147,#25148,#25149,#25150,#25151,#25152,#25153,#25154,#25155,
#25156),.UNSPECIFIED.,.F.,.F.,(4,3,3,3,3,3,3,3,3,3,3,3,3,3,3,3,3,3,3,3,
3,3,3,3,3,3,3,3,3,3,3,4),(21.9911485751285,22.0685137227498,22.14588444626,
22.2232545020621,22.3006419241412,22.3392429283936,22.416747967466,22.4942389148803,
22.571721306756,22.6492098441894,22.7266981666165,22.804202644015,22.8355172628674,
22.9130222902497,22.9905132258493,23.0679956058247,23.1454841313203,23.2229724418092,
23.3004769073466,23.3317915973412,23.4092966269243,23.486787564739,23.5642699469356,
23.641758474646,23.7192467873425,23.7967512550612,23.828065931815,23.9055702049626,
23.9833003073723,24.0607857874918,24.1386382010467,24.2164906146016),
 .UNSPECIFIED.);
#2966=B_SPLINE_CURVE_WITH_KNOTS('',3,(#25157,#25158,#25159,#25160,#25161,
#25162,#25163,#25164,#25165,#25166,#25167,#25168),.UNSPECIFIED.,.F.,.F.,
(4,1,1,1,1,1,1,1,1,4),(17.9333400728794,18.3690482526032,18.865322587077,
19.3615969215508,19.8578712560246,20.3541455904984,20.8504199249722,21.346694259446,
21.8429685939198,21.9911485487957),.UNSPECIFIED.);
#2967=B_SPLINE_CURVE_WITH_KNOTS('',3,(#25805,#25806,#25807,#25808,#25809,
#25810,#25811,#25812,#25813,#25814,#25815,#25816,#25817,#25818,#25819,#25820,
#25821,#25822,#25823,#25824,#25825,#25826,#25827,#25828,#25829,#25830,#25831,
#25832,#25833,#25834,#25835,#25836,#25837,#25838,#25839,#25840,#25841,#25842,
#25843,#25844,#25845,#25846,#25847,#25848,#25849,#25850,#25851,#25852,#25853,
#25854,#25855,#25856,#25857,#25858,#25859,#25860,#25861,#25862,#25863,#25864,
#25865,#25866,#25867,#25868,#25869,#25870,#25871,#25872,#25873,#25874,#25875,
#25876,#25877,#25878,#25879,#25880,#25881,#25882,#25883,#25884,#25885,#25886,
#25887,#25888,#25889,#25890,#25891,#25892,#25893,#25894,#25895,#25896,#25897,
#25898,#25899,#25900,#25901,#25902,#25903,#25904,#25905,#25906,#25907,#25908,
#25909,#25910,#25911,#25912,#25913),.UNSPECIFIED.,.F.,.F.,(4,3,3,3,3,3,
3,3,3,3,3,3,3,3,3,3,3,3,3,3,3,3,3,3,3,3,3,3,3,3,3,3,3,3,3,3,4),(0.,0.0625573555055976,
0.125878327368043,0.18909072172842,0.251393671417134,0.304922771869898,
0.312525381797511,0.319603549735867,0.381466347527152,0.398722998462767,
0.460761132960107,0.522788946210543,0.584119984043925,0.609251897050035,
0.616406215049582,0.623860834291625,0.684593333574402,0.744931857036463,
0.784341213415679,0.847163709339813,0.909986205263948,0.918319049054216,
0.97788433880908,1.03729699480677,1.09693860144022,1.15658020807367,1.18303706385244,
1.19757756249814,1.20796090274694,1.26646558172373,1.3247313868406,1.36823505430382,
1.37738657121944,1.43493464047012,1.49171401465407,1.51467421871742,1.53973642054055),
 .UNSPECIFIED.);
#2968=B_SPLINE_CURVE_WITH_KNOTS('',3,(#25914,#25915,#25916,#25917,#25918,
#25919,#25920,#25921,#25922,#25923,#25924,#25925,#25926,#25927,#25928,#25929,
#25930,#25931,#25932,#25933,#25934,#25935,#25936,#25937,#25938,#25939,#25940,
#25941,#25942,#25943,#25944,#25945,#25946,#25947,#25948,#25949,#25950,#25951,
#25952,#25953,#25954,#25955,#25956,#25957,#25958,#25959,#25960,#25961,#25962,
#25963,#25964,#25965,#25966,#25967,#25968,#25969,#25970,#25971,#25972,#25973,
#25974,#25975,#25976,#25977,#25978,#25979,#25980,#25981,#25982,#25983,#25984,
#25985,#25986,#25987,#25988,#25989,#25990,#25991,#25992,#25993,#25994,#25995,
#25996,#25997,#25998,#25999,#26000,#26001,#26002,#26003,#26004,#26005,#26006,
#26007,#26008,#26009,#26010,#26011,#26012,#26013,#26014,#26015,#26016,#26017,
#26018,#26019,#26020,#26021,#26022,#26023,#26024,#26025,#26026,#26027,#26028,
#26029,#26030,#26031),.UNSPECIFIED.,.F.,.F.,(4,3,3,3,3,3,3,3,3,3,3,3,3,
3,3,3,3,3,3,3,3,3,3,3,3,3,3,3,3,3,3,3,3,3,3,3,3,3,3,4),(0.,0.0558770828944057,
0.113141002024866,0.170836081600947,0.226512310746881,0.254350425319848,
0.268269482606332,0.277344944194597,0.282188539892815,0.341010793961021,
0.356700869327603,0.414900143477246,0.473727786287952,0.532755410441651,
0.550847767022388,0.561747769745167,0.570285683041986,0.630075869297723,
0.690421239086179,0.726872796438621,0.786792026171573,0.847034073674744,
0.85453090427754,0.863944001987961,0.925525636112025,0.986994127643801,
1.04863233306401,1.11027053848422,1.15749615432221,1.16513297885951,1.22688035244015,
1.28927963589503,1.32015168917181,1.33465273393439,1.34439171958657,1.35395106897205,
1.4172068923124,1.4805171829652,1.50616871736932,1.53495510956274),
 .UNSPECIFIED.);
#2969=B_SPLINE_CURVE_WITH_KNOTS('',3,(#26668,#26669,#26670,#26671,#26672,
#26673,#26674,#26675,#26676,#26677,#26678,#26679,#26680,#26681,#26682,#26683,
#26684,#26685,#26686,#26687,#26688,#26689,#26690,#26691,#26692,#26693,#26694,
#26695,#26696,#26697,#26698,#26699,#26700,#26701,#26702,#26703,#26704,#26705,
#26706,#26707,#26708,#26709,#26710,#26711,#26712,#26713,#26714,#26715,#26716,
#26717,#26718,#26719,#26720,#26721,#26722,#26723,#26724,#26725,#26726,#26727,
#26728,#26729,#26730,#26731,#26732,#26733,#26734,#26735,#26736,#26737,#26738,
#26739,#26740,#26741,#26742,#26743,#26744,#26745,#26746,#26747,#26748,#26749,
#26750,#26751,#26752,#26753,#26754,#26755,#26756,#26757,#26758,#26759,#26760,
#26761,#26762,#26763,#26764,#26765,#26766,#26767,#26768,#26769,#26770,#26771,
#26772,#26773),.UNSPECIFIED.,.F.,.F.,(4,3,3,3,3,3,3,3,3,3,3,3,3,3,3,3,3,
3,3,3,3,3,3,3,3,3,3,3,3,3,3,3,3,3,3,4),(0.,0.0558602583733117,0.113102874179053,
0.170787757446949,0.228459514024139,0.275917418730984,0.284810036819283,
0.343644920942749,0.35670086932759,0.414962508627316,0.47376239878265,0.532768485616126,
0.557903354456782,0.567232860585173,0.62699085349851,0.687333251691766,
0.726872796438614,0.78679202603564,0.847034072316043,0.85453090427055,0.861553469994431,
0.923732737116866,0.985191220366593,1.04773087942538,1.11027053848417,1.15749615445995,
1.16513297888962,1.22688035264506,1.2892796358153,1.32015168909275,1.34459345495989,
1.35352159663707,1.41677518013709,1.48008662244226,1.50616871736924,1.53495770636289),
 .UNSPECIFIED.);
#2970=B_SPLINE_CURVE_WITH_KNOTS('',3,(#26775,#26776,#26777,#26778),
 .UNSPECIFIED.,.F.,.F.,(4,4),(-0.000938309331961322,0.),.UNSPECIFIED.);
#2971=B_SPLINE_CURVE_WITH_KNOTS('',3,(#26779,#26780,#26781,#26782,#26783,
#26784,#26785,#26786,#26787,#26788,#26789,#26790,#26791,#26792,#26793,#26794,
#26795,#26796,#26797,#26798,#26799,#26800,#26801,#26802,#26803,#26804,#26805,
#26806,#26807,#26808,#26809,#26810,#26811,#26812,#26813,#26814,#26815,#26816,
#26817,#26818,#26819,#26820,#26821,#26822,#26823,#26824,#26825,#26826,#26827,
#26828,#26829,#26830,#26831,#26832,#26833,#26834,#26835,#26836,#26837,#26838,
#26839,#26840,#26841,#26842,#26843,#26844,#26845,#26846,#26847,#26848,#26849,
#26850,#26851,#26852,#26853,#26854,#26855,#26856,#26857,#26858,#26859,#26860,
#26861,#26862,#26863,#26864,#26865,#26866,#26867,#26868,#26869,#26870,#26871,
#26872,#26873,#26874,#26875,#26876,#26877,#26878,#26879,#26880,#26881,#26882,
#26883,#26884,#26885,#26886,#26887,#26888,#26889,#26890,#26891,#26892,#26893),
 .UNSPECIFIED.,.F.,.F.,(4,3,3,3,3,3,3,3,3,3,3,3,3,3,3,3,3,3,3,3,3,3,3,3,
3,3,3,3,3,3,3,3,3,3,3,3,3,3,4),(8.32765479367532E-15,0.0625573555448621,
0.125878327380841,0.189090721668103,0.251393670961933,0.304922771867042,
0.312525381935688,0.319603549767331,0.38146634752137,0.398722998462751,
0.460761132980128,0.522788946141237,0.584119984199227,0.609251897024497,
0.616406215120755,0.623860834300335,0.684593333606756,0.744931857050254,
0.784341213415659,0.845068255831707,0.884007249861946,0.901043059750176,
0.912236715472706,0.920839905576931,0.980342222581217,1.03974346201836,
1.09825254793676,1.15658020807362,1.18303706386245,1.1975775625098,1.20796090260796,
1.26646558135057,1.32473138703364,1.36823505438423,1.37738657107583,1.43493464029449,
1.49171401425249,1.51467421871737,1.53973642054051),.UNSPECIFIED.);
#2972=B_SPLINE_CURVE_WITH_KNOTS('',3,(#27208,#27209,#27210,#27211,#27212,
#27213,#27214,#27215),.UNSPECIFIED.,.F.,.F.,(4,2,2,4),(9.38674526974159E-7,
0.197912071307587,0.244750653263811,0.283675624189322),.UNSPECIFIED.);
#2973=B_SPLINE_CURVE_WITH_KNOTS('',3,(#27217,#27218,#27219,#27220,#27221,
#27222,#27223,#27224,#27225,#27226),.UNSPECIFIED.,.F.,.F.,(4,2,2,2,4),(0.,
0.00238154318238252,0.00529193749553023,0.0121953093380869,0.0169288782364552),
 .UNSPECIFIED.);
#2974=B_SPLINE_CURVE_WITH_KNOTS('',3,(#27235,#27236,#27237,#27238,#27239,
#27240,#27241,#27242),.UNSPECIFIED.,.F.,.F.,(4,2,2,4),(9.39134819485715E-7,
0.313007067364836,0.466067686181722,0.641395236280365),.UNSPECIFIED.);
#2975=B_SPLINE_CURVE_WITH_KNOTS('',3,(#27244,#27245,#27246,#27247,#27248,
#27249,#27250,#27251,#27252,#27253),.UNSPECIFIED.,.F.,.F.,(4,2,2,2,4),(0.,
0.00238340067887078,0.00529624616302871,0.0122051825225569,0.0169424867765656),
 .UNSPECIFIED.);
#2976=B_SPLINE_CURVE_WITH_KNOTS('',3,(#27262,#27263,#27264,#27265,#27266,
#27267,#27268,#27269),.UNSPECIFIED.,.F.,.F.,(4,2,2,4),(9.38674282470181E-7,
0.197987316009641,0.244851770135215,0.28379594641037),.UNSPECIFIED.);
#2977=B_SPLINE_CURVE_WITH_KNOTS('',3,(#27271,#27272,#27273,#27274,#27275,
#27276,#27277,#27278),.UNSPECIFIED.,.F.,.F.,(4,2,2,4),(0.,0.0047633736137187,
0.00902722460288498,0.0150831942940084),.UNSPECIFIED.);
#2978=B_SPLINE_CURVE_WITH_KNOTS('',3,(#27287,#27288,#27289,#27290,#27291,
#27292,#27293,#27294),.UNSPECIFIED.,.F.,.F.,(4,2,2,4),(9.39136670358377E-7,
0.313011184875832,0.466084249009382,0.641473613344403),.UNSPECIFIED.);
#2979=B_SPLINE_CURVE_WITH_KNOTS('',3,(#27296,#27297,#27298,#27299,#27300,
#27301,#27302,#27303,#27304,#27305),.UNSPECIFIED.,.F.,.F.,(4,2,2,2,4),(0.,
0.00237357460738177,0.0052734579858211,0.0121529658906331,0.0168705147066673),
 .UNSPECIFIED.);
#2980=B_SPLINE_CURVE_WITH_KNOTS('',3,(#27314,#27315,#27316,#27317,#27318,
#27319,#27320,#27321),.UNSPECIFIED.,.F.,.F.,(4,2,2,4),(9.39136720441153E-7,
0.313011292240562,0.466084402983163,0.641474389410526),.UNSPECIFIED.);
#2981=B_SPLINE_CURVE_WITH_KNOTS('',3,(#27323,#27324,#27325,#27326,#27327,
#27328,#27329,#27330,#27331,#27332),.UNSPECIFIED.,.F.,.F.,(4,2,2,2,4),(0.,
0.0023782900743644,0.00528439250760633,0.0121780205899161,0.0169050485394452),
 .UNSPECIFIED.);
#2982=B_SPLINE_CURVE_WITH_KNOTS('',3,(#27341,#27342,#27343,#27344,#27345,
#27346,#27347,#27348),.UNSPECIFIED.,.F.,.F.,(4,2,2,4),(9.38674284612347E-7,
0.197985480739605,0.244849302967186,0.283793010207111),.UNSPECIFIED.);
#2983=B_SPLINE_CURVE_WITH_KNOTS('',3,(#27350,#27351,#27352,#27353,#27354,
#27355,#27356,#27357,#27358,#27359),.UNSPECIFIED.,.F.,.F.,(4,2,2,2,4),(0.,
0.00238320602712813,0.00529579462832576,0.0122041478366525,0.016941060634997),
 .UNSPECIFIED.);
#2984=B_SPLINE_CURVE_WITH_KNOTS('',3,(#27368,#27369,#27370,#27371,#27372,
#27373,#27374,#27375),.UNSPECIFIED.,.F.,.F.,(4,2,2,4),(9.39134818369318E-7,
0.31300706365764,0.466067681436598,0.641395213194101),.UNSPECIFIED.);
#2985=B_SPLINE_CURVE_WITH_KNOTS('',3,(#27377,#27378,#27379,#27380,#27381,
#27382,#27383,#27384),.UNSPECIFIED.,.F.,.F.,(4,2,2,4),(0.,0.00476388970796606,
0.00902830722597645,0.0150851135700706),.UNSPECIFIED.);
#2986=B_SPLINE_CURVE_WITH_KNOTS('',3,(#27393,#27394,#27395,#27396,#27397,
#27398,#27399,#27400),.UNSPECIFIED.,.F.,.F.,(4,2,2,4),(9.39135631813739E-7,
0.313008884693273,0.466070291990264,0.641408534042971),.UNSPECIFIED.);
#2987=B_SPLINE_CURVE_WITH_KNOTS('',3,(#27402,#27403,#27404,#27405,#27406,
#27407,#27408,#27409,#27410,#27411),.UNSPECIFIED.,.F.,.F.,(4,2,2,2,4),(0.,
0.0023785439095033,0.00528498118810588,0.0121793694890388,0.0169069077752386),
 .UNSPECIFIED.);
#2988=B_SPLINE_CURVE_WITH_KNOTS('',3,(#27420,#27421,#27422,#27423,#27424,
#27425,#27426,#27427),.UNSPECIFIED.,.F.,.F.,(4,2,2,4),(9.39138223560896E-7,
0.313014634420147,0.466099866256976,0.641546846663167),.UNSPECIFIED.);
#2989=B_SPLINE_CURVE_WITH_KNOTS('',3,(#27429,#27430,#27431,#27432,#27433,
#27434,#27435,#27436,#27437,#27438),.UNSPECIFIED.,.F.,.F.,(4,2,2,2,4),(0.,
0.00237319534257096,0.0052725786320786,0.0121509510394241,0.0168677375635532),
 .UNSPECIFIED.);
#2990=B_SPLINE_CURVE_WITH_KNOTS('',3,(#27447,#27448,#27449,#27450,#27451,
#27452,#27453,#27454),.UNSPECIFIED.,.F.,.F.,(4,2,2,4),(9.38674527823462E-7,
0.197912070601848,0.244750652620493,0.283675623600454),.UNSPECIFIED.);
#2991=B_SPLINE_CURVE_WITH_KNOTS('',3,(#27456,#27457,#27458,#27459,#27460,
#27461,#27462,#27463,#27464,#27465),.UNSPECIFIED.,.F.,.F.,(4,2,2,2,4),(0.,
0.00238154317971207,0.00529193748943623,0.012195309323669,0.0169288782166237),
 .UNSPECIFIED.);
#2992=B_SPLINE_CURVE_WITH_KNOTS('',3,(#27474,#27475,#27476,#27477,#27478,
#27479,#27480,#27481),.UNSPECIFIED.,.F.,.F.,(4,2,2,4),(9.3913481761243E-7,
0.31300706664949,0.466067685923882,0.641395236588582),.UNSPECIFIED.);
#2993=B_SPLINE_CURVE_WITH_KNOTS('',3,(#27483,#27484,#27485,#27486,#27487,
#27488,#27489,#27490),.UNSPECIFIED.,.F.,.F.,(4,2,2,4),(0.,0.00476393585611593,
0.00902840402447764,0.0150852851575008),.UNSPECIFIED.);
#2994=B_SPLINE_CURVE_WITH_KNOTS('',3,(#27499,#27500,#27501,#27502,#27503,
#27504,#27505,#27506),.UNSPECIFIED.,.F.,.F.,(4,2,2,4),(9.38674282697379E-7,
0.197987318201236,0.24485177211621,0.283795948207931),.UNSPECIFIED.);
#2995=B_SPLINE_CURVE_WITH_KNOTS('',3,(#27508,#27509,#27510,#27511,#27512,
#27513,#27514,#27515,#27516,#27517),.UNSPECIFIED.,.F.,.F.,(4,2,2,2,4),(0.,
0.0023816918039995,0.00529228222519305,0.0121960992691896,0.0169299670267326),
 .UNSPECIFIED.);
#2996=B_SPLINE_CURVE_WITH_KNOTS('',3,(#27526,#27527,#27528,#27529,#27530,
#27531,#27532,#27533),.UNSPECIFIED.,.F.,.F.,(4,2,2,4),(9.39136669948809E-7,
0.313011185099831,0.466084249090031,0.641473613246853),.UNSPECIFIED.);
#2997=B_SPLINE_CURVE_WITH_KNOTS('',3,(#27535,#27536,#27537,#27538,#27539,
#27540,#27541,#27542,#27543,#27544),.UNSPECIFIED.,.F.,.F.,(4,2,2,2,4),(0.,
0.00237357460648197,0.00527345798380301,0.0121529658846397,0.016870514699817),
 .UNSPECIFIED.);
#2998=B_SPLINE_CURVE_WITH_KNOTS('',3,(#27553,#27554,#27555,#27556,#27557,
#27558,#27559,#27560),.UNSPECIFIED.,.F.,.F.,(4,2,2,4),(9.39136719522134E-7,
0.313011292197314,0.466084402967806,0.641474389430124),.UNSPECIFIED.);
#2999=B_SPLINE_CURVE_WITH_KNOTS('',3,(#27562,#27563,#27564,#27565,#27566,
#27567,#27568,#27569,#27570,#27571),.UNSPECIFIED.,.F.,.F.,(4,2,2,2,4),(0.,
0.00237829007741614,0.00528439251454885,0.0121780206098593,0.0169050485629513),
 .UNSPECIFIED.);
#3000=B_SPLINE_CURVE_WITH_KNOTS('',3,(#27580,#27581,#27582,#27583,#27584,
#27585,#27586,#27587),.UNSPECIFIED.,.F.,.F.,(4,2,2,4),(9.38674290583485E-7,
0.197985478708047,0.244849301132532,0.283793008543649),.UNSPECIFIED.);
#3001=B_SPLINE_CURVE_WITH_KNOTS('',3,(#27589,#27590,#27591,#27592,#27593,
#27594,#27595,#27596,#27597,#27598),.UNSPECIFIED.,.F.,.F.,(4,2,2,2,4),(0.,
0.00238320602681499,0.00529579462760504,0.0122041478355376,0.0169410606327885),
 .UNSPECIFIED.);
#3002=B_SPLINE_CURVE_WITH_KNOTS('',3,(#27607,#27608,#27609,#27610,#27611,
#27612,#27613,#27614),.UNSPECIFIED.,.F.,.F.,(4,2,2,4),(9.39134818485942E-7,
0.313007063639476,0.466067681430211,0.641395213202689),.UNSPECIFIED.);
#3003=B_SPLINE_CURVE_WITH_KNOTS('',3,(#27616,#27617,#27618,#27619,#27620,
#27621,#27622,#27623,#27624,#27625),.UNSPECIFIED.,.F.,.F.,(4,2,2,2,4),(0.,
0.00288584394666921,0.00676564596185734,0.0194599953243108,0.045988200349411),
 .UNSPECIFIED.);
#3004=B_SPLINE_CURVE_WITH_KNOTS('',3,(#27634,#27635,#27636,#27637,#27638,
#27639,#27640,#27641),.UNSPECIFIED.,.F.,.F.,(4,2,2,4),(9.39138223334931E-7,
0.31301463434841,0.466099866231014,0.641546846692122),.UNSPECIFIED.);
#3005=B_SPLINE_CURVE_WITH_KNOTS('',3,(#27643,#27644,#27645,#27646,#27647,
#27648,#27649,#27650,#27651,#27652),.UNSPECIFIED.,.F.,.F.,(4,2,2,2,4),(0.,
0.00288578889265372,0.00676552602658123,0.0194588364051688,0.0459849509963726),
 .UNSPECIFIED.);
#3006=B_SPLINE_CURVE_WITH_KNOTS('',3,(#27661,#27662,#27663,#27664,#27665,
#27666,#27667,#27668),.UNSPECIFIED.,.F.,.F.,(4,2,2,4),(9.38674512203643E-7,
0.197915707554863,0.244755539870822,0.283681439071384),.UNSPECIFIED.);
#3007=B_SPLINE_CURVE_WITH_KNOTS('',3,(#27670,#27671,#27672,#27673,#27674,
#27675,#27676,#27677,#27678,#27679),.UNSPECIFIED.,.F.,.F.,(4,2,2,2,4),(0.,
0.00288581812123732,0.00676558988611721,0.0194594510099433,0.0459866741536432),
 .UNSPECIFIED.);
#3008=B_SPLINE_CURVE_WITH_KNOTS('',3,(#27692,#27693,#27694,#27695,#27696,
#27697,#27698,#27699),.UNSPECIFIED.,.F.,.F.,(4,2,2,4),(9.3913745254888E-7,
0.313012920882138,0.466097404509773,0.641534556152897),.UNSPECIFIED.);
#3009=B_SPLINE_CURVE_WITH_KNOTS('',3,(#27703,#27704,#27705,#27706,#27707,
#27708,#27709,#27710,#27711,#27712),.UNSPECIFIED.,.F.,.F.,(4,2,2,2,4),(0.,
0.00288577255855134,0.00676549015491415,0.0194584932984043,0.0459839884509012),
 .UNSPECIFIED.);
#3010=B_SPLINE_CURVE_WITH_KNOTS('',3,(#27725,#27726,#27727,#27728,#27729,
#27730,#27731,#27732,#27733,#27734),.UNSPECIFIED.,.F.,.F.,(4,2,2,2,4),(9.38676322936076E-7,
0.190216558583583,0.359875507174653,0.441533870949612,0.507581347070439),
 .UNSPECIFIED.);
#3011=B_SPLINE_CURVE_WITH_KNOTS('',3,(#27738,#27739,#27740,#27741,#27742,
#27743,#27744,#27745),.UNSPECIFIED.,.F.,.F.,(4,2,2,4),(0.,0.00476287317060948,
0.0090261747394427,0.0150813329561307),.UNSPECIFIED.);
#3012=B_SPLINE_CURVE_WITH_KNOTS('',3,(#27758,#27759,#27760,#27761,#27762,
#27763,#27764,#27765,#27766,#27767),.UNSPECIFIED.,.F.,.F.,(4,2,2,2,4),(9.38676132424859E-7,
0.190216675552138,0.359875382199115,0.441534255569763,0.507580281805651),
 .UNSPECIFIED.);
#3013=B_SPLINE_CURVE_WITH_KNOTS('',3,(#27771,#27772,#27773,#27774,#27775,
#27776,#27777,#27778,#27779,#27780),.UNSPECIFIED.,.F.,.F.,(4,2,2,2,4),(0.,
0.00288584518508398,0.00676564864347784,0.0194600214082376,0.0459882734084581),
 .UNSPECIFIED.);
#3014=B_SPLINE_CURVE_WITH_KNOTS('',3,(#27793,#27794,#27795,#27796,#27797,
#27798,#27799,#27800),.UNSPECIFIED.,.F.,.F.,(4,2,2,4),(9.38674377615734E-7,
0.19795837352917,0.244812875199329,0.283749664140645),.UNSPECIFIED.);
#3015=B_SPLINE_CURVE_WITH_KNOTS('',3,(#27804,#27805,#27806,#27807,#27808,
#27809,#27810,#27811),.UNSPECIFIED.,.F.,.F.,(4,2,2,4),(0.,0.00476368678937328,
0.00902788155483768,0.0150843589237395),.UNSPECIFIED.);
#3016=B_SPLINE_CURVE_WITH_KNOTS('',3,(#27824,#27825,#27826,#27827,#27828,
#27829,#27830,#27831,#27832,#27833),.UNSPECIFIED.,.F.,.F.,(4,2,2,2,4),(9.38677117360782E-7,
0.190216058945539,0.359865342787696,0.44150491422111,0.507545138629862),
 .UNSPECIFIED.);
#3017=B_SPLINE_CURVE_WITH_KNOTS('',3,(#27837,#27838,#27839,#27840,#27841,
#27842,#27843,#27844,#27845,#27846),.UNSPECIFIED.,.F.,.F.,(4,2,2,2,4),(0.,
0.00288580557302315,0.00676556252532466,0.0194591867332428,0.0459859327527602),
 .UNSPECIFIED.);
#3018=B_SPLINE_CURVE_WITH_KNOTS('',3,(#27859,#27860,#27861,#27862,#27863,
#27864,#27865,#27866,#27867,#27868),.UNSPECIFIED.,.F.,.F.,(4,2,2,2,4),(9.38676644870429E-7,
0.190216354160521,0.359865058426445,0.441505964266297,0.507542572156931),
 .UNSPECIFIED.);
#3019=B_SPLINE_CURVE_WITH_KNOTS('',3,(#27872,#27873,#27874,#27875,#27876,
#27877,#27878,#27879,#27880,#27881),.UNSPECIFIED.,.F.,.F.,(4,2,2,2,4),(0.,
0.00288580454690941,0.00676556028459874,0.0194591651238233,0.0459858721133107),
 .UNSPECIFIED.);
#3020=B_SPLINE_CURVE_WITH_KNOTS('',3,(#27894,#27895,#27896,#27897,#27898,
#27899,#27900,#27901,#27902,#27903),.UNSPECIFIED.,.F.,.F.,(4,2,2,2,4),(9.38676160620083E-7,
0.19021666331625,0.359875396536414,0.441534218705211,0.507580398815235),
 .UNSPECIFIED.);
#3021=B_SPLINE_CURVE_WITH_KNOTS('',3,(#27907,#27908,#27909,#27910,#27911,
#27912,#27913,#27914),.UNSPECIFIED.,.F.,.F.,(4,2,2,4),(0.,0.00476366682174163,
0.00902783959238785,0.0150842843350958),.UNSPECIFIED.);
#3022=B_SPLINE_CURVE_WITH_KNOTS('',3,(#27927,#27928,#27929,#27930,#27931,
#27932,#27933,#27934),.UNSPECIFIED.,.F.,.F.,(4,2,2,4),(9.38674218968633E-7,
0.198006053174433,0.24487695114834,0.283825910095945),.UNSPECIFIED.);
#3023=B_SPLINE_CURVE_WITH_KNOTS('',3,(#27938,#27939,#27940,#27941,#27942,
#27943,#27944,#27945,#27946,#27947),.UNSPECIFIED.,.F.,.F.,(4,2,2,2,4),(0.,
0.00288584520885465,0.00676564869365475,0.0194600220037921,0.0459882752473628),
 .UNSPECIFIED.);
#3024=B_SPLINE_CURVE_WITH_KNOTS('',3,(#27960,#27961,#27962,#27963,#27964,
#27965,#27966,#27967,#27968,#27969),.UNSPECIFIED.,.F.,.F.,(4,2,2,2,4),(9.38676621047222E-7,
0.190216370014355,0.35986504387141,0.4415060225351,0.507542435940933),
 .UNSPECIFIED.);
#3025=B_SPLINE_CURVE_WITH_KNOTS('',3,(#27973,#27974,#27975,#27976,#27977,
#27978,#27979,#27980,#27981,#27982),.UNSPECIFIED.,.F.,.F.,(4,2,2,2,4),(0.,
0.00288582767659631,0.00676561067367699,0.0194596521031919,0.0459872376775252),
 .UNSPECIFIED.);
#3026=B_SPLINE_CURVE_WITH_KNOTS('',3,(#27995,#27996,#27997,#27998,#27999,
#28000,#28001,#28002,#28003,#28004),.UNSPECIFIED.,.F.,.F.,(4,2,2,2,4),(9.38677156228019E-7,
0.190216034794342,0.359865371222063,0.44150484321002,0.507545363962411),
 .UNSPECIFIED.);
#3027=B_SPLINE_CURVE_WITH_KNOTS('',3,(#28008,#28009,#28010,#28011,#28012,
#28013,#28014,#28015,#28016,#28017),.UNSPECIFIED.,.F.,.F.,(4,2,2,2,4),(0.,
0.00288577255842772,0.00676549015463377,0.0194584932973895,0.0459839884562596),
 .UNSPECIFIED.);
#3028=B_SPLINE_CURVE_WITH_KNOTS('',3,(#28030,#28031,#28032,#28033,#28034,
#28035,#28036,#28037,#28038,#28039),.UNSPECIFIED.,.F.,.F.,(4,2,2,2,4),(9.38676323177046E-7,
0.190216558327547,0.359875507149927,0.441533871021912,0.507581347237268),
 .UNSPECIFIED.);
#3029=B_SPLINE_CURVE_WITH_KNOTS('',3,(#28043,#28044,#28045,#28046,#28047,
#28048,#28049,#28050),.UNSPECIFIED.,.F.,.F.,(4,2,2,4),(0.,0.00476287319732046,
0.00902617482142203,0.0150813331688102),.UNSPECIFIED.);
#3030=B_SPLINE_CURVE_WITH_KNOTS('',3,(#28063,#28064,#28065,#28066,#28067,
#28068,#28069,#28070),.UNSPECIFIED.,.F.,.F.,(4,2,2,4),(9.38674206481295E-7,
0.198010313344894,0.244882676520894,0.28383272291311),.UNSPECIFIED.);
#3031=B_SPLINE_CURVE_WITH_KNOTS('',3,(#28074,#28075,#28076,#28077,#28078,
#28079,#28080,#28081,#28082,#28083),.UNSPECIFIED.,.F.,.F.,(4,2,2,2,4),(0.,
0.00288584517738443,0.00676564862539164,0.0194600213508031,0.0459882734381834),
 .UNSPECIFIED.);
#3032=B_SPLINE_CURVE_WITH_KNOTS('',3,(#28096,#28097,#28098,#28099,#28100,
#28101,#28102,#28103,#28104,#28105),.UNSPECIFIED.,.F.,.F.,(4,2,2,2,4),(9.38676310254617E-7,
0.190216568196222,0.359875496482002,0.441533899642992,0.507581258743622),
 .UNSPECIFIED.);
#3033=B_SPLINE_CURVE_WITH_KNOTS('',3,(#28109,#28110,#28111,#28112,#28113,
#28114,#28115,#28116),.UNSPECIFIED.,.F.,.F.,(4,2,2,4),(0.,0.00476368668604745,
0.0090278812393193,0.0150843581077754),.UNSPECIFIED.);
#3034=B_SPLINE_CURVE_WITH_KNOTS('',3,(#28129,#28130,#28131,#28132,#28133,
#28134,#28135,#28136,#28137,#28138),.UNSPECIFIED.,.F.,.F.,(4,2,2,2,4),(9.38677117179183E-7,
0.190216058846508,0.359865342778253,0.44150491424923,0.507545138694429),
 .UNSPECIFIED.);
#3035=B_SPLINE_CURVE_WITH_KNOTS('',3,(#28142,#28143,#28144,#28145,#28146,
#28147,#28148,#28149,#28150,#28151),.UNSPECIFIED.,.F.,.F.,(4,2,2,2,4),(0.,
0.0028858055760958,0.00676556253253746,0.0194591867562179,0.0459859327383561),
 .UNSPECIFIED.);
#3036=B_SPLINE_CURVE_WITH_KNOTS('',3,(#28164,#28165,#28166,#28167,#28168,
#28169,#28170,#28171,#28172,#28173),.UNSPECIFIED.,.F.,.F.,(4,2,2,2,4),(9.38676644713873E-7,
0.190216354185753,0.359865058428838,0.441505964259139,0.507542572138923),
 .UNSPECIFIED.);
#3037=B_SPLINE_CURVE_WITH_KNOTS('',3,(#28177,#28178,#28179,#28180,#28181,
#28182,#28183,#28184,#28185,#28186),.UNSPECIFIED.,.F.,.F.,(4,2,2,2,4),(0.,
0.00288580454917283,0.00676556028991565,0.0194591651405655,0.045985872109436),
 .UNSPECIFIED.);
#3038=B_SPLINE_CURVE_WITH_KNOTS('',3,(#28199,#28200,#28201,#28202,#28203,
#28204,#28205,#28206,#28207,#28208),.UNSPECIFIED.,.F.,.F.,(4,2,2,2,4),(9.38676160335773E-7,
0.190216663193983,0.35987539652473,0.441534218739778,0.507580398893346),
 .UNSPECIFIED.);
#3039=B_SPLINE_CURVE_WITH_KNOTS('',3,(#28212,#28213,#28214,#28215,#28216,
#28217,#28218,#28219),.UNSPECIFIED.,.F.,.F.,(4,2,2,4),(0.,0.00476366691827938,
0.00902783988845374,0.0150842851027805),.UNSPECIFIED.);
#3040=B_SPLINE_CURVE_WITH_KNOTS('',3,(#28232,#28233,#28234,#28235,#28236,
#28237,#28238,#28239),.UNSPECIFIED.,.F.,.F.,(4,2,2,4),(9.39134874106605E-7,
0.313007195011186,0.466067869529335,0.641396175473332),.UNSPECIFIED.);
#3041=B_SPLINE_CURVE_WITH_KNOTS('',3,(#28243,#28244,#28245,#28246,#28247,
#28248,#28249,#28250,#28251,#28252),.UNSPECIFIED.,.F.,.F.,(4,2,2,2,4),(0.,
0.00288584520947008,0.00676564869509268,0.019460022008105,0.0459882752517017),
 .UNSPECIFIED.);
#3042=B_SPLINE_CURVE_WITH_KNOTS('',3,(#28265,#28266,#28267,#28268,#28269,
#28270,#28271,#28272),.UNSPECIFIED.,.F.,.F.,(4,2,2,4),(9.39136080394831E-7,
0.313009874980368,0.466082370050846,0.641464116445783),.UNSPECIFIED.);
#3043=B_SPLINE_CURVE_WITH_KNOTS('',3,(#28276,#28277,#28278,#28279,#28280,
#28281,#28282,#28283),.UNSPECIFIED.,.F.,.F.,(4,2,2,4),(0.,0.0047629124728381,
0.00902625721222522,0.0150814792303183),.UNSPECIFIED.);
#3044=B_SPLINE_CURVE_WITH_KNOTS('',3,(#28400,#28401,#28402,#28403,#28404,
#28405),.UNSPECIFIED.,.F.,.F.,(4,2,4),(-0.00983438259802202,-0.00492102107344964,
0.),.UNSPECIFIED.);
#3045=B_SPLINE_CURVE_WITH_KNOTS('',3,(#28432,#28433,#28434,#28435,#28436,
#28437),.UNSPECIFIED.,.F.,.F.,(4,2,4),(-0.00983535924918913,-0.00492266478240658,
0.),.UNSPECIFIED.);
#3046=B_SPLINE_CURVE_WITH_KNOTS('',3,(#28473,#28474,#28475,#28476,#28477,
#28478),.UNSPECIFIED.,.F.,.F.,(4,2,4),(-0.00983535878889612,-0.00492266422265586,
0.),.UNSPECIFIED.);
#3047=B_SPLINE_CURVE_WITH_KNOTS('',3,(#28514,#28515,#28516,#28517,#28518,
#28519),.UNSPECIFIED.,.F.,.F.,(4,2,4),(-0.0098353587479088,-0.00492266417261958,
0.),.UNSPECIFIED.);
#3048=B_SPLINE_CURVE_WITH_KNOTS('',3,(#28564,#28565,#28566,#28567,#28568,
#28569),.UNSPECIFIED.,.F.,.F.,(4,2,4),(-0.00983437497489847,-0.00492101512779726,
0.),.UNSPECIFIED.);
#3049=B_SPLINE_CURVE_WITH_KNOTS('',3,(#28578,#28579,#28580,#28581,#28582,
#28583),.UNSPECIFIED.,.F.,.F.,(4,2,4),(-0.0098343785393361,-0.00492101790414255,
0.),.UNSPECIFIED.);
#3050=B_SPLINE_CURVE_WITH_KNOTS('',3,(#28588,#28589,#28590,#28591,#28592,
#28593),.UNSPECIFIED.,.F.,.F.,(4,2,4),(-0.00983438488091109,-0.00492102285998894,
0.),.UNSPECIFIED.);
#3051=B_SPLINE_CURVE_WITH_KNOTS('',3,(#28602,#28603,#28604,#28605,#28606,
#28607),.UNSPECIFIED.,.F.,.F.,(4,2,4),(-0.00983535969514932,-0.00492266532538871,
0.),.UNSPECIFIED.);
#3052=B_SPLINE_CURVE_WITH_KNOTS('',3,(#28616,#28617,#28618,#28619,#28620,
#28621),.UNSPECIFIED.,.F.,.F.,(4,2,4),(-0.00983437480440195,-0.00492101499529718,
0.),.UNSPECIFIED.);
#3053=B_SPLINE_CURVE_WITH_KNOTS('',3,(#28630,#28631,#28632,#28633,#28634,
#28635),.UNSPECIFIED.,.F.,.F.,(4,2,4),(-0.00983535897005503,-0.00492266444295711,
0.),.UNSPECIFIED.);
#3054=B_SPLINE_CURVE_WITH_KNOTS('',3,(#28644,#28645,#28646,#28647,#28648,
#28649),.UNSPECIFIED.,.F.,.F.,(4,2,4),(-0.00983438028091156,-0.00492101926303028,
0.),.UNSPECIFIED.);
#3055=B_SPLINE_CURVE_WITH_KNOTS('',3,(#28658,#28659,#28660,#28661,#28662,
#28663),.UNSPECIFIED.,.F.,.F.,(4,2,4),(-0.00983438042371488,-0.00492101937453644,
0.),.UNSPECIFIED.);
#3056=B_SPLINE_CURVE_WITH_KNOTS('',3,(#28672,#28673,#28674,#28675,#28676,
#28677),.UNSPECIFIED.,.F.,.F.,(4,2,4),(-0.00983535898766203,-0.00492266446437622,
0.),.UNSPECIFIED.);
#3057=B_SPLINE_CURVE_WITH_KNOTS('',3,(#28686,#28687,#28688,#28689,#28690,
#28691),.UNSPECIFIED.,.F.,.F.,(4,2,4),(-0.00983437480033418,-0.00492101499217869,
0.),.UNSPECIFIED.);
#3058=B_SPLINE_CURVE_WITH_KNOTS('',3,(#28700,#28701,#28702,#28703,#28704,
#28705),.UNSPECIFIED.,.F.,.F.,(4,2,4),(-0.00983437721979582,-0.00492101687559478,
0.),.UNSPECIFIED.);
#3059=B_SPLINE_CURVE_WITH_KNOTS('',3,(#28714,#28715,#28716,#28717,#28718,
#28719),.UNSPECIFIED.,.F.,.F.,(4,2,4),(-0.00983438488112925,-0.00492102286014865,
0.),.UNSPECIFIED.);
#3060=B_SPLINE_CURVE_WITH_KNOTS('',3,(#28728,#28729,#28730,#28731,#28732,
#28733),.UNSPECIFIED.,.F.,.F.,(4,2,4),(-0.00983535969514463,-0.0049226653253664,
0.),.UNSPECIFIED.);
#3061=B_SPLINE_CURVE_WITH_KNOTS('',3,(#28742,#28743,#28744,#28745,#28746,
#28747),.UNSPECIFIED.,.F.,.F.,(4,2,4),(-0.00983437480384014,-0.00492101499504691,
0.),.UNSPECIFIED.);
#3062=B_SPLINE_CURVE_WITH_KNOTS('',3,(#28756,#28757,#28758,#28759,#28760,
#28761),.UNSPECIFIED.,.F.,.F.,(4,2,4),(-0.00983535896995666,-0.00492266444279139,
0.),.UNSPECIFIED.);
#3063=B_SPLINE_CURVE_WITH_KNOTS('',3,(#28770,#28771,#28772,#28773,#28774,
#28775),.UNSPECIFIED.,.F.,.F.,(4,2,4),(-0.00983438028095572,-0.00492101926308378,
0.),.UNSPECIFIED.);
#3064=B_SPLINE_CURVE_WITH_KNOTS('',3,(#28784,#28785,#28786,#28787,#28788,
#28789),.UNSPECIFIED.,.F.,.F.,(4,2,4),(-0.00983438042362209,-0.00492101937455925,
0.),.UNSPECIFIED.);
#3065=B_SPLINE_CURVE_WITH_KNOTS('',3,(#28798,#28799,#28800,#28801,#28802,
#28803),.UNSPECIFIED.,.F.,.F.,(4,2,4),(-0.00983535898790276,-0.00492266446462651,
0.),.UNSPECIFIED.);
#3066=B_SPLINE_CURVE_WITH_KNOTS('',3,(#28812,#28813,#28814,#28815,#28816,
#28817),.UNSPECIFIED.,.F.,.F.,(4,2,4),(-0.00983437479993856,-0.00492101499183855,
0.),.UNSPECIFIED.);
#3067=B_SPLINE_CURVE_WITH_KNOTS('',3,(#28826,#28827,#28828,#28829,#28830,
#28831),.UNSPECIFIED.,.F.,.F.,(4,2,4),(-0.00983535966014206,-0.00492266528281923,
0.),.UNSPECIFIED.);
#3068=B_SPLINE_CURVE_WITH_KNOTS('',3,(#28838,#28839,#28840,#28841,#28842,
#28843,#28844,#28845,#28846,#28847,#28848,#28849,#28850,#28851),
 .UNSPECIFIED.,.F.,.F.,(4,2,2,2,2,2,4),(-0.82600395443711,-0.625773509086572,
-0.500319880314509,-0.4128988677948,-0.323416359045162,-0.187269988974532,
-3.37805815843223E-6),.UNSPECIFIED.);
#3069=B_SPLINE_CURVE_WITH_KNOTS('',3,(#28852,#28853,#28854,#28855,#28856,
#28857,#28858,#28859,#28860,#28861,#28862,#28863,#28864,#28865),
 .UNSPECIFIED.,.F.,.F.,(4,2,2,2,2,2,4),(-0.826003693746637,-0.62577441198849,
-0.500320233133826,-0.41289872345655,-0.323415723219816,-0.187268878424026,
-3.38098086435097E-6),.UNSPECIFIED.);
#3070=B_SPLINE_CURVE_WITH_KNOTS('',3,(#28867,#28868,#28869,#28870,#28871,
#28872,#28873,#28874,#28875,#28876,#28877,#28878,#28879,#28880),
 .UNSPECIFIED.,.F.,.F.,(4,2,2,2,2,2,4),(-0.826160973205696,-0.625505733497847,
-0.500256557879679,-0.412982835097184,-0.323646851595676,-0.187689432402941,
-2.22228171383796E-6),.UNSPECIFIED.);
#3071=B_SPLINE_CURVE_WITH_KNOTS('',3,(#28881,#28882,#28883,#28884,#28885,
#28886,#28887,#28888,#28889,#28890,#28891,#28892,#28893,#28894),
 .UNSPECIFIED.,.F.,.F.,(4,2,2,2,2,2,4),(-0.826160921263055,-0.625505869063133,
-0.500256603642305,-0.412982806908025,-0.323646750043836,-0.187689250732374,
-2.2228099030522E-6),.UNSPECIFIED.);
#3072=B_SPLINE_CURVE_WITH_KNOTS('',3,(#28896,#28897,#28898,#28899,#28900,
#28901,#28902,#28903,#28904,#28905,#28906,#28907,#28908,#28909),
 .UNSPECIFIED.,.F.,.F.,(4,2,2,2,2,2,4),(-0.826002804744842,-0.625777498404662,
-0.500321440270458,-0.412898231168244,-0.323413550926482,-0.187265084649461,
-3.39095613572205E-6),.UNSPECIFIED.);
#3073=B_SPLINE_CURVE_WITH_KNOTS('',3,(#28910,#28911,#28912,#28913,#28914,
#28915,#28916,#28917,#28918,#28919,#28920,#28921,#28922,#28923),
 .UNSPECIFIED.,.F.,.F.,(4,2,2,2,2,2,4),(-0.826160850959899,-0.625506052002871,
-0.50025666536275,-0.412982768750562,-0.323646612808788,-0.187689005398769,
-2.22350912481821E-6),.UNSPECIFIED.);
#3074=B_SPLINE_CURVE_WITH_KNOTS('',3,(#28925,#28926,#28927,#28928,#28929,
#28930,#28931,#28932,#28933,#28934,#28935,#28936,#28937,#28938),
 .UNSPECIFIED.,.F.,.F.,(4,2,2,2,2,2,4),(-0.826160879595006,-0.625505976987524,
-0.500256640008355,-0.412982784285415,-0.32364666890615,-0.18768910580297,
-2.22321262101263E-6),.UNSPECIFIED.);
#3075=B_SPLINE_CURVE_WITH_KNOTS('',3,(#28939,#28940,#28941,#28942,#28943,
#28944,#28945,#28946,#28947,#28948,#28949,#28950,#28951,#28952),
 .UNSPECIFIED.,.F.,.F.,(4,2,2,2,2,2,4),(-0.826160915626209,-0.625505883254,
-0.500256608389856,-0.412982803848779,-0.323646739244151,-0.187689231547272,
-2.22285427832525E-6),.UNSPECIFIED.);
#3076=B_SPLINE_CURVE_WITH_KNOTS('',3,(#28954,#28955,#28956,#28957,#28958,
#28959,#28960,#28961,#28962,#28963,#28964,#28965,#28966,#28967),
 .UNSPECIFIED.,.F.,.F.,(4,2,2,2,2,2,4),(-0.826003429306002,-0.625775328896998,
-0.500320591576485,-0.412898577035401,-0.32341507769936,-0.187267750996852,
-3.38394675953995E-6),.UNSPECIFIED.);
#3077=B_SPLINE_CURVE_WITH_KNOTS('',3,(#28968,#28969,#28970,#28971,#28972,
#28973,#28974,#28975,#28976,#28977,#28978,#28979,#28980,#28981),
 .UNSPECIFIED.,.F.,.F.,(4,2,2,2,2,2,4),(-0.826161221320018,-0.625505089589237,
-0.500256340926373,-0.412982969745037,-0.323647335030655,-0.187690296613032,
-2.21982746541616E-6),.UNSPECIFIED.);
#3078=B_SPLINE_CURVE_WITH_KNOTS('',3,(#28983,#28984,#28985,#28986,#28987,
#28988,#28989,#28990,#28991,#28992,#28993,#28994,#28995,#28996),
 .UNSPECIFIED.,.F.,.F.,(4,2,2,2,2,2,4),(-0.826003445592927,-0.625775272398046,
-0.500320569485795,-0.412898586055166,-0.323415117474739,-0.187267820464824,
-3.38376405458033E-6),.UNSPECIFIED.);
#3079=B_SPLINE_CURVE_WITH_KNOTS('',3,(#28997,#28998,#28999,#29000,#29001,
#29002,#29003,#29004,#29005,#29006,#29007,#29008,#29009,#29010),
 .UNSPECIFIED.,.F.,.F.,(4,2,2,2,2,2,4),(-0.826161044059661,-0.625505549780422,
-0.500256495972241,-0.412982873540227,-0.323646989578432,-0.187689678966569,
-2.22158898431419E-6),.UNSPECIFIED.);
#3080=B_SPLINE_CURVE_WITH_KNOTS('',3,(#29012,#29013,#29014,#29015,#29016,
#29017,#29018,#29019,#29020,#29021,#29022,#29023,#29024,#29025),
 .UNSPECIFIED.,.F.,.F.,(4,2,2,2,2,2,4),(-0.826160881882724,-0.62550597104126,
-0.500256638003748,-0.412982785530703,-0.323646673376656,-0.187689113795201,
-2.22318986310915E-6),.UNSPECIFIED.);
#3081=B_SPLINE_CURVE_WITH_KNOTS('',3,(#29026,#29027,#29028,#29029,#29030,
#29031,#29032,#29033,#29034,#29035,#29036,#29037,#29038,#29039),
 .UNSPECIFIED.,.F.,.F.,(4,2,2,2,2,2,4),(-0.826160858333095,-0.625506032805967,
-0.50025665888393,-0.412982772750447,-0.323646627202582,-0.187689031129653,
-2.22343578162597E-6),.UNSPECIFIED.);
#3082=B_SPLINE_CURVE_WITH_KNOTS('',3,(#29041,#29042,#29043,#29044,#29045,
#29046,#29047,#29048,#29049,#29050,#29051,#29052,#29053,#29054),
 .UNSPECIFIED.,.F.,.F.,(4,2,2,2,2,2,4),(-0.82600280426376,-0.625777500099417,
-0.500321440937581,-0.412898230912546,-0.323413549762581,-0.187265082618854,
-3.3909615432171E-6),.UNSPECIFIED.);
#3083=B_SPLINE_CURVE_WITH_KNOTS('',3,(#29055,#29056,#29057,#29058,#29059,
#29060,#29061,#29062,#29063,#29064,#29065,#29066,#29067,#29068),
 .UNSPECIFIED.,.F.,.F.,(4,2,2,2,2,2,4),(-0.826160856252331,-0.625506037746287,
-0.500256660510859,-0.412982771619331,-0.323646623338634,-0.187689024343634,
-2.22344480128072E-6),.UNSPECIFIED.);
#3084=B_SPLINE_CURVE_WITH_KNOTS('',3,(#29070,#29071,#29072,#29073,#29074,
#29075,#29076,#29077,#29078,#29079,#29080,#29081,#29082,#29083),
 .UNSPECIFIED.,.F.,.F.,(4,2,2,2,2,2,4),(-0.826003080122764,-0.625776541178574,
-0.500321065714738,-0.412898383680039,-0.323414224480335,-0.187266260903283,
-3.3878648413558E-6),.UNSPECIFIED.);
#3085=B_SPLINE_CURVE_WITH_KNOTS('',3,(#29084,#29085,#29086,#29087,#29088,
#29089,#29090,#29091,#29092,#29093,#29094,#29095,#29096,#29097),
 .UNSPECIFIED.,.F.,.F.,(4,2,2,2,2,2,4),(-0.826161034493358,-0.625505574643043,
-0.500256504354302,-0.412982868350074,-0.323646970925289,-0.187689645618028,
-2.2216840828131E-6),.UNSPECIFIED.);
#3086=B_SPLINE_CURVE_WITH_KNOTS('',3,(#29099,#29100,#29101,#29102,#29103,
#29104,#29105,#29106,#29107,#29108,#29109,#29110,#29111,#29112),
 .UNSPECIFIED.,.F.,.F.,(4,2,2,2,2,2,4),(-0.826003954437199,-0.62577350908337,
-0.500319880312736,-0.412898867793276,-0.32341635904328,-0.187269988970896,
-3.37805815897863E-6),.UNSPECIFIED.);
#3087=B_SPLINE_CURVE_WITH_KNOTS('',3,(#29113,#29114,#29115,#29116,#29117,
#29118,#29119,#29120,#29121,#29122,#29123,#29124,#29125,#29126),
 .UNSPECIFIED.,.F.,.F.,(4,2,2,2,2,2,4),(-0.826161235539218,-0.62550505270487,
-0.500256328505594,-0.412982977460568,-0.323647362721577,-0.187690346125095,
-2.21968621033823E-6),.UNSPECIFIED.);
#3088=B_SPLINE_CURVE_WITH_KNOTS('',3,(#29128,#29129,#29130,#29131,#29132,
#29133,#29134,#29135,#29136,#29137,#29138,#29139,#29140,#29141),
 .UNSPECIFIED.,.F.,.F.,(4,2,2,2,2,2,4),(-0.826160973205453,-0.625505733506315,
-0.500256557884447,-0.412982835101311,-0.323646851600755,-0.187689432412604,
-2.22228171405919E-6),.UNSPECIFIED.);
#3089=B_SPLINE_CURVE_WITH_KNOTS('',3,(#29142,#29143,#29144,#29145,#29146,
#29147,#29148,#29149,#29150,#29151,#29152,#29153,#29154,#29155),
 .UNSPECIFIED.,.F.,.F.,(4,2,2,2,2,2,4),(-0.826160921263198,-0.625505869052163,
-0.500256603636118,-0.412982806902687,-0.32364675003728,-0.187689250719983,
-2.222809903634E-6),.UNSPECIFIED.);
#3090=B_SPLINE_CURVE_WITH_KNOTS('',3,(#29157,#29158,#29159,#29160,#29161,
#29162,#29163,#29164,#29165,#29166,#29167,#29168,#29169,#29170),
 .UNSPECIFIED.,.F.,.F.,(4,2,2,2,2,2,4),(-0.826002804744918,-0.625777498402643,
-0.500321440269319,-0.412898231167257,-0.323413550925271,-0.187265084647106,
-3.39095613619537E-6),.UNSPECIFIED.);
#3091=B_SPLINE_CURVE_WITH_KNOTS('',3,(#29171,#29172,#29173,#29174,#29175,
#29176,#29177,#29178,#29179,#29180,#29181,#29182,#29183,#29184),
 .UNSPECIFIED.,.F.,.F.,(4,2,2,2,2,2,4),(-0.826160850943245,-0.625506051581447,
-0.500256665182958,-0.412982768745325,-0.32364661298202,-0.187689005830614,
-2.22349760923232E-6),.UNSPECIFIED.);
#3092=B_SPLINE_CURVE_WITH_KNOTS('',3,(#29186,#29187,#29188,#29189,#29190,
#29191,#29192,#29193,#29194,#29195,#29196,#29197,#29198,#29199),
 .UNSPECIFIED.,.F.,.F.,(4,2,2,2,2,2,4),(-0.826160879595277,-0.625505977003457,
-0.500256640017278,-0.412982784293015,-0.32364666891538,-0.187689105820326,
-2.22321261846373E-6),.UNSPECIFIED.);
#3093=B_SPLINE_CURVE_WITH_KNOTS('',3,(#29200,#29201,#29202,#29203,#29204,
#29205,#29206,#29207,#29208,#29209,#29210,#29211,#29212,#29213),
 .UNSPECIFIED.,.F.,.F.,(4,2,2,2,2,2,4),(-0.826160915642974,-0.625505883674515,
-0.500256608569079,-0.41298280385346,-0.323646739070228,-0.187689231114119,
-2.2228657925752E-6),.UNSPECIFIED.);
#3094=B_SPLINE_CURVE_WITH_KNOTS('',3,(#29215,#29216,#29217,#29218,#29219,
#29220,#29221,#29222,#29223,#29224,#29225,#29226,#29227,#29228),
 .UNSPECIFIED.,.F.,.F.,(4,2,2,2,2,2,4),(-0.826003429305969,-0.62577532888724,
-0.500320591570943,-0.412898577030623,-0.323415077693532,-0.187267750985861,
-3.38394675763227E-6),.UNSPECIFIED.);
#3095=B_SPLINE_CURVE_WITH_KNOTS('',3,(#29229,#29230,#29231,#29232,#29233,
#29234,#29235,#29236,#29237,#29238,#29239,#29240,#29241,#29242),
 .UNSPECIFIED.,.F.,.F.,(4,2,2,2,2,2,4),(-0.826161221319965,-0.62550508958843,
-0.500256340925903,-0.412982969744594,-0.323647335030077,-0.187690296611956,
-2.21982746525486E-6),.UNSPECIFIED.);
#3096=B_SPLINE_CURVE_WITH_KNOTS('',3,(#29244,#29245,#29246,#29247,#29248,
#29249,#29250,#29251,#29252,#29253,#29254,#29255,#29256,#29257),
 .UNSPECIFIED.,.F.,.F.,(4,2,2,2,2,2,4),(-0.826003445593229,-0.625775272394187,
-0.500320569483619,-0.41289858605328,-0.323415117472456,-0.187267820460476,
-3.38376405419045E-6),.UNSPECIFIED.);
#3097=B_SPLINE_CURVE_WITH_KNOTS('',3,(#29258,#29259,#29260,#29261,#29262,
#29263,#29264,#29265,#29266,#29267,#29268,#29269,#29270,#29271),
 .UNSPECIFIED.,.F.,.F.,(4,2,2,2,2,2,4),(-0.826161044059727,-0.625505549788039,
-0.500256495976546,-0.412982873543913,-0.32364698958292,-0.187689678975083,
-2.22158898273768E-6),.UNSPECIFIED.);
#3098=B_SPLINE_CURVE_WITH_KNOTS('',3,(#29273,#29274,#29275,#29276,#29277,
#29278,#29279,#29280,#29281,#29282,#29283,#29284,#29285,#29286),
 .UNSPECIFIED.,.F.,.F.,(4,2,2,2,2,2,4),(-0.826160881882804,-0.625505971051268,
-0.500256638009421,-0.412982785535515,-0.32364667338246,-0.187689113806309,
-2.2231898652661E-6),.UNSPECIFIED.);
#3099=B_SPLINE_CURVE_WITH_KNOTS('',3,(#29287,#29288,#29289,#29290,#29291,
#29292,#29293,#29294,#29295,#29296,#29297,#29298,#29299,#29300),
 .UNSPECIFIED.,.F.,.F.,(4,2,2,2,2,2,4),(-0.82616085833322,-0.625506032808248,
-0.500256658885217,-0.412982772751494,-0.323646627203788,-0.187689031131961,
-2.22343578221399E-6),.UNSPECIFIED.);
#3100=B_SPLINE_CURVE_WITH_KNOTS('',3,(#29302,#29303,#29304,#29305,#29306,
#29307,#29308,#29309,#29310,#29311,#29312,#29313,#29314,#29315),
 .UNSPECIFIED.,.F.,.F.,(4,2,2,2,2,2,4),(-0.826002804263561,-0.625777500092833,
-0.500321440933868,-0.412898230909481,-0.32341354975897,-0.187265082612001,
-3.39096154339912E-6),.UNSPECIFIED.);
#3101=B_SPLINE_CURVE_WITH_KNOTS('',3,(#29316,#29317,#29318,#29319,#29320,
#29321,#29322,#29323,#29324,#29325,#29326,#29327,#29328,#29329),
 .UNSPECIFIED.,.F.,.F.,(4,2,2,2,2,2,4),(-0.826002824122889,-0.625777431019925,
-0.500321413899708,-0.412898241904804,-0.323413598347589,-0.187265167461547,
-3.39073857045983E-6),.UNSPECIFIED.);
#3102=B_SPLINE_CURVE_WITH_KNOTS('',3,(#29331,#29332,#29333,#29334,#29335,
#29336,#29337,#29338,#29339,#29340,#29341,#29342,#29343,#29344),
 .UNSPECIFIED.,.F.,.F.,(4,2,2,2,2,2,4),(-0.826160968685895,-0.625505745254935,
-0.500256561845671,-0.412982832646704,-0.323646842781018,-0.187689416644658,
-2.22232665636257E-6),.UNSPECIFIED.);
#3103=B_SPLINE_CURVE_WITH_KNOTS('',3,(#29345,#29346,#29347,#29348,#29349,
#29350,#29351,#29352,#29353,#29354,#29355,#29356,#29357,#29358),
 .UNSPECIFIED.,.F.,.F.,(4,2,2,2,2,2,4),(-0.826003230622126,-0.625776018447498,
-0.500320861233349,-0.412898467008696,-0.323414592324213,-0.18726690330586,
-3.38617589407379E-6),.UNSPECIFIED.);
#3104=B_SPLINE_CURVE_WITH_KNOTS('',3,(#29375,#29376,#29377,#29378),
 .UNSPECIFIED.,.F.,.F.,(4,4),(-0.228509057368285,0.828509057368286),
 .UNSPECIFIED.);
#3105=B_SPLINE_CURVE_WITH_KNOTS('',3,(#29379,#29380,#29381,#29382),
 .UNSPECIFIED.,.F.,.F.,(4,4),(-0.228566601102733,0.828566601102733),
 .UNSPECIFIED.);
#3106=B_SPLINE_CURVE_WITH_KNOTS('',3,(#29399,#29400,#29401,#29402),
 .UNSPECIFIED.,.F.,.F.,(4,4),(-0.228509057368286,0.828509057368286),
 .UNSPECIFIED.);
#3107=B_SPLINE_CURVE_WITH_KNOTS('',3,(#29403,#29404,#29405,#29406),
 .UNSPECIFIED.,.F.,.F.,(4,4),(-0.228566601102733,0.828566601102733),
 .UNSPECIFIED.);
#3108=B_SPLINE_CURVE_WITH_KNOTS('',3,(#29423,#29424,#29425,#29426),
 .UNSPECIFIED.,.F.,.F.,(4,4),(-0.228509057368285,0.828509057368286),
 .UNSPECIFIED.);
#3109=B_SPLINE_CURVE_WITH_KNOTS('',3,(#29427,#29428,#29429,#29430),
 .UNSPECIFIED.,.F.,.F.,(4,4),(-0.228566601102733,0.828566601102733),
 .UNSPECIFIED.);
#3110=B_SPLINE_CURVE_WITH_KNOTS('',3,(#29447,#29448,#29449,#29450),
 .UNSPECIFIED.,.F.,.F.,(4,4),(-0.228509057368286,0.828509057368286),
 .UNSPECIFIED.);
#3111=B_SPLINE_CURVE_WITH_KNOTS('',3,(#29451,#29452,#29453,#29454),
 .UNSPECIFIED.,.F.,.F.,(4,4),(-0.228566601102733,0.828566601102733),
 .UNSPECIFIED.);
#3112=B_SPLINE_CURVE_WITH_KNOTS('',3,(#29471,#29472,#29473,#29474),
 .UNSPECIFIED.,.F.,.F.,(4,4),(-0.228509057368286,0.828509057368286),
 .UNSPECIFIED.);
#3113=B_SPLINE_CURVE_WITH_KNOTS('',3,(#29475,#29476,#29477,#29478),
 .UNSPECIFIED.,.F.,.F.,(4,4),(-0.228566601102733,0.828566601102733),
 .UNSPECIFIED.);
#3114=B_SPLINE_CURVE_WITH_KNOTS('',3,(#29495,#29496,#29497,#29498),
 .UNSPECIFIED.,.F.,.F.,(4,4),(-0.228509057368285,0.828509057368286),
 .UNSPECIFIED.);
#3115=B_SPLINE_CURVE_WITH_KNOTS('',3,(#29499,#29500,#29501,#29502),
 .UNSPECIFIED.,.F.,.F.,(4,4),(-0.228566601102733,0.828566601102733),
 .UNSPECIFIED.);
#3116=B_SPLINE_CURVE_WITH_KNOTS('',3,(#29519,#29520,#29521,#29522),
 .UNSPECIFIED.,.F.,.F.,(4,4),(-0.228509057368285,0.828509057368286),
 .UNSPECIFIED.);
#3117=B_SPLINE_CURVE_WITH_KNOTS('',3,(#29523,#29524,#29525,#29526),
 .UNSPECIFIED.,.F.,.F.,(4,4),(-0.228566601102733,0.828566601102733),
 .UNSPECIFIED.);
#3118=B_SPLINE_CURVE_WITH_KNOTS('',3,(#29543,#29544,#29545,#29546),
 .UNSPECIFIED.,.F.,.F.,(4,4),(-0.228509057368286,0.828509057368286),
 .UNSPECIFIED.);
#3119=B_SPLINE_CURVE_WITH_KNOTS('',3,(#29547,#29548,#29549,#29550),
 .UNSPECIFIED.,.F.,.F.,(4,4),(-0.228566601102733,0.828566601102733),
 .UNSPECIFIED.);
#3120=B_SPLINE_CURVE_WITH_KNOTS('',3,(#29567,#29568,#29569,#29570),
 .UNSPECIFIED.,.F.,.F.,(4,4),(-0.228509057368285,0.828509057368286),
 .UNSPECIFIED.);
#3121=B_SPLINE_CURVE_WITH_KNOTS('',3,(#29571,#29572,#29573,#29574),
 .UNSPECIFIED.,.F.,.F.,(4,4),(-0.228566601102733,0.828566601102733),
 .UNSPECIFIED.);
#3122=B_SPLINE_CURVE_WITH_KNOTS('',3,(#29591,#29592,#29593,#29594),
 .UNSPECIFIED.,.F.,.F.,(4,4),(-0.228509057368285,0.828509057368286),
 .UNSPECIFIED.);
#3123=B_SPLINE_CURVE_WITH_KNOTS('',3,(#29595,#29596,#29597,#29598),
 .UNSPECIFIED.,.F.,.F.,(4,4),(-0.228566601102733,0.828566601102733),
 .UNSPECIFIED.);
#3124=B_SPLINE_CURVE_WITH_KNOTS('',3,(#29615,#29616,#29617,#29618),
 .UNSPECIFIED.,.F.,.F.,(4,4),(-0.228509057368286,0.828509057368286),
 .UNSPECIFIED.);
#3125=B_SPLINE_CURVE_WITH_KNOTS('',3,(#29619,#29620,#29621,#29622),
 .UNSPECIFIED.,.F.,.F.,(4,4),(-0.228566601102733,0.828566601102733),
 .UNSPECIFIED.);
#3126=B_SPLINE_CURVE_WITH_KNOTS('',3,(#29639,#29640,#29641,#29642),
 .UNSPECIFIED.,.F.,.F.,(4,4),(-0.228509057368285,0.828509057368286),
 .UNSPECIFIED.);
#3127=B_SPLINE_CURVE_WITH_KNOTS('',3,(#29643,#29644,#29645,#29646),
 .UNSPECIFIED.,.F.,.F.,(4,4),(-0.228566601102733,0.828566601102733),
 .UNSPECIFIED.);
#3128=B_SPLINE_CURVE_WITH_KNOTS('',3,(#29663,#29664,#29665,#29666),
 .UNSPECIFIED.,.F.,.F.,(4,4),(-0.228509057368285,0.828509057368286),
 .UNSPECIFIED.);
#3129=B_SPLINE_CURVE_WITH_KNOTS('',3,(#29667,#29668,#29669,#29670),
 .UNSPECIFIED.,.F.,.F.,(4,4),(-0.228566601102734,0.828566601102734),
 .UNSPECIFIED.);
#3130=B_SPLINE_CURVE_WITH_KNOTS('',3,(#29687,#29688,#29689,#29690),
 .UNSPECIFIED.,.F.,.F.,(4,4),(-0.228509057368285,0.828509057368286),
 .UNSPECIFIED.);
#3131=B_SPLINE_CURVE_WITH_KNOTS('',3,(#29691,#29692,#29693,#29694),
 .UNSPECIFIED.,.F.,.F.,(4,4),(-0.228566601102733,0.828566601102733),
 .UNSPECIFIED.);
#3132=B_SPLINE_CURVE_WITH_KNOTS('',3,(#29711,#29712,#29713,#29714),
 .UNSPECIFIED.,.F.,.F.,(4,4),(-0.228509057368285,0.828509057368286),
 .UNSPECIFIED.);
#3133=B_SPLINE_CURVE_WITH_KNOTS('',3,(#29715,#29716,#29717,#29718),
 .UNSPECIFIED.,.F.,.F.,(4,4),(-0.228566601102733,0.828566601102733),
 .UNSPECIFIED.);
#3134=B_SPLINE_CURVE_WITH_KNOTS('',3,(#29735,#29736,#29737,#29738),
 .UNSPECIFIED.,.F.,.F.,(4,4),(-0.228509057368285,0.828509057368286),
 .UNSPECIFIED.);
#3135=B_SPLINE_CURVE_WITH_KNOTS('',3,(#29739,#29740,#29741,#29742),
 .UNSPECIFIED.,.F.,.F.,(4,4),(-0.228566601102733,0.828566601102733),
 .UNSPECIFIED.);
#3136=B_SPLINE_CURVE_WITH_KNOTS('',3,(#29759,#29760,#29761,#29762),
 .UNSPECIFIED.,.F.,.F.,(4,4),(-0.228509057368285,0.828509057368286),
 .UNSPECIFIED.);
#3137=B_SPLINE_CURVE_WITH_KNOTS('',3,(#29763,#29764,#29765,#29766),
 .UNSPECIFIED.,.F.,.F.,(4,4),(-0.228566601102733,0.828566601102733),
 .UNSPECIFIED.);
#3138=B_SPLINE_CURVE_WITH_KNOTS('',3,(#29783,#29784,#29785,#29786),
 .UNSPECIFIED.,.F.,.F.,(4,4),(-0.228509057368285,0.828509057368286),
 .UNSPECIFIED.);
#3139=B_SPLINE_CURVE_WITH_KNOTS('',3,(#29787,#29788,#29789,#29790),
 .UNSPECIFIED.,.F.,.F.,(4,4),(-0.228566601102733,0.828566601102733),
 .UNSPECIFIED.);
#3140=B_SPLINE_CURVE_WITH_KNOTS('',3,(#29819,#29820,#29821,#29822),
 .UNSPECIFIED.,.F.,.F.,(4,4),(-0.228509057368286,0.828509057368286),
 .UNSPECIFIED.);
#3141=B_SPLINE_CURVE_WITH_KNOTS('',3,(#29907,#29908,#29909,#29910),
 .UNSPECIFIED.,.F.,.F.,(4,4),(-0.228509057368286,0.828509057368286),
 .UNSPECIFIED.);
#3142=B_SPLINE_CURVE_WITH_KNOTS('',3,(#29999,#30000,#30001,#30002),
 .UNSPECIFIED.,.F.,.F.,(4,4),(-0.228509057368285,0.828509057368286),
 .UNSPECIFIED.);
#3143=B_SPLINE_CURVE_WITH_KNOTS('',3,(#30091,#30092,#30093,#30094),
 .UNSPECIFIED.,.F.,.F.,(4,4),(-0.228509057368286,0.828509057368286),
 .UNSPECIFIED.);
#3144=B_SPLINE_CURVE_WITH_KNOTS('',3,(#30183,#30184,#30185,#30186),
 .UNSPECIFIED.,.F.,.F.,(4,4),(-0.228509057368286,0.828509057368286),
 .UNSPECIFIED.);
#3145=B_SPLINE_CURVE_WITH_KNOTS('',3,(#30279,#30280,#30281,#30282),
 .UNSPECIFIED.,.F.,.F.,(4,4),(-0.228509057368287,0.828509057368287),
 .UNSPECIFIED.);
#3146=B_SPLINE_CURVE_WITH_KNOTS('',3,(#30371,#30372,#30373,#30374),
 .UNSPECIFIED.,.F.,.F.,(4,4),(-0.228509057368286,0.828509057368286),
 .UNSPECIFIED.);
#3147=B_SPLINE_CURVE_WITH_KNOTS('',3,(#30467,#30468,#30469,#30470),
 .UNSPECIFIED.,.F.,.F.,(4,4),(-0.228509057368286,0.828509057368286),
 .UNSPECIFIED.);
#3148=B_SPLINE_CURVE_WITH_KNOTS('',3,(#30559,#30560,#30561,#30562),
 .UNSPECIFIED.,.F.,.F.,(4,4),(-0.228509057368286,0.828509057368286),
 .UNSPECIFIED.);
#3149=B_SPLINE_CURVE_WITH_KNOTS('',3,(#30651,#30652,#30653,#30654),
 .UNSPECIFIED.,.F.,.F.,(4,4),(-0.228509057368286,0.828509057368287),
 .UNSPECIFIED.);
#3150=B_SPLINE_CURVE_WITH_KNOTS('',3,(#30743,#30744,#30745,#30746),
 .UNSPECIFIED.,.F.,.F.,(4,4),(-0.228509057368286,0.828509057368286),
 .UNSPECIFIED.);
#3151=B_SPLINE_CURVE_WITH_KNOTS('',3,(#30839,#30840,#30841,#30842),
 .UNSPECIFIED.,.F.,.F.,(4,4),(-0.228509057368285,0.828509057368286),
 .UNSPECIFIED.);
#3152=B_SPLINE_CURVE_WITH_KNOTS('',3,(#30931,#30932,#30933,#30934),
 .UNSPECIFIED.,.F.,.F.,(4,4),(-0.228509057368286,0.828509057368286),
 .UNSPECIFIED.);
#3153=B_SPLINE_CURVE_WITH_KNOTS('',3,(#31023,#31024,#31025,#31026),
 .UNSPECIFIED.,.F.,.F.,(4,4),(-0.228509057368286,0.828509057368286),
 .UNSPECIFIED.);
#3154=B_SPLINE_CURVE_WITH_KNOTS('',3,(#31119,#31120,#31121,#31122),
 .UNSPECIFIED.,.F.,.F.,(4,4),(-0.228509057368286,0.828509057368286),
 .UNSPECIFIED.);
#3155=B_SPLINE_CURVE_WITH_KNOTS('',3,(#31211,#31212,#31213,#31214),
 .UNSPECIFIED.,.F.,.F.,(4,4),(-0.228509057368286,0.828509057368287),
 .UNSPECIFIED.);
#3156=B_SPLINE_CURVE_WITH_KNOTS('',3,(#31307,#31308,#31309,#31310),
 .UNSPECIFIED.,.F.,.F.,(4,4),(-0.228509057368286,0.828509057368286),
 .UNSPECIFIED.);
#3157=B_SPLINE_CURVE_WITH_KNOTS('',3,(#31399,#31400,#31401,#31402),
 .UNSPECIFIED.,.F.,.F.,(4,4),(-0.228509057368285,0.828509057368286),
 .UNSPECIFIED.);
#3158=B_SPLINE_CURVE_WITH_KNOTS('',3,(#31481,#31482,#31483,#31484,#31485,
#31486,#31487,#31488,#31489,#31490,#31491,#31492,#31493),.UNSPECIFIED.,
 .F.,.F.,(4,3,3,3,4),(-0.301665508889116,0.,0.301549467956627,0.603098935913254,
0.904721008425295),.UNSPECIFIED.);
#3159=B_SPLINE_CURVE_WITH_KNOTS('',3,(#31510,#31511,#31512,#31513),
 .UNSPECIFIED.,.F.,.F.,(4,4),(-0.228566601102733,0.828566601102733),
 .UNSPECIFIED.);
#3160=B_SPLINE_CURVE_WITH_KNOTS('',3,(#31531,#31532,#31533,#31534,#31535,
#31536,#31537,#31538,#31539,#31540,#31541,#31542,#31543),.UNSPECIFIED.,
 .F.,.F.,(4,3,3,3,4),(-0.301622072512042,0.,0.301549467956626,0.603098935913254,
0.90476444480237),.UNSPECIFIED.);
#3161=B_SPLINE_CURVE_WITH_KNOTS('',3,(#31548,#31549,#31550,#31551,#31552,
#31553,#31554,#31555,#31556,#31557,#31558,#31559,#31560),.UNSPECIFIED.,
 .F.,.F.,(4,3,3,3,4),(-0.301622072512042,0.,0.301549467956627,0.603098935913254,
0.904764444802371),.UNSPECIFIED.);
#3162=B_SPLINE_CURVE_WITH_KNOTS('',3,(#31563,#31564,#31565,#31566,#31567,
#31568,#31569,#31570,#31571,#31572,#31573,#31574,#31575),.UNSPECIFIED.,
 .F.,.F.,(4,3,3,3,4),(-0.301665508889117,0.,0.301549467956628,0.603098935913255,
0.904721008425297),.UNSPECIFIED.);
#3163=B_SPLINE_CURVE_WITH_KNOTS('',3,(#31594,#31595,#31596,#31597,#31598,
#31599,#31600,#31601,#31602,#31603,#31604,#31605,#31606),.UNSPECIFIED.,
 .F.,.F.,(4,3,3,3,4),(-0.301622072512041,0.,0.301549467956627,0.603098935913255,
0.904764444802372),.UNSPECIFIED.);
#3164=B_SPLINE_CURVE_WITH_KNOTS('',3,(#31608,#31609,#31610,#31611),
 .UNSPECIFIED.,.F.,.F.,(4,4),(-0.228566601102733,0.828566601102733),
 .UNSPECIFIED.);
#3165=B_SPLINE_CURVE_WITH_KNOTS('',3,(#31663,#31664,#31665,#31666,#31667,
#31668,#31669,#31670,#31671,#31672,#31673,#31674,#31675),.UNSPECIFIED.,
 .F.,.F.,(4,3,3,3,4),(-0.301665508889116,0.,0.301549467956627,0.603098935913254,
0.904721008425296),.UNSPECIFIED.);
#3166=B_SPLINE_CURVE_WITH_KNOTS('',3,(#31693,#31694,#31695,#31696,#31697,
#31698,#31699,#31700,#31701,#31702,#31703,#31704,#31705),.UNSPECIFIED.,
 .F.,.F.,(4,3,3,3,4),(-0.301622072512042,0.,0.301549467956626,0.603098935913253,
0.90476444480237),.UNSPECIFIED.);
#3167=B_SPLINE_CURVE_WITH_KNOTS('',3,(#31707,#31708,#31709,#31710),
 .UNSPECIFIED.,.F.,.F.,(4,4),(-0.228566601102733,0.828566601102733),
 .UNSPECIFIED.);
#3168=B_SPLINE_CURVE_WITH_KNOTS('',3,(#31804,#31805,#31806,#31807,#31808,
#31809,#31810,#31811,#31812,#31813,#31814,#31815,#31816),.UNSPECIFIED.,
 .F.,.F.,(4,3,3,3,4),(-0.301665508889116,0.,0.301549467956627,0.603098935913254,
0.904721008425295),.UNSPECIFIED.);
#3169=B_SPLINE_CURVE_WITH_KNOTS('',3,(#31849,#31850,#31851,#31852),
 .UNSPECIFIED.,.F.,.F.,(4,4),(-0.228566601102733,0.828566601102733),
 .UNSPECIFIED.);
#3170=B_SPLINE_CURVE_WITH_KNOTS('',3,(#31869,#31870,#31871,#31872,#31873,
#31874,#31875,#31876,#31877,#31878,#31879,#31880,#31881),.UNSPECIFIED.,
 .F.,.F.,(4,3,3,3,4),(-0.301622072512042,0.,0.301549467956627,0.603098935913254,
0.90476444480237),.UNSPECIFIED.);
#3171=B_SPLINE_CURVE_WITH_KNOTS('',3,(#31884,#31885,#31886,#31887,#31888,
#31889,#31890,#31891,#31892,#31893,#31894,#31895,#31896),.UNSPECIFIED.,
 .F.,.F.,(4,3,3,3,4),(-0.301665508889116,0.,0.301549467956627,0.603098935913254,
0.904721008425296),.UNSPECIFIED.);
#3172=B_SPLINE_CURVE_WITH_KNOTS('',3,(#31913,#31914,#31915,#31916,#31917,
#31918,#31919,#31920,#31921,#31922,#31923,#31924,#31925),.UNSPECIFIED.,
 .F.,.F.,(4,3,3,3,4),(-0.301622072512042,0.,0.301549467956627,0.603098935913254,
0.90476444480237),.UNSPECIFIED.);
#3173=B_SPLINE_CURVE_WITH_KNOTS('',3,(#31926,#31927,#31928,#31929),
 .UNSPECIFIED.,.F.,.F.,(4,4),(-0.228566601102733,0.828566601102733),
 .UNSPECIFIED.);
#3174=B_SPLINE_CURVE_WITH_KNOTS('',3,(#31978,#31979,#31980,#31981,#31982,
#31983,#31984,#31985,#31986,#31987,#31988,#31989,#31990),.UNSPECIFIED.,
 .F.,.F.,(4,3,3,3,4),(-0.301665508889117,0.,0.301549467956627,0.603098935913253,
0.904721008425295),.UNSPECIFIED.);
#3175=B_SPLINE_CURVE_WITH_KNOTS('',3,(#32007,#32008,#32009,#32010,#32011,
#32012,#32013,#32014,#32015,#32016,#32017,#32018,#32019),.UNSPECIFIED.,
 .F.,.F.,(4,3,3,3,4),(-0.301622072512042,0.,0.301549467956627,0.603098935913255,
0.904764444802371),.UNSPECIFIED.);
#3176=B_SPLINE_CURVE_WITH_KNOTS('',3,(#32020,#32021,#32022,#32023),
 .UNSPECIFIED.,.F.,.F.,(4,4),(-0.228566601102733,0.828566601102733),
 .UNSPECIFIED.);
#3177=B_SPLINE_CURVE_WITH_KNOTS('',3,(#32041,#32042,#32043,#32044,#32045,
#32046,#32047,#32048,#32049,#32050,#32051,#32052,#32053),.UNSPECIFIED.,
 .F.,.F.,(4,3,3,3,4),(-0.301665508889116,0.,0.301549467956625,0.603098935913253,
0.904721008425295),.UNSPECIFIED.);
#3178=B_SPLINE_CURVE_WITH_KNOTS('',3,(#32086,#32087,#32088,#32089),
 .UNSPECIFIED.,.F.,.F.,(4,4),(-0.228566601102733,0.828566601102734),
 .UNSPECIFIED.);
#3179=B_SPLINE_CURVE_WITH_KNOTS('',3,(#32106,#32107,#32108,#32109,#32110,
#32111,#32112,#32113,#32114,#32115,#32116,#32117,#32118),.UNSPECIFIED.,
 .F.,.F.,(4,3,3,3,4),(-0.301622072512042,0.,0.301549467956624,0.603098935913253,
0.90476444480237),.UNSPECIFIED.);
#3180=B_SPLINE_CURVE_WITH_KNOTS('',3,(#32121,#32122,#32123,#32124,#32125,
#32126,#32127,#32128,#32129,#32130,#32131,#32132,#32133),.UNSPECIFIED.,
 .F.,.F.,(4,3,3,3,4),(-0.301665508889116,0.,0.301549467956627,0.603098935913255,
0.904721008425296),.UNSPECIFIED.);
#3181=B_SPLINE_CURVE_WITH_KNOTS('',3,(#32150,#32151,#32152,#32153,#32154,
#32155,#32156,#32157,#32158,#32159,#32160,#32161,#32162),.UNSPECIFIED.,
 .F.,.F.,(4,3,3,3,4),(-0.301622072512042,0.,0.301549467956627,0.603098935913254,
0.904764444802371),.UNSPECIFIED.);
#3182=B_SPLINE_CURVE_WITH_KNOTS('',3,(#32163,#32164,#32165,#32166),
 .UNSPECIFIED.,.F.,.F.,(4,4),(-0.228566601102733,0.828566601102733),
 .UNSPECIFIED.);
#3183=B_SPLINE_CURVE_WITH_KNOTS('',3,(#32215,#32216,#32217,#32218,#32219,
#32220,#32221,#32222,#32223,#32224,#32225,#32226,#32227),.UNSPECIFIED.,
 .F.,.F.,(4,3,3,3,4),(-0.301665508889116,0.,0.301549467956627,0.603098935913254,
0.904721008425295),.UNSPECIFIED.);
#3184=B_SPLINE_CURVE_WITH_KNOTS('',3,(#32244,#32245,#32246,#32247,#32248,
#32249,#32250,#32251,#32252,#32253,#32254,#32255,#32256),.UNSPECIFIED.,
 .F.,.F.,(4,3,3,3,4),(-0.301622072512041,0.,0.301549467956627,0.603098935913254,
0.904764444802371),.UNSPECIFIED.);
#3185=B_SPLINE_CURVE_WITH_KNOTS('',3,(#32257,#32258,#32259,#32260),
 .UNSPECIFIED.,.F.,.F.,(4,4),(-0.228566601102733,0.828566601102734),
 .UNSPECIFIED.);
#3186=B_SPLINE_CURVE_WITH_KNOTS('',3,(#32278,#32279,#32280,#32281,#32282,
#32283,#32284,#32285,#32286,#32287,#32288,#32289,#32290),.UNSPECIFIED.,
 .F.,.F.,(4,3,3,3,4),(-0.301665508889116,0.,0.301549467956629,0.603098935913255,
0.904721008425297),.UNSPECIFIED.);
#3187=B_SPLINE_CURVE_WITH_KNOTS('',3,(#32323,#32324,#32325,#32326),
 .UNSPECIFIED.,.F.,.F.,(4,4),(-0.228566601102733,0.828566601102733),
 .UNSPECIFIED.);
#3188=B_SPLINE_CURVE_WITH_KNOTS('',3,(#32343,#32344,#32345,#32346,#32347,
#32348,#32349,#32350,#32351,#32352,#32353,#32354,#32355),.UNSPECIFIED.,
 .F.,.F.,(4,3,3,3,4),(-0.301622072512042,0.,0.301549467956625,0.603098935913252,
0.904764444802369),.UNSPECIFIED.);
#3189=B_SPLINE_CURVE_WITH_KNOTS('',3,(#32358,#32359,#32360,#32361,#32362,
#32363,#32364,#32365,#32366,#32367,#32368,#32369,#32370),.UNSPECIFIED.,
 .F.,.F.,(4,3,3,3,4),(-0.301665508889116,0.,0.301549467956628,0.603098935913255,
0.904721008425296),.UNSPECIFIED.);
#3190=B_SPLINE_CURVE_WITH_KNOTS('',3,(#32387,#32388,#32389,#32390,#32391,
#32392,#32393,#32394,#32395,#32396,#32397,#32398,#32399),.UNSPECIFIED.,
 .F.,.F.,(4,3,3,3,4),(-0.301622072512042,0.,0.301549467956627,0.603098935913253,
0.90476444480237),.UNSPECIFIED.);
#3191=B_SPLINE_CURVE_WITH_KNOTS('',3,(#32400,#32401,#32402,#32403),
 .UNSPECIFIED.,.F.,.F.,(4,4),(-0.228566601102733,0.828566601102734),
 .UNSPECIFIED.);
#3192=B_SPLINE_CURVE_WITH_KNOTS('',3,(#32452,#32453,#32454,#32455,#32456,
#32457,#32458,#32459,#32460,#32461,#32462,#32463,#32464),.UNSPECIFIED.,
 .F.,.F.,(4,3,3,3,4),(-0.301665508889116,0.,0.301549467956626,0.603098935913255,
0.904721008425298),.UNSPECIFIED.);
#3193=B_SPLINE_CURVE_WITH_KNOTS('',3,(#32481,#32482,#32483,#32484,#32485,
#32486,#32487,#32488,#32489,#32490,#32491,#32492,#32493),.UNSPECIFIED.,
 .F.,.F.,(4,3,3,3,4),(-0.301622072512042,0.,0.301549467956627,0.603098935913252,
0.904764444802368),.UNSPECIFIED.);
#3194=B_SPLINE_CURVE_WITH_KNOTS('',3,(#32494,#32495,#32496,#32497),
 .UNSPECIFIED.,.F.,.F.,(4,4),(-0.228566601102733,0.828566601102733),
 .UNSPECIFIED.);
#3195=B_SPLINE_CURVE_WITH_KNOTS('',3,(#32515,#32516,#32517,#32518,#32519,
#32520,#32521,#32522,#32523,#32524,#32525,#32526,#32527),.UNSPECIFIED.,
 .F.,.F.,(4,3,3,3,4),(-0.301665508889117,0.,0.301549467956627,0.603098935913254,
0.904721008425296),.UNSPECIFIED.);
#3196=B_SPLINE_CURVE_WITH_KNOTS('',3,(#32560,#32561,#32562,#32563),
 .UNSPECIFIED.,.F.,.F.,(4,4),(-0.228566601102733,0.828566601102733),
 .UNSPECIFIED.);
#3197=B_SPLINE_CURVE_WITH_KNOTS('',3,(#32580,#32581,#32582,#32583,#32584,
#32585,#32586,#32587,#32588,#32589,#32590,#32591,#32592),.UNSPECIFIED.,
 .F.,.F.,(4,3,3,3,4),(-0.301622072512042,0.,0.301549467956627,0.603098935913254,
0.90476444480237),.UNSPECIFIED.);
#3198=B_SPLINE_CURVE_WITH_KNOTS('',3,(#32595,#32596,#32597,#32598,#32599,
#32600,#32601,#32602,#32603,#32604,#32605,#32606,#32607),.UNSPECIFIED.,
 .F.,.F.,(4,3,3,3,4),(-0.301665508889116,0.,0.301549467956627,0.603098935913254,
0.904721008425295),.UNSPECIFIED.);
#3199=B_SPLINE_CURVE_WITH_KNOTS('',3,(#32624,#32625,#32626,#32627,#32628,
#32629,#32630,#32631,#32632,#32633,#32634,#32635,#32636),.UNSPECIFIED.,
 .F.,.F.,(4,3,3,3,4),(-0.301622072512042,0.,0.301549467956627,0.603098935913254,
0.904764444802371),.UNSPECIFIED.);
#3200=B_SPLINE_CURVE_WITH_KNOTS('',3,(#32637,#32638,#32639,#32640),
 .UNSPECIFIED.,.F.,.F.,(4,4),(-0.228566601102733,0.828566601102733),
 .UNSPECIFIED.);
#3201=B_SPLINE_CURVE_WITH_KNOTS('',3,(#32689,#32690,#32691,#32692,#32693,
#32694,#32695,#32696,#32697,#32698,#32699,#32700,#32701),.UNSPECIFIED.,
 .F.,.F.,(4,3,3,3,4),(-0.301665508889117,0.,0.301549467956628,0.603098935913255,
0.904721008425296),.UNSPECIFIED.);
#3202=B_SPLINE_CURVE_WITH_KNOTS('',3,(#32718,#32719,#32720,#32721,#32722,
#32723,#32724,#32725,#32726,#32727,#32728,#32729,#32730),.UNSPECIFIED.,
 .F.,.F.,(4,3,3,3,4),(-0.301622072512041,0.,0.301549467956627,0.603098935913255,
0.904764444802371),.UNSPECIFIED.);
#3203=B_SPLINE_CURVE_WITH_KNOTS('',3,(#32731,#32732,#32733,#32734),
 .UNSPECIFIED.,.F.,.F.,(4,4),(-0.228566601102733,0.828566601102733),
 .UNSPECIFIED.);
#3204=B_SPLINE_CURVE_WITH_KNOTS('',3,(#32752,#32753,#32754,#32755,#32756,
#32757,#32758,#32759,#32760,#32761,#32762,#32763,#32764),.UNSPECIFIED.,
 .F.,.F.,(4,3,3,3,4),(-0.301665508889117,0.,0.301549467956625,0.603098935913254,
0.904721008425296),.UNSPECIFIED.);
#3205=B_SPLINE_CURVE_WITH_KNOTS('',3,(#32797,#32798,#32799,#32800),
 .UNSPECIFIED.,.F.,.F.,(4,4),(-0.228566601102733,0.828566601102733),
 .UNSPECIFIED.);
#3206=B_SPLINE_CURVE_WITH_KNOTS('',3,(#32817,#32818,#32819,#32820,#32821,
#32822,#32823,#32824,#32825,#32826,#32827,#32828,#32829),.UNSPECIFIED.,
 .F.,.F.,(4,3,3,3,4),(-0.301622072512042,0.,0.301549467956625,0.603098935913253,
0.90476444480237),.UNSPECIFIED.);
#3207=B_SPLINE_CURVE_WITH_KNOTS('',3,(#32832,#32833,#32834,#32835,#32836,
#32837,#32838,#32839,#32840,#32841,#32842,#32843,#32844),.UNSPECIFIED.,
 .F.,.F.,(4,3,3,3,4),(-0.301665508889116,0.,0.301549467956627,0.603098935913254,
0.904721008425295),.UNSPECIFIED.);
#3208=B_SPLINE_CURVE_WITH_KNOTS('',3,(#32861,#32862,#32863,#32864,#32865,
#32866,#32867,#32868,#32869,#32870,#32871,#32872,#32873),.UNSPECIFIED.,
 .F.,.F.,(4,3,3,3,4),(-0.301622072512042,0.,0.301549467956627,0.603098935913254,
0.90476444480237),.UNSPECIFIED.);
#3209=B_SPLINE_CURVE_WITH_KNOTS('',3,(#32874,#32875,#32876,#32877),
 .UNSPECIFIED.,.F.,.F.,(4,4),(-0.228566601102733,0.828566601102733),
 .UNSPECIFIED.);
#3210=B_SPLINE_CURVE_WITH_KNOTS('',3,(#32926,#32927,#32928,#32929,#32930,
#32931,#32932,#32933,#32934,#32935,#32936,#32937,#32938),.UNSPECIFIED.,
 .F.,.F.,(4,3,3,3,4),(-0.301665508889116,0.,0.301549467956627,0.603098935913253,
0.904721008425295),.UNSPECIFIED.);
#3211=B_SPLINE_CURVE_WITH_KNOTS('',3,(#32955,#32956,#32957,#32958),
 .UNSPECIFIED.,.F.,.F.,(4,4),(-0.228566601102733,0.828566601102733),
 .UNSPECIFIED.);
#3675=LINE('',#17358,#4145);
#3676=LINE('',#17382,#4146);
#3677=LINE('',#17752,#4147);
#3678=LINE('',#18130,#4148);
#3679=LINE('',#18586,#4149);
#3680=LINE('',#18970,#4150);
#3681=LINE('',#19422,#4151);
#3682=LINE('',#19806,#4152);
#3683=LINE('',#20104,#4153);
#3684=LINE('',#20396,#4154);
#3685=LINE('',#20692,#4155);
#3686=LINE('',#20989,#4156);
#3687=LINE('',#21186,#4157);
#3688=LINE('',#21289,#4158);
#3689=LINE('',#21481,#4159);
#3690=LINE('',#21773,#4160);
#3691=LINE('',#22068,#4161);
#3692=LINE('',#22363,#4162);
#3693=LINE('',#22659,#4163);
#3694=LINE('',#23075,#4164);
#3695=LINE('',#23264,#4165);
#3696=LINE('',#23678,#4166);
#3697=LINE('',#23979,#4167);
#3698=LINE('',#24393,#4168);
#3699=LINE('',#26899,#4169);
#3700=LINE('',#26903,#4170);
#3701=LINE('',#26907,#4171);
#3702=LINE('',#26911,#4172);
#3703=LINE('',#26915,#4173);
#3704=LINE('',#26919,#4174);
#3705=LINE('',#26923,#4175);
#3706=LINE('',#26927,#4176);
#3707=LINE('',#26931,#4177);
#3708=LINE('',#26935,#4178);
#3709=LINE('',#26939,#4179);
#3710=LINE('',#26943,#4180);
#3711=LINE('',#26947,#4181);
#3712=LINE('',#26951,#4182);
#3713=LINE('',#26955,#4183);
#3714=LINE('',#26959,#4184);
#3715=LINE('',#26963,#4185);
#3716=LINE('',#26967,#4186);
#3717=LINE('',#26971,#4187);
#3718=LINE('',#26975,#4188);
#3719=LINE('',#26979,#4189);
#3720=LINE('',#26983,#4190);
#3721=LINE('',#26987,#4191);
#3722=LINE('',#26991,#4192);
#3723=LINE('',#26995,#4193);
#3724=LINE('',#26999,#4194);
#3725=LINE('',#27003,#4195);
#3726=LINE('',#27007,#4196);
#3727=LINE('',#27011,#4197);
#3728=LINE('',#27015,#4198);
#3729=LINE('',#27019,#4199);
#3730=LINE('',#27023,#4200);
#3731=LINE('',#27027,#4201);
#3732=LINE('',#27031,#4202);
#3733=LINE('',#27035,#4203);
#3734=LINE('',#27038,#4204);
#3735=LINE('',#27042,#4205);
#3736=LINE('',#27046,#4206);
#3737=LINE('',#27051,#4207);
#3738=LINE('',#27055,#4208);
#3739=LINE('',#27060,#4209);
#3740=LINE('',#27064,#4210);
#3741=LINE('',#27069,#4211);
#3742=LINE('',#27073,#4212);
#3743=LINE('',#27078,#4213);
#3744=LINE('',#27082,#4214);
#3745=LINE('',#27087,#4215);
#3746=LINE('',#27091,#4216);
#3747=LINE('',#27096,#4217);
#3748=LINE('',#27100,#4218);
#3749=LINE('',#27105,#4219);
#3750=LINE('',#27109,#4220);
#3751=LINE('',#27114,#4221);
#3752=LINE('',#27118,#4222);
#3753=LINE('',#27123,#4223);
#3754=LINE('',#27127,#4224);
#3755=LINE('',#27132,#4225);
#3756=LINE('',#27136,#4226);
#3757=LINE('',#27141,#4227);
#3758=LINE('',#27145,#4228);
#3759=LINE('',#27150,#4229);
#3760=LINE('',#27154,#4230);
#3761=LINE('',#27159,#4231);
#3762=LINE('',#27163,#4232);
#3763=LINE('',#27168,#4233);
#3764=LINE('',#27172,#4234);
#3765=LINE('',#27177,#4235);
#3766=LINE('',#27181,#4236);
#3767=LINE('',#27186,#4237);
#3768=LINE('',#27190,#4238);
#3769=LINE('',#27195,#4239);
#3770=LINE('',#27199,#4240);
#3771=LINE('',#27207,#4241);
#3772=LINE('',#27227,#4242);
#3773=LINE('',#27234,#4243);
#3774=LINE('',#27254,#4244);
#3775=LINE('',#27261,#4245);
#3776=LINE('',#27279,#4246);
#3777=LINE('',#27286,#4247);
#3778=LINE('',#27306,#4248);
#3779=LINE('',#27313,#4249);
#3780=LINE('',#27333,#4250);
#3781=LINE('',#27340,#4251);
#3782=LINE('',#27360,#4252);
#3783=LINE('',#27367,#4253);
#3784=LINE('',#27385,#4254);
#3785=LINE('',#27392,#4255);
#3786=LINE('',#27412,#4256);
#3787=LINE('',#27419,#4257);
#3788=LINE('',#27439,#4258);
#3789=LINE('',#27446,#4259);
#3790=LINE('',#27466,#4260);
#3791=LINE('',#27473,#4261);
#3792=LINE('',#27491,#4262);
#3793=LINE('',#27498,#4263);
#3794=LINE('',#27518,#4264);
#3795=LINE('',#27525,#4265);
#3796=LINE('',#27545,#4266);
#3797=LINE('',#27552,#4267);
#3798=LINE('',#27572,#4268);
#3799=LINE('',#27579,#4269);
#3800=LINE('',#27599,#4270);
#3801=LINE('',#27606,#4271);
#3802=LINE('',#27626,#4272);
#3803=LINE('',#27633,#4273);
#3804=LINE('',#27653,#4274);
#3805=LINE('',#27660,#4275);
#3806=LINE('',#27680,#4276);
#3807=LINE('',#27690,#4277);
#3808=LINE('',#27713,#4278);
#3809=LINE('',#27723,#4279);
#3810=LINE('',#27746,#4280);
#3811=LINE('',#27756,#4281);
#3812=LINE('',#27781,#4282);
#3813=LINE('',#27791,#4283);
#3814=LINE('',#27812,#4284);
#3815=LINE('',#27822,#4285);
#3816=LINE('',#27847,#4286);
#3817=LINE('',#27857,#4287);
#3818=LINE('',#27882,#4288);
#3819=LINE('',#27892,#4289);
#3820=LINE('',#27915,#4290);
#3821=LINE('',#27925,#4291);
#3822=LINE('',#27948,#4292);
#3823=LINE('',#27958,#4293);
#3824=LINE('',#27983,#4294);
#3825=LINE('',#27993,#4295);
#3826=LINE('',#28018,#4296);
#3827=LINE('',#28028,#4297);
#3828=LINE('',#28051,#4298);
#3829=LINE('',#28061,#4299);
#3830=LINE('',#28084,#4300);
#3831=LINE('',#28094,#4301);
#3832=LINE('',#28117,#4302);
#3833=LINE('',#28127,#4303);
#3834=LINE('',#28152,#4304);
#3835=LINE('',#28162,#4305);
#3836=LINE('',#28187,#4306);
#3837=LINE('',#28197,#4307);
#3838=LINE('',#28220,#4308);
#3839=LINE('',#28230,#4309);
#3840=LINE('',#28253,#4310);
#3841=LINE('',#28263,#4311);
#3842=LINE('',#28284,#4312);
#3843=LINE('',#28287,#4313);
#3844=LINE('',#28289,#4314);
#3845=LINE('',#28293,#4315);
#3846=LINE('',#28295,#4316);
#3847=LINE('',#28299,#4317);
#3848=LINE('',#28301,#4318);
#3849=LINE('',#28305,#4319);
#3850=LINE('',#28307,#4320);
#3851=LINE('',#28311,#4321);
#3852=LINE('',#28313,#4322);
#3853=LINE('',#28317,#4323);
#3854=LINE('',#28319,#4324);
#3855=LINE('',#28323,#4325);
#3856=LINE('',#28325,#4326);
#3857=LINE('',#28329,#4327);
#3858=LINE('',#28331,#4328);
#3859=LINE('',#28335,#4329);
#3860=LINE('',#28337,#4330);
#3861=LINE('',#28341,#4331);
#3862=LINE('',#28343,#4332);
#3863=LINE('',#28347,#4333);
#3864=LINE('',#28349,#4334);
#3865=LINE('',#28353,#4335);
#3866=LINE('',#28355,#4336);
#3867=LINE('',#28359,#4337);
#3868=LINE('',#28361,#4338);
#3869=LINE('',#28365,#4339);
#3870=LINE('',#28367,#4340);
#3871=LINE('',#28371,#4341);
#3872=LINE('',#28373,#4342);
#3873=LINE('',#28377,#4343);
#3874=LINE('',#28379,#4344);
#3875=LINE('',#28383,#4345);
#3876=LINE('',#28385,#4346);
#3877=LINE('',#28389,#4347);
#3878=LINE('',#28391,#4348);
#3879=LINE('',#31480,#4349);
#3880=LINE('',#31544,#4350);
#3881=LINE('',#31607,#4351);
#3882=LINE('',#31628,#4352);
#3883=LINE('',#31662,#4353);
#3884=LINE('',#31706,#4354);
#3885=LINE('',#31731,#4355);
#3886=LINE('',#31733,#4356);
#3887=LINE('',#31736,#4357);
#3888=LINE('',#31738,#4358);
#3889=LINE('',#31741,#4359);
#3890=LINE('',#31743,#4360);
#3891=LINE('',#31746,#4361);
#3892=LINE('',#31748,#4362);
#3893=LINE('',#31751,#4363);
#3894=LINE('',#31753,#4364);
#3895=LINE('',#31756,#4365);
#3896=LINE('',#31758,#4366);
#3897=LINE('',#31761,#4367);
#3898=LINE('',#31763,#4368);
#3899=LINE('',#31766,#4369);
#3900=LINE('',#31768,#4370);
#3901=LINE('',#31771,#4371);
#3902=LINE('',#31773,#4372);
#3903=LINE('',#31776,#4373);
#3904=LINE('',#31778,#4374);
#3905=LINE('',#31781,#4375);
#3906=LINE('',#31783,#4376);
#3907=LINE('',#31786,#4377);
#3908=LINE('',#31788,#4378);
#3909=LINE('',#31791,#4379);
#3910=LINE('',#31793,#4380);
#3911=LINE('',#31796,#4381);
#3912=LINE('',#31798,#4382);
#3913=LINE('',#31801,#4383);
#3914=LINE('',#31802,#4384);
#4145=VECTOR('',#14385,8.12525);
#4146=VECTOR('',#14390,8.12525);
#4147=VECTOR('',#14393,8.12525);
#4148=VECTOR('',#14396,8.12525);
#4149=VECTOR('',#14399,8.12525);
#4150=VECTOR('',#14402,8.12525);
#4151=VECTOR('',#14405,8.12525);
#4152=VECTOR('',#14408,8.12525);
#4153=VECTOR('',#14411,8.12525);
#4154=VECTOR('',#14414,8.12525);
#4155=VECTOR('',#14417,8.12525);
#4156=VECTOR('',#14420,8.12525);
#4157=VECTOR('',#14425,7.01125);
#4158=VECTOR('',#14430,7.01125);
#4159=VECTOR('',#14433,7.01125);
#4160=VECTOR('',#14436,7.01125);
#4161=VECTOR('',#14439,7.01125);
#4162=VECTOR('',#14442,7.01125);
#4163=VECTOR('',#14445,7.01125);
#4164=VECTOR('',#14448,7.01125);
#4165=VECTOR('',#14451,7.01125);
#4166=VECTOR('',#14454,7.01125);
#4167=VECTOR('',#14457,7.01125);
#4168=VECTOR('',#14460,7.01125);
#4169=VECTOR('',#14471,10.);
#4170=VECTOR('',#14474,10.);
#4171=VECTOR('',#14477,10.);
#4172=VECTOR('',#14480,10.);
#4173=VECTOR('',#14483,10.);
#4174=VECTOR('',#14486,10.);
#4175=VECTOR('',#14489,10.);
#4176=VECTOR('',#14492,10.);
#4177=VECTOR('',#14495,10.);
#4178=VECTOR('',#14498,10.);
#4179=VECTOR('',#14501,10.);
#4180=VECTOR('',#14504,10.);
#4181=VECTOR('',#14507,10.);
#4182=VECTOR('',#14510,10.);
#4183=VECTOR('',#14513,10.);
#4184=VECTOR('',#14516,10.);
#4185=VECTOR('',#14519,10.);
#4186=VECTOR('',#14522,10.);
#4187=VECTOR('',#14525,10.);
#4188=VECTOR('',#14528,10.);
#4189=VECTOR('',#14531,10.);
#4190=VECTOR('',#14534,10.);
#4191=VECTOR('',#14537,10.);
#4192=VECTOR('',#14540,10.);
#4193=VECTOR('',#14543,10.);
#4194=VECTOR('',#14546,10.);
#4195=VECTOR('',#14549,10.);
#4196=VECTOR('',#14552,10.);
#4197=VECTOR('',#14555,10.);
#4198=VECTOR('',#14558,10.);
#4199=VECTOR('',#14561,10.);
#4200=VECTOR('',#14564,10.);
#4201=VECTOR('',#14567,10.);
#4202=VECTOR('',#14570,10.);
#4203=VECTOR('',#14573,10.);
#4204=VECTOR('',#14576,10.);
#4205=VECTOR('',#14579,10.);
#4206=VECTOR('',#14582,10.);
#4207=VECTOR('',#14587,10.);
#4208=VECTOR('',#14590,10.);
#4209=VECTOR('',#14595,10.);
#4210=VECTOR('',#14598,10.);
#4211=VECTOR('',#14603,10.);
#4212=VECTOR('',#14606,10.);
#4213=VECTOR('',#14611,10.);
#4214=VECTOR('',#14614,10.);
#4215=VECTOR('',#14619,10.);
#4216=VECTOR('',#14622,10.);
#4217=VECTOR('',#14627,10.);
#4218=VECTOR('',#14630,10.);
#4219=VECTOR('',#14635,10.);
#4220=VECTOR('',#14638,10.);
#4221=VECTOR('',#14643,10.);
#4222=VECTOR('',#14646,10.);
#4223=VECTOR('',#14651,10.);
#4224=VECTOR('',#14654,10.);
#4225=VECTOR('',#14659,10.);
#4226=VECTOR('',#14662,10.);
#4227=VECTOR('',#14667,10.);
#4228=VECTOR('',#14670,10.);
#4229=VECTOR('',#14675,10.);
#4230=VECTOR('',#14678,10.);
#4231=VECTOR('',#14683,10.);
#4232=VECTOR('',#14686,10.);
#4233=VECTOR('',#14691,10.);
#4234=VECTOR('',#14694,10.);
#4235=VECTOR('',#14699,10.);
#4236=VECTOR('',#14702,10.);
#4237=VECTOR('',#14707,10.);
#4238=VECTOR('',#14710,10.);
#4239=VECTOR('',#14715,10.);
#4240=VECTOR('',#14718,10.);
#4241=VECTOR('',#14727,10.);
#4242=VECTOR('',#14728,10.);
#4243=VECTOR('',#14735,10.);
#4244=VECTOR('',#14736,10.);
#4245=VECTOR('',#14743,10.);
#4246=VECTOR('',#14744,10.);
#4247=VECTOR('',#14751,10.);
#4248=VECTOR('',#14752,10.);
#4249=VECTOR('',#14759,10.);
#4250=VECTOR('',#14760,10.);
#4251=VECTOR('',#14767,10.);
#4252=VECTOR('',#14768,10.);
#4253=VECTOR('',#14775,10.);
#4254=VECTOR('',#14776,10.);
#4255=VECTOR('',#14783,10.);
#4256=VECTOR('',#14784,10.);
#4257=VECTOR('',#14791,10.);
#4258=VECTOR('',#14792,10.);
#4259=VECTOR('',#14799,10.);
#4260=VECTOR('',#14800,10.);
#4261=VECTOR('',#14807,10.);
#4262=VECTOR('',#14808,10.);
#4263=VECTOR('',#14815,10.);
#4264=VECTOR('',#14816,10.);
#4265=VECTOR('',#14823,10.);
#4266=VECTOR('',#14824,10.);
#4267=VECTOR('',#14831,10.);
#4268=VECTOR('',#14832,10.);
#4269=VECTOR('',#14839,10.);
#4270=VECTOR('',#14840,10.);
#4271=VECTOR('',#14847,10.);
#4272=VECTOR('',#14848,10.);
#4273=VECTOR('',#14855,10.);
#4274=VECTOR('',#14856,10.);
#4275=VECTOR('',#14863,10.);
#4276=VECTOR('',#14864,10.);
#4277=VECTOR('',#14873,10.);
#4278=VECTOR('',#14876,10.);
#4279=VECTOR('',#14885,10.);
#4280=VECTOR('',#14888,10.);
#4281=VECTOR('',#14897,10.);
#4282=VECTOR('',#14900,10.);
#4283=VECTOR('',#14909,10.);
#4284=VECTOR('',#14912,10.);
#4285=VECTOR('',#14921,10.);
#4286=VECTOR('',#14924,10.);
#4287=VECTOR('',#14933,10.);
#4288=VECTOR('',#14936,10.);
#4289=VECTOR('',#14945,10.);
#4290=VECTOR('',#14948,10.);
#4291=VECTOR('',#14957,10.);
#4292=VECTOR('',#14960,10.);
#4293=VECTOR('',#14969,10.);
#4294=VECTOR('',#14972,10.);
#4295=VECTOR('',#14981,10.);
#4296=VECTOR('',#14984,10.);
#4297=VECTOR('',#14993,10.);
#4298=VECTOR('',#14996,10.);
#4299=VECTOR('',#15005,10.);
#4300=VECTOR('',#15008,10.);
#4301=VECTOR('',#15017,10.);
#4302=VECTOR('',#15020,10.);
#4303=VECTOR('',#15029,10.);
#4304=VECTOR('',#15032,10.);
#4305=VECTOR('',#15041,10.);
#4306=VECTOR('',#15044,10.);
#4307=VECTOR('',#15053,10.);
#4308=VECTOR('',#15056,10.);
#4309=VECTOR('',#15065,10.);
#4310=VECTOR('',#15068,10.);
#4311=VECTOR('',#15077,10.);
#4312=VECTOR('',#15080,10.);
#4313=VECTOR('',#15083,10.);
#4314=VECTOR('',#15084,10.);
#4315=VECTOR('',#15089,10.);
#4316=VECTOR('',#15090,10.);
#4317=VECTOR('',#15095,10.);
#4318=VECTOR('',#15096,10.);
#4319=VECTOR('',#15101,10.);
#4320=VECTOR('',#15102,10.);
#4321=VECTOR('',#15107,10.);
#4322=VECTOR('',#15108,10.);
#4323=VECTOR('',#15113,10.);
#4324=VECTOR('',#15114,10.);
#4325=VECTOR('',#15119,10.);
#4326=VECTOR('',#15120,10.);
#4327=VECTOR('',#15125,10.);
#4328=VECTOR('',#15126,10.);
#4329=VECTOR('',#15131,10.);
#4330=VECTOR('',#15132,10.);
#4331=VECTOR('',#15137,10.);
#4332=VECTOR('',#15138,10.);
#4333=VECTOR('',#15143,10.);
#4334=VECTOR('',#15144,10.);
#4335=VECTOR('',#15149,10.);
#4336=VECTOR('',#15150,10.);
#4337=VECTOR('',#15155,10.);
#4338=VECTOR('',#15156,10.);
#4339=VECTOR('',#15161,10.);
#4340=VECTOR('',#15162,10.);
#4341=VECTOR('',#15167,10.);
#4342=VECTOR('',#15168,10.);
#4343=VECTOR('',#15173,10.);
#4344=VECTOR('',#15174,10.);
#4345=VECTOR('',#15179,10.);
#4346=VECTOR('',#15180,10.);
#4347=VECTOR('',#15185,10.);
#4348=VECTOR('',#15186,10.);
#4349=VECTOR('',#15681,10.);
#4350=VECTOR('',#15682,10.);
#4351=VECTOR('',#15691,10.);
#4352=VECTOR('',#15692,10.);
#4353=VECTOR('',#15693,10.);
#4354=VECTOR('',#15694,10.);
#4355=VECTOR('',#15701,10.);
#4356=VECTOR('',#15702,10.);
#4357=VECTOR('',#15705,10.);
#4358=VECTOR('',#15706,10.);
#4359=VECTOR('',#15709,10.);
#4360=VECTOR('',#15710,10.);
#4361=VECTOR('',#15713,10.);
#4362=VECTOR('',#15714,10.);
#4363=VECTOR('',#15717,10.);
#4364=VECTOR('',#15718,10.);
#4365=VECTOR('',#15721,10.);
#4366=VECTOR('',#15722,10.);
#4367=VECTOR('',#15725,10.);
#4368=VECTOR('',#15726,10.);
#4369=VECTOR('',#15729,10.);
#4370=VECTOR('',#15730,10.);
#4371=VECTOR('',#15733,10.);
#4372=VECTOR('',#15734,10.);
#4373=VECTOR('',#15737,10.);
#4374=VECTOR('',#15738,10.);
#4375=VECTOR('',#15741,10.);
#4376=VECTOR('',#15742,10.);
#4377=VECTOR('',#15745,10.);
#4378=VECTOR('',#15746,10.);
#4379=VECTOR('',#15749,10.);
#4380=VECTOR('',#15750,10.);
#4381=VECTOR('',#15753,10.);
#4382=VECTOR('',#15754,10.);
#4383=VECTOR('',#15757,10.);
#4384=VECTOR('',#15758,10.);
#4615=VERTEX_POINT('',#17356);
#4616=VERTEX_POINT('',#17357);
#4617=VERTEX_POINT('',#17359);
#4618=VERTEX_POINT('',#17368);
#4619=VERTEX_POINT('',#17380);
#4620=VERTEX_POINT('',#17381);
#4621=VERTEX_POINT('',#17383);
#4622=VERTEX_POINT('',#17567);
#4623=VERTEX_POINT('',#17750);
#4624=VERTEX_POINT('',#17751);
#4625=VERTEX_POINT('',#17753);
#4626=VERTEX_POINT('',#17860);
#4627=VERTEX_POINT('',#18128);
#4628=VERTEX_POINT('',#18129);
#4629=VERTEX_POINT('',#18131);
#4630=VERTEX_POINT('',#18313);
#4631=VERTEX_POINT('',#18584);
#4632=VERTEX_POINT('',#18585);
#4633=VERTEX_POINT('',#18587);
#4634=VERTEX_POINT('',#18857);
#4635=VERTEX_POINT('',#18968);
#4636=VERTEX_POINT('',#18969);
#4637=VERTEX_POINT('',#18971);
#4638=VERTEX_POINT('',#19238);
#4639=VERTEX_POINT('',#19420);
#4640=VERTEX_POINT('',#19421);
#4641=VERTEX_POINT('',#19423);
#4642=VERTEX_POINT('',#19533);
#4643=VERTEX_POINT('',#19804);
#4644=VERTEX_POINT('',#19805);
#4645=VERTEX_POINT('',#19807);
#4646=VERTEX_POINT('',#19991);
#4647=VERTEX_POINT('',#20102);
#4648=VERTEX_POINT('',#20103);
#4649=VERTEX_POINT('',#20105);
#4650=VERTEX_POINT('',#20212);
#4651=VERTEX_POINT('',#20394);
#4652=VERTEX_POINT('',#20395);
#4653=VERTEX_POINT('',#20397);
#4654=VERTEX_POINT('',#20579);
#4655=VERTEX_POINT('',#20690);
#4656=VERTEX_POINT('',#20691);
#4657=VERTEX_POINT('',#20693);
#4658=VERTEX_POINT('',#20801);
#4659=VERTEX_POINT('',#20987);
#4660=VERTEX_POINT('',#20988);
#4661=VERTEX_POINT('',#20990);
#4662=VERTEX_POINT('',#21000);
#4663=VERTEX_POINT('',#21007);
#4664=VERTEX_POINT('',#21009);
#4665=VERTEX_POINT('',#21184);
#4666=VERTEX_POINT('',#21185);
#4667=VERTEX_POINT('',#21187);
#4668=VERTEX_POINT('',#21196);
#4669=VERTEX_POINT('',#21287);
#4670=VERTEX_POINT('',#21288);
#4671=VERTEX_POINT('',#21444);
#4672=VERTEX_POINT('',#21479);
#4673=VERTEX_POINT('',#21480);
#4674=VERTEX_POINT('',#21482);
#4675=VERTEX_POINT('',#21511);
#4676=VERTEX_POINT('',#21771);
#4677=VERTEX_POINT('',#21772);
#4678=VERTEX_POINT('',#21774);
#4679=VERTEX_POINT('',#22032);
#4680=VERTEX_POINT('',#22066);
#4681=VERTEX_POINT('',#22067);
#4682=VERTEX_POINT('',#22069);
#4683=VERTEX_POINT('',#22102);
#4684=VERTEX_POINT('',#22361);
#4685=VERTEX_POINT('',#22362);
#4686=VERTEX_POINT('',#22364);
#4687=VERTEX_POINT('',#22623);
#4688=VERTEX_POINT('',#22657);
#4689=VERTEX_POINT('',#22658);
#4690=VERTEX_POINT('',#22660);
#4691=VERTEX_POINT('',#22813);
#4692=VERTEX_POINT('',#23073);
#4693=VERTEX_POINT('',#23074);
#4694=VERTEX_POINT('',#23228);
#4695=VERTEX_POINT('',#23262);
#4696=VERTEX_POINT('',#23263);
#4697=VERTEX_POINT('',#23265);
#4698=VERTEX_POINT('',#23531);
#4699=VERTEX_POINT('',#23676);
#4700=VERTEX_POINT('',#23677);
#4701=VERTEX_POINT('',#23679);
#4702=VERTEX_POINT('',#23977);
#4703=VERTEX_POINT('',#23978);
#4704=VERTEX_POINT('',#24128);
#4705=VERTEX_POINT('',#24391);
#4706=VERTEX_POINT('',#24392);
#4707=VERTEX_POINT('',#24394);
#4708=VERTEX_POINT('',#24400);
#4709=VERTEX_POINT('',#24561);
#4710=VERTEX_POINT('',#24702);
#4711=VERTEX_POINT('',#24847);
#4712=VERTEX_POINT('',#24881);
#4713=VERTEX_POINT('',#25062);
#4714=VERTEX_POINT('',#26774);
#4715=VERTEX_POINT('',#26895);
#4716=VERTEX_POINT('',#26896);
#4717=VERTEX_POINT('',#26898);
#4718=VERTEX_POINT('',#26900);
#4719=VERTEX_POINT('',#26902);
#4720=VERTEX_POINT('',#26904);
#4721=VERTEX_POINT('',#26906);
#4722=VERTEX_POINT('',#26908);
#4723=VERTEX_POINT('',#26910);
#4724=VERTEX_POINT('',#26912);
#4725=VERTEX_POINT('',#26914);
#4726=VERTEX_POINT('',#26916);
#4727=VERTEX_POINT('',#26918);
#4728=VERTEX_POINT('',#26920);
#4729=VERTEX_POINT('',#26922);
#4730=VERTEX_POINT('',#26924);
#4731=VERTEX_POINT('',#26926);
#4732=VERTEX_POINT('',#26928);
#4733=VERTEX_POINT('',#26930);
#4734=VERTEX_POINT('',#26932);
#4735=VERTEX_POINT('',#26934);
#4736=VERTEX_POINT('',#26936);
#4737=VERTEX_POINT('',#26938);
#4738=VERTEX_POINT('',#26940);
#4739=VERTEX_POINT('',#26942);
#4740=VERTEX_POINT('',#26944);
#4741=VERTEX_POINT('',#26946);
#4742=VERTEX_POINT('',#26948);
#4743=VERTEX_POINT('',#26950);
#4744=VERTEX_POINT('',#26952);
#4745=VERTEX_POINT('',#26954);
#4746=VERTEX_POINT('',#26956);
#4747=VERTEX_POINT('',#26958);
#4748=VERTEX_POINT('',#26960);
#4749=VERTEX_POINT('',#26962);
#4750=VERTEX_POINT('',#26964);
#4751=VERTEX_POINT('',#26966);
#4752=VERTEX_POINT('',#26968);
#4753=VERTEX_POINT('',#26970);
#4754=VERTEX_POINT('',#26972);
#4755=VERTEX_POINT('',#26974);
#4756=VERTEX_POINT('',#26976);
#4757=VERTEX_POINT('',#26978);
#4758=VERTEX_POINT('',#26980);
#4759=VERTEX_POINT('',#26982);
#4760=VERTEX_POINT('',#26984);
#4761=VERTEX_POINT('',#26986);
#4762=VERTEX_POINT('',#26988);
#4763=VERTEX_POINT('',#26990);
#4764=VERTEX_POINT('',#26992);
#4765=VERTEX_POINT('',#26994);
#4766=VERTEX_POINT('',#26996);
#4767=VERTEX_POINT('',#26998);
#4768=VERTEX_POINT('',#27000);
#4769=VERTEX_POINT('',#27002);
#4770=VERTEX_POINT('',#27004);
#4771=VERTEX_POINT('',#27006);
#4772=VERTEX_POINT('',#27008);
#4773=VERTEX_POINT('',#27010);
#4774=VERTEX_POINT('',#27012);
#4775=VERTEX_POINT('',#27014);
#4776=VERTEX_POINT('',#27016);
#4777=VERTEX_POINT('',#27018);
#4778=VERTEX_POINT('',#27020);
#4779=VERTEX_POINT('',#27022);
#4780=VERTEX_POINT('',#27024);
#4781=VERTEX_POINT('',#27026);
#4782=VERTEX_POINT('',#27028);
#4783=VERTEX_POINT('',#27030);
#4784=VERTEX_POINT('',#27032);
#4785=VERTEX_POINT('',#27034);
#4786=VERTEX_POINT('',#27036);
#4787=VERTEX_POINT('',#27040);
#4788=VERTEX_POINT('',#27041);
#4789=VERTEX_POINT('',#27043);
#4790=VERTEX_POINT('',#27045);
#4791=VERTEX_POINT('',#27049);
#4792=VERTEX_POINT('',#27050);
#4793=VERTEX_POINT('',#27052);
#4794=VERTEX_POINT('',#27054);
#4795=VERTEX_POINT('',#27058);
#4796=VERTEX_POINT('',#27059);
#4797=VERTEX_POINT('',#27061);
#4798=VERTEX_POINT('',#27063);
#4799=VERTEX_POINT('',#27067);
#4800=VERTEX_POINT('',#27068);
#4801=VERTEX_POINT('',#27070);
#4802=VERTEX_POINT('',#27072);
#4803=VERTEX_POINT('',#27076);
#4804=VERTEX_POINT('',#27077);
#4805=VERTEX_POINT('',#27079);
#4806=VERTEX_POINT('',#27081);
#4807=VERTEX_POINT('',#27085);
#4808=VERTEX_POINT('',#27086);
#4809=VERTEX_POINT('',#27088);
#4810=VERTEX_POINT('',#27090);
#4811=VERTEX_POINT('',#27094);
#4812=VERTEX_POINT('',#27095);
#4813=VERTEX_POINT('',#27097);
#4814=VERTEX_POINT('',#27099);
#4815=VERTEX_POINT('',#27103);
#4816=VERTEX_POINT('',#27104);
#4817=VERTEX_POINT('',#27106);
#4818=VERTEX_POINT('',#27108);
#4819=VERTEX_POINT('',#27112);
#4820=VERTEX_POINT('',#27113);
#4821=VERTEX_POINT('',#27115);
#4822=VERTEX_POINT('',#27117);
#4823=VERTEX_POINT('',#27121);
#4824=VERTEX_POINT('',#27122);
#4825=VERTEX_POINT('',#27124);
#4826=VERTEX_POINT('',#27126);
#4827=VERTEX_POINT('',#27130);
#4828=VERTEX_POINT('',#27131);
#4829=VERTEX_POINT('',#27133);
#4830=VERTEX_POINT('',#27135);
#4831=VERTEX_POINT('',#27139);
#4832=VERTEX_POINT('',#27140);
#4833=VERTEX_POINT('',#27142);
#4834=VERTEX_POINT('',#27144);
#4835=VERTEX_POINT('',#27148);
#4836=VERTEX_POINT('',#27149);
#4837=VERTEX_POINT('',#27151);
#4838=VERTEX_POINT('',#27153);
#4839=VERTEX_POINT('',#27157);
#4840=VERTEX_POINT('',#27158);
#4841=VERTEX_POINT('',#27160);
#4842=VERTEX_POINT('',#27162);
#4843=VERTEX_POINT('',#27166);
#4844=VERTEX_POINT('',#27167);
#4845=VERTEX_POINT('',#27169);
#4846=VERTEX_POINT('',#27171);
#4847=VERTEX_POINT('',#27175);
#4848=VERTEX_POINT('',#27176);
#4849=VERTEX_POINT('',#27178);
#4850=VERTEX_POINT('',#27180);
#4851=VERTEX_POINT('',#27184);
#4852=VERTEX_POINT('',#27185);
#4853=VERTEX_POINT('',#27187);
#4854=VERTEX_POINT('',#27189);
#4855=VERTEX_POINT('',#27193);
#4856=VERTEX_POINT('',#27194);
#4857=VERTEX_POINT('',#27196);
#4858=VERTEX_POINT('',#27198);
#4859=VERTEX_POINT('',#27202);
#4860=VERTEX_POINT('',#27204);
#4861=VERTEX_POINT('',#27206);
#4862=VERTEX_POINT('',#27216);
#4863=VERTEX_POINT('',#27229);
#4864=VERTEX_POINT('',#27231);
#4865=VERTEX_POINT('',#27233);
#4866=VERTEX_POINT('',#27243);
#4867=VERTEX_POINT('',#27256);
#4868=VERTEX_POINT('',#27258);
#4869=VERTEX_POINT('',#27260);
#4870=VERTEX_POINT('',#27270);
#4871=VERTEX_POINT('',#27281);
#4872=VERTEX_POINT('',#27283);
#4873=VERTEX_POINT('',#27285);
#4874=VERTEX_POINT('',#27295);
#4875=VERTEX_POINT('',#27308);
#4876=VERTEX_POINT('',#27310);
#4877=VERTEX_POINT('',#27312);
#4878=VERTEX_POINT('',#27322);
#4879=VERTEX_POINT('',#27335);
#4880=VERTEX_POINT('',#27337);
#4881=VERTEX_POINT('',#27339);
#4882=VERTEX_POINT('',#27349);
#4883=VERTEX_POINT('',#27362);
#4884=VERTEX_POINT('',#27364);
#4885=VERTEX_POINT('',#27366);
#4886=VERTEX_POINT('',#27376);
#4887=VERTEX_POINT('',#27387);
#4888=VERTEX_POINT('',#27389);
#4889=VERTEX_POINT('',#27391);
#4890=VERTEX_POINT('',#27401);
#4891=VERTEX_POINT('',#27414);
#4892=VERTEX_POINT('',#27416);
#4893=VERTEX_POINT('',#27418);
#4894=VERTEX_POINT('',#27428);
#4895=VERTEX_POINT('',#27441);
#4896=VERTEX_POINT('',#27443);
#4897=VERTEX_POINT('',#27445);
#4898=VERTEX_POINT('',#27455);
#4899=VERTEX_POINT('',#27468);
#4900=VERTEX_POINT('',#27470);
#4901=VERTEX_POINT('',#27472);
#4902=VERTEX_POINT('',#27482);
#4903=VERTEX_POINT('',#27493);
#4904=VERTEX_POINT('',#27495);
#4905=VERTEX_POINT('',#27497);
#4906=VERTEX_POINT('',#27507);
#4907=VERTEX_POINT('',#27520);
#4908=VERTEX_POINT('',#27522);
#4909=VERTEX_POINT('',#27524);
#4910=VERTEX_POINT('',#27534);
#4911=VERTEX_POINT('',#27547);
#4912=VERTEX_POINT('',#27549);
#4913=VERTEX_POINT('',#27551);
#4914=VERTEX_POINT('',#27561);
#4915=VERTEX_POINT('',#27574);
#4916=VERTEX_POINT('',#27576);
#4917=VERTEX_POINT('',#27578);
#4918=VERTEX_POINT('',#27588);
#4919=VERTEX_POINT('',#27601);
#4920=VERTEX_POINT('',#27603);
#4921=VERTEX_POINT('',#27605);
#4922=VERTEX_POINT('',#27615);
#4923=VERTEX_POINT('',#27628);
#4924=VERTEX_POINT('',#27630);
#4925=VERTEX_POINT('',#27632);
#4926=VERTEX_POINT('',#27642);
#4927=VERTEX_POINT('',#27655);
#4928=VERTEX_POINT('',#27657);
#4929=VERTEX_POINT('',#27659);
#4930=VERTEX_POINT('',#27669);
#4931=VERTEX_POINT('',#27682);
#4932=VERTEX_POINT('',#27683);
#4933=VERTEX_POINT('',#27685);
#4934=VERTEX_POINT('',#27687);
#4935=VERTEX_POINT('',#27689);
#4936=VERTEX_POINT('',#27691);
#4937=VERTEX_POINT('',#27700);
#4938=VERTEX_POINT('',#27702);
#4939=VERTEX_POINT('',#27715);
#4940=VERTEX_POINT('',#27716);
#4941=VERTEX_POINT('',#27718);
#4942=VERTEX_POINT('',#27720);
#4943=VERTEX_POINT('',#27722);
#4944=VERTEX_POINT('',#27724);
#4945=VERTEX_POINT('',#27735);
#4946=VERTEX_POINT('',#27737);
#4947=VERTEX_POINT('',#27748);
#4948=VERTEX_POINT('',#27749);
#4949=VERTEX_POINT('',#27751);
#4950=VERTEX_POINT('',#27753);
#4951=VERTEX_POINT('',#27755);
#4952=VERTEX_POINT('',#27757);
#4953=VERTEX_POINT('',#27768);
#4954=VERTEX_POINT('',#27770);
#4955=VERTEX_POINT('',#27783);
#4956=VERTEX_POINT('',#27784);
#4957=VERTEX_POINT('',#27786);
#4958=VERTEX_POINT('',#27788);
#4959=VERTEX_POINT('',#27790);
#4960=VERTEX_POINT('',#27792);
#4961=VERTEX_POINT('',#27801);
#4962=VERTEX_POINT('',#27803);
#4963=VERTEX_POINT('',#27814);
#4964=VERTEX_POINT('',#27815);
#4965=VERTEX_POINT('',#27817);
#4966=VERTEX_POINT('',#27819);
#4967=VERTEX_POINT('',#27821);
#4968=VERTEX_POINT('',#27823);
#4969=VERTEX_POINT('',#27834);
#4970=VERTEX_POINT('',#27836);
#4971=VERTEX_POINT('',#27849);
#4972=VERTEX_POINT('',#27850);
#4973=VERTEX_POINT('',#27852);
#4974=VERTEX_POINT('',#27854);
#4975=VERTEX_POINT('',#27856);
#4976=VERTEX_POINT('',#27858);
#4977=VERTEX_POINT('',#27869);
#4978=VERTEX_POINT('',#27871);
#4979=VERTEX_POINT('',#27884);
#4980=VERTEX_POINT('',#27885);
#4981=VERTEX_POINT('',#27887);
#4982=VERTEX_POINT('',#27889);
#4983=VERTEX_POINT('',#27891);
#4984=VERTEX_POINT('',#27893);
#4985=VERTEX_POINT('',#27904);
#4986=VERTEX_POINT('',#27906);
#4987=VERTEX_POINT('',#27917);
#4988=VERTEX_POINT('',#27918);
#4989=VERTEX_POINT('',#27920);
#4990=VERTEX_POINT('',#27922);
#4991=VERTEX_POINT('',#27924);
#4992=VERTEX_POINT('',#27926);
#4993=VERTEX_POINT('',#27935);
#4994=VERTEX_POINT('',#27937);
#4995=VERTEX_POINT('',#27950);
#4996=VERTEX_POINT('',#27951);
#4997=VERTEX_POINT('',#27953);
#4998=VERTEX_POINT('',#27955);
#4999=VERTEX_POINT('',#27957);
#5000=VERTEX_POINT('',#27959);
#5001=VERTEX_POINT('',#27970);
#5002=VERTEX_POINT('',#27972);
#5003=VERTEX_POINT('',#27985);
#5004=VERTEX_POINT('',#27986);
#5005=VERTEX_POINT('',#27988);
#5006=VERTEX_POINT('',#27990);
#5007=VERTEX_POINT('',#27992);
#5008=VERTEX_POINT('',#27994);
#5009=VERTEX_POINT('',#28005);
#5010=VERTEX_POINT('',#28007);
#5011=VERTEX_POINT('',#28020);
#5012=VERTEX_POINT('',#28021);
#5013=VERTEX_POINT('',#28023);
#5014=VERTEX_POINT('',#28025);
#5015=VERTEX_POINT('',#28027);
#5016=VERTEX_POINT('',#28029);
#5017=VERTEX_POINT('',#28040);
#5018=VERTEX_POINT('',#28042);
#5019=VERTEX_POINT('',#28053);
#5020=VERTEX_POINT('',#28054);
#5021=VERTEX_POINT('',#28056);
#5022=VERTEX_POINT('',#28058);
#5023=VERTEX_POINT('',#28060);
#5024=VERTEX_POINT('',#28062);
#5025=VERTEX_POINT('',#28071);
#5026=VERTEX_POINT('',#28073);
#5027=VERTEX_POINT('',#28086);
#5028=VERTEX_POINT('',#28087);
#5029=VERTEX_POINT('',#28089);
#5030=VERTEX_POINT('',#28091);
#5031=VERTEX_POINT('',#28093);
#5032=VERTEX_POINT('',#28095);
#5033=VERTEX_POINT('',#28106);
#5034=VERTEX_POINT('',#28108);
#5035=VERTEX_POINT('',#28119);
#5036=VERTEX_POINT('',#28120);
#5037=VERTEX_POINT('',#28122);
#5038=VERTEX_POINT('',#28124);
#5039=VERTEX_POINT('',#28126);
#5040=VERTEX_POINT('',#28128);
#5041=VERTEX_POINT('',#28139);
#5042=VERTEX_POINT('',#28141);
#5043=VERTEX_POINT('',#28154);
#5044=VERTEX_POINT('',#28155);
#5045=VERTEX_POINT('',#28157);
#5046=VERTEX_POINT('',#28159);
#5047=VERTEX_POINT('',#28161);
#5048=VERTEX_POINT('',#28163);
#5049=VERTEX_POINT('',#28174);
#5050=VERTEX_POINT('',#28176);
#5051=VERTEX_POINT('',#28189);
#5052=VERTEX_POINT('',#28190);
#5053=VERTEX_POINT('',#28192);
#5054=VERTEX_POINT('',#28194);
#5055=VERTEX_POINT('',#28196);
#5056=VERTEX_POINT('',#28198);
#5057=VERTEX_POINT('',#28209);
#5058=VERTEX_POINT('',#28211);
#5059=VERTEX_POINT('',#28222);
#5060=VERTEX_POINT('',#28223);
#5061=VERTEX_POINT('',#28225);
#5062=VERTEX_POINT('',#28227);
#5063=VERTEX_POINT('',#28229);
#5064=VERTEX_POINT('',#28231);
#5065=VERTEX_POINT('',#28240);
#5066=VERTEX_POINT('',#28242);
#5067=VERTEX_POINT('',#28255);
#5068=VERTEX_POINT('',#28256);
#5069=VERTEX_POINT('',#28258);
#5070=VERTEX_POINT('',#28260);
#5071=VERTEX_POINT('',#28262);
#5072=VERTEX_POINT('',#28264);
#5073=VERTEX_POINT('',#28273);
#5074=VERTEX_POINT('',#28275);
#5075=VERTEX_POINT('',#28286);
#5076=VERTEX_POINT('',#28288);
#5077=VERTEX_POINT('',#28292);
#5078=VERTEX_POINT('',#28294);
#5079=VERTEX_POINT('',#28298);
#5080=VERTEX_POINT('',#28300);
#5081=VERTEX_POINT('',#28304);
#5082=VERTEX_POINT('',#28306);
#5083=VERTEX_POINT('',#28310);
#5084=VERTEX_POINT('',#28312);
#5085=VERTEX_POINT('',#28316);
#5086=VERTEX_POINT('',#28318);
#5087=VERTEX_POINT('',#28322);
#5088=VERTEX_POINT('',#28324);
#5089=VERTEX_POINT('',#28328);
#5090=VERTEX_POINT('',#28330);
#5091=VERTEX_POINT('',#28334);
#5092=VERTEX_POINT('',#28336);
#5093=VERTEX_POINT('',#28340);
#5094=VERTEX_POINT('',#28342);
#5095=VERTEX_POINT('',#28346);
#5096=VERTEX_POINT('',#28348);
#5097=VERTEX_POINT('',#28352);
#5098=VERTEX_POINT('',#28354);
#5099=VERTEX_POINT('',#28358);
#5100=VERTEX_POINT('',#28360);
#5101=VERTEX_POINT('',#28364);
#5102=VERTEX_POINT('',#28366);
#5103=VERTEX_POINT('',#28370);
#5104=VERTEX_POINT('',#28372);
#5105=VERTEX_POINT('',#28376);
#5106=VERTEX_POINT('',#28378);
#5107=VERTEX_POINT('',#28382);
#5108=VERTEX_POINT('',#28384);
#5109=VERTEX_POINT('',#28388);
#5110=VERTEX_POINT('',#28390);
#5111=VERTEX_POINT('',#28394);
#5112=VERTEX_POINT('',#28395);
#5113=VERTEX_POINT('',#28397);
#5114=VERTEX_POINT('',#28399);
#5115=VERTEX_POINT('',#28408);
#5116=VERTEX_POINT('',#28409);
#5117=VERTEX_POINT('',#28411);
#5118=VERTEX_POINT('',#28413);
#5119=VERTEX_POINT('',#28417);
#5120=VERTEX_POINT('',#28418);
#5121=VERTEX_POINT('',#28420);
#5122=VERTEX_POINT('',#28422);
#5123=VERTEX_POINT('',#28426);
#5124=VERTEX_POINT('',#28427);
#5125=VERTEX_POINT('',#28429);
#5126=VERTEX_POINT('',#28431);
#5127=VERTEX_POINT('',#28440);
#5128=VERTEX_POINT('',#28441);
#5129=VERTEX_POINT('',#28443);
#5130=VERTEX_POINT('',#28445);
#5131=VERTEX_POINT('',#28449);
#5132=VERTEX_POINT('',#28450);
#5133=VERTEX_POINT('',#28452);
#5134=VERTEX_POINT('',#28454);
#5135=VERTEX_POINT('',#28458);
#5136=VERTEX_POINT('',#28459);
#5137=VERTEX_POINT('',#28461);
#5138=VERTEX_POINT('',#28463);
#5139=VERTEX_POINT('',#28467);
#5140=VERTEX_POINT('',#28468);
#5141=VERTEX_POINT('',#28470);
#5142=VERTEX_POINT('',#28472);
#5143=VERTEX_POINT('',#28481);
#5144=VERTEX_POINT('',#28482);
#5145=VERTEX_POINT('',#28484);
#5146=VERTEX_POINT('',#28486);
#5147=VERTEX_POINT('',#28490);
#5148=VERTEX_POINT('',#28491);
#5149=VERTEX_POINT('',#28493);
#5150=VERTEX_POINT('',#28495);
#5151=VERTEX_POINT('',#28499);
#5152=VERTEX_POINT('',#28500);
#5153=VERTEX_POINT('',#28502);
#5154=VERTEX_POINT('',#28504);
#5155=VERTEX_POINT('',#28508);
#5156=VERTEX_POINT('',#28509);
#5157=VERTEX_POINT('',#28511);
#5158=VERTEX_POINT('',#28513);
#5159=VERTEX_POINT('',#28522);
#5160=VERTEX_POINT('',#28523);
#5161=VERTEX_POINT('',#28525);
#5162=VERTEX_POINT('',#28527);
#5163=VERTEX_POINT('',#28531);
#5164=VERTEX_POINT('',#28532);
#5165=VERTEX_POINT('',#28534);
#5166=VERTEX_POINT('',#28536);
#5167=VERTEX_POINT('',#28540);
#5168=VERTEX_POINT('',#28541);
#5169=VERTEX_POINT('',#28543);
#5170=VERTEX_POINT('',#28545);
#5171=VERTEX_POINT('',#28549);
#5172=VERTEX_POINT('',#28550);
#5173=VERTEX_POINT('',#28552);
#5174=VERTEX_POINT('',#28554);
#5175=VERTEX_POINT('',#28558);
#5176=VERTEX_POINT('',#28559);
#5177=VERTEX_POINT('',#28561);
#5178=VERTEX_POINT('',#28563);
#5179=VERTEX_POINT('',#28572);
#5180=VERTEX_POINT('',#28573);
#5181=VERTEX_POINT('',#28575);
#5182=VERTEX_POINT('',#28577);
#5183=VERTEX_POINT('',#28586);
#5184=VERTEX_POINT('',#28587);
#5185=VERTEX_POINT('',#28594);
#5186=VERTEX_POINT('',#28596);
#5187=VERTEX_POINT('',#28600);
#5188=VERTEX_POINT('',#28601);
#5189=VERTEX_POINT('',#28608);
#5190=VERTEX_POINT('',#28610);
#5191=VERTEX_POINT('',#28614);
#5192=VERTEX_POINT('',#28615);
#5193=VERTEX_POINT('',#28622);
#5194=VERTEX_POINT('',#28624);
#5195=VERTEX_POINT('',#28628);
#5196=VERTEX_POINT('',#28629);
#5197=VERTEX_POINT('',#28636);
#5198=VERTEX_POINT('',#28638);
#5199=VERTEX_POINT('',#28642);
#5200=VERTEX_POINT('',#28643);
#5201=VERTEX_POINT('',#28650);
#5202=VERTEX_POINT('',#28652);
#5203=VERTEX_POINT('',#28656);
#5204=VERTEX_POINT('',#28657);
#5205=VERTEX_POINT('',#28664);
#5206=VERTEX_POINT('',#28666);
#5207=VERTEX_POINT('',#28670);
#5208=VERTEX_POINT('',#28671);
#5209=VERTEX_POINT('',#28678);
#5210=VERTEX_POINT('',#28680);
#5211=VERTEX_POINT('',#28684);
#5212=VERTEX_POINT('',#28685);
#5213=VERTEX_POINT('',#28692);
#5214=VERTEX_POINT('',#28694);
#5215=VERTEX_POINT('',#28698);
#5216=VERTEX_POINT('',#28699);
#5217=VERTEX_POINT('',#28706);
#5218=VERTEX_POINT('',#28708);
#5219=VERTEX_POINT('',#28712);
#5220=VERTEX_POINT('',#28713);
#5221=VERTEX_POINT('',#28720);
#5222=VERTEX_POINT('',#28722);
#5223=VERTEX_POINT('',#28726);
#5224=VERTEX_POINT('',#28727);
#5225=VERTEX_POINT('',#28734);
#5226=VERTEX_POINT('',#28736);
#5227=VERTEX_POINT('',#28740);
#5228=VERTEX_POINT('',#28741);
#5229=VERTEX_POINT('',#28748);
#5230=VERTEX_POINT('',#28750);
#5231=VERTEX_POINT('',#28754);
#5232=VERTEX_POINT('',#28755);
#5233=VERTEX_POINT('',#28762);
#5234=VERTEX_POINT('',#28764);
#5235=VERTEX_POINT('',#28768);
#5236=VERTEX_POINT('',#28769);
#5237=VERTEX_POINT('',#28776);
#5238=VERTEX_POINT('',#28778);
#5239=VERTEX_POINT('',#28782);
#5240=VERTEX_POINT('',#28783);
#5241=VERTEX_POINT('',#28790);
#5242=VERTEX_POINT('',#28792);
#5243=VERTEX_POINT('',#28796);
#5244=VERTEX_POINT('',#28797);
#5245=VERTEX_POINT('',#28804);
#5246=VERTEX_POINT('',#28806);
#5247=VERTEX_POINT('',#28810);
#5248=VERTEX_POINT('',#28811);
#5249=VERTEX_POINT('',#28818);
#5250=VERTEX_POINT('',#28820);
#5251=VERTEX_POINT('',#28824);
#5252=VERTEX_POINT('',#28825);
#5253=VERTEX_POINT('',#28832);
#5254=VERTEX_POINT('',#28834);
#5255=VERTEX_POINT('',#31479);
#5256=VERTEX_POINT('',#31530);
#5257=VERTEX_POINT('',#31546);
#5258=VERTEX_POINT('',#31562);
#5259=VERTEX_POINT('',#31593);
#5260=VERTEX_POINT('',#31661);
#5261=VERTEX_POINT('',#31692);
#5262=VERTEX_POINT('',#31729);
#5263=VERTEX_POINT('',#31732);
#5264=VERTEX_POINT('',#31734);
#5265=VERTEX_POINT('',#31737);
#5266=VERTEX_POINT('',#31739);
#5267=VERTEX_POINT('',#31742);
#5268=VERTEX_POINT('',#31744);
#5269=VERTEX_POINT('',#31747);
#5270=VERTEX_POINT('',#31749);
#5271=VERTEX_POINT('',#31752);
#5272=VERTEX_POINT('',#31754);
#5273=VERTEX_POINT('',#31757);
#5274=VERTEX_POINT('',#31759);
#5275=VERTEX_POINT('',#31762);
#5276=VERTEX_POINT('',#31764);
#5277=VERTEX_POINT('',#31767);
#5278=VERTEX_POINT('',#31769);
#5279=VERTEX_POINT('',#31772);
#5280=VERTEX_POINT('',#31774);
#5281=VERTEX_POINT('',#31777);
#5282=VERTEX_POINT('',#31779);
#5283=VERTEX_POINT('',#31782);
#5284=VERTEX_POINT('',#31784);
#5285=VERTEX_POINT('',#31787);
#5286=VERTEX_POINT('',#31789);
#5287=VERTEX_POINT('',#31792);
#5288=VERTEX_POINT('',#31794);
#5289=VERTEX_POINT('',#31797);
#5290=VERTEX_POINT('',#31799);
#6048=EDGE_CURVE('',#4615,#4616,#3675,.T.);
#6049=EDGE_CURVE('',#4616,#4617,#2872,.T.);
#6050=EDGE_CURVE('',#4618,#4617,#2221,.T.);
#6051=EDGE_CURVE('',#4615,#4618,#2873,.T.);
#6052=EDGE_CURVE('',#4619,#4620,#3676,.T.);
#6053=EDGE_CURVE('',#4620,#4621,#2874,.T.);
#6054=EDGE_CURVE('',#4621,#4616,#2875,.T.);
#6055=EDGE_CURVE('',#4622,#4615,#2876,.T.);
#6056=EDGE_CURVE('',#4619,#4622,#2877,.T.);
#6057=EDGE_CURVE('',#4623,#4624,#3677,.T.);
#6058=EDGE_CURVE('',#4624,#4625,#2878,.T.);
#6059=EDGE_CURVE('',#4625,#4620,#2879,.T.);
#6060=EDGE_CURVE('',#4626,#4619,#2880,.T.);
#6061=EDGE_CURVE('',#4623,#4626,#2881,.T.);
#6062=EDGE_CURVE('',#4627,#4628,#3678,.T.);
#6063=EDGE_CURVE('',#4628,#4629,#2882,.T.);
#6064=EDGE_CURVE('',#4629,#4624,#2883,.T.);
#6065=EDGE_CURVE('',#4630,#4623,#2884,.T.);
#6066=EDGE_CURVE('',#4627,#4630,#2885,.T.);
#6067=EDGE_CURVE('',#4631,#4632,#3679,.T.);
#6068=EDGE_CURVE('',#4632,#4633,#2886,.T.);
#6069=EDGE_CURVE('',#4633,#4628,#2887,.T.);
#6070=EDGE_CURVE('',#4634,#4627,#2888,.T.);
#6071=EDGE_CURVE('',#4631,#4634,#2889,.T.);
#6072=EDGE_CURVE('',#4635,#4636,#3680,.T.);
#6073=EDGE_CURVE('',#4636,#4637,#2890,.T.);
#6074=EDGE_CURVE('',#4637,#4632,#2891,.T.);
#6075=EDGE_CURVE('',#4638,#4631,#2892,.T.);
#6076=EDGE_CURVE('',#4635,#4638,#2893,.T.);
#6077=EDGE_CURVE('',#4639,#4640,#3681,.T.);
#6078=EDGE_CURVE('',#4640,#4641,#2894,.T.);
#6079=EDGE_CURVE('',#4641,#4636,#2895,.T.);
#6080=EDGE_CURVE('',#4642,#4635,#2896,.T.);
#6081=EDGE_CURVE('',#4639,#4642,#2897,.T.);
#6082=EDGE_CURVE('',#4643,#4644,#3682,.T.);
#6083=EDGE_CURVE('',#4644,#4645,#2898,.T.);
#6084=EDGE_CURVE('',#4645,#4640,#2899,.T.);
#6085=EDGE_CURVE('',#4646,#4639,#2900,.T.);
#6086=EDGE_CURVE('',#4643,#4646,#2901,.T.);
#6087=EDGE_CURVE('',#4647,#4648,#3683,.T.);
#6088=EDGE_CURVE('',#4648,#4649,#2902,.T.);
#6089=EDGE_CURVE('',#4649,#4644,#2903,.T.);
#6090=EDGE_CURVE('',#4650,#4643,#2904,.T.);
#6091=EDGE_CURVE('',#4647,#4650,#2905,.T.);
#6092=EDGE_CURVE('',#4651,#4652,#3684,.T.);
#6093=EDGE_CURVE('',#4652,#4653,#2906,.T.);
#6094=EDGE_CURVE('',#4653,#4648,#2907,.T.);
#6095=EDGE_CURVE('',#4654,#4647,#2908,.T.);
#6096=EDGE_CURVE('',#4651,#4654,#2909,.T.);
#6097=EDGE_CURVE('',#4655,#4656,#3685,.T.);
#6098=EDGE_CURVE('',#4656,#4657,#2910,.T.);
#6099=EDGE_CURVE('',#4657,#4652,#2911,.T.);
#6100=EDGE_CURVE('',#4658,#4651,#2912,.T.);
#6101=EDGE_CURVE('',#4655,#4658,#2913,.T.);
#6102=EDGE_CURVE('',#4659,#4660,#3686,.T.);
#6103=EDGE_CURVE('',#4661,#4659,#2914,.T.);
#6104=EDGE_CURVE('',#4662,#4661,#2915,.T.);
#6105=EDGE_CURVE('',#4663,#4662,#2222,.T.);
#6106=EDGE_CURVE('',#4663,#4664,#2916,.T.);
#6107=EDGE_CURVE('',#4664,#4660,#2917,.T.);
#6108=EDGE_CURVE('',#4665,#4666,#3687,.T.);
#6109=EDGE_CURVE('',#4666,#4667,#2918,.T.);
#6110=EDGE_CURVE('',#4668,#4667,#2223,.T.);
#6111=EDGE_CURVE('',#4668,#4665,#2919,.T.);
#6112=EDGE_CURVE('',#4669,#4670,#3688,.T.);
#6113=EDGE_CURVE('',#4670,#4666,#2920,.T.);
#6114=EDGE_CURVE('',#4665,#4671,#2921,.T.);
#6115=EDGE_CURVE('',#4671,#4669,#2922,.T.);
#6116=EDGE_CURVE('',#4672,#4673,#3689,.T.);
#6117=EDGE_CURVE('',#4673,#4674,#2923,.T.);
#6118=EDGE_CURVE('',#4674,#4670,#2924,.T.);
#6119=EDGE_CURVE('',#4669,#4675,#2925,.T.);
#6120=EDGE_CURVE('',#4675,#4672,#2926,.T.);
#6121=EDGE_CURVE('',#4676,#4677,#3690,.T.);
#6122=EDGE_CURVE('',#4677,#4678,#2927,.T.);
#6123=EDGE_CURVE('',#4678,#4673,#2928,.T.);
#6124=EDGE_CURVE('',#4672,#4679,#2929,.T.);
#6125=EDGE_CURVE('',#4679,#4676,#2930,.T.);
#6126=EDGE_CURVE('',#4680,#4681,#3691,.T.);
#6127=EDGE_CURVE('',#4681,#4682,#2931,.T.);
#6128=EDGE_CURVE('',#4682,#4677,#2932,.T.);
#6129=EDGE_CURVE('',#4676,#4683,#2933,.T.);
#6130=EDGE_CURVE('',#4683,#4680,#2934,.T.);
#6131=EDGE_CURVE('',#4684,#4685,#3692,.T.);
#6132=EDGE_CURVE('',#4685,#4686,#2935,.T.);
#6133=EDGE_CURVE('',#4686,#4681,#2936,.T.);
#6134=EDGE_CURVE('',#4680,#4687,#2937,.T.);
#6135=EDGE_CURVE('',#4687,#4684,#2938,.T.);
#6136=EDGE_CURVE('',#4688,#4689,#3693,.T.);
#6137=EDGE_CURVE('',#4689,#4690,#2939,.T.);
#6138=EDGE_CURVE('',#4690,#4685,#2940,.T.);
#6139=EDGE_CURVE('',#4684,#4691,#2941,.T.);
#6140=EDGE_CURVE('',#4691,#4688,#2942,.T.);
#6141=EDGE_CURVE('',#4692,#4693,#3694,.T.);
#6142=EDGE_CURVE('',#4693,#4689,#2943,.T.);
#6143=EDGE_CURVE('',#4688,#4694,#2944,.T.);
#6144=EDGE_CURVE('',#4694,#4692,#2945,.T.);
#6145=EDGE_CURVE('',#4695,#4696,#3695,.T.);
#6146=EDGE_CURVE('',#4696,#4697,#2946,.T.);
#6147=EDGE_CURVE('',#4697,#4693,#2947,.T.);
#6148=EDGE_CURVE('',#4692,#4698,#2948,.T.);
#6149=EDGE_CURVE('',#4698,#4695,#2949,.T.);
#6150=EDGE_CURVE('',#4699,#4700,#3696,.T.);
#6151=EDGE_CURVE('',#4700,#4701,#2950,.T.);
#6152=EDGE_CURVE('',#4701,#4696,#2951,.T.);
#6153=EDGE_CURVE('',#4695,#4699,#2952,.T.);
#6154=EDGE_CURVE('',#4702,#4703,#3697,.T.);
#6155=EDGE_CURVE('',#4703,#4700,#2953,.T.);
#6156=EDGE_CURVE('',#4699,#4704,#2954,.T.);
#6157=EDGE_CURVE('',#4704,#4702,#2955,.T.);
#6158=EDGE_CURVE('',#4705,#4706,#3698,.T.);
#6159=EDGE_CURVE('',#4705,#4707,#2956,.T.);
#6160=EDGE_CURVE('',#4707,#4708,#2957,.T.);
#6161=EDGE_CURVE('',#4709,#4708,#2224,.F.);
#6162=EDGE_CURVE('',#4709,#4706,#2958,.T.);
#6163=EDGE_CURVE('',#4706,#4710,#2959,.T.);
#6164=EDGE_CURVE('',#4710,#4703,#2960,.T.);
#6165=EDGE_CURVE('',#4702,#4711,#2961,.T.);
#6166=EDGE_CURVE('',#4711,#4705,#2962,.T.);
#6167=EDGE_CURVE('',#4660,#4712,#2963,.T.);
#6168=EDGE_CURVE('',#4712,#4656,#2964,.T.);
#6169=EDGE_CURVE('',#4713,#4655,#2965,.T.);
#6170=EDGE_CURVE('',#4659,#4713,#2966,.T.);
#6171=EDGE_CURVE('',#4617,#4668,#2967,.T.);
#6172=EDGE_CURVE('',#4708,#4663,#2968,.T.);
#6173=EDGE_CURVE('',#4667,#4618,#2969,.T.);
#6174=EDGE_CURVE('',#4714,#4709,#2970,.T.);
#6175=EDGE_CURVE('',#4662,#4714,#2971,.T.);
#6176=EDGE_CURVE('',#4715,#4716,#2225,.T.);
#6177=EDGE_CURVE('',#4716,#4717,#3699,.T.);
#6178=EDGE_CURVE('',#4717,#4718,#2226,.T.);
#6179=EDGE_CURVE('',#4718,#4719,#3700,.T.);
#6180=EDGE_CURVE('',#4719,#4720,#2227,.T.);
#6181=EDGE_CURVE('',#4720,#4721,#3701,.T.);
#6182=EDGE_CURVE('',#4721,#4722,#2228,.T.);
#6183=EDGE_CURVE('',#4722,#4723,#3702,.T.);
#6184=EDGE_CURVE('',#4723,#4724,#2229,.T.);
#6185=EDGE_CURVE('',#4724,#4725,#3703,.T.);
#6186=EDGE_CURVE('',#4725,#4726,#2230,.T.);
#6187=EDGE_CURVE('',#4726,#4727,#3704,.T.);
#6188=EDGE_CURVE('',#4727,#4728,#2231,.T.);
#6189=EDGE_CURVE('',#4728,#4729,#3705,.T.);
#6190=EDGE_CURVE('',#4729,#4730,#2232,.T.);
#6191=EDGE_CURVE('',#4730,#4731,#3706,.T.);
#6192=EDGE_CURVE('',#4731,#4732,#2233,.T.);
#6193=EDGE_CURVE('',#4732,#4733,#3707,.T.);
#6194=EDGE_CURVE('',#4733,#4734,#2234,.T.);
#6195=EDGE_CURVE('',#4734,#4735,#3708,.T.);
#6196=EDGE_CURVE('',#4735,#4736,#2235,.T.);
#6197=EDGE_CURVE('',#4736,#4737,#3709,.T.);
#6198=EDGE_CURVE('',#4737,#4738,#2236,.T.);
#6199=EDGE_CURVE('',#4738,#4739,#3710,.T.);
#6200=EDGE_CURVE('',#4739,#4740,#2237,.T.);
#6201=EDGE_CURVE('',#4740,#4741,#3711,.T.);
#6202=EDGE_CURVE('',#4741,#4742,#2238,.T.);
#6203=EDGE_CURVE('',#4742,#4743,#3712,.T.);
#6204=EDGE_CURVE('',#4743,#4744,#2239,.T.);
#6205=EDGE_CURVE('',#4744,#4745,#3713,.T.);
#6206=EDGE_CURVE('',#4745,#4746,#2240,.T.);
#6207=EDGE_CURVE('',#4746,#4747,#3714,.T.);
#6208=EDGE_CURVE('',#4747,#4748,#2241,.T.);
#6209=EDGE_CURVE('',#4748,#4749,#3715,.T.);
#6210=EDGE_CURVE('',#4749,#4750,#2242,.T.);
#6211=EDGE_CURVE('',#4750,#4751,#3716,.T.);
#6212=EDGE_CURVE('',#4751,#4752,#2243,.T.);
#6213=EDGE_CURVE('',#4752,#4753,#3717,.T.);
#6214=EDGE_CURVE('',#4753,#4754,#2244,.T.);
#6215=EDGE_CURVE('',#4754,#4755,#3718,.T.);
#6216=EDGE_CURVE('',#4755,#4756,#2245,.T.);
#6217=EDGE_CURVE('',#4756,#4757,#3719,.T.);
#6218=EDGE_CURVE('',#4757,#4758,#2246,.T.);
#6219=EDGE_CURVE('',#4758,#4759,#3720,.T.);
#6220=EDGE_CURVE('',#4759,#4760,#2247,.T.);
#6221=EDGE_CURVE('',#4760,#4761,#3721,.T.);
#6222=EDGE_CURVE('',#4761,#4762,#2248,.T.);
#6223=EDGE_CURVE('',#4762,#4763,#3722,.T.);
#6224=EDGE_CURVE('',#4763,#4764,#2249,.T.);
#6225=EDGE_CURVE('',#4764,#4765,#3723,.T.);
#6226=EDGE_CURVE('',#4765,#4766,#2250,.T.);
#6227=EDGE_CURVE('',#4766,#4767,#3724,.T.);
#6228=EDGE_CURVE('',#4767,#4768,#2251,.T.);
#6229=EDGE_CURVE('',#4768,#4769,#3725,.T.);
#6230=EDGE_CURVE('',#4769,#4770,#2252,.T.);
#6231=EDGE_CURVE('',#4770,#4771,#3726,.T.);
#6232=EDGE_CURVE('',#4771,#4772,#2253,.T.);
#6233=EDGE_CURVE('',#4772,#4773,#3727,.T.);
#6234=EDGE_CURVE('',#4773,#4774,#2254,.T.);
#6235=EDGE_CURVE('',#4774,#4775,#3728,.T.);
#6236=EDGE_CURVE('',#4775,#4776,#2255,.T.);
#6237=EDGE_CURVE('',#4776,#4777,#3729,.T.);
#6238=EDGE_CURVE('',#4777,#4778,#2256,.T.);
#6239=EDGE_CURVE('',#4778,#4779,#3730,.T.);
#6240=EDGE_CURVE('',#4779,#4780,#2257,.T.);
#6241=EDGE_CURVE('',#4780,#4781,#3731,.T.);
#6242=EDGE_CURVE('',#4781,#4782,#2258,.T.);
#6243=EDGE_CURVE('',#4782,#4783,#3732,.T.);
#6244=EDGE_CURVE('',#4783,#4784,#2259,.T.);
#6245=EDGE_CURVE('',#4784,#4785,#3733,.T.);
#6246=EDGE_CURVE('',#4785,#4786,#2260,.T.);
#6247=EDGE_CURVE('',#4786,#4715,#3734,.T.);
#6248=EDGE_CURVE('',#4787,#4788,#3735,.T.);
#6249=EDGE_CURVE('',#4789,#4787,#2261,.T.);
#6250=EDGE_CURVE('',#4790,#4789,#3736,.T.);
#6251=EDGE_CURVE('',#4788,#4790,#2262,.T.);
#6252=EDGE_CURVE('',#4791,#4792,#3737,.T.);
#6253=EDGE_CURVE('',#4793,#4791,#2263,.T.);
#6254=EDGE_CURVE('',#4794,#4793,#3738,.T.);
#6255=EDGE_CURVE('',#4792,#4794,#2264,.T.);
#6256=EDGE_CURVE('',#4795,#4796,#3739,.T.);
#6257=EDGE_CURVE('',#4797,#4795,#2265,.T.);
#6258=EDGE_CURVE('',#4798,#4797,#3740,.T.);
#6259=EDGE_CURVE('',#4796,#4798,#2266,.T.);
#6260=EDGE_CURVE('',#4799,#4800,#3741,.T.);
#6261=EDGE_CURVE('',#4801,#4799,#2267,.T.);
#6262=EDGE_CURVE('',#4802,#4801,#3742,.T.);
#6263=EDGE_CURVE('',#4800,#4802,#2268,.T.);
#6264=EDGE_CURVE('',#4803,#4804,#3743,.T.);
#6265=EDGE_CURVE('',#4805,#4803,#2269,.T.);
#6266=EDGE_CURVE('',#4806,#4805,#3744,.T.);
#6267=EDGE_CURVE('',#4804,#4806,#2270,.T.);
#6268=EDGE_CURVE('',#4807,#4808,#3745,.T.);
#6269=EDGE_CURVE('',#4809,#4807,#2271,.T.);
#6270=EDGE_CURVE('',#4810,#4809,#3746,.T.);
#6271=EDGE_CURVE('',#4808,#4810,#2272,.T.);
#6272=EDGE_CURVE('',#4811,#4812,#3747,.T.);
#6273=EDGE_CURVE('',#4813,#4811,#2273,.T.);
#6274=EDGE_CURVE('',#4814,#4813,#3748,.T.);
#6275=EDGE_CURVE('',#4812,#4814,#2274,.T.);
#6276=EDGE_CURVE('',#4815,#4816,#3749,.T.);
#6277=EDGE_CURVE('',#4817,#4815,#2275,.T.);
#6278=EDGE_CURVE('',#4818,#4817,#3750,.T.);
#6279=EDGE_CURVE('',#4816,#4818,#2276,.T.);
#6280=EDGE_CURVE('',#4819,#4820,#3751,.T.);
#6281=EDGE_CURVE('',#4821,#4819,#2277,.T.);
#6282=EDGE_CURVE('',#4822,#4821,#3752,.T.);
#6283=EDGE_CURVE('',#4820,#4822,#2278,.T.);
#6284=EDGE_CURVE('',#4823,#4824,#3753,.T.);
#6285=EDGE_CURVE('',#4825,#4823,#2279,.T.);
#6286=EDGE_CURVE('',#4826,#4825,#3754,.T.);
#6287=EDGE_CURVE('',#4824,#4826,#2280,.T.);
#6288=EDGE_CURVE('',#4827,#4828,#3755,.T.);
#6289=EDGE_CURVE('',#4829,#4827,#2281,.T.);
#6290=EDGE_CURVE('',#4830,#4829,#3756,.T.);
#6291=EDGE_CURVE('',#4828,#4830,#2282,.T.);
#6292=EDGE_CURVE('',#4831,#4832,#3757,.T.);
#6293=EDGE_CURVE('',#4833,#4831,#2283,.T.);
#6294=EDGE_CURVE('',#4834,#4833,#3758,.T.);
#6295=EDGE_CURVE('',#4832,#4834,#2284,.T.);
#6296=EDGE_CURVE('',#4835,#4836,#3759,.T.);
#6297=EDGE_CURVE('',#4837,#4835,#2285,.T.);
#6298=EDGE_CURVE('',#4838,#4837,#3760,.T.);
#6299=EDGE_CURVE('',#4836,#4838,#2286,.T.);
#6300=EDGE_CURVE('',#4839,#4840,#3761,.T.);
#6301=EDGE_CURVE('',#4841,#4839,#2287,.T.);
#6302=EDGE_CURVE('',#4842,#4841,#3762,.T.);
#6303=EDGE_CURVE('',#4840,#4842,#2288,.T.);
#6304=EDGE_CURVE('',#4843,#4844,#3763,.T.);
#6305=EDGE_CURVE('',#4845,#4843,#2289,.T.);
#6306=EDGE_CURVE('',#4846,#4845,#3764,.T.);
#6307=EDGE_CURVE('',#4844,#4846,#2290,.T.);
#6308=EDGE_CURVE('',#4847,#4848,#3765,.T.);
#6309=EDGE_CURVE('',#4849,#4847,#2291,.T.);
#6310=EDGE_CURVE('',#4850,#4849,#3766,.T.);
#6311=EDGE_CURVE('',#4848,#4850,#2292,.T.);
#6312=EDGE_CURVE('',#4851,#4852,#3767,.T.);
#6313=EDGE_CURVE('',#4853,#4851,#2293,.T.);
#6314=EDGE_CURVE('',#4854,#4853,#3768,.T.);
#6315=EDGE_CURVE('',#4852,#4854,#2294,.T.);
#6316=EDGE_CURVE('',#4855,#4856,#3769,.T.);
#6317=EDGE_CURVE('',#4857,#4855,#2295,.T.);
#6318=EDGE_CURVE('',#4858,#4857,#3770,.T.);
#6319=EDGE_CURVE('',#4856,#4858,#2296,.T.);
#6320=EDGE_CURVE('',#4724,#4859,#2297,.T.);
#6321=EDGE_CURVE('',#4860,#4723,#2298,.T.);
#6322=EDGE_CURVE('',#4861,#4860,#3771,.T.);
#6323=EDGE_CURVE('',#4849,#4861,#2972,.T.);
#6324=EDGE_CURVE('',#4862,#4847,#2973,.T.);
#6325=EDGE_CURVE('',#4859,#4862,#3772,.T.);
#6326=EDGE_CURVE('',#4728,#4863,#2299,.T.);
#6327=EDGE_CURVE('',#4864,#4727,#2300,.T.);
#6328=EDGE_CURVE('',#4865,#4864,#3773,.T.);
#6329=EDGE_CURVE('',#4845,#4865,#2974,.T.);
#6330=EDGE_CURVE('',#4866,#4843,#2975,.T.);
#6331=EDGE_CURVE('',#4863,#4866,#3774,.T.);
#6332=EDGE_CURVE('',#4732,#4867,#2301,.T.);
#6333=EDGE_CURVE('',#4868,#4731,#2302,.T.);
#6334=EDGE_CURVE('',#4869,#4868,#3775,.T.);
#6335=EDGE_CURVE('',#4841,#4869,#2976,.T.);
#6336=EDGE_CURVE('',#4870,#4839,#2977,.T.);
#6337=EDGE_CURVE('',#4867,#4870,#3776,.T.);
#6338=EDGE_CURVE('',#4736,#4871,#2303,.T.);
#6339=EDGE_CURVE('',#4872,#4735,#2304,.T.);
#6340=EDGE_CURVE('',#4873,#4872,#3777,.T.);
#6341=EDGE_CURVE('',#4837,#4873,#2978,.T.);
#6342=EDGE_CURVE('',#4874,#4835,#2979,.T.);
#6343=EDGE_CURVE('',#4871,#4874,#3778,.T.);
#6344=EDGE_CURVE('',#4740,#4875,#2305,.T.);
#6345=EDGE_CURVE('',#4876,#4739,#2306,.T.);
#6346=EDGE_CURVE('',#4877,#4876,#3779,.T.);
#6347=EDGE_CURVE('',#4833,#4877,#2980,.T.);
#6348=EDGE_CURVE('',#4878,#4831,#2981,.T.);
#6349=EDGE_CURVE('',#4875,#4878,#3780,.T.);
#6350=EDGE_CURVE('',#4744,#4879,#2307,.T.);
#6351=EDGE_CURVE('',#4880,#4743,#2308,.T.);
#6352=EDGE_CURVE('',#4881,#4880,#3781,.T.);
#6353=EDGE_CURVE('',#4829,#4881,#2982,.T.);
#6354=EDGE_CURVE('',#4882,#4827,#2983,.T.);
#6355=EDGE_CURVE('',#4879,#4882,#3782,.T.);
#6356=EDGE_CURVE('',#4748,#4883,#2309,.T.);
#6357=EDGE_CURVE('',#4884,#4747,#2310,.T.);
#6358=EDGE_CURVE('',#4885,#4884,#3783,.T.);
#6359=EDGE_CURVE('',#4825,#4885,#2984,.T.);
#6360=EDGE_CURVE('',#4886,#4823,#2985,.T.);
#6361=EDGE_CURVE('',#4883,#4886,#3784,.T.);
#6362=EDGE_CURVE('',#4752,#4887,#2311,.T.);
#6363=EDGE_CURVE('',#4888,#4751,#2312,.T.);
#6364=EDGE_CURVE('',#4889,#4888,#3785,.T.);
#6365=EDGE_CURVE('',#4821,#4889,#2986,.T.);
#6366=EDGE_CURVE('',#4890,#4819,#2987,.T.);
#6367=EDGE_CURVE('',#4887,#4890,#3786,.T.);
#6368=EDGE_CURVE('',#4756,#4891,#2313,.T.);
#6369=EDGE_CURVE('',#4892,#4755,#2314,.T.);
#6370=EDGE_CURVE('',#4893,#4892,#3787,.T.);
#6371=EDGE_CURVE('',#4817,#4893,#2988,.T.);
#6372=EDGE_CURVE('',#4894,#4815,#2989,.T.);
#6373=EDGE_CURVE('',#4891,#4894,#3788,.T.);
#6374=EDGE_CURVE('',#4760,#4895,#2315,.T.);
#6375=EDGE_CURVE('',#4896,#4759,#2316,.T.);
#6376=EDGE_CURVE('',#4897,#4896,#3789,.T.);
#6377=EDGE_CURVE('',#4813,#4897,#2990,.T.);
#6378=EDGE_CURVE('',#4898,#4811,#2991,.T.);
#6379=EDGE_CURVE('',#4895,#4898,#3790,.T.);
#6380=EDGE_CURVE('',#4764,#4899,#2317,.T.);
#6381=EDGE_CURVE('',#4900,#4763,#2318,.T.);
#6382=EDGE_CURVE('',#4901,#4900,#3791,.T.);
#6383=EDGE_CURVE('',#4809,#4901,#2992,.T.);
#6384=EDGE_CURVE('',#4902,#4807,#2993,.T.);
#6385=EDGE_CURVE('',#4899,#4902,#3792,.T.);
#6386=EDGE_CURVE('',#4768,#4903,#2319,.T.);
#6387=EDGE_CURVE('',#4904,#4767,#2320,.T.);
#6388=EDGE_CURVE('',#4905,#4904,#3793,.T.);
#6389=EDGE_CURVE('',#4805,#4905,#2994,.T.);
#6390=EDGE_CURVE('',#4906,#4803,#2995,.T.);
#6391=EDGE_CURVE('',#4903,#4906,#3794,.T.);
#6392=EDGE_CURVE('',#4772,#4907,#2321,.T.);
#6393=EDGE_CURVE('',#4908,#4771,#2322,.T.);
#6394=EDGE_CURVE('',#4909,#4908,#3795,.T.);
#6395=EDGE_CURVE('',#4801,#4909,#2996,.T.);
#6396=EDGE_CURVE('',#4910,#4799,#2997,.T.);
#6397=EDGE_CURVE('',#4907,#4910,#3796,.T.);
#6398=EDGE_CURVE('',#4776,#4911,#2323,.T.);
#6399=EDGE_CURVE('',#4912,#4775,#2324,.T.);
#6400=EDGE_CURVE('',#4913,#4912,#3797,.T.);
#6401=EDGE_CURVE('',#4797,#4913,#2998,.T.);
#6402=EDGE_CURVE('',#4914,#4795,#2999,.T.);
#6403=EDGE_CURVE('',#4911,#4914,#3798,.T.);
#6404=EDGE_CURVE('',#4780,#4915,#2325,.T.);
#6405=EDGE_CURVE('',#4916,#4779,#2326,.T.);
#6406=EDGE_CURVE('',#4917,#4916,#3799,.T.);
#6407=EDGE_CURVE('',#4793,#4917,#3000,.T.);
#6408=EDGE_CURVE('',#4918,#4791,#3001,.T.);
#6409=EDGE_CURVE('',#4915,#4918,#3800,.T.);
#6410=EDGE_CURVE('',#4784,#4919,#2327,.T.);
#6411=EDGE_CURVE('',#4920,#4783,#2328,.T.);
#6412=EDGE_CURVE('',#4921,#4920,#3801,.T.);
#6413=EDGE_CURVE('',#4789,#4921,#3002,.T.);
#6414=EDGE_CURVE('',#4922,#4787,#3003,.T.);
#6415=EDGE_CURVE('',#4919,#4922,#3802,.T.);
#6416=EDGE_CURVE('',#4720,#4923,#2329,.T.);
#6417=EDGE_CURVE('',#4924,#4719,#2330,.T.);
#6418=EDGE_CURVE('',#4925,#4924,#3803,.T.);
#6419=EDGE_CURVE('',#4853,#4925,#3004,.T.);
#6420=EDGE_CURVE('',#4926,#4851,#3005,.T.);
#6421=EDGE_CURVE('',#4923,#4926,#3804,.T.);
#6422=EDGE_CURVE('',#4716,#4927,#2331,.T.);
#6423=EDGE_CURVE('',#4928,#4715,#2332,.T.);
#6424=EDGE_CURVE('',#4929,#4928,#3805,.T.);
#6425=EDGE_CURVE('',#4857,#4929,#3006,.T.);
#6426=EDGE_CURVE('',#4930,#4855,#3007,.T.);
#6427=EDGE_CURVE('',#4927,#4930,#3806,.T.);
#6428=EDGE_CURVE('',#4931,#4932,#2333,.T.);
#6429=EDGE_CURVE('',#4933,#4931,#2334,.T.);
#6430=EDGE_CURVE('',#4934,#4933,#2335,.T.);
#6431=EDGE_CURVE('',#4935,#4934,#3807,.T.);
#6432=EDGE_CURVE('',#4936,#4935,#3008,.T.);
#6433=EDGE_CURVE('',#4937,#4936,#2336,.T.);
#6434=EDGE_CURVE('',#4938,#4937,#3009,.T.);
#6435=EDGE_CURVE('',#4932,#4938,#3808,.T.);
#6436=EDGE_CURVE('',#4939,#4940,#2337,.T.);
#6437=EDGE_CURVE('',#4941,#4939,#2338,.T.);
#6438=EDGE_CURVE('',#4942,#4941,#2339,.T.);
#6439=EDGE_CURVE('',#4943,#4942,#3809,.T.);
#6440=EDGE_CURVE('',#4944,#4943,#3010,.T.);
#6441=EDGE_CURVE('',#4945,#4944,#2340,.T.);
#6442=EDGE_CURVE('',#4946,#4945,#3011,.T.);
#6443=EDGE_CURVE('',#4940,#4946,#3810,.T.);
#6444=EDGE_CURVE('',#4947,#4948,#2341,.T.);
#6445=EDGE_CURVE('',#4949,#4947,#2342,.T.);
#6446=EDGE_CURVE('',#4950,#4949,#2343,.T.);
#6447=EDGE_CURVE('',#4951,#4950,#3811,.T.);
#6448=EDGE_CURVE('',#4952,#4951,#3012,.T.);
#6449=EDGE_CURVE('',#4953,#4952,#2344,.T.);
#6450=EDGE_CURVE('',#4954,#4953,#3013,.T.);
#6451=EDGE_CURVE('',#4948,#4954,#3812,.T.);
#6452=EDGE_CURVE('',#4955,#4956,#2345,.T.);
#6453=EDGE_CURVE('',#4957,#4955,#2346,.T.);
#6454=EDGE_CURVE('',#4958,#4957,#2347,.T.);
#6455=EDGE_CURVE('',#4959,#4958,#3813,.T.);
#6456=EDGE_CURVE('',#4960,#4959,#3014,.T.);
#6457=EDGE_CURVE('',#4961,#4960,#2348,.T.);
#6458=EDGE_CURVE('',#4962,#4961,#3015,.T.);
#6459=EDGE_CURVE('',#4956,#4962,#3814,.T.);
#6460=EDGE_CURVE('',#4963,#4964,#2349,.T.);
#6461=EDGE_CURVE('',#4965,#4963,#2350,.T.);
#6462=EDGE_CURVE('',#4966,#4965,#2351,.T.);
#6463=EDGE_CURVE('',#4967,#4966,#3815,.T.);
#6464=EDGE_CURVE('',#4968,#4967,#3016,.T.);
#6465=EDGE_CURVE('',#4969,#4968,#2352,.T.);
#6466=EDGE_CURVE('',#4970,#4969,#3017,.T.);
#6467=EDGE_CURVE('',#4964,#4970,#3816,.T.);
#6468=EDGE_CURVE('',#4971,#4972,#2353,.T.);
#6469=EDGE_CURVE('',#4973,#4971,#2354,.T.);
#6470=EDGE_CURVE('',#4974,#4973,#2355,.T.);
#6471=EDGE_CURVE('',#4975,#4974,#3817,.T.);
#6472=EDGE_CURVE('',#4976,#4975,#3018,.T.);
#6473=EDGE_CURVE('',#4977,#4976,#2356,.T.);
#6474=EDGE_CURVE('',#4978,#4977,#3019,.T.);
#6475=EDGE_CURVE('',#4972,#4978,#3818,.T.);
#6476=EDGE_CURVE('',#4979,#4980,#2357,.T.);
#6477=EDGE_CURVE('',#4981,#4979,#2358,.T.);
#6478=EDGE_CURVE('',#4982,#4981,#2359,.T.);
#6479=EDGE_CURVE('',#4983,#4982,#3819,.T.);
#6480=EDGE_CURVE('',#4984,#4983,#3020,.T.);
#6481=EDGE_CURVE('',#4985,#4984,#2360,.T.);
#6482=EDGE_CURVE('',#4986,#4985,#3021,.T.);
#6483=EDGE_CURVE('',#4980,#4986,#3820,.T.);
#6484=EDGE_CURVE('',#4987,#4988,#2361,.T.);
#6485=EDGE_CURVE('',#4989,#4987,#2362,.T.);
#6486=EDGE_CURVE('',#4990,#4989,#2363,.T.);
#6487=EDGE_CURVE('',#4991,#4990,#3821,.T.);
#6488=EDGE_CURVE('',#4992,#4991,#3022,.T.);
#6489=EDGE_CURVE('',#4993,#4992,#2364,.T.);
#6490=EDGE_CURVE('',#4994,#4993,#3023,.T.);
#6491=EDGE_CURVE('',#4988,#4994,#3822,.T.);
#6492=EDGE_CURVE('',#4995,#4996,#2365,.T.);
#6493=EDGE_CURVE('',#4997,#4995,#2366,.T.);
#6494=EDGE_CURVE('',#4998,#4997,#2367,.T.);
#6495=EDGE_CURVE('',#4999,#4998,#3823,.T.);
#6496=EDGE_CURVE('',#5000,#4999,#3024,.T.);
#6497=EDGE_CURVE('',#5001,#5000,#2368,.T.);
#6498=EDGE_CURVE('',#5002,#5001,#3025,.T.);
#6499=EDGE_CURVE('',#4996,#5002,#3824,.T.);
#6500=EDGE_CURVE('',#5003,#5004,#2369,.T.);
#6501=EDGE_CURVE('',#5005,#5003,#2370,.T.);
#6502=EDGE_CURVE('',#5006,#5005,#2371,.T.);
#6503=EDGE_CURVE('',#5007,#5006,#3825,.T.);
#6504=EDGE_CURVE('',#5008,#5007,#3026,.T.);
#6505=EDGE_CURVE('',#5009,#5008,#2372,.T.);
#6506=EDGE_CURVE('',#5010,#5009,#3027,.T.);
#6507=EDGE_CURVE('',#5004,#5010,#3826,.T.);
#6508=EDGE_CURVE('',#5011,#5012,#2373,.T.);
#6509=EDGE_CURVE('',#5013,#5011,#2374,.T.);
#6510=EDGE_CURVE('',#5014,#5013,#2375,.T.);
#6511=EDGE_CURVE('',#5015,#5014,#3827,.T.);
#6512=EDGE_CURVE('',#5016,#5015,#3028,.T.);
#6513=EDGE_CURVE('',#5017,#5016,#2376,.T.);
#6514=EDGE_CURVE('',#5018,#5017,#3029,.T.);
#6515=EDGE_CURVE('',#5012,#5018,#3828,.T.);
#6516=EDGE_CURVE('',#5019,#5020,#2377,.T.);
#6517=EDGE_CURVE('',#5021,#5019,#2378,.T.);
#6518=EDGE_CURVE('',#5022,#5021,#2379,.T.);
#6519=EDGE_CURVE('',#5023,#5022,#3829,.T.);
#6520=EDGE_CURVE('',#5024,#5023,#3030,.T.);
#6521=EDGE_CURVE('',#5025,#5024,#2380,.T.);
#6522=EDGE_CURVE('',#5026,#5025,#3031,.T.);
#6523=EDGE_CURVE('',#5020,#5026,#3830,.T.);
#6524=EDGE_CURVE('',#5027,#5028,#2381,.T.);
#6525=EDGE_CURVE('',#5029,#5027,#2382,.T.);
#6526=EDGE_CURVE('',#5030,#5029,#2383,.T.);
#6527=EDGE_CURVE('',#5031,#5030,#3831,.T.);
#6528=EDGE_CURVE('',#5032,#5031,#3032,.T.);
#6529=EDGE_CURVE('',#5033,#5032,#2384,.T.);
#6530=EDGE_CURVE('',#5034,#5033,#3033,.T.);
#6531=EDGE_CURVE('',#5028,#5034,#3832,.T.);
#6532=EDGE_CURVE('',#5035,#5036,#2385,.T.);
#6533=EDGE_CURVE('',#5037,#5035,#2386,.T.);
#6534=EDGE_CURVE('',#5038,#5037,#2387,.T.);
#6535=EDGE_CURVE('',#5039,#5038,#3833,.T.);
#6536=EDGE_CURVE('',#5040,#5039,#3034,.T.);
#6537=EDGE_CURVE('',#5041,#5040,#2388,.T.);
#6538=EDGE_CURVE('',#5042,#5041,#3035,.T.);
#6539=EDGE_CURVE('',#5036,#5042,#3834,.T.);
#6540=EDGE_CURVE('',#5043,#5044,#2389,.T.);
#6541=EDGE_CURVE('',#5045,#5043,#2390,.T.);
#6542=EDGE_CURVE('',#5046,#5045,#2391,.T.);
#6543=EDGE_CURVE('',#5047,#5046,#3835,.T.);
#6544=EDGE_CURVE('',#5048,#5047,#3036,.T.);
#6545=EDGE_CURVE('',#5049,#5048,#2392,.T.);
#6546=EDGE_CURVE('',#5050,#5049,#3037,.T.);
#6547=EDGE_CURVE('',#5044,#5050,#3836,.T.);
#6548=EDGE_CURVE('',#5051,#5052,#2393,.T.);
#6549=EDGE_CURVE('',#5053,#5051,#2394,.T.);
#6550=EDGE_CURVE('',#5054,#5053,#2395,.T.);
#6551=EDGE_CURVE('',#5055,#5054,#3837,.T.);
#6552=EDGE_CURVE('',#5056,#5055,#3038,.T.);
#6553=EDGE_CURVE('',#5057,#5056,#2396,.T.);
#6554=EDGE_CURVE('',#5058,#5057,#3039,.T.);
#6555=EDGE_CURVE('',#5052,#5058,#3838,.T.);
#6556=EDGE_CURVE('',#5059,#5060,#2397,.T.);
#6557=EDGE_CURVE('',#5061,#5059,#2398,.T.);
#6558=EDGE_CURVE('',#5062,#5061,#2399,.T.);
#6559=EDGE_CURVE('',#5063,#5062,#3839,.T.);
#6560=EDGE_CURVE('',#5064,#5063,#3040,.T.);
#6561=EDGE_CURVE('',#5065,#5064,#2400,.T.);
#6562=EDGE_CURVE('',#5066,#5065,#3041,.T.);
#6563=EDGE_CURVE('',#5060,#5066,#3840,.T.);
#6564=EDGE_CURVE('',#5067,#5068,#2401,.T.);
#6565=EDGE_CURVE('',#5069,#5067,#2402,.T.);
#6566=EDGE_CURVE('',#5070,#5069,#2403,.T.);
#6567=EDGE_CURVE('',#5071,#5070,#3841,.T.);
#6568=EDGE_CURVE('',#5072,#5071,#3042,.T.);
#6569=EDGE_CURVE('',#5073,#5072,#2404,.T.);
#6570=EDGE_CURVE('',#5074,#5073,#3043,.T.);
#6571=EDGE_CURVE('',#5068,#5074,#3842,.T.);
#6572=EDGE_CURVE('',#4937,#5075,#3843,.T.);
#6573=EDGE_CURVE('',#5076,#4936,#3844,.T.);
#6574=EDGE_CURVE('',#5075,#5076,#2405,.T.);
#6575=EDGE_CURVE('',#4945,#5077,#3845,.T.);
#6576=EDGE_CURVE('',#5078,#4944,#3846,.T.);
#6577=EDGE_CURVE('',#5077,#5078,#2406,.T.);
#6578=EDGE_CURVE('',#4953,#5079,#3847,.T.);
#6579=EDGE_CURVE('',#5080,#4952,#3848,.T.);
#6580=EDGE_CURVE('',#5079,#5080,#2407,.T.);
#6581=EDGE_CURVE('',#4961,#5081,#3849,.T.);
#6582=EDGE_CURVE('',#5082,#4960,#3850,.T.);
#6583=EDGE_CURVE('',#5081,#5082,#2408,.T.);
#6584=EDGE_CURVE('',#4969,#5083,#3851,.T.);
#6585=EDGE_CURVE('',#5084,#4968,#3852,.T.);
#6586=EDGE_CURVE('',#5083,#5084,#2409,.T.);
#6587=EDGE_CURVE('',#4977,#5085,#3853,.T.);
#6588=EDGE_CURVE('',#5086,#4976,#3854,.T.);
#6589=EDGE_CURVE('',#5085,#5086,#2410,.T.);
#6590=EDGE_CURVE('',#4985,#5087,#3855,.T.);
#6591=EDGE_CURVE('',#5088,#4984,#3856,.T.);
#6592=EDGE_CURVE('',#5087,#5088,#2411,.T.);
#6593=EDGE_CURVE('',#4993,#5089,#3857,.T.);
#6594=EDGE_CURVE('',#5090,#4992,#3858,.T.);
#6595=EDGE_CURVE('',#5089,#5090,#2412,.T.);
#6596=EDGE_CURVE('',#5001,#5091,#3859,.T.);
#6597=EDGE_CURVE('',#5092,#5000,#3860,.T.);
#6598=EDGE_CURVE('',#5091,#5092,#2413,.T.);
#6599=EDGE_CURVE('',#5009,#5093,#3861,.T.);
#6600=EDGE_CURVE('',#5094,#5008,#3862,.T.);
#6601=EDGE_CURVE('',#5093,#5094,#2414,.T.);
#6602=EDGE_CURVE('',#5017,#5095,#3863,.T.);
#6603=EDGE_CURVE('',#5096,#5016,#3864,.T.);
#6604=EDGE_CURVE('',#5095,#5096,#2415,.T.);
#6605=EDGE_CURVE('',#5025,#5097,#3865,.T.);
#6606=EDGE_CURVE('',#5098,#5024,#3866,.T.);
#6607=EDGE_CURVE('',#5097,#5098,#2416,.T.);
#6608=EDGE_CURVE('',#5033,#5099,#3867,.T.);
#6609=EDGE_CURVE('',#5100,#5032,#3868,.T.);
#6610=EDGE_CURVE('',#5099,#5100,#2417,.T.);
#6611=EDGE_CURVE('',#5041,#5101,#3869,.T.);
#6612=EDGE_CURVE('',#5102,#5040,#3870,.T.);
#6613=EDGE_CURVE('',#5101,#5102,#2418,.T.);
#6614=EDGE_CURVE('',#5049,#5103,#3871,.T.);
#6615=EDGE_CURVE('',#5104,#5048,#3872,.T.);
#6616=EDGE_CURVE('',#5103,#5104,#2419,.T.);
#6617=EDGE_CURVE('',#5057,#5105,#3873,.T.);
#6618=EDGE_CURVE('',#5106,#5056,#3874,.T.);
#6619=EDGE_CURVE('',#5105,#5106,#2420,.T.);
#6620=EDGE_CURVE('',#5065,#5107,#3875,.T.);
#6621=EDGE_CURVE('',#5108,#5064,#3876,.T.);
#6622=EDGE_CURVE('',#5107,#5108,#2421,.T.);
#6623=EDGE_CURVE('',#5073,#5109,#3877,.T.);
#6624=EDGE_CURVE('',#5110,#5072,#3878,.T.);
#6625=EDGE_CURVE('',#5109,#5110,#2422,.T.);
#6626=EDGE_CURVE('',#5111,#5112,#190,.T.);
#6627=EDGE_CURVE('',#5113,#5111,#2423,.T.);
#6628=EDGE_CURVE('',#5114,#5113,#3044,.T.);
#6629=EDGE_CURVE('',#5112,#5114,#2424,.T.);
#6630=EDGE_CURVE('',#5115,#5116,#191,.T.);
#6631=EDGE_CURVE('',#5117,#5115,#2425,.T.);
#6632=EDGE_CURVE('',#5118,#5117,#192,.T.);
#6633=EDGE_CURVE('',#5116,#5118,#2426,.T.);
#6634=EDGE_CURVE('',#5119,#5120,#193,.T.);
#6635=EDGE_CURVE('',#5121,#5119,#2427,.T.);
#6636=EDGE_CURVE('',#5122,#5121,#194,.T.);
#6637=EDGE_CURVE('',#5120,#5122,#2428,.T.);
#6638=EDGE_CURVE('',#5123,#5124,#195,.T.);
#6639=EDGE_CURVE('',#5125,#5123,#2429,.T.);
#6640=EDGE_CURVE('',#5126,#5125,#3045,.T.);
#6641=EDGE_CURVE('',#5124,#5126,#2430,.T.);
#6642=EDGE_CURVE('',#5127,#5128,#196,.T.);
#6643=EDGE_CURVE('',#5129,#5127,#2431,.T.);
#6644=EDGE_CURVE('',#5130,#5129,#197,.T.);
#6645=EDGE_CURVE('',#5128,#5130,#2432,.T.);
#6646=EDGE_CURVE('',#5131,#5132,#198,.T.);
#6647=EDGE_CURVE('',#5133,#5131,#2433,.T.);
#6648=EDGE_CURVE('',#5134,#5133,#199,.T.);
#6649=EDGE_CURVE('',#5132,#5134,#2434,.T.);
#6650=EDGE_CURVE('',#5135,#5136,#200,.T.);
#6651=EDGE_CURVE('',#5137,#5135,#2435,.T.);
#6652=EDGE_CURVE('',#5138,#5137,#201,.T.);
#6653=EDGE_CURVE('',#5136,#5138,#2436,.T.);
#6654=EDGE_CURVE('',#5139,#5140,#202,.T.);
#6655=EDGE_CURVE('',#5141,#5139,#2437,.T.);
#6656=EDGE_CURVE('',#5142,#5141,#3046,.T.);
#6657=EDGE_CURVE('',#5140,#5142,#2438,.T.);
#6658=EDGE_CURVE('',#5143,#5144,#203,.T.);
#6659=EDGE_CURVE('',#5145,#5143,#2439,.T.);
#6660=EDGE_CURVE('',#5146,#5145,#204,.T.);
#6661=EDGE_CURVE('',#5144,#5146,#2440,.T.);
#6662=EDGE_CURVE('',#5147,#5148,#205,.T.);
#6663=EDGE_CURVE('',#5149,#5147,#2441,.T.);
#6664=EDGE_CURVE('',#5150,#5149,#206,.T.);
#6665=EDGE_CURVE('',#5148,#5150,#2442,.T.);
#6666=EDGE_CURVE('',#5151,#5152,#207,.T.);
#6667=EDGE_CURVE('',#5153,#5151,#2443,.T.);
#6668=EDGE_CURVE('',#5154,#5153,#208,.T.);
#6669=EDGE_CURVE('',#5152,#5154,#2444,.T.);
#6670=EDGE_CURVE('',#5155,#5156,#209,.T.);
#6671=EDGE_CURVE('',#5157,#5155,#2445,.T.);
#6672=EDGE_CURVE('',#5158,#5157,#3047,.T.);
#6673=EDGE_CURVE('',#5156,#5158,#2446,.T.);
#6674=EDGE_CURVE('',#5159,#5160,#210,.T.);
#6675=EDGE_CURVE('',#5161,#5159,#2447,.T.);
#6676=EDGE_CURVE('',#5162,#5161,#211,.T.);
#6677=EDGE_CURVE('',#5160,#5162,#2448,.T.);
#6678=EDGE_CURVE('',#5163,#5164,#212,.T.);
#6679=EDGE_CURVE('',#5165,#5163,#2449,.T.);
#6680=EDGE_CURVE('',#5166,#5165,#213,.T.);
#6681=EDGE_CURVE('',#5164,#5166,#2450,.T.);
#6682=EDGE_CURVE('',#5167,#5168,#214,.T.);
#6683=EDGE_CURVE('',#5169,#5167,#2451,.T.);
#6684=EDGE_CURVE('',#5170,#5169,#215,.T.);
#6685=EDGE_CURVE('',#5168,#5170,#2452,.T.);
#6686=EDGE_CURVE('',#5171,#5172,#216,.T.);
#6687=EDGE_CURVE('',#5173,#5171,#2453,.T.);
#6688=EDGE_CURVE('',#5174,#5173,#217,.T.);
#6689=EDGE_CURVE('',#5172,#5174,#2454,.T.);
#6690=EDGE_CURVE('',#5175,#5176,#218,.T.);
#6691=EDGE_CURVE('',#5177,#5175,#2455,.T.);
#6692=EDGE_CURVE('',#5178,#5177,#3048,.T.);
#6693=EDGE_CURVE('',#5176,#5178,#2456,.T.);
#6694=EDGE_CURVE('',#5179,#5180,#219,.T.);
#6695=EDGE_CURVE('',#5181,#5179,#2457,.T.);
#6696=EDGE_CURVE('',#5182,#5181,#3049,.T.);
#6697=EDGE_CURVE('',#5180,#5182,#2458,.T.);
#6698=EDGE_CURVE('',#5183,#5184,#3050,.T.);
#6699=EDGE_CURVE('',#5183,#5185,#2459,.T.);
#6700=EDGE_CURVE('',#5186,#5185,#220,.T.);
#6701=EDGE_CURVE('',#5184,#5186,#2460,.T.);
#6702=EDGE_CURVE('',#5187,#5188,#3051,.T.);
#6703=EDGE_CURVE('',#5187,#5189,#2461,.T.);
#6704=EDGE_CURVE('',#5190,#5189,#221,.T.);
#6705=EDGE_CURVE('',#5188,#5190,#2462,.T.);
#6706=EDGE_CURVE('',#5191,#5192,#3052,.T.);
#6707=EDGE_CURVE('',#5191,#5193,#2463,.T.);
#6708=EDGE_CURVE('',#5194,#5193,#222,.T.);
#6709=EDGE_CURVE('',#5192,#5194,#2464,.T.);
#6710=EDGE_CURVE('',#5195,#5196,#3053,.T.);
#6711=EDGE_CURVE('',#5195,#5197,#2465,.T.);
#6712=EDGE_CURVE('',#5198,#5197,#223,.T.);
#6713=EDGE_CURVE('',#5196,#5198,#2466,.T.);
#6714=EDGE_CURVE('',#5199,#5200,#3054,.T.);
#6715=EDGE_CURVE('',#5199,#5201,#2467,.T.);
#6716=EDGE_CURVE('',#5202,#5201,#224,.T.);
#6717=EDGE_CURVE('',#5200,#5202,#2468,.T.);
#6718=EDGE_CURVE('',#5203,#5204,#3055,.T.);
#6719=EDGE_CURVE('',#5203,#5205,#2469,.T.);
#6720=EDGE_CURVE('',#5206,#5205,#225,.T.);
#6721=EDGE_CURVE('',#5204,#5206,#2470,.T.);
#6722=EDGE_CURVE('',#5207,#5208,#3056,.T.);
#6723=EDGE_CURVE('',#5207,#5209,#2471,.T.);
#6724=EDGE_CURVE('',#5210,#5209,#226,.T.);
#6725=EDGE_CURVE('',#5208,#5210,#2472,.T.);
#6726=EDGE_CURVE('',#5211,#5212,#3057,.T.);
#6727=EDGE_CURVE('',#5211,#5213,#2473,.T.);
#6728=EDGE_CURVE('',#5214,#5213,#227,.T.);
#6729=EDGE_CURVE('',#5212,#5214,#2474,.T.);
#6730=EDGE_CURVE('',#5215,#5216,#3058,.T.);
#6731=EDGE_CURVE('',#5215,#5217,#2475,.T.);
#6732=EDGE_CURVE('',#5218,#5217,#228,.T.);
#6733=EDGE_CURVE('',#5216,#5218,#2476,.T.);
#6734=EDGE_CURVE('',#5219,#5220,#3059,.T.);
#6735=EDGE_CURVE('',#5219,#5221,#2477,.T.);
#6736=EDGE_CURVE('',#5222,#5221,#229,.T.);
#6737=EDGE_CURVE('',#5220,#5222,#2478,.T.);
#6738=EDGE_CURVE('',#5223,#5224,#3060,.T.);
#6739=EDGE_CURVE('',#5223,#5225,#2479,.T.);
#6740=EDGE_CURVE('',#5226,#5225,#230,.T.);
#6741=EDGE_CURVE('',#5224,#5226,#2480,.T.);
#6742=EDGE_CURVE('',#5227,#5228,#3061,.T.);
#6743=EDGE_CURVE('',#5227,#5229,#2481,.T.);
#6744=EDGE_CURVE('',#5230,#5229,#231,.T.);
#6745=EDGE_CURVE('',#5228,#5230,#2482,.T.);
#6746=EDGE_CURVE('',#5231,#5232,#3062,.T.);
#6747=EDGE_CURVE('',#5231,#5233,#2483,.T.);
#6748=EDGE_CURVE('',#5234,#5233,#232,.T.);
#6749=EDGE_CURVE('',#5232,#5234,#2484,.T.);
#6750=EDGE_CURVE('',#5235,#5236,#3063,.T.);
#6751=EDGE_CURVE('',#5235,#5237,#2485,.T.);
#6752=EDGE_CURVE('',#5238,#5237,#233,.T.);
#6753=EDGE_CURVE('',#5236,#5238,#2486,.T.);
#6754=EDGE_CURVE('',#5239,#5240,#3064,.T.);
#6755=EDGE_CURVE('',#5239,#5241,#2487,.T.);
#6756=EDGE_CURVE('',#5242,#5241,#234,.T.);
#6757=EDGE_CURVE('',#5240,#5242,#2488,.T.);
#6758=EDGE_CURVE('',#5243,#5244,#3065,.T.);
#6759=EDGE_CURVE('',#5243,#5245,#2489,.T.);
#6760=EDGE_CURVE('',#5246,#5245,#235,.T.);
#6761=EDGE_CURVE('',#5244,#5246,#2490,.T.);
#6762=EDGE_CURVE('',#5247,#5248,#3066,.T.);
#6763=EDGE_CURVE('',#5247,#5249,#2491,.T.);
#6764=EDGE_CURVE('',#5250,#5249,#236,.T.);
#6765=EDGE_CURVE('',#5248,#5250,#2492,.T.);
#6766=EDGE_CURVE('',#5251,#5252,#3067,.T.);
#6767=EDGE_CURVE('',#5251,#5253,#2493,.T.);
#6768=EDGE_CURVE('',#5254,#5253,#237,.T.);
#6769=EDGE_CURVE('',#5252,#5254,#2494,.T.);
#6770=EDGE_CURVE('',#5112,#5183,#3068,.T.);
#6771=EDGE_CURVE('',#5185,#5114,#3069,.T.);
#6772=EDGE_CURVE('',#5116,#5187,#3070,.T.);
#6773=EDGE_CURVE('',#5189,#5118,#3071,.T.);
#6774=EDGE_CURVE('',#5120,#5191,#3072,.T.);
#6775=EDGE_CURVE('',#5193,#5122,#3073,.T.);
#6776=EDGE_CURVE('',#5124,#5195,#3074,.T.);
#6777=EDGE_CURVE('',#5197,#5126,#3075,.T.);
#6778=EDGE_CURVE('',#5128,#5199,#3076,.T.);
#6779=EDGE_CURVE('',#5201,#5130,#3077,.T.);
#6780=EDGE_CURVE('',#5132,#5203,#3078,.T.);
#6781=EDGE_CURVE('',#5205,#5134,#3079,.T.);
#6782=EDGE_CURVE('',#5136,#5207,#3080,.T.);
#6783=EDGE_CURVE('',#5209,#5138,#3081,.T.);
#6784=EDGE_CURVE('',#5140,#5211,#3082,.T.);
#6785=EDGE_CURVE('',#5213,#5142,#3083,.T.);
#6786=EDGE_CURVE('',#5144,#5215,#3084,.T.);
#6787=EDGE_CURVE('',#5217,#5146,#3085,.T.);
#6788=EDGE_CURVE('',#5148,#5219,#3086,.T.);
#6789=EDGE_CURVE('',#5221,#5150,#3087,.T.);
#6790=EDGE_CURVE('',#5152,#5223,#3088,.T.);
#6791=EDGE_CURVE('',#5225,#5154,#3089,.T.);
#6792=EDGE_CURVE('',#5156,#5227,#3090,.T.);
#6793=EDGE_CURVE('',#5229,#5158,#3091,.T.);
#6794=EDGE_CURVE('',#5160,#5231,#3092,.T.);
#6795=EDGE_CURVE('',#5233,#5162,#3093,.T.);
#6796=EDGE_CURVE('',#5164,#5235,#3094,.T.);
#6797=EDGE_CURVE('',#5237,#5166,#3095,.T.);
#6798=EDGE_CURVE('',#5168,#5239,#3096,.T.);
#6799=EDGE_CURVE('',#5241,#5170,#3097,.T.);
#6800=EDGE_CURVE('',#5172,#5243,#3098,.T.);
#6801=EDGE_CURVE('',#5245,#5174,#3099,.T.);
#6802=EDGE_CURVE('',#5176,#5247,#3100,.T.);
#6803=EDGE_CURVE('',#5249,#5178,#3101,.T.);
#6804=EDGE_CURVE('',#5180,#5251,#3102,.T.);
#6805=EDGE_CURVE('',#5253,#5182,#3103,.T.);
#6806=EDGE_CURVE('',#5071,#4930,#3104,.T.);
#6807=EDGE_CURVE('',#5070,#4927,#3105,.T.);
#6808=EDGE_CURVE('',#5063,#4922,#3106,.T.);
#6809=EDGE_CURVE('',#5062,#4919,#3107,.T.);
#6810=EDGE_CURVE('',#5055,#4918,#3108,.T.);
#6811=EDGE_CURVE('',#5054,#4915,#3109,.T.);
#6812=EDGE_CURVE('',#5047,#4914,#3110,.T.);
#6813=EDGE_CURVE('',#5046,#4911,#3111,.T.);
#6814=EDGE_CURVE('',#5039,#4910,#3112,.T.);
#6815=EDGE_CURVE('',#5038,#4907,#3113,.T.);
#6816=EDGE_CURVE('',#5031,#4906,#3114,.T.);
#6817=EDGE_CURVE('',#5030,#4903,#3115,.T.);
#6818=EDGE_CURVE('',#5023,#4902,#3116,.T.);
#6819=EDGE_CURVE('',#5022,#4899,#3117,.T.);
#6820=EDGE_CURVE('',#5015,#4898,#3118,.T.);
#6821=EDGE_CURVE('',#5014,#4895,#3119,.T.);
#6822=EDGE_CURVE('',#5007,#4894,#3120,.T.);
#6823=EDGE_CURVE('',#5006,#4891,#3121,.T.);
#6824=EDGE_CURVE('',#4999,#4890,#3122,.T.);
#6825=EDGE_CURVE('',#4998,#4887,#3123,.T.);
#6826=EDGE_CURVE('',#4991,#4886,#3124,.T.);
#6827=EDGE_CURVE('',#4990,#4883,#3125,.T.);
#6828=EDGE_CURVE('',#4983,#4882,#3126,.T.);
#6829=EDGE_CURVE('',#4982,#4879,#3127,.T.);
#6830=EDGE_CURVE('',#4975,#4878,#3128,.T.);
#6831=EDGE_CURVE('',#4974,#4875,#3129,.T.);
#6832=EDGE_CURVE('',#4967,#4874,#3130,.T.);
#6833=EDGE_CURVE('',#4966,#4871,#3131,.T.);
#6834=EDGE_CURVE('',#4959,#4870,#3132,.T.);
#6835=EDGE_CURVE('',#4958,#4867,#3133,.T.);
#6836=EDGE_CURVE('',#4951,#4866,#3134,.T.);
#6837=EDGE_CURVE('',#4950,#4863,#3135,.T.);
#6838=EDGE_CURVE('',#4943,#4862,#3136,.T.);
#6839=EDGE_CURVE('',#4942,#4859,#3137,.T.);
#6840=EDGE_CURVE('',#4935,#4926,#3138,.T.);
#6841=EDGE_CURVE('',#4934,#4923,#3139,.T.);
#6842=EDGE_CURVE('',#5074,#4929,#3140,.T.);
#6843=EDGE_CURVE('',#5109,#5179,#2495,.T.);
#6844=EDGE_CURVE('',#5252,#4858,#2496,.T.);
#6845=EDGE_CURVE('',#5254,#4856,#2497,.T.);
#6846=EDGE_CURVE('',#5110,#5181,#2498,.T.);
#6847=EDGE_CURVE('',#5066,#4921,#3141,.T.);
#6848=EDGE_CURVE('',#5107,#5175,#2499,.T.);
#6849=EDGE_CURVE('',#5248,#4790,#2500,.T.);
#6850=EDGE_CURVE('',#5250,#4788,#2501,.T.);
#6851=EDGE_CURVE('',#5108,#5177,#2502,.T.);
#6852=EDGE_CURVE('',#5058,#4917,#3142,.T.);
#6853=EDGE_CURVE('',#5105,#5171,#2503,.T.);
#6854=EDGE_CURVE('',#5244,#4794,#2504,.T.);
#6855=EDGE_CURVE('',#5246,#4792,#2505,.T.);
#6856=EDGE_CURVE('',#5106,#5173,#2506,.T.);
#6857=EDGE_CURVE('',#5050,#4913,#3143,.T.);
#6858=EDGE_CURVE('',#5103,#5167,#2507,.T.);
#6859=EDGE_CURVE('',#5240,#4798,#2508,.T.);
#6860=EDGE_CURVE('',#5242,#4796,#2509,.T.);
#6861=EDGE_CURVE('',#5104,#5169,#2510,.T.);
#6862=EDGE_CURVE('',#5042,#4909,#3144,.T.);
#6863=EDGE_CURVE('',#5101,#5163,#2511,.T.);
#6864=EDGE_CURVE('',#5236,#4802,#2512,.T.);
#6865=EDGE_CURVE('',#5238,#4800,#2513,.T.);
#6866=EDGE_CURVE('',#5102,#5165,#2514,.T.);
#6867=EDGE_CURVE('',#5034,#4905,#3145,.T.);
#6868=EDGE_CURVE('',#5099,#5159,#2515,.T.);
#6869=EDGE_CURVE('',#5232,#4806,#2516,.T.);
#6870=EDGE_CURVE('',#5234,#4804,#2517,.T.);
#6871=EDGE_CURVE('',#5100,#5161,#2518,.T.);
#6872=EDGE_CURVE('',#5026,#4901,#3146,.T.);
#6873=EDGE_CURVE('',#5097,#5155,#2519,.T.);
#6874=EDGE_CURVE('',#5228,#4810,#2520,.T.);
#6875=EDGE_CURVE('',#5230,#4808,#2521,.T.);
#6876=EDGE_CURVE('',#5098,#5157,#2522,.T.);
#6877=EDGE_CURVE('',#5018,#4897,#3147,.T.);
#6878=EDGE_CURVE('',#5095,#5151,#2523,.T.);
#6879=EDGE_CURVE('',#5224,#4814,#2524,.T.);
#6880=EDGE_CURVE('',#5226,#4812,#2525,.T.);
#6881=EDGE_CURVE('',#5096,#5153,#2526,.T.);
#6882=EDGE_CURVE('',#5010,#4893,#3148,.T.);
#6883=EDGE_CURVE('',#5093,#5147,#2527,.T.);
#6884=EDGE_CURVE('',#5220,#4818,#2528,.T.);
#6885=EDGE_CURVE('',#5222,#4816,#2529,.T.);
#6886=EDGE_CURVE('',#5094,#5149,#2530,.T.);
#6887=EDGE_CURVE('',#5002,#4889,#3149,.T.);
#6888=EDGE_CURVE('',#5091,#5143,#2531,.T.);
#6889=EDGE_CURVE('',#5216,#4822,#2532,.T.);
#6890=EDGE_CURVE('',#5218,#4820,#2533,.T.);
#6891=EDGE_CURVE('',#5092,#5145,#2534,.T.);
#6892=EDGE_CURVE('',#4994,#4885,#3150,.T.);
#6893=EDGE_CURVE('',#5089,#5139,#2535,.T.);
#6894=EDGE_CURVE('',#5212,#4826,#2536,.T.);
#6895=EDGE_CURVE('',#5214,#4824,#2537,.T.);
#6896=EDGE_CURVE('',#5090,#5141,#2538,.T.);
#6897=EDGE_CURVE('',#4986,#4881,#3151,.T.);
#6898=EDGE_CURVE('',#5087,#5135,#2539,.T.);
#6899=EDGE_CURVE('',#5208,#4830,#2540,.T.);
#6900=EDGE_CURVE('',#5210,#4828,#2541,.T.);
#6901=EDGE_CURVE('',#5088,#5137,#2542,.T.);
#6902=EDGE_CURVE('',#4978,#4877,#3152,.T.);
#6903=EDGE_CURVE('',#5085,#5131,#2543,.T.);
#6904=EDGE_CURVE('',#5204,#4834,#2544,.T.);
#6905=EDGE_CURVE('',#5206,#4832,#2545,.T.);
#6906=EDGE_CURVE('',#5086,#5133,#2546,.T.);
#6907=EDGE_CURVE('',#4970,#4873,#3153,.T.);
#6908=EDGE_CURVE('',#5083,#5127,#2547,.T.);
#6909=EDGE_CURVE('',#5200,#4838,#2548,.T.);
#6910=EDGE_CURVE('',#5202,#4836,#2549,.T.);
#6911=EDGE_CURVE('',#5084,#5129,#2550,.T.);
#6912=EDGE_CURVE('',#4962,#4869,#3154,.T.);
#6913=EDGE_CURVE('',#5081,#5123,#2551,.T.);
#6914=EDGE_CURVE('',#5196,#4842,#2552,.T.);
#6915=EDGE_CURVE('',#5198,#4840,#2553,.T.);
#6916=EDGE_CURVE('',#5082,#5125,#2554,.T.);
#6917=EDGE_CURVE('',#4954,#4865,#3155,.T.);
#6918=EDGE_CURVE('',#5079,#5119,#2555,.T.);
#6919=EDGE_CURVE('',#5192,#4846,#2556,.T.);
#6920=EDGE_CURVE('',#5194,#4844,#2557,.T.);
#6921=EDGE_CURVE('',#5080,#5121,#2558,.T.);
#6922=EDGE_CURVE('',#4946,#4861,#3156,.T.);
#6923=EDGE_CURVE('',#5077,#5115,#2559,.T.);
#6924=EDGE_CURVE('',#5188,#4850,#2560,.T.);
#6925=EDGE_CURVE('',#5190,#4848,#2561,.T.);
#6926=EDGE_CURVE('',#5078,#5117,#2562,.T.);
#6927=EDGE_CURVE('',#4938,#4925,#3157,.T.);
#6928=EDGE_CURVE('',#5075,#5111,#2563,.T.);
#6929=EDGE_CURVE('',#5184,#4854,#2564,.T.);
#6930=EDGE_CURVE('',#5186,#4852,#2565,.T.);
#6931=EDGE_CURVE('',#5076,#5113,#2566,.T.);
#6932=EDGE_CURVE('',#5255,#5069,#3879,.F.);
#6933=EDGE_CURVE('',#4717,#5255,#3158,.T.);
#6934=EDGE_CURVE('',#5068,#4928,#3159,.T.);
#6935=EDGE_CURVE('',#5256,#4786,#3160,.T.);
#6936=EDGE_CURVE('',#5256,#5067,#3880,.T.);
#6937=EDGE_CURVE('',#5255,#5257,#2567,.T.);
#6938=EDGE_CURVE('',#5257,#4718,#3161,.T.);
#6939=EDGE_CURVE('',#4785,#5258,#3162,.T.);
#6940=EDGE_CURVE('',#5258,#5256,#2568,.T.);
#6941=EDGE_CURVE('',#5259,#4782,#3163,.T.);
#6942=EDGE_CURVE('',#5259,#5059,#3881,.T.);
#6943=EDGE_CURVE('',#5060,#4920,#3164,.T.);
#6944=EDGE_CURVE('',#5258,#5061,#3882,.F.);
#6945=EDGE_CURVE('',#5260,#5053,#3883,.F.);
#6946=EDGE_CURVE('',#4781,#5260,#3165,.T.);
#6947=EDGE_CURVE('',#5261,#4778,#3166,.T.);
#6948=EDGE_CURVE('',#5261,#5051,#3884,.T.);
#6949=EDGE_CURVE('',#5052,#4916,#3167,.T.);
#6950=EDGE_CURVE('',#5260,#5259,#2569,.T.);
#6951=EDGE_CURVE('',#5262,#5261,#2570,.T.);
#6952=EDGE_CURVE('',#5262,#5045,#3885,.F.);
#6953=EDGE_CURVE('',#5263,#5043,#3886,.T.);
#6954=EDGE_CURVE('',#5264,#5263,#2571,.T.);
#6955=EDGE_CURVE('',#5264,#5037,#3887,.F.);
#6956=EDGE_CURVE('',#5265,#5035,#3888,.T.);
#6957=EDGE_CURVE('',#5266,#5265,#2572,.T.);
#6958=EDGE_CURVE('',#5266,#5029,#3889,.F.);
#6959=EDGE_CURVE('',#5267,#5027,#3890,.T.);
#6960=EDGE_CURVE('',#5268,#5267,#2573,.T.);
#6961=EDGE_CURVE('',#5268,#5021,#3891,.F.);
#6962=EDGE_CURVE('',#5269,#5019,#3892,.T.);
#6963=EDGE_CURVE('',#5270,#5269,#2574,.T.);
#6964=EDGE_CURVE('',#5270,#5013,#3893,.F.);
#6965=EDGE_CURVE('',#5271,#5011,#3894,.T.);
#6966=EDGE_CURVE('',#5272,#5271,#2575,.T.);
#6967=EDGE_CURVE('',#5272,#5005,#3895,.F.);
#6968=EDGE_CURVE('',#5273,#5003,#3896,.T.);
#6969=EDGE_CURVE('',#5274,#5273,#2576,.T.);
#6970=EDGE_CURVE('',#5274,#4997,#3897,.F.);
#6971=EDGE_CURVE('',#5275,#4995,#3898,.T.);
#6972=EDGE_CURVE('',#5276,#5275,#2577,.T.);
#6973=EDGE_CURVE('',#5276,#4989,#3899,.F.);
#6974=EDGE_CURVE('',#5277,#4987,#3900,.T.);
#6975=EDGE_CURVE('',#5278,#5277,#2578,.T.);
#6976=EDGE_CURVE('',#5278,#4981,#3901,.F.);
#6977=EDGE_CURVE('',#5279,#4979,#3902,.T.);
#6978=EDGE_CURVE('',#5280,#5279,#2579,.T.);
#6979=EDGE_CURVE('',#5280,#4973,#3903,.F.);
#6980=EDGE_CURVE('',#5281,#4971,#3904,.T.);
#6981=EDGE_CURVE('',#5282,#5281,#2580,.T.);
#6982=EDGE_CURVE('',#5282,#4965,#3905,.F.);
#6983=EDGE_CURVE('',#5283,#4963,#3906,.T.);
#6984=EDGE_CURVE('',#5284,#5283,#2581,.T.);
#6985=EDGE_CURVE('',#5284,#4957,#3907,.F.);
#6986=EDGE_CURVE('',#5285,#4955,#3908,.T.);
#6987=EDGE_CURVE('',#5286,#5285,#2582,.T.);
#6988=EDGE_CURVE('',#5286,#4949,#3909,.F.);
#6989=EDGE_CURVE('',#5287,#4947,#3910,.T.);
#6990=EDGE_CURVE('',#5288,#5287,#2583,.T.);
#6991=EDGE_CURVE('',#5288,#4941,#3911,.F.);
#6992=EDGE_CURVE('',#5289,#4939,#3912,.T.);
#6993=EDGE_CURVE('',#5290,#5289,#2584,.T.);
#6994=EDGE_CURVE('',#5290,#4933,#3913,.F.);
#6995=EDGE_CURVE('',#5257,#4931,#3914,.T.);
#6996=EDGE_CURVE('',#4777,#5262,#3168,.T.);
#6997=EDGE_CURVE('',#5044,#4912,#3169,.T.);
#6998=EDGE_CURVE('',#5263,#4774,#3170,.T.);
#6999=EDGE_CURVE('',#4773,#5264,#3171,.T.);
#7000=EDGE_CURVE('',#5265,#4770,#3172,.T.);
#7001=EDGE_CURVE('',#5036,#4908,#3173,.T.);
#7002=EDGE_CURVE('',#4769,#5266,#3174,.T.);
#7003=EDGE_CURVE('',#5267,#4766,#3175,.T.);
#7004=EDGE_CURVE('',#5028,#4904,#3176,.T.);
#7005=EDGE_CURVE('',#4765,#5268,#3177,.T.);
#7006=EDGE_CURVE('',#5020,#4900,#3178,.T.);
#7007=EDGE_CURVE('',#5269,#4762,#3179,.T.);
#7008=EDGE_CURVE('',#4761,#5270,#3180,.T.);
#7009=EDGE_CURVE('',#5271,#4758,#3181,.T.);
#7010=EDGE_CURVE('',#5012,#4896,#3182,.T.);
#7011=EDGE_CURVE('',#4757,#5272,#3183,.T.);
#7012=EDGE_CURVE('',#5273,#4754,#3184,.T.);
#7013=EDGE_CURVE('',#5004,#4892,#3185,.T.);
#7014=EDGE_CURVE('',#4753,#5274,#3186,.T.);
#7015=EDGE_CURVE('',#4996,#4888,#3187,.T.);
#7016=EDGE_CURVE('',#5275,#4750,#3188,.T.);
#7017=EDGE_CURVE('',#4749,#5276,#3189,.T.);
#7018=EDGE_CURVE('',#5277,#4746,#3190,.T.);
#7019=EDGE_CURVE('',#4988,#4884,#3191,.T.);
#7020=EDGE_CURVE('',#4745,#5278,#3192,.T.);
#7021=EDGE_CURVE('',#5279,#4742,#3193,.T.);
#7022=EDGE_CURVE('',#4980,#4880,#3194,.T.);
#7023=EDGE_CURVE('',#4741,#5280,#3195,.T.);
#7024=EDGE_CURVE('',#4972,#4876,#3196,.T.);
#7025=EDGE_CURVE('',#5281,#4738,#3197,.T.);
#7026=EDGE_CURVE('',#4737,#5282,#3198,.T.);
#7027=EDGE_CURVE('',#5283,#4734,#3199,.T.);
#7028=EDGE_CURVE('',#4964,#4872,#3200,.T.);
#7029=EDGE_CURVE('',#4733,#5284,#3201,.T.);
#7030=EDGE_CURVE('',#5285,#4730,#3202,.T.);
#7031=EDGE_CURVE('',#4956,#4868,#3203,.T.);
#7032=EDGE_CURVE('',#4729,#5286,#3204,.T.);
#7033=EDGE_CURVE('',#4948,#4864,#3205,.T.);
#7034=EDGE_CURVE('',#5287,#4726,#3206,.T.);
#7035=EDGE_CURVE('',#4725,#5288,#3207,.T.);
#7036=EDGE_CURVE('',#5289,#4722,#3208,.T.);
#7037=EDGE_CURVE('',#4940,#4860,#3209,.T.);
#7038=EDGE_CURVE('',#4721,#5290,#3210,.T.);
#7039=EDGE_CURVE('',#4932,#4924,#3211,.T.);
#8072=ORIENTED_EDGE('',*,*,#6048,.T.);
#8073=ORIENTED_EDGE('',*,*,#6049,.T.);
#8074=ORIENTED_EDGE('',*,*,#6050,.F.);
#8075=ORIENTED_EDGE('',*,*,#6051,.F.);
#8076=ORIENTED_EDGE('',*,*,#6052,.T.);
#8077=ORIENTED_EDGE('',*,*,#6053,.T.);
#8078=ORIENTED_EDGE('',*,*,#6054,.T.);
#8079=ORIENTED_EDGE('',*,*,#6048,.F.);
#8080=ORIENTED_EDGE('',*,*,#6055,.F.);
#8081=ORIENTED_EDGE('',*,*,#6056,.F.);
#8082=ORIENTED_EDGE('',*,*,#6057,.T.);
#8083=ORIENTED_EDGE('',*,*,#6058,.T.);
#8084=ORIENTED_EDGE('',*,*,#6059,.T.);
#8085=ORIENTED_EDGE('',*,*,#6052,.F.);
#8086=ORIENTED_EDGE('',*,*,#6060,.F.);
#8087=ORIENTED_EDGE('',*,*,#6061,.F.);
#8088=ORIENTED_EDGE('',*,*,#6062,.T.);
#8089=ORIENTED_EDGE('',*,*,#6063,.T.);
#8090=ORIENTED_EDGE('',*,*,#6064,.T.);
#8091=ORIENTED_EDGE('',*,*,#6057,.F.);
#8092=ORIENTED_EDGE('',*,*,#6065,.F.);
#8093=ORIENTED_EDGE('',*,*,#6066,.F.);
#8094=ORIENTED_EDGE('',*,*,#6067,.T.);
#8095=ORIENTED_EDGE('',*,*,#6068,.T.);
#8096=ORIENTED_EDGE('',*,*,#6069,.T.);
#8097=ORIENTED_EDGE('',*,*,#6062,.F.);
#8098=ORIENTED_EDGE('',*,*,#6070,.F.);
#8099=ORIENTED_EDGE('',*,*,#6071,.F.);
#8100=ORIENTED_EDGE('',*,*,#6072,.T.);
#8101=ORIENTED_EDGE('',*,*,#6073,.T.);
#8102=ORIENTED_EDGE('',*,*,#6074,.T.);
#8103=ORIENTED_EDGE('',*,*,#6067,.F.);
#8104=ORIENTED_EDGE('',*,*,#6075,.F.);
#8105=ORIENTED_EDGE('',*,*,#6076,.F.);
#8106=ORIENTED_EDGE('',*,*,#6077,.T.);
#8107=ORIENTED_EDGE('',*,*,#6078,.T.);
#8108=ORIENTED_EDGE('',*,*,#6079,.T.);
#8109=ORIENTED_EDGE('',*,*,#6072,.F.);
#8110=ORIENTED_EDGE('',*,*,#6080,.F.);
#8111=ORIENTED_EDGE('',*,*,#6081,.F.);
#8112=ORIENTED_EDGE('',*,*,#6082,.T.);
#8113=ORIENTED_EDGE('',*,*,#6083,.T.);
#8114=ORIENTED_EDGE('',*,*,#6084,.T.);
#8115=ORIENTED_EDGE('',*,*,#6077,.F.);
#8116=ORIENTED_EDGE('',*,*,#6085,.F.);
#8117=ORIENTED_EDGE('',*,*,#6086,.F.);
#8118=ORIENTED_EDGE('',*,*,#6087,.T.);
#8119=ORIENTED_EDGE('',*,*,#6088,.T.);
#8120=ORIENTED_EDGE('',*,*,#6089,.T.);
#8121=ORIENTED_EDGE('',*,*,#6082,.F.);
#8122=ORIENTED_EDGE('',*,*,#6090,.F.);
#8123=ORIENTED_EDGE('',*,*,#6091,.F.);
#8124=ORIENTED_EDGE('',*,*,#6092,.T.);
#8125=ORIENTED_EDGE('',*,*,#6093,.T.);
#8126=ORIENTED_EDGE('',*,*,#6094,.T.);
#8127=ORIENTED_EDGE('',*,*,#6087,.F.);
#8128=ORIENTED_EDGE('',*,*,#6095,.F.);
#8129=ORIENTED_EDGE('',*,*,#6096,.F.);
#8130=ORIENTED_EDGE('',*,*,#6097,.T.);
#8131=ORIENTED_EDGE('',*,*,#6098,.T.);
#8132=ORIENTED_EDGE('',*,*,#6099,.T.);
#8133=ORIENTED_EDGE('',*,*,#6092,.F.);
#8134=ORIENTED_EDGE('',*,*,#6100,.F.);
#8135=ORIENTED_EDGE('',*,*,#6101,.F.);
#8136=ORIENTED_EDGE('',*,*,#6102,.F.);
#8137=ORIENTED_EDGE('',*,*,#6103,.F.);
#8138=ORIENTED_EDGE('',*,*,#6104,.F.);
#8139=ORIENTED_EDGE('',*,*,#6105,.F.);
#8140=ORIENTED_EDGE('',*,*,#6106,.T.);
#8141=ORIENTED_EDGE('',*,*,#6107,.T.);
#8142=ORIENTED_EDGE('',*,*,#6108,.T.);
#8143=ORIENTED_EDGE('',*,*,#6109,.T.);
#8144=ORIENTED_EDGE('',*,*,#6110,.F.);
#8145=ORIENTED_EDGE('',*,*,#6111,.T.);
#8146=ORIENTED_EDGE('',*,*,#6112,.T.);
#8147=ORIENTED_EDGE('',*,*,#6113,.T.);
#8148=ORIENTED_EDGE('',*,*,#6108,.F.);
#8149=ORIENTED_EDGE('',*,*,#6114,.T.);
#8150=ORIENTED_EDGE('',*,*,#6115,.T.);
#8151=ORIENTED_EDGE('',*,*,#6116,.T.);
#8152=ORIENTED_EDGE('',*,*,#6117,.T.);
#8153=ORIENTED_EDGE('',*,*,#6118,.T.);
#8154=ORIENTED_EDGE('',*,*,#6112,.F.);
#8155=ORIENTED_EDGE('',*,*,#6119,.T.);
#8156=ORIENTED_EDGE('',*,*,#6120,.T.);
#8157=ORIENTED_EDGE('',*,*,#6121,.T.);
#8158=ORIENTED_EDGE('',*,*,#6122,.T.);
#8159=ORIENTED_EDGE('',*,*,#6123,.T.);
#8160=ORIENTED_EDGE('',*,*,#6116,.F.);
#8161=ORIENTED_EDGE('',*,*,#6124,.T.);
#8162=ORIENTED_EDGE('',*,*,#6125,.T.);
#8163=ORIENTED_EDGE('',*,*,#6126,.T.);
#8164=ORIENTED_EDGE('',*,*,#6127,.T.);
#8165=ORIENTED_EDGE('',*,*,#6128,.T.);
#8166=ORIENTED_EDGE('',*,*,#6121,.F.);
#8167=ORIENTED_EDGE('',*,*,#6129,.T.);
#8168=ORIENTED_EDGE('',*,*,#6130,.T.);
#8169=ORIENTED_EDGE('',*,*,#6131,.T.);
#8170=ORIENTED_EDGE('',*,*,#6132,.T.);
#8171=ORIENTED_EDGE('',*,*,#6133,.T.);
#8172=ORIENTED_EDGE('',*,*,#6126,.F.);
#8173=ORIENTED_EDGE('',*,*,#6134,.T.);
#8174=ORIENTED_EDGE('',*,*,#6135,.T.);
#8175=ORIENTED_EDGE('',*,*,#6136,.T.);
#8176=ORIENTED_EDGE('',*,*,#6137,.T.);
#8177=ORIENTED_EDGE('',*,*,#6138,.T.);
#8178=ORIENTED_EDGE('',*,*,#6131,.F.);
#8179=ORIENTED_EDGE('',*,*,#6139,.T.);
#8180=ORIENTED_EDGE('',*,*,#6140,.T.);
#8181=ORIENTED_EDGE('',*,*,#6141,.T.);
#8182=ORIENTED_EDGE('',*,*,#6142,.T.);
#8183=ORIENTED_EDGE('',*,*,#6136,.F.);
#8184=ORIENTED_EDGE('',*,*,#6143,.T.);
#8185=ORIENTED_EDGE('',*,*,#6144,.T.);
#8186=ORIENTED_EDGE('',*,*,#6145,.T.);
#8187=ORIENTED_EDGE('',*,*,#6146,.T.);
#8188=ORIENTED_EDGE('',*,*,#6147,.T.);
#8189=ORIENTED_EDGE('',*,*,#6141,.F.);
#8190=ORIENTED_EDGE('',*,*,#6148,.T.);
#8191=ORIENTED_EDGE('',*,*,#6149,.T.);
#8192=ORIENTED_EDGE('',*,*,#6150,.T.);
#8193=ORIENTED_EDGE('',*,*,#6151,.T.);
#8194=ORIENTED_EDGE('',*,*,#6152,.T.);
#8195=ORIENTED_EDGE('',*,*,#6145,.F.);
#8196=ORIENTED_EDGE('',*,*,#6153,.T.);
#8197=ORIENTED_EDGE('',*,*,#6154,.T.);
#8198=ORIENTED_EDGE('',*,*,#6155,.T.);
#8199=ORIENTED_EDGE('',*,*,#6150,.F.);
#8200=ORIENTED_EDGE('',*,*,#6156,.T.);
#8201=ORIENTED_EDGE('',*,*,#6157,.T.);
#8202=ORIENTED_EDGE('',*,*,#6158,.F.);
#8203=ORIENTED_EDGE('',*,*,#6159,.T.);
#8204=ORIENTED_EDGE('',*,*,#6160,.T.);
#8205=ORIENTED_EDGE('',*,*,#6161,.F.);
#8206=ORIENTED_EDGE('',*,*,#6162,.T.);
#8207=ORIENTED_EDGE('',*,*,#6158,.T.);
#8208=ORIENTED_EDGE('',*,*,#6163,.T.);
#8209=ORIENTED_EDGE('',*,*,#6164,.T.);
#8210=ORIENTED_EDGE('',*,*,#6154,.F.);
#8211=ORIENTED_EDGE('',*,*,#6165,.T.);
#8212=ORIENTED_EDGE('',*,*,#6166,.T.);
#8213=ORIENTED_EDGE('',*,*,#6102,.T.);
#8214=ORIENTED_EDGE('',*,*,#6167,.T.);
#8215=ORIENTED_EDGE('',*,*,#6168,.T.);
#8216=ORIENTED_EDGE('',*,*,#6097,.F.);
#8217=ORIENTED_EDGE('',*,*,#6169,.F.);
#8218=ORIENTED_EDGE('',*,*,#6170,.F.);
#8219=ORIENTED_EDGE('',*,*,#6171,.F.);
#8220=ORIENTED_EDGE('',*,*,#6049,.F.);
#8221=ORIENTED_EDGE('',*,*,#6054,.F.);
#8222=ORIENTED_EDGE('',*,*,#6053,.F.);
#8223=ORIENTED_EDGE('',*,*,#6059,.F.);
#8224=ORIENTED_EDGE('',*,*,#6058,.F.);
#8225=ORIENTED_EDGE('',*,*,#6064,.F.);
#8226=ORIENTED_EDGE('',*,*,#6063,.F.);
#8227=ORIENTED_EDGE('',*,*,#6069,.F.);
#8228=ORIENTED_EDGE('',*,*,#6068,.F.);
#8229=ORIENTED_EDGE('',*,*,#6074,.F.);
#8230=ORIENTED_EDGE('',*,*,#6073,.F.);
#8231=ORIENTED_EDGE('',*,*,#6079,.F.);
#8232=ORIENTED_EDGE('',*,*,#6078,.F.);
#8233=ORIENTED_EDGE('',*,*,#6084,.F.);
#8234=ORIENTED_EDGE('',*,*,#6083,.F.);
#8235=ORIENTED_EDGE('',*,*,#6089,.F.);
#8236=ORIENTED_EDGE('',*,*,#6088,.F.);
#8237=ORIENTED_EDGE('',*,*,#6094,.F.);
#8238=ORIENTED_EDGE('',*,*,#6093,.F.);
#8239=ORIENTED_EDGE('',*,*,#6099,.F.);
#8240=ORIENTED_EDGE('',*,*,#6098,.F.);
#8241=ORIENTED_EDGE('',*,*,#6168,.F.);
#8242=ORIENTED_EDGE('',*,*,#6167,.F.);
#8243=ORIENTED_EDGE('',*,*,#6107,.F.);
#8244=ORIENTED_EDGE('',*,*,#6106,.F.);
#8245=ORIENTED_EDGE('',*,*,#6172,.F.);
#8246=ORIENTED_EDGE('',*,*,#6160,.F.);
#8247=ORIENTED_EDGE('',*,*,#6159,.F.);
#8248=ORIENTED_EDGE('',*,*,#6166,.F.);
#8249=ORIENTED_EDGE('',*,*,#6165,.F.);
#8250=ORIENTED_EDGE('',*,*,#6157,.F.);
#8251=ORIENTED_EDGE('',*,*,#6156,.F.);
#8252=ORIENTED_EDGE('',*,*,#6153,.F.);
#8253=ORIENTED_EDGE('',*,*,#6149,.F.);
#8254=ORIENTED_EDGE('',*,*,#6148,.F.);
#8255=ORIENTED_EDGE('',*,*,#6144,.F.);
#8256=ORIENTED_EDGE('',*,*,#6143,.F.);
#8257=ORIENTED_EDGE('',*,*,#6140,.F.);
#8258=ORIENTED_EDGE('',*,*,#6139,.F.);
#8259=ORIENTED_EDGE('',*,*,#6135,.F.);
#8260=ORIENTED_EDGE('',*,*,#6134,.F.);
#8261=ORIENTED_EDGE('',*,*,#6130,.F.);
#8262=ORIENTED_EDGE('',*,*,#6129,.F.);
#8263=ORIENTED_EDGE('',*,*,#6125,.F.);
#8264=ORIENTED_EDGE('',*,*,#6124,.F.);
#8265=ORIENTED_EDGE('',*,*,#6120,.F.);
#8266=ORIENTED_EDGE('',*,*,#6119,.F.);
#8267=ORIENTED_EDGE('',*,*,#6115,.F.);
#8268=ORIENTED_EDGE('',*,*,#6114,.F.);
#8269=ORIENTED_EDGE('',*,*,#6111,.F.);
#8270=ORIENTED_EDGE('',*,*,#6173,.F.);
#8271=ORIENTED_EDGE('',*,*,#6109,.F.);
#8272=ORIENTED_EDGE('',*,*,#6113,.F.);
#8273=ORIENTED_EDGE('',*,*,#6118,.F.);
#8274=ORIENTED_EDGE('',*,*,#6117,.F.);
#8275=ORIENTED_EDGE('',*,*,#6123,.F.);
#8276=ORIENTED_EDGE('',*,*,#6122,.F.);
#8277=ORIENTED_EDGE('',*,*,#6128,.F.);
#8278=ORIENTED_EDGE('',*,*,#6127,.F.);
#8279=ORIENTED_EDGE('',*,*,#6133,.F.);
#8280=ORIENTED_EDGE('',*,*,#6132,.F.);
#8281=ORIENTED_EDGE('',*,*,#6138,.F.);
#8282=ORIENTED_EDGE('',*,*,#6137,.F.);
#8283=ORIENTED_EDGE('',*,*,#6142,.F.);
#8284=ORIENTED_EDGE('',*,*,#6147,.F.);
#8285=ORIENTED_EDGE('',*,*,#6146,.F.);
#8286=ORIENTED_EDGE('',*,*,#6152,.F.);
#8287=ORIENTED_EDGE('',*,*,#6151,.F.);
#8288=ORIENTED_EDGE('',*,*,#6155,.F.);
#8289=ORIENTED_EDGE('',*,*,#6164,.F.);
#8290=ORIENTED_EDGE('',*,*,#6163,.F.);
#8291=ORIENTED_EDGE('',*,*,#6162,.F.);
#8292=ORIENTED_EDGE('',*,*,#6174,.F.);
#8293=ORIENTED_EDGE('',*,*,#6175,.F.);
#8294=ORIENTED_EDGE('',*,*,#6104,.T.);
#8295=ORIENTED_EDGE('',*,*,#6103,.T.);
#8296=ORIENTED_EDGE('',*,*,#6170,.T.);
#8297=ORIENTED_EDGE('',*,*,#6169,.T.);
#8298=ORIENTED_EDGE('',*,*,#6101,.T.);
#8299=ORIENTED_EDGE('',*,*,#6100,.T.);
#8300=ORIENTED_EDGE('',*,*,#6096,.T.);
#8301=ORIENTED_EDGE('',*,*,#6095,.T.);
#8302=ORIENTED_EDGE('',*,*,#6091,.T.);
#8303=ORIENTED_EDGE('',*,*,#6090,.T.);
#8304=ORIENTED_EDGE('',*,*,#6086,.T.);
#8305=ORIENTED_EDGE('',*,*,#6085,.T.);
#8306=ORIENTED_EDGE('',*,*,#6081,.T.);
#8307=ORIENTED_EDGE('',*,*,#6080,.T.);
#8308=ORIENTED_EDGE('',*,*,#6076,.T.);
#8309=ORIENTED_EDGE('',*,*,#6075,.T.);
#8310=ORIENTED_EDGE('',*,*,#6071,.T.);
#8311=ORIENTED_EDGE('',*,*,#6070,.T.);
#8312=ORIENTED_EDGE('',*,*,#6066,.T.);
#8313=ORIENTED_EDGE('',*,*,#6065,.T.);
#8314=ORIENTED_EDGE('',*,*,#6061,.T.);
#8315=ORIENTED_EDGE('',*,*,#6060,.T.);
#8316=ORIENTED_EDGE('',*,*,#6056,.T.);
#8317=ORIENTED_EDGE('',*,*,#6055,.T.);
#8318=ORIENTED_EDGE('',*,*,#6051,.T.);
#8319=ORIENTED_EDGE('',*,*,#6176,.T.);
#8320=ORIENTED_EDGE('',*,*,#6177,.T.);
#8321=ORIENTED_EDGE('',*,*,#6178,.T.);
#8322=ORIENTED_EDGE('',*,*,#6179,.T.);
#8323=ORIENTED_EDGE('',*,*,#6180,.T.);
#8324=ORIENTED_EDGE('',*,*,#6181,.T.);
#8325=ORIENTED_EDGE('',*,*,#6182,.T.);
#8326=ORIENTED_EDGE('',*,*,#6183,.T.);
#8327=ORIENTED_EDGE('',*,*,#6184,.T.);
#8328=ORIENTED_EDGE('',*,*,#6185,.T.);
#8329=ORIENTED_EDGE('',*,*,#6186,.T.);
#8330=ORIENTED_EDGE('',*,*,#6187,.T.);
#8331=ORIENTED_EDGE('',*,*,#6188,.T.);
#8332=ORIENTED_EDGE('',*,*,#6189,.T.);
#8333=ORIENTED_EDGE('',*,*,#6190,.T.);
#8334=ORIENTED_EDGE('',*,*,#6191,.T.);
#8335=ORIENTED_EDGE('',*,*,#6192,.T.);
#8336=ORIENTED_EDGE('',*,*,#6193,.T.);
#8337=ORIENTED_EDGE('',*,*,#6194,.T.);
#8338=ORIENTED_EDGE('',*,*,#6195,.T.);
#8339=ORIENTED_EDGE('',*,*,#6196,.T.);
#8340=ORIENTED_EDGE('',*,*,#6197,.T.);
#8341=ORIENTED_EDGE('',*,*,#6198,.T.);
#8342=ORIENTED_EDGE('',*,*,#6199,.T.);
#8343=ORIENTED_EDGE('',*,*,#6200,.T.);
#8344=ORIENTED_EDGE('',*,*,#6201,.T.);
#8345=ORIENTED_EDGE('',*,*,#6202,.T.);
#8346=ORIENTED_EDGE('',*,*,#6203,.T.);
#8347=ORIENTED_EDGE('',*,*,#6204,.T.);
#8348=ORIENTED_EDGE('',*,*,#6205,.T.);
#8349=ORIENTED_EDGE('',*,*,#6206,.T.);
#8350=ORIENTED_EDGE('',*,*,#6207,.T.);
#8351=ORIENTED_EDGE('',*,*,#6208,.T.);
#8352=ORIENTED_EDGE('',*,*,#6209,.T.);
#8353=ORIENTED_EDGE('',*,*,#6210,.T.);
#8354=ORIENTED_EDGE('',*,*,#6211,.T.);
#8355=ORIENTED_EDGE('',*,*,#6212,.T.);
#8356=ORIENTED_EDGE('',*,*,#6213,.T.);
#8357=ORIENTED_EDGE('',*,*,#6214,.T.);
#8358=ORIENTED_EDGE('',*,*,#6215,.T.);
#8359=ORIENTED_EDGE('',*,*,#6216,.T.);
#8360=ORIENTED_EDGE('',*,*,#6217,.T.);
#8361=ORIENTED_EDGE('',*,*,#6218,.T.);
#8362=ORIENTED_EDGE('',*,*,#6219,.T.);
#8363=ORIENTED_EDGE('',*,*,#6220,.T.);
#8364=ORIENTED_EDGE('',*,*,#6221,.T.);
#8365=ORIENTED_EDGE('',*,*,#6222,.T.);
#8366=ORIENTED_EDGE('',*,*,#6223,.T.);
#8367=ORIENTED_EDGE('',*,*,#6224,.T.);
#8368=ORIENTED_EDGE('',*,*,#6225,.T.);
#8369=ORIENTED_EDGE('',*,*,#6226,.T.);
#8370=ORIENTED_EDGE('',*,*,#6227,.T.);
#8371=ORIENTED_EDGE('',*,*,#6228,.T.);
#8372=ORIENTED_EDGE('',*,*,#6229,.T.);
#8373=ORIENTED_EDGE('',*,*,#6230,.T.);
#8374=ORIENTED_EDGE('',*,*,#6231,.T.);
#8375=ORIENTED_EDGE('',*,*,#6232,.T.);
#8376=ORIENTED_EDGE('',*,*,#6233,.T.);
#8377=ORIENTED_EDGE('',*,*,#6234,.T.);
#8378=ORIENTED_EDGE('',*,*,#6235,.T.);
#8379=ORIENTED_EDGE('',*,*,#6236,.T.);
#8380=ORIENTED_EDGE('',*,*,#6237,.T.);
#8381=ORIENTED_EDGE('',*,*,#6238,.T.);
#8382=ORIENTED_EDGE('',*,*,#6239,.T.);
#8383=ORIENTED_EDGE('',*,*,#6240,.T.);
#8384=ORIENTED_EDGE('',*,*,#6241,.T.);
#8385=ORIENTED_EDGE('',*,*,#6242,.T.);
#8386=ORIENTED_EDGE('',*,*,#6243,.T.);
#8387=ORIENTED_EDGE('',*,*,#6244,.T.);
#8388=ORIENTED_EDGE('',*,*,#6245,.T.);
#8389=ORIENTED_EDGE('',*,*,#6246,.T.);
#8390=ORIENTED_EDGE('',*,*,#6247,.T.);
#8391=ORIENTED_EDGE('',*,*,#6173,.T.);
#8392=ORIENTED_EDGE('',*,*,#6050,.T.);
#8393=ORIENTED_EDGE('',*,*,#6171,.T.);
#8394=ORIENTED_EDGE('',*,*,#6110,.T.);
#8395=ORIENTED_EDGE('',*,*,#6248,.F.);
#8396=ORIENTED_EDGE('',*,*,#6249,.F.);
#8397=ORIENTED_EDGE('',*,*,#6250,.F.);
#8398=ORIENTED_EDGE('',*,*,#6251,.F.);
#8399=ORIENTED_EDGE('',*,*,#6252,.F.);
#8400=ORIENTED_EDGE('',*,*,#6253,.F.);
#8401=ORIENTED_EDGE('',*,*,#6254,.F.);
#8402=ORIENTED_EDGE('',*,*,#6255,.F.);
#8403=ORIENTED_EDGE('',*,*,#6256,.F.);
#8404=ORIENTED_EDGE('',*,*,#6257,.F.);
#8405=ORIENTED_EDGE('',*,*,#6258,.F.);
#8406=ORIENTED_EDGE('',*,*,#6259,.F.);
#8407=ORIENTED_EDGE('',*,*,#6260,.F.);
#8408=ORIENTED_EDGE('',*,*,#6261,.F.);
#8409=ORIENTED_EDGE('',*,*,#6262,.F.);
#8410=ORIENTED_EDGE('',*,*,#6263,.F.);
#8411=ORIENTED_EDGE('',*,*,#6264,.F.);
#8412=ORIENTED_EDGE('',*,*,#6265,.F.);
#8413=ORIENTED_EDGE('',*,*,#6266,.F.);
#8414=ORIENTED_EDGE('',*,*,#6267,.F.);
#8415=ORIENTED_EDGE('',*,*,#6268,.F.);
#8416=ORIENTED_EDGE('',*,*,#6269,.F.);
#8417=ORIENTED_EDGE('',*,*,#6270,.F.);
#8418=ORIENTED_EDGE('',*,*,#6271,.F.);
#8419=ORIENTED_EDGE('',*,*,#6272,.F.);
#8420=ORIENTED_EDGE('',*,*,#6273,.F.);
#8421=ORIENTED_EDGE('',*,*,#6274,.F.);
#8422=ORIENTED_EDGE('',*,*,#6275,.F.);
#8423=ORIENTED_EDGE('',*,*,#6276,.F.);
#8424=ORIENTED_EDGE('',*,*,#6277,.F.);
#8425=ORIENTED_EDGE('',*,*,#6278,.F.);
#8426=ORIENTED_EDGE('',*,*,#6279,.F.);
#8427=ORIENTED_EDGE('',*,*,#6280,.F.);
#8428=ORIENTED_EDGE('',*,*,#6281,.F.);
#8429=ORIENTED_EDGE('',*,*,#6282,.F.);
#8430=ORIENTED_EDGE('',*,*,#6283,.F.);
#8431=ORIENTED_EDGE('',*,*,#6284,.F.);
#8432=ORIENTED_EDGE('',*,*,#6285,.F.);
#8433=ORIENTED_EDGE('',*,*,#6286,.F.);
#8434=ORIENTED_EDGE('',*,*,#6287,.F.);
#8435=ORIENTED_EDGE('',*,*,#6288,.F.);
#8436=ORIENTED_EDGE('',*,*,#6289,.F.);
#8437=ORIENTED_EDGE('',*,*,#6290,.F.);
#8438=ORIENTED_EDGE('',*,*,#6291,.F.);
#8439=ORIENTED_EDGE('',*,*,#6292,.F.);
#8440=ORIENTED_EDGE('',*,*,#6293,.F.);
#8441=ORIENTED_EDGE('',*,*,#6294,.F.);
#8442=ORIENTED_EDGE('',*,*,#6295,.F.);
#8443=ORIENTED_EDGE('',*,*,#6296,.F.);
#8444=ORIENTED_EDGE('',*,*,#6297,.F.);
#8445=ORIENTED_EDGE('',*,*,#6298,.F.);
#8446=ORIENTED_EDGE('',*,*,#6299,.F.);
#8447=ORIENTED_EDGE('',*,*,#6300,.F.);
#8448=ORIENTED_EDGE('',*,*,#6301,.F.);
#8449=ORIENTED_EDGE('',*,*,#6302,.F.);
#8450=ORIENTED_EDGE('',*,*,#6303,.F.);
#8451=ORIENTED_EDGE('',*,*,#6304,.F.);
#8452=ORIENTED_EDGE('',*,*,#6305,.F.);
#8453=ORIENTED_EDGE('',*,*,#6306,.F.);
#8454=ORIENTED_EDGE('',*,*,#6307,.F.);
#8455=ORIENTED_EDGE('',*,*,#6308,.F.);
#8456=ORIENTED_EDGE('',*,*,#6309,.F.);
#8457=ORIENTED_EDGE('',*,*,#6310,.F.);
#8458=ORIENTED_EDGE('',*,*,#6311,.F.);
#8459=ORIENTED_EDGE('',*,*,#6312,.F.);
#8460=ORIENTED_EDGE('',*,*,#6313,.F.);
#8461=ORIENTED_EDGE('',*,*,#6314,.F.);
#8462=ORIENTED_EDGE('',*,*,#6315,.F.);
#8463=ORIENTED_EDGE('',*,*,#6316,.F.);
#8464=ORIENTED_EDGE('',*,*,#6317,.F.);
#8465=ORIENTED_EDGE('',*,*,#6318,.F.);
#8466=ORIENTED_EDGE('',*,*,#6319,.F.);
#8467=ORIENTED_EDGE('',*,*,#6320,.F.);
#8468=ORIENTED_EDGE('',*,*,#6184,.F.);
#8469=ORIENTED_EDGE('',*,*,#6321,.F.);
#8470=ORIENTED_EDGE('',*,*,#6322,.F.);
#8471=ORIENTED_EDGE('',*,*,#6323,.F.);
#8472=ORIENTED_EDGE('',*,*,#6309,.T.);
#8473=ORIENTED_EDGE('',*,*,#6324,.F.);
#8474=ORIENTED_EDGE('',*,*,#6325,.F.);
#8475=ORIENTED_EDGE('',*,*,#6326,.F.);
#8476=ORIENTED_EDGE('',*,*,#6188,.F.);
#8477=ORIENTED_EDGE('',*,*,#6327,.F.);
#8478=ORIENTED_EDGE('',*,*,#6328,.F.);
#8479=ORIENTED_EDGE('',*,*,#6329,.F.);
#8480=ORIENTED_EDGE('',*,*,#6305,.T.);
#8481=ORIENTED_EDGE('',*,*,#6330,.F.);
#8482=ORIENTED_EDGE('',*,*,#6331,.F.);
#8483=ORIENTED_EDGE('',*,*,#6332,.F.);
#8484=ORIENTED_EDGE('',*,*,#6192,.F.);
#8485=ORIENTED_EDGE('',*,*,#6333,.F.);
#8486=ORIENTED_EDGE('',*,*,#6334,.F.);
#8487=ORIENTED_EDGE('',*,*,#6335,.F.);
#8488=ORIENTED_EDGE('',*,*,#6301,.T.);
#8489=ORIENTED_EDGE('',*,*,#6336,.F.);
#8490=ORIENTED_EDGE('',*,*,#6337,.F.);
#8491=ORIENTED_EDGE('',*,*,#6338,.F.);
#8492=ORIENTED_EDGE('',*,*,#6196,.F.);
#8493=ORIENTED_EDGE('',*,*,#6339,.F.);
#8494=ORIENTED_EDGE('',*,*,#6340,.F.);
#8495=ORIENTED_EDGE('',*,*,#6341,.F.);
#8496=ORIENTED_EDGE('',*,*,#6297,.T.);
#8497=ORIENTED_EDGE('',*,*,#6342,.F.);
#8498=ORIENTED_EDGE('',*,*,#6343,.F.);
#8499=ORIENTED_EDGE('',*,*,#6344,.F.);
#8500=ORIENTED_EDGE('',*,*,#6200,.F.);
#8501=ORIENTED_EDGE('',*,*,#6345,.F.);
#8502=ORIENTED_EDGE('',*,*,#6346,.F.);
#8503=ORIENTED_EDGE('',*,*,#6347,.F.);
#8504=ORIENTED_EDGE('',*,*,#6293,.T.);
#8505=ORIENTED_EDGE('',*,*,#6348,.F.);
#8506=ORIENTED_EDGE('',*,*,#6349,.F.);
#8507=ORIENTED_EDGE('',*,*,#6350,.F.);
#8508=ORIENTED_EDGE('',*,*,#6204,.F.);
#8509=ORIENTED_EDGE('',*,*,#6351,.F.);
#8510=ORIENTED_EDGE('',*,*,#6352,.F.);
#8511=ORIENTED_EDGE('',*,*,#6353,.F.);
#8512=ORIENTED_EDGE('',*,*,#6289,.T.);
#8513=ORIENTED_EDGE('',*,*,#6354,.F.);
#8514=ORIENTED_EDGE('',*,*,#6355,.F.);
#8515=ORIENTED_EDGE('',*,*,#6356,.F.);
#8516=ORIENTED_EDGE('',*,*,#6208,.F.);
#8517=ORIENTED_EDGE('',*,*,#6357,.F.);
#8518=ORIENTED_EDGE('',*,*,#6358,.F.);
#8519=ORIENTED_EDGE('',*,*,#6359,.F.);
#8520=ORIENTED_EDGE('',*,*,#6285,.T.);
#8521=ORIENTED_EDGE('',*,*,#6360,.F.);
#8522=ORIENTED_EDGE('',*,*,#6361,.F.);
#8523=ORIENTED_EDGE('',*,*,#6362,.F.);
#8524=ORIENTED_EDGE('',*,*,#6212,.F.);
#8525=ORIENTED_EDGE('',*,*,#6363,.F.);
#8526=ORIENTED_EDGE('',*,*,#6364,.F.);
#8527=ORIENTED_EDGE('',*,*,#6365,.F.);
#8528=ORIENTED_EDGE('',*,*,#6281,.T.);
#8529=ORIENTED_EDGE('',*,*,#6366,.F.);
#8530=ORIENTED_EDGE('',*,*,#6367,.F.);
#8531=ORIENTED_EDGE('',*,*,#6368,.F.);
#8532=ORIENTED_EDGE('',*,*,#6216,.F.);
#8533=ORIENTED_EDGE('',*,*,#6369,.F.);
#8534=ORIENTED_EDGE('',*,*,#6370,.F.);
#8535=ORIENTED_EDGE('',*,*,#6371,.F.);
#8536=ORIENTED_EDGE('',*,*,#6277,.T.);
#8537=ORIENTED_EDGE('',*,*,#6372,.F.);
#8538=ORIENTED_EDGE('',*,*,#6373,.F.);
#8539=ORIENTED_EDGE('',*,*,#6374,.F.);
#8540=ORIENTED_EDGE('',*,*,#6220,.F.);
#8541=ORIENTED_EDGE('',*,*,#6375,.F.);
#8542=ORIENTED_EDGE('',*,*,#6376,.F.);
#8543=ORIENTED_EDGE('',*,*,#6377,.F.);
#8544=ORIENTED_EDGE('',*,*,#6273,.T.);
#8545=ORIENTED_EDGE('',*,*,#6378,.F.);
#8546=ORIENTED_EDGE('',*,*,#6379,.F.);
#8547=ORIENTED_EDGE('',*,*,#6380,.F.);
#8548=ORIENTED_EDGE('',*,*,#6224,.F.);
#8549=ORIENTED_EDGE('',*,*,#6381,.F.);
#8550=ORIENTED_EDGE('',*,*,#6382,.F.);
#8551=ORIENTED_EDGE('',*,*,#6383,.F.);
#8552=ORIENTED_EDGE('',*,*,#6269,.T.);
#8553=ORIENTED_EDGE('',*,*,#6384,.F.);
#8554=ORIENTED_EDGE('',*,*,#6385,.F.);
#8555=ORIENTED_EDGE('',*,*,#6386,.F.);
#8556=ORIENTED_EDGE('',*,*,#6228,.F.);
#8557=ORIENTED_EDGE('',*,*,#6387,.F.);
#8558=ORIENTED_EDGE('',*,*,#6388,.F.);
#8559=ORIENTED_EDGE('',*,*,#6389,.F.);
#8560=ORIENTED_EDGE('',*,*,#6265,.T.);
#8561=ORIENTED_EDGE('',*,*,#6390,.F.);
#8562=ORIENTED_EDGE('',*,*,#6391,.F.);
#8563=ORIENTED_EDGE('',*,*,#6392,.F.);
#8564=ORIENTED_EDGE('',*,*,#6232,.F.);
#8565=ORIENTED_EDGE('',*,*,#6393,.F.);
#8566=ORIENTED_EDGE('',*,*,#6394,.F.);
#8567=ORIENTED_EDGE('',*,*,#6395,.F.);
#8568=ORIENTED_EDGE('',*,*,#6261,.T.);
#8569=ORIENTED_EDGE('',*,*,#6396,.F.);
#8570=ORIENTED_EDGE('',*,*,#6397,.F.);
#8571=ORIENTED_EDGE('',*,*,#6398,.F.);
#8572=ORIENTED_EDGE('',*,*,#6236,.F.);
#8573=ORIENTED_EDGE('',*,*,#6399,.F.);
#8574=ORIENTED_EDGE('',*,*,#6400,.F.);
#8575=ORIENTED_EDGE('',*,*,#6401,.F.);
#8576=ORIENTED_EDGE('',*,*,#6257,.T.);
#8577=ORIENTED_EDGE('',*,*,#6402,.F.);
#8578=ORIENTED_EDGE('',*,*,#6403,.F.);
#8579=ORIENTED_EDGE('',*,*,#6404,.F.);
#8580=ORIENTED_EDGE('',*,*,#6240,.F.);
#8581=ORIENTED_EDGE('',*,*,#6405,.F.);
#8582=ORIENTED_EDGE('',*,*,#6406,.F.);
#8583=ORIENTED_EDGE('',*,*,#6407,.F.);
#8584=ORIENTED_EDGE('',*,*,#6253,.T.);
#8585=ORIENTED_EDGE('',*,*,#6408,.F.);
#8586=ORIENTED_EDGE('',*,*,#6409,.F.);
#8587=ORIENTED_EDGE('',*,*,#6410,.F.);
#8588=ORIENTED_EDGE('',*,*,#6244,.F.);
#8589=ORIENTED_EDGE('',*,*,#6411,.F.);
#8590=ORIENTED_EDGE('',*,*,#6412,.F.);
#8591=ORIENTED_EDGE('',*,*,#6413,.F.);
#8592=ORIENTED_EDGE('',*,*,#6249,.T.);
#8593=ORIENTED_EDGE('',*,*,#6414,.F.);
#8594=ORIENTED_EDGE('',*,*,#6415,.F.);
#8595=ORIENTED_EDGE('',*,*,#6416,.F.);
#8596=ORIENTED_EDGE('',*,*,#6180,.F.);
#8597=ORIENTED_EDGE('',*,*,#6417,.F.);
#8598=ORIENTED_EDGE('',*,*,#6418,.F.);
#8599=ORIENTED_EDGE('',*,*,#6419,.F.);
#8600=ORIENTED_EDGE('',*,*,#6313,.T.);
#8601=ORIENTED_EDGE('',*,*,#6420,.F.);
#8602=ORIENTED_EDGE('',*,*,#6421,.F.);
#8603=ORIENTED_EDGE('',*,*,#6422,.F.);
#8604=ORIENTED_EDGE('',*,*,#6176,.F.);
#8605=ORIENTED_EDGE('',*,*,#6423,.F.);
#8606=ORIENTED_EDGE('',*,*,#6424,.F.);
#8607=ORIENTED_EDGE('',*,*,#6425,.F.);
#8608=ORIENTED_EDGE('',*,*,#6317,.T.);
#8609=ORIENTED_EDGE('',*,*,#6426,.F.);
#8610=ORIENTED_EDGE('',*,*,#6427,.F.);
#8611=ORIENTED_EDGE('',*,*,#6428,.F.);
#8612=ORIENTED_EDGE('',*,*,#6429,.F.);
#8613=ORIENTED_EDGE('',*,*,#6430,.F.);
#8614=ORIENTED_EDGE('',*,*,#6431,.F.);
#8615=ORIENTED_EDGE('',*,*,#6432,.F.);
#8616=ORIENTED_EDGE('',*,*,#6433,.F.);
#8617=ORIENTED_EDGE('',*,*,#6434,.F.);
#8618=ORIENTED_EDGE('',*,*,#6435,.F.);
#8619=ORIENTED_EDGE('',*,*,#6436,.F.);
#8620=ORIENTED_EDGE('',*,*,#6437,.F.);
#8621=ORIENTED_EDGE('',*,*,#6438,.F.);
#8622=ORIENTED_EDGE('',*,*,#6439,.F.);
#8623=ORIENTED_EDGE('',*,*,#6440,.F.);
#8624=ORIENTED_EDGE('',*,*,#6441,.F.);
#8625=ORIENTED_EDGE('',*,*,#6442,.F.);
#8626=ORIENTED_EDGE('',*,*,#6443,.F.);
#8627=ORIENTED_EDGE('',*,*,#6444,.F.);
#8628=ORIENTED_EDGE('',*,*,#6445,.F.);
#8629=ORIENTED_EDGE('',*,*,#6446,.F.);
#8630=ORIENTED_EDGE('',*,*,#6447,.F.);
#8631=ORIENTED_EDGE('',*,*,#6448,.F.);
#8632=ORIENTED_EDGE('',*,*,#6449,.F.);
#8633=ORIENTED_EDGE('',*,*,#6450,.F.);
#8634=ORIENTED_EDGE('',*,*,#6451,.F.);
#8635=ORIENTED_EDGE('',*,*,#6452,.F.);
#8636=ORIENTED_EDGE('',*,*,#6453,.F.);
#8637=ORIENTED_EDGE('',*,*,#6454,.F.);
#8638=ORIENTED_EDGE('',*,*,#6455,.F.);
#8639=ORIENTED_EDGE('',*,*,#6456,.F.);
#8640=ORIENTED_EDGE('',*,*,#6457,.F.);
#8641=ORIENTED_EDGE('',*,*,#6458,.F.);
#8642=ORIENTED_EDGE('',*,*,#6459,.F.);
#8643=ORIENTED_EDGE('',*,*,#6460,.F.);
#8644=ORIENTED_EDGE('',*,*,#6461,.F.);
#8645=ORIENTED_EDGE('',*,*,#6462,.F.);
#8646=ORIENTED_EDGE('',*,*,#6463,.F.);
#8647=ORIENTED_EDGE('',*,*,#6464,.F.);
#8648=ORIENTED_EDGE('',*,*,#6465,.F.);
#8649=ORIENTED_EDGE('',*,*,#6466,.F.);
#8650=ORIENTED_EDGE('',*,*,#6467,.F.);
#8651=ORIENTED_EDGE('',*,*,#6468,.F.);
#8652=ORIENTED_EDGE('',*,*,#6469,.F.);
#8653=ORIENTED_EDGE('',*,*,#6470,.F.);
#8654=ORIENTED_EDGE('',*,*,#6471,.F.);
#8655=ORIENTED_EDGE('',*,*,#6472,.F.);
#8656=ORIENTED_EDGE('',*,*,#6473,.F.);
#8657=ORIENTED_EDGE('',*,*,#6474,.F.);
#8658=ORIENTED_EDGE('',*,*,#6475,.F.);
#8659=ORIENTED_EDGE('',*,*,#6476,.F.);
#8660=ORIENTED_EDGE('',*,*,#6477,.F.);
#8661=ORIENTED_EDGE('',*,*,#6478,.F.);
#8662=ORIENTED_EDGE('',*,*,#6479,.F.);
#8663=ORIENTED_EDGE('',*,*,#6480,.F.);
#8664=ORIENTED_EDGE('',*,*,#6481,.F.);
#8665=ORIENTED_EDGE('',*,*,#6482,.F.);
#8666=ORIENTED_EDGE('',*,*,#6483,.F.);
#8667=ORIENTED_EDGE('',*,*,#6484,.F.);
#8668=ORIENTED_EDGE('',*,*,#6485,.F.);
#8669=ORIENTED_EDGE('',*,*,#6486,.F.);
#8670=ORIENTED_EDGE('',*,*,#6487,.F.);
#8671=ORIENTED_EDGE('',*,*,#6488,.F.);
#8672=ORIENTED_EDGE('',*,*,#6489,.F.);
#8673=ORIENTED_EDGE('',*,*,#6490,.F.);
#8674=ORIENTED_EDGE('',*,*,#6491,.F.);
#8675=ORIENTED_EDGE('',*,*,#6492,.F.);
#8676=ORIENTED_EDGE('',*,*,#6493,.F.);
#8677=ORIENTED_EDGE('',*,*,#6494,.F.);
#8678=ORIENTED_EDGE('',*,*,#6495,.F.);
#8679=ORIENTED_EDGE('',*,*,#6496,.F.);
#8680=ORIENTED_EDGE('',*,*,#6497,.F.);
#8681=ORIENTED_EDGE('',*,*,#6498,.F.);
#8682=ORIENTED_EDGE('',*,*,#6499,.F.);
#8683=ORIENTED_EDGE('',*,*,#6500,.F.);
#8684=ORIENTED_EDGE('',*,*,#6501,.F.);
#8685=ORIENTED_EDGE('',*,*,#6502,.F.);
#8686=ORIENTED_EDGE('',*,*,#6503,.F.);
#8687=ORIENTED_EDGE('',*,*,#6504,.F.);
#8688=ORIENTED_EDGE('',*,*,#6505,.F.);
#8689=ORIENTED_EDGE('',*,*,#6506,.F.);
#8690=ORIENTED_EDGE('',*,*,#6507,.F.);
#8691=ORIENTED_EDGE('',*,*,#6508,.F.);
#8692=ORIENTED_EDGE('',*,*,#6509,.F.);
#8693=ORIENTED_EDGE('',*,*,#6510,.F.);
#8694=ORIENTED_EDGE('',*,*,#6511,.F.);
#8695=ORIENTED_EDGE('',*,*,#6512,.F.);
#8696=ORIENTED_EDGE('',*,*,#6513,.F.);
#8697=ORIENTED_EDGE('',*,*,#6514,.F.);
#8698=ORIENTED_EDGE('',*,*,#6515,.F.);
#8699=ORIENTED_EDGE('',*,*,#6516,.F.);
#8700=ORIENTED_EDGE('',*,*,#6517,.F.);
#8701=ORIENTED_EDGE('',*,*,#6518,.F.);
#8702=ORIENTED_EDGE('',*,*,#6519,.F.);
#8703=ORIENTED_EDGE('',*,*,#6520,.F.);
#8704=ORIENTED_EDGE('',*,*,#6521,.F.);
#8705=ORIENTED_EDGE('',*,*,#6522,.F.);
#8706=ORIENTED_EDGE('',*,*,#6523,.F.);
#8707=ORIENTED_EDGE('',*,*,#6524,.F.);
#8708=ORIENTED_EDGE('',*,*,#6525,.F.);
#8709=ORIENTED_EDGE('',*,*,#6526,.F.);
#8710=ORIENTED_EDGE('',*,*,#6527,.F.);
#8711=ORIENTED_EDGE('',*,*,#6528,.F.);
#8712=ORIENTED_EDGE('',*,*,#6529,.F.);
#8713=ORIENTED_EDGE('',*,*,#6530,.F.);
#8714=ORIENTED_EDGE('',*,*,#6531,.F.);
#8715=ORIENTED_EDGE('',*,*,#6532,.F.);
#8716=ORIENTED_EDGE('',*,*,#6533,.F.);
#8717=ORIENTED_EDGE('',*,*,#6534,.F.);
#8718=ORIENTED_EDGE('',*,*,#6535,.F.);
#8719=ORIENTED_EDGE('',*,*,#6536,.F.);
#8720=ORIENTED_EDGE('',*,*,#6537,.F.);
#8721=ORIENTED_EDGE('',*,*,#6538,.F.);
#8722=ORIENTED_EDGE('',*,*,#6539,.F.);
#8723=ORIENTED_EDGE('',*,*,#6540,.F.);
#8724=ORIENTED_EDGE('',*,*,#6541,.F.);
#8725=ORIENTED_EDGE('',*,*,#6542,.F.);
#8726=ORIENTED_EDGE('',*,*,#6543,.F.);
#8727=ORIENTED_EDGE('',*,*,#6544,.F.);
#8728=ORIENTED_EDGE('',*,*,#6545,.F.);
#8729=ORIENTED_EDGE('',*,*,#6546,.F.);
#8730=ORIENTED_EDGE('',*,*,#6547,.F.);
#8731=ORIENTED_EDGE('',*,*,#6548,.F.);
#8732=ORIENTED_EDGE('',*,*,#6549,.F.);
#8733=ORIENTED_EDGE('',*,*,#6550,.F.);
#8734=ORIENTED_EDGE('',*,*,#6551,.F.);
#8735=ORIENTED_EDGE('',*,*,#6552,.F.);
#8736=ORIENTED_EDGE('',*,*,#6553,.F.);
#8737=ORIENTED_EDGE('',*,*,#6554,.F.);
#8738=ORIENTED_EDGE('',*,*,#6555,.F.);
#8739=ORIENTED_EDGE('',*,*,#6556,.F.);
#8740=ORIENTED_EDGE('',*,*,#6557,.F.);
#8741=ORIENTED_EDGE('',*,*,#6558,.F.);
#8742=ORIENTED_EDGE('',*,*,#6559,.F.);
#8743=ORIENTED_EDGE('',*,*,#6560,.F.);
#8744=ORIENTED_EDGE('',*,*,#6561,.F.);
#8745=ORIENTED_EDGE('',*,*,#6562,.F.);
#8746=ORIENTED_EDGE('',*,*,#6563,.F.);
#8747=ORIENTED_EDGE('',*,*,#6564,.F.);
#8748=ORIENTED_EDGE('',*,*,#6565,.F.);
#8749=ORIENTED_EDGE('',*,*,#6566,.F.);
#8750=ORIENTED_EDGE('',*,*,#6567,.F.);
#8751=ORIENTED_EDGE('',*,*,#6568,.F.);
#8752=ORIENTED_EDGE('',*,*,#6569,.F.);
#8753=ORIENTED_EDGE('',*,*,#6570,.F.);
#8754=ORIENTED_EDGE('',*,*,#6571,.F.);
#8755=ORIENTED_EDGE('',*,*,#6572,.F.);
#8756=ORIENTED_EDGE('',*,*,#6433,.T.);
#8757=ORIENTED_EDGE('',*,*,#6573,.F.);
#8758=ORIENTED_EDGE('',*,*,#6574,.F.);
#8759=ORIENTED_EDGE('',*,*,#6575,.F.);
#8760=ORIENTED_EDGE('',*,*,#6441,.T.);
#8761=ORIENTED_EDGE('',*,*,#6576,.F.);
#8762=ORIENTED_EDGE('',*,*,#6577,.F.);
#8763=ORIENTED_EDGE('',*,*,#6578,.F.);
#8764=ORIENTED_EDGE('',*,*,#6449,.T.);
#8765=ORIENTED_EDGE('',*,*,#6579,.F.);
#8766=ORIENTED_EDGE('',*,*,#6580,.F.);
#8767=ORIENTED_EDGE('',*,*,#6581,.F.);
#8768=ORIENTED_EDGE('',*,*,#6457,.T.);
#8769=ORIENTED_EDGE('',*,*,#6582,.F.);
#8770=ORIENTED_EDGE('',*,*,#6583,.F.);
#8771=ORIENTED_EDGE('',*,*,#6584,.F.);
#8772=ORIENTED_EDGE('',*,*,#6465,.T.);
#8773=ORIENTED_EDGE('',*,*,#6585,.F.);
#8774=ORIENTED_EDGE('',*,*,#6586,.F.);
#8775=ORIENTED_EDGE('',*,*,#6587,.F.);
#8776=ORIENTED_EDGE('',*,*,#6473,.T.);
#8777=ORIENTED_EDGE('',*,*,#6588,.F.);
#8778=ORIENTED_EDGE('',*,*,#6589,.F.);
#8779=ORIENTED_EDGE('',*,*,#6590,.F.);
#8780=ORIENTED_EDGE('',*,*,#6481,.T.);
#8781=ORIENTED_EDGE('',*,*,#6591,.F.);
#8782=ORIENTED_EDGE('',*,*,#6592,.F.);
#8783=ORIENTED_EDGE('',*,*,#6593,.F.);
#8784=ORIENTED_EDGE('',*,*,#6489,.T.);
#8785=ORIENTED_EDGE('',*,*,#6594,.F.);
#8786=ORIENTED_EDGE('',*,*,#6595,.F.);
#8787=ORIENTED_EDGE('',*,*,#6596,.F.);
#8788=ORIENTED_EDGE('',*,*,#6497,.T.);
#8789=ORIENTED_EDGE('',*,*,#6597,.F.);
#8790=ORIENTED_EDGE('',*,*,#6598,.F.);
#8791=ORIENTED_EDGE('',*,*,#6599,.F.);
#8792=ORIENTED_EDGE('',*,*,#6505,.T.);
#8793=ORIENTED_EDGE('',*,*,#6600,.F.);
#8794=ORIENTED_EDGE('',*,*,#6601,.F.);
#8795=ORIENTED_EDGE('',*,*,#6602,.F.);
#8796=ORIENTED_EDGE('',*,*,#6513,.T.);
#8797=ORIENTED_EDGE('',*,*,#6603,.F.);
#8798=ORIENTED_EDGE('',*,*,#6604,.F.);
#8799=ORIENTED_EDGE('',*,*,#6605,.F.);
#8800=ORIENTED_EDGE('',*,*,#6521,.T.);
#8801=ORIENTED_EDGE('',*,*,#6606,.F.);
#8802=ORIENTED_EDGE('',*,*,#6607,.F.);
#8803=ORIENTED_EDGE('',*,*,#6608,.F.);
#8804=ORIENTED_EDGE('',*,*,#6529,.T.);
#8805=ORIENTED_EDGE('',*,*,#6609,.F.);
#8806=ORIENTED_EDGE('',*,*,#6610,.F.);
#8807=ORIENTED_EDGE('',*,*,#6611,.F.);
#8808=ORIENTED_EDGE('',*,*,#6537,.T.);
#8809=ORIENTED_EDGE('',*,*,#6612,.F.);
#8810=ORIENTED_EDGE('',*,*,#6613,.F.);
#8811=ORIENTED_EDGE('',*,*,#6614,.F.);
#8812=ORIENTED_EDGE('',*,*,#6545,.T.);
#8813=ORIENTED_EDGE('',*,*,#6615,.F.);
#8814=ORIENTED_EDGE('',*,*,#6616,.F.);
#8815=ORIENTED_EDGE('',*,*,#6617,.F.);
#8816=ORIENTED_EDGE('',*,*,#6553,.T.);
#8817=ORIENTED_EDGE('',*,*,#6618,.F.);
#8818=ORIENTED_EDGE('',*,*,#6619,.F.);
#8819=ORIENTED_EDGE('',*,*,#6620,.F.);
#8820=ORIENTED_EDGE('',*,*,#6561,.T.);
#8821=ORIENTED_EDGE('',*,*,#6621,.F.);
#8822=ORIENTED_EDGE('',*,*,#6622,.F.);
#8823=ORIENTED_EDGE('',*,*,#6623,.F.);
#8824=ORIENTED_EDGE('',*,*,#6569,.T.);
#8825=ORIENTED_EDGE('',*,*,#6624,.F.);
#8826=ORIENTED_EDGE('',*,*,#6625,.F.);
#8827=ORIENTED_EDGE('',*,*,#6626,.F.);
#8828=ORIENTED_EDGE('',*,*,#6627,.F.);
#8829=ORIENTED_EDGE('',*,*,#6628,.F.);
#8830=ORIENTED_EDGE('',*,*,#6629,.F.);
#8831=ORIENTED_EDGE('',*,*,#6630,.F.);
#8832=ORIENTED_EDGE('',*,*,#6631,.F.);
#8833=ORIENTED_EDGE('',*,*,#6632,.F.);
#8834=ORIENTED_EDGE('',*,*,#6633,.F.);
#8835=ORIENTED_EDGE('',*,*,#6634,.F.);
#8836=ORIENTED_EDGE('',*,*,#6635,.F.);
#8837=ORIENTED_EDGE('',*,*,#6636,.F.);
#8838=ORIENTED_EDGE('',*,*,#6637,.F.);
#8839=ORIENTED_EDGE('',*,*,#6638,.F.);
#8840=ORIENTED_EDGE('',*,*,#6639,.F.);
#8841=ORIENTED_EDGE('',*,*,#6640,.F.);
#8842=ORIENTED_EDGE('',*,*,#6641,.F.);
#8843=ORIENTED_EDGE('',*,*,#6642,.F.);
#8844=ORIENTED_EDGE('',*,*,#6643,.F.);
#8845=ORIENTED_EDGE('',*,*,#6644,.F.);
#8846=ORIENTED_EDGE('',*,*,#6645,.F.);
#8847=ORIENTED_EDGE('',*,*,#6646,.F.);
#8848=ORIENTED_EDGE('',*,*,#6647,.F.);
#8849=ORIENTED_EDGE('',*,*,#6648,.F.);
#8850=ORIENTED_EDGE('',*,*,#6649,.F.);
#8851=ORIENTED_EDGE('',*,*,#6650,.F.);
#8852=ORIENTED_EDGE('',*,*,#6651,.F.);
#8853=ORIENTED_EDGE('',*,*,#6652,.F.);
#8854=ORIENTED_EDGE('',*,*,#6653,.F.);
#8855=ORIENTED_EDGE('',*,*,#6654,.F.);
#8856=ORIENTED_EDGE('',*,*,#6655,.F.);
#8857=ORIENTED_EDGE('',*,*,#6656,.F.);
#8858=ORIENTED_EDGE('',*,*,#6657,.F.);
#8859=ORIENTED_EDGE('',*,*,#6658,.F.);
#8860=ORIENTED_EDGE('',*,*,#6659,.F.);
#8861=ORIENTED_EDGE('',*,*,#6660,.F.);
#8862=ORIENTED_EDGE('',*,*,#6661,.F.);
#8863=ORIENTED_EDGE('',*,*,#6662,.F.);
#8864=ORIENTED_EDGE('',*,*,#6663,.F.);
#8865=ORIENTED_EDGE('',*,*,#6664,.F.);
#8866=ORIENTED_EDGE('',*,*,#6665,.F.);
#8867=ORIENTED_EDGE('',*,*,#6666,.F.);
#8868=ORIENTED_EDGE('',*,*,#6667,.F.);
#8869=ORIENTED_EDGE('',*,*,#6668,.F.);
#8870=ORIENTED_EDGE('',*,*,#6669,.F.);
#8871=ORIENTED_EDGE('',*,*,#6670,.F.);
#8872=ORIENTED_EDGE('',*,*,#6671,.F.);
#8873=ORIENTED_EDGE('',*,*,#6672,.F.);
#8874=ORIENTED_EDGE('',*,*,#6673,.F.);
#8875=ORIENTED_EDGE('',*,*,#6674,.F.);
#8876=ORIENTED_EDGE('',*,*,#6675,.F.);
#8877=ORIENTED_EDGE('',*,*,#6676,.F.);
#8878=ORIENTED_EDGE('',*,*,#6677,.F.);
#8879=ORIENTED_EDGE('',*,*,#6678,.F.);
#8880=ORIENTED_EDGE('',*,*,#6679,.F.);
#8881=ORIENTED_EDGE('',*,*,#6680,.F.);
#8882=ORIENTED_EDGE('',*,*,#6681,.F.);
#8883=ORIENTED_EDGE('',*,*,#6682,.F.);
#8884=ORIENTED_EDGE('',*,*,#6683,.F.);
#8885=ORIENTED_EDGE('',*,*,#6684,.F.);
#8886=ORIENTED_EDGE('',*,*,#6685,.F.);
#8887=ORIENTED_EDGE('',*,*,#6686,.F.);
#8888=ORIENTED_EDGE('',*,*,#6687,.F.);
#8889=ORIENTED_EDGE('',*,*,#6688,.F.);
#8890=ORIENTED_EDGE('',*,*,#6689,.F.);
#8891=ORIENTED_EDGE('',*,*,#6690,.F.);
#8892=ORIENTED_EDGE('',*,*,#6691,.F.);
#8893=ORIENTED_EDGE('',*,*,#6692,.F.);
#8894=ORIENTED_EDGE('',*,*,#6693,.F.);
#8895=ORIENTED_EDGE('',*,*,#6694,.F.);
#8896=ORIENTED_EDGE('',*,*,#6695,.F.);
#8897=ORIENTED_EDGE('',*,*,#6696,.F.);
#8898=ORIENTED_EDGE('',*,*,#6697,.F.);
#8899=ORIENTED_EDGE('',*,*,#6698,.F.);
#8900=ORIENTED_EDGE('',*,*,#6699,.T.);
#8901=ORIENTED_EDGE('',*,*,#6700,.F.);
#8902=ORIENTED_EDGE('',*,*,#6701,.F.);
#8903=ORIENTED_EDGE('',*,*,#6702,.F.);
#8904=ORIENTED_EDGE('',*,*,#6703,.T.);
#8905=ORIENTED_EDGE('',*,*,#6704,.F.);
#8906=ORIENTED_EDGE('',*,*,#6705,.F.);
#8907=ORIENTED_EDGE('',*,*,#6706,.F.);
#8908=ORIENTED_EDGE('',*,*,#6707,.T.);
#8909=ORIENTED_EDGE('',*,*,#6708,.F.);
#8910=ORIENTED_EDGE('',*,*,#6709,.F.);
#8911=ORIENTED_EDGE('',*,*,#6710,.F.);
#8912=ORIENTED_EDGE('',*,*,#6711,.T.);
#8913=ORIENTED_EDGE('',*,*,#6712,.F.);
#8914=ORIENTED_EDGE('',*,*,#6713,.F.);
#8915=ORIENTED_EDGE('',*,*,#6714,.F.);
#8916=ORIENTED_EDGE('',*,*,#6715,.T.);
#8917=ORIENTED_EDGE('',*,*,#6716,.F.);
#8918=ORIENTED_EDGE('',*,*,#6717,.F.);
#8919=ORIENTED_EDGE('',*,*,#6718,.F.);
#8920=ORIENTED_EDGE('',*,*,#6719,.T.);
#8921=ORIENTED_EDGE('',*,*,#6720,.F.);
#8922=ORIENTED_EDGE('',*,*,#6721,.F.);
#8923=ORIENTED_EDGE('',*,*,#6722,.F.);
#8924=ORIENTED_EDGE('',*,*,#6723,.T.);
#8925=ORIENTED_EDGE('',*,*,#6724,.F.);
#8926=ORIENTED_EDGE('',*,*,#6725,.F.);
#8927=ORIENTED_EDGE('',*,*,#6726,.F.);
#8928=ORIENTED_EDGE('',*,*,#6727,.T.);
#8929=ORIENTED_EDGE('',*,*,#6728,.F.);
#8930=ORIENTED_EDGE('',*,*,#6729,.F.);
#8931=ORIENTED_EDGE('',*,*,#6730,.F.);
#8932=ORIENTED_EDGE('',*,*,#6731,.T.);
#8933=ORIENTED_EDGE('',*,*,#6732,.F.);
#8934=ORIENTED_EDGE('',*,*,#6733,.F.);
#8935=ORIENTED_EDGE('',*,*,#6734,.F.);
#8936=ORIENTED_EDGE('',*,*,#6735,.T.);
#8937=ORIENTED_EDGE('',*,*,#6736,.F.);
#8938=ORIENTED_EDGE('',*,*,#6737,.F.);
#8939=ORIENTED_EDGE('',*,*,#6738,.F.);
#8940=ORIENTED_EDGE('',*,*,#6739,.T.);
#8941=ORIENTED_EDGE('',*,*,#6740,.F.);
#8942=ORIENTED_EDGE('',*,*,#6741,.F.);
#8943=ORIENTED_EDGE('',*,*,#6742,.F.);
#8944=ORIENTED_EDGE('',*,*,#6743,.T.);
#8945=ORIENTED_EDGE('',*,*,#6744,.F.);
#8946=ORIENTED_EDGE('',*,*,#6745,.F.);
#8947=ORIENTED_EDGE('',*,*,#6746,.F.);
#8948=ORIENTED_EDGE('',*,*,#6747,.T.);
#8949=ORIENTED_EDGE('',*,*,#6748,.F.);
#8950=ORIENTED_EDGE('',*,*,#6749,.F.);
#8951=ORIENTED_EDGE('',*,*,#6750,.F.);
#8952=ORIENTED_EDGE('',*,*,#6751,.T.);
#8953=ORIENTED_EDGE('',*,*,#6752,.F.);
#8954=ORIENTED_EDGE('',*,*,#6753,.F.);
#8955=ORIENTED_EDGE('',*,*,#6754,.F.);
#8956=ORIENTED_EDGE('',*,*,#6755,.T.);
#8957=ORIENTED_EDGE('',*,*,#6756,.F.);
#8958=ORIENTED_EDGE('',*,*,#6757,.F.);
#8959=ORIENTED_EDGE('',*,*,#6758,.F.);
#8960=ORIENTED_EDGE('',*,*,#6759,.T.);
#8961=ORIENTED_EDGE('',*,*,#6760,.F.);
#8962=ORIENTED_EDGE('',*,*,#6761,.F.);
#8963=ORIENTED_EDGE('',*,*,#6762,.F.);
#8964=ORIENTED_EDGE('',*,*,#6763,.T.);
#8965=ORIENTED_EDGE('',*,*,#6764,.F.);
#8966=ORIENTED_EDGE('',*,*,#6765,.F.);
#8967=ORIENTED_EDGE('',*,*,#6766,.F.);
#8968=ORIENTED_EDGE('',*,*,#6767,.T.);
#8969=ORIENTED_EDGE('',*,*,#6768,.F.);
#8970=ORIENTED_EDGE('',*,*,#6769,.F.);
#8971=ORIENTED_EDGE('',*,*,#6770,.F.);
#8972=ORIENTED_EDGE('',*,*,#6629,.T.);
#8973=ORIENTED_EDGE('',*,*,#6771,.F.);
#8974=ORIENTED_EDGE('',*,*,#6699,.F.);
#8975=ORIENTED_EDGE('',*,*,#6772,.F.);
#8976=ORIENTED_EDGE('',*,*,#6633,.T.);
#8977=ORIENTED_EDGE('',*,*,#6773,.F.);
#8978=ORIENTED_EDGE('',*,*,#6703,.F.);
#8979=ORIENTED_EDGE('',*,*,#6774,.F.);
#8980=ORIENTED_EDGE('',*,*,#6637,.T.);
#8981=ORIENTED_EDGE('',*,*,#6775,.F.);
#8982=ORIENTED_EDGE('',*,*,#6707,.F.);
#8983=ORIENTED_EDGE('',*,*,#6776,.F.);
#8984=ORIENTED_EDGE('',*,*,#6641,.T.);
#8985=ORIENTED_EDGE('',*,*,#6777,.F.);
#8986=ORIENTED_EDGE('',*,*,#6711,.F.);
#8987=ORIENTED_EDGE('',*,*,#6778,.F.);
#8988=ORIENTED_EDGE('',*,*,#6645,.T.);
#8989=ORIENTED_EDGE('',*,*,#6779,.F.);
#8990=ORIENTED_EDGE('',*,*,#6715,.F.);
#8991=ORIENTED_EDGE('',*,*,#6780,.F.);
#8992=ORIENTED_EDGE('',*,*,#6649,.T.);
#8993=ORIENTED_EDGE('',*,*,#6781,.F.);
#8994=ORIENTED_EDGE('',*,*,#6719,.F.);
#8995=ORIENTED_EDGE('',*,*,#6782,.F.);
#8996=ORIENTED_EDGE('',*,*,#6653,.T.);
#8997=ORIENTED_EDGE('',*,*,#6783,.F.);
#8998=ORIENTED_EDGE('',*,*,#6723,.F.);
#8999=ORIENTED_EDGE('',*,*,#6784,.F.);
#9000=ORIENTED_EDGE('',*,*,#6657,.T.);
#9001=ORIENTED_EDGE('',*,*,#6785,.F.);
#9002=ORIENTED_EDGE('',*,*,#6727,.F.);
#9003=ORIENTED_EDGE('',*,*,#6786,.F.);
#9004=ORIENTED_EDGE('',*,*,#6661,.T.);
#9005=ORIENTED_EDGE('',*,*,#6787,.F.);
#9006=ORIENTED_EDGE('',*,*,#6731,.F.);
#9007=ORIENTED_EDGE('',*,*,#6788,.F.);
#9008=ORIENTED_EDGE('',*,*,#6665,.T.);
#9009=ORIENTED_EDGE('',*,*,#6789,.F.);
#9010=ORIENTED_EDGE('',*,*,#6735,.F.);
#9011=ORIENTED_EDGE('',*,*,#6790,.F.);
#9012=ORIENTED_EDGE('',*,*,#6669,.T.);
#9013=ORIENTED_EDGE('',*,*,#6791,.F.);
#9014=ORIENTED_EDGE('',*,*,#6739,.F.);
#9015=ORIENTED_EDGE('',*,*,#6792,.F.);
#9016=ORIENTED_EDGE('',*,*,#6673,.T.);
#9017=ORIENTED_EDGE('',*,*,#6793,.F.);
#9018=ORIENTED_EDGE('',*,*,#6743,.F.);
#9019=ORIENTED_EDGE('',*,*,#6794,.F.);
#9020=ORIENTED_EDGE('',*,*,#6677,.T.);
#9021=ORIENTED_EDGE('',*,*,#6795,.F.);
#9022=ORIENTED_EDGE('',*,*,#6747,.F.);
#9023=ORIENTED_EDGE('',*,*,#6796,.F.);
#9024=ORIENTED_EDGE('',*,*,#6681,.T.);
#9025=ORIENTED_EDGE('',*,*,#6797,.F.);
#9026=ORIENTED_EDGE('',*,*,#6751,.F.);
#9027=ORIENTED_EDGE('',*,*,#6798,.F.);
#9028=ORIENTED_EDGE('',*,*,#6685,.T.);
#9029=ORIENTED_EDGE('',*,*,#6799,.F.);
#9030=ORIENTED_EDGE('',*,*,#6755,.F.);
#9031=ORIENTED_EDGE('',*,*,#6800,.F.);
#9032=ORIENTED_EDGE('',*,*,#6689,.T.);
#9033=ORIENTED_EDGE('',*,*,#6801,.F.);
#9034=ORIENTED_EDGE('',*,*,#6759,.F.);
#9035=ORIENTED_EDGE('',*,*,#6802,.F.);
#9036=ORIENTED_EDGE('',*,*,#6693,.T.);
#9037=ORIENTED_EDGE('',*,*,#6803,.F.);
#9038=ORIENTED_EDGE('',*,*,#6763,.F.);
#9039=ORIENTED_EDGE('',*,*,#6804,.F.);
#9040=ORIENTED_EDGE('',*,*,#6697,.T.);
#9041=ORIENTED_EDGE('',*,*,#6805,.F.);
#9042=ORIENTED_EDGE('',*,*,#6767,.F.);
#9043=ORIENTED_EDGE('',*,*,#6427,.T.);
#9044=ORIENTED_EDGE('',*,*,#6806,.F.);
#9045=ORIENTED_EDGE('',*,*,#6567,.T.);
#9046=ORIENTED_EDGE('',*,*,#6807,.T.);
#9047=ORIENTED_EDGE('',*,*,#6415,.T.);
#9048=ORIENTED_EDGE('',*,*,#6808,.F.);
#9049=ORIENTED_EDGE('',*,*,#6559,.T.);
#9050=ORIENTED_EDGE('',*,*,#6809,.T.);
#9051=ORIENTED_EDGE('',*,*,#6409,.T.);
#9052=ORIENTED_EDGE('',*,*,#6810,.F.);
#9053=ORIENTED_EDGE('',*,*,#6551,.T.);
#9054=ORIENTED_EDGE('',*,*,#6811,.T.);
#9055=ORIENTED_EDGE('',*,*,#6403,.T.);
#9056=ORIENTED_EDGE('',*,*,#6812,.F.);
#9057=ORIENTED_EDGE('',*,*,#6543,.T.);
#9058=ORIENTED_EDGE('',*,*,#6813,.T.);
#9059=ORIENTED_EDGE('',*,*,#6397,.T.);
#9060=ORIENTED_EDGE('',*,*,#6814,.F.);
#9061=ORIENTED_EDGE('',*,*,#6535,.T.);
#9062=ORIENTED_EDGE('',*,*,#6815,.T.);
#9063=ORIENTED_EDGE('',*,*,#6391,.T.);
#9064=ORIENTED_EDGE('',*,*,#6816,.F.);
#9065=ORIENTED_EDGE('',*,*,#6527,.T.);
#9066=ORIENTED_EDGE('',*,*,#6817,.T.);
#9067=ORIENTED_EDGE('',*,*,#6385,.T.);
#9068=ORIENTED_EDGE('',*,*,#6818,.F.);
#9069=ORIENTED_EDGE('',*,*,#6519,.T.);
#9070=ORIENTED_EDGE('',*,*,#6819,.T.);
#9071=ORIENTED_EDGE('',*,*,#6379,.T.);
#9072=ORIENTED_EDGE('',*,*,#6820,.F.);
#9073=ORIENTED_EDGE('',*,*,#6511,.T.);
#9074=ORIENTED_EDGE('',*,*,#6821,.T.);
#9075=ORIENTED_EDGE('',*,*,#6373,.T.);
#9076=ORIENTED_EDGE('',*,*,#6822,.F.);
#9077=ORIENTED_EDGE('',*,*,#6503,.T.);
#9078=ORIENTED_EDGE('',*,*,#6823,.T.);
#9079=ORIENTED_EDGE('',*,*,#6367,.T.);
#9080=ORIENTED_EDGE('',*,*,#6824,.F.);
#9081=ORIENTED_EDGE('',*,*,#6495,.T.);
#9082=ORIENTED_EDGE('',*,*,#6825,.T.);
#9083=ORIENTED_EDGE('',*,*,#6361,.T.);
#9084=ORIENTED_EDGE('',*,*,#6826,.F.);
#9085=ORIENTED_EDGE('',*,*,#6487,.T.);
#9086=ORIENTED_EDGE('',*,*,#6827,.T.);
#9087=ORIENTED_EDGE('',*,*,#6355,.T.);
#9088=ORIENTED_EDGE('',*,*,#6828,.F.);
#9089=ORIENTED_EDGE('',*,*,#6479,.T.);
#9090=ORIENTED_EDGE('',*,*,#6829,.T.);
#9091=ORIENTED_EDGE('',*,*,#6349,.T.);
#9092=ORIENTED_EDGE('',*,*,#6830,.F.);
#9093=ORIENTED_EDGE('',*,*,#6471,.T.);
#9094=ORIENTED_EDGE('',*,*,#6831,.T.);
#9095=ORIENTED_EDGE('',*,*,#6343,.T.);
#9096=ORIENTED_EDGE('',*,*,#6832,.F.);
#9097=ORIENTED_EDGE('',*,*,#6463,.T.);
#9098=ORIENTED_EDGE('',*,*,#6833,.T.);
#9099=ORIENTED_EDGE('',*,*,#6337,.T.);
#9100=ORIENTED_EDGE('',*,*,#6834,.F.);
#9101=ORIENTED_EDGE('',*,*,#6455,.T.);
#9102=ORIENTED_EDGE('',*,*,#6835,.T.);
#9103=ORIENTED_EDGE('',*,*,#6331,.T.);
#9104=ORIENTED_EDGE('',*,*,#6836,.F.);
#9105=ORIENTED_EDGE('',*,*,#6447,.T.);
#9106=ORIENTED_EDGE('',*,*,#6837,.T.);
#9107=ORIENTED_EDGE('',*,*,#6325,.T.);
#9108=ORIENTED_EDGE('',*,*,#6838,.F.);
#9109=ORIENTED_EDGE('',*,*,#6439,.T.);
#9110=ORIENTED_EDGE('',*,*,#6839,.T.);
#9111=ORIENTED_EDGE('',*,*,#6421,.T.);
#9112=ORIENTED_EDGE('',*,*,#6840,.F.);
#9113=ORIENTED_EDGE('',*,*,#6431,.T.);
#9114=ORIENTED_EDGE('',*,*,#6841,.T.);
#9115=ORIENTED_EDGE('',*,*,#6318,.T.);
#9116=ORIENTED_EDGE('',*,*,#6425,.T.);
#9117=ORIENTED_EDGE('',*,*,#6842,.F.);
#9118=ORIENTED_EDGE('',*,*,#6570,.T.);
#9119=ORIENTED_EDGE('',*,*,#6623,.T.);
#9120=ORIENTED_EDGE('',*,*,#6843,.T.);
#9121=ORIENTED_EDGE('',*,*,#6694,.T.);
#9122=ORIENTED_EDGE('',*,*,#6804,.T.);
#9123=ORIENTED_EDGE('',*,*,#6766,.T.);
#9124=ORIENTED_EDGE('',*,*,#6844,.T.);
#9125=ORIENTED_EDGE('',*,*,#6426,.T.);
#9126=ORIENTED_EDGE('',*,*,#6316,.T.);
#9127=ORIENTED_EDGE('',*,*,#6845,.F.);
#9128=ORIENTED_EDGE('',*,*,#6768,.T.);
#9129=ORIENTED_EDGE('',*,*,#6805,.T.);
#9130=ORIENTED_EDGE('',*,*,#6696,.T.);
#9131=ORIENTED_EDGE('',*,*,#6846,.F.);
#9132=ORIENTED_EDGE('',*,*,#6624,.T.);
#9133=ORIENTED_EDGE('',*,*,#6568,.T.);
#9134=ORIENTED_EDGE('',*,*,#6806,.T.);
#9135=ORIENTED_EDGE('',*,*,#6625,.T.);
#9136=ORIENTED_EDGE('',*,*,#6846,.T.);
#9137=ORIENTED_EDGE('',*,*,#6695,.T.);
#9138=ORIENTED_EDGE('',*,*,#6843,.F.);
#9139=ORIENTED_EDGE('',*,*,#6319,.T.);
#9140=ORIENTED_EDGE('',*,*,#6844,.F.);
#9141=ORIENTED_EDGE('',*,*,#6769,.T.);
#9142=ORIENTED_EDGE('',*,*,#6845,.T.);
#9143=ORIENTED_EDGE('',*,*,#6250,.T.);
#9144=ORIENTED_EDGE('',*,*,#6413,.T.);
#9145=ORIENTED_EDGE('',*,*,#6847,.F.);
#9146=ORIENTED_EDGE('',*,*,#6562,.T.);
#9147=ORIENTED_EDGE('',*,*,#6620,.T.);
#9148=ORIENTED_EDGE('',*,*,#6848,.T.);
#9149=ORIENTED_EDGE('',*,*,#6690,.T.);
#9150=ORIENTED_EDGE('',*,*,#6802,.T.);
#9151=ORIENTED_EDGE('',*,*,#6762,.T.);
#9152=ORIENTED_EDGE('',*,*,#6849,.T.);
#9153=ORIENTED_EDGE('',*,*,#6414,.T.);
#9154=ORIENTED_EDGE('',*,*,#6248,.T.);
#9155=ORIENTED_EDGE('',*,*,#6850,.F.);
#9156=ORIENTED_EDGE('',*,*,#6764,.T.);
#9157=ORIENTED_EDGE('',*,*,#6803,.T.);
#9158=ORIENTED_EDGE('',*,*,#6692,.T.);
#9159=ORIENTED_EDGE('',*,*,#6851,.F.);
#9160=ORIENTED_EDGE('',*,*,#6621,.T.);
#9161=ORIENTED_EDGE('',*,*,#6560,.T.);
#9162=ORIENTED_EDGE('',*,*,#6808,.T.);
#9163=ORIENTED_EDGE('',*,*,#6622,.T.);
#9164=ORIENTED_EDGE('',*,*,#6851,.T.);
#9165=ORIENTED_EDGE('',*,*,#6691,.T.);
#9166=ORIENTED_EDGE('',*,*,#6848,.F.);
#9167=ORIENTED_EDGE('',*,*,#6251,.T.);
#9168=ORIENTED_EDGE('',*,*,#6849,.F.);
#9169=ORIENTED_EDGE('',*,*,#6765,.T.);
#9170=ORIENTED_EDGE('',*,*,#6850,.T.);
#9171=ORIENTED_EDGE('',*,*,#6254,.T.);
#9172=ORIENTED_EDGE('',*,*,#6407,.T.);
#9173=ORIENTED_EDGE('',*,*,#6852,.F.);
#9174=ORIENTED_EDGE('',*,*,#6554,.T.);
#9175=ORIENTED_EDGE('',*,*,#6617,.T.);
#9176=ORIENTED_EDGE('',*,*,#6853,.T.);
#9177=ORIENTED_EDGE('',*,*,#6686,.T.);
#9178=ORIENTED_EDGE('',*,*,#6800,.T.);
#9179=ORIENTED_EDGE('',*,*,#6758,.T.);
#9180=ORIENTED_EDGE('',*,*,#6854,.T.);
#9181=ORIENTED_EDGE('',*,*,#6408,.T.);
#9182=ORIENTED_EDGE('',*,*,#6252,.T.);
#9183=ORIENTED_EDGE('',*,*,#6855,.F.);
#9184=ORIENTED_EDGE('',*,*,#6760,.T.);
#9185=ORIENTED_EDGE('',*,*,#6801,.T.);
#9186=ORIENTED_EDGE('',*,*,#6688,.T.);
#9187=ORIENTED_EDGE('',*,*,#6856,.F.);
#9188=ORIENTED_EDGE('',*,*,#6618,.T.);
#9189=ORIENTED_EDGE('',*,*,#6552,.T.);
#9190=ORIENTED_EDGE('',*,*,#6810,.T.);
#9191=ORIENTED_EDGE('',*,*,#6619,.T.);
#9192=ORIENTED_EDGE('',*,*,#6856,.T.);
#9193=ORIENTED_EDGE('',*,*,#6687,.T.);
#9194=ORIENTED_EDGE('',*,*,#6853,.F.);
#9195=ORIENTED_EDGE('',*,*,#6255,.T.);
#9196=ORIENTED_EDGE('',*,*,#6854,.F.);
#9197=ORIENTED_EDGE('',*,*,#6761,.T.);
#9198=ORIENTED_EDGE('',*,*,#6855,.T.);
#9199=ORIENTED_EDGE('',*,*,#6258,.T.);
#9200=ORIENTED_EDGE('',*,*,#6401,.T.);
#9201=ORIENTED_EDGE('',*,*,#6857,.F.);
#9202=ORIENTED_EDGE('',*,*,#6546,.T.);
#9203=ORIENTED_EDGE('',*,*,#6614,.T.);
#9204=ORIENTED_EDGE('',*,*,#6858,.T.);
#9205=ORIENTED_EDGE('',*,*,#6682,.T.);
#9206=ORIENTED_EDGE('',*,*,#6798,.T.);
#9207=ORIENTED_EDGE('',*,*,#6754,.T.);
#9208=ORIENTED_EDGE('',*,*,#6859,.T.);
#9209=ORIENTED_EDGE('',*,*,#6402,.T.);
#9210=ORIENTED_EDGE('',*,*,#6256,.T.);
#9211=ORIENTED_EDGE('',*,*,#6860,.F.);
#9212=ORIENTED_EDGE('',*,*,#6756,.T.);
#9213=ORIENTED_EDGE('',*,*,#6799,.T.);
#9214=ORIENTED_EDGE('',*,*,#6684,.T.);
#9215=ORIENTED_EDGE('',*,*,#6861,.F.);
#9216=ORIENTED_EDGE('',*,*,#6615,.T.);
#9217=ORIENTED_EDGE('',*,*,#6544,.T.);
#9218=ORIENTED_EDGE('',*,*,#6812,.T.);
#9219=ORIENTED_EDGE('',*,*,#6616,.T.);
#9220=ORIENTED_EDGE('',*,*,#6861,.T.);
#9221=ORIENTED_EDGE('',*,*,#6683,.T.);
#9222=ORIENTED_EDGE('',*,*,#6858,.F.);
#9223=ORIENTED_EDGE('',*,*,#6259,.T.);
#9224=ORIENTED_EDGE('',*,*,#6859,.F.);
#9225=ORIENTED_EDGE('',*,*,#6757,.T.);
#9226=ORIENTED_EDGE('',*,*,#6860,.T.);
#9227=ORIENTED_EDGE('',*,*,#6262,.T.);
#9228=ORIENTED_EDGE('',*,*,#6395,.T.);
#9229=ORIENTED_EDGE('',*,*,#6862,.F.);
#9230=ORIENTED_EDGE('',*,*,#6538,.T.);
#9231=ORIENTED_EDGE('',*,*,#6611,.T.);
#9232=ORIENTED_EDGE('',*,*,#6863,.T.);
#9233=ORIENTED_EDGE('',*,*,#6678,.T.);
#9234=ORIENTED_EDGE('',*,*,#6796,.T.);
#9235=ORIENTED_EDGE('',*,*,#6750,.T.);
#9236=ORIENTED_EDGE('',*,*,#6864,.T.);
#9237=ORIENTED_EDGE('',*,*,#6396,.T.);
#9238=ORIENTED_EDGE('',*,*,#6260,.T.);
#9239=ORIENTED_EDGE('',*,*,#6865,.F.);
#9240=ORIENTED_EDGE('',*,*,#6752,.T.);
#9241=ORIENTED_EDGE('',*,*,#6797,.T.);
#9242=ORIENTED_EDGE('',*,*,#6680,.T.);
#9243=ORIENTED_EDGE('',*,*,#6866,.F.);
#9244=ORIENTED_EDGE('',*,*,#6612,.T.);
#9245=ORIENTED_EDGE('',*,*,#6536,.T.);
#9246=ORIENTED_EDGE('',*,*,#6814,.T.);
#9247=ORIENTED_EDGE('',*,*,#6613,.T.);
#9248=ORIENTED_EDGE('',*,*,#6866,.T.);
#9249=ORIENTED_EDGE('',*,*,#6679,.T.);
#9250=ORIENTED_EDGE('',*,*,#6863,.F.);
#9251=ORIENTED_EDGE('',*,*,#6263,.T.);
#9252=ORIENTED_EDGE('',*,*,#6864,.F.);
#9253=ORIENTED_EDGE('',*,*,#6753,.T.);
#9254=ORIENTED_EDGE('',*,*,#6865,.T.);
#9255=ORIENTED_EDGE('',*,*,#6266,.T.);
#9256=ORIENTED_EDGE('',*,*,#6389,.T.);
#9257=ORIENTED_EDGE('',*,*,#6867,.F.);
#9258=ORIENTED_EDGE('',*,*,#6530,.T.);
#9259=ORIENTED_EDGE('',*,*,#6608,.T.);
#9260=ORIENTED_EDGE('',*,*,#6868,.T.);
#9261=ORIENTED_EDGE('',*,*,#6674,.T.);
#9262=ORIENTED_EDGE('',*,*,#6794,.T.);
#9263=ORIENTED_EDGE('',*,*,#6746,.T.);
#9264=ORIENTED_EDGE('',*,*,#6869,.T.);
#9265=ORIENTED_EDGE('',*,*,#6390,.T.);
#9266=ORIENTED_EDGE('',*,*,#6264,.T.);
#9267=ORIENTED_EDGE('',*,*,#6870,.F.);
#9268=ORIENTED_EDGE('',*,*,#6748,.T.);
#9269=ORIENTED_EDGE('',*,*,#6795,.T.);
#9270=ORIENTED_EDGE('',*,*,#6676,.T.);
#9271=ORIENTED_EDGE('',*,*,#6871,.F.);
#9272=ORIENTED_EDGE('',*,*,#6609,.T.);
#9273=ORIENTED_EDGE('',*,*,#6528,.T.);
#9274=ORIENTED_EDGE('',*,*,#6816,.T.);
#9275=ORIENTED_EDGE('',*,*,#6610,.T.);
#9276=ORIENTED_EDGE('',*,*,#6871,.T.);
#9277=ORIENTED_EDGE('',*,*,#6675,.T.);
#9278=ORIENTED_EDGE('',*,*,#6868,.F.);
#9279=ORIENTED_EDGE('',*,*,#6267,.T.);
#9280=ORIENTED_EDGE('',*,*,#6869,.F.);
#9281=ORIENTED_EDGE('',*,*,#6749,.T.);
#9282=ORIENTED_EDGE('',*,*,#6870,.T.);
#9283=ORIENTED_EDGE('',*,*,#6270,.T.);
#9284=ORIENTED_EDGE('',*,*,#6383,.T.);
#9285=ORIENTED_EDGE('',*,*,#6872,.F.);
#9286=ORIENTED_EDGE('',*,*,#6522,.T.);
#9287=ORIENTED_EDGE('',*,*,#6605,.T.);
#9288=ORIENTED_EDGE('',*,*,#6873,.T.);
#9289=ORIENTED_EDGE('',*,*,#6670,.T.);
#9290=ORIENTED_EDGE('',*,*,#6792,.T.);
#9291=ORIENTED_EDGE('',*,*,#6742,.T.);
#9292=ORIENTED_EDGE('',*,*,#6874,.T.);
#9293=ORIENTED_EDGE('',*,*,#6384,.T.);
#9294=ORIENTED_EDGE('',*,*,#6268,.T.);
#9295=ORIENTED_EDGE('',*,*,#6875,.F.);
#9296=ORIENTED_EDGE('',*,*,#6744,.T.);
#9297=ORIENTED_EDGE('',*,*,#6793,.T.);
#9298=ORIENTED_EDGE('',*,*,#6672,.T.);
#9299=ORIENTED_EDGE('',*,*,#6876,.F.);
#9300=ORIENTED_EDGE('',*,*,#6606,.T.);
#9301=ORIENTED_EDGE('',*,*,#6520,.T.);
#9302=ORIENTED_EDGE('',*,*,#6818,.T.);
#9303=ORIENTED_EDGE('',*,*,#6607,.T.);
#9304=ORIENTED_EDGE('',*,*,#6876,.T.);
#9305=ORIENTED_EDGE('',*,*,#6671,.T.);
#9306=ORIENTED_EDGE('',*,*,#6873,.F.);
#9307=ORIENTED_EDGE('',*,*,#6271,.T.);
#9308=ORIENTED_EDGE('',*,*,#6874,.F.);
#9309=ORIENTED_EDGE('',*,*,#6745,.T.);
#9310=ORIENTED_EDGE('',*,*,#6875,.T.);
#9311=ORIENTED_EDGE('',*,*,#6274,.T.);
#9312=ORIENTED_EDGE('',*,*,#6377,.T.);
#9313=ORIENTED_EDGE('',*,*,#6877,.F.);
#9314=ORIENTED_EDGE('',*,*,#6514,.T.);
#9315=ORIENTED_EDGE('',*,*,#6602,.T.);
#9316=ORIENTED_EDGE('',*,*,#6878,.T.);
#9317=ORIENTED_EDGE('',*,*,#6666,.T.);
#9318=ORIENTED_EDGE('',*,*,#6790,.T.);
#9319=ORIENTED_EDGE('',*,*,#6738,.T.);
#9320=ORIENTED_EDGE('',*,*,#6879,.T.);
#9321=ORIENTED_EDGE('',*,*,#6378,.T.);
#9322=ORIENTED_EDGE('',*,*,#6272,.T.);
#9323=ORIENTED_EDGE('',*,*,#6880,.F.);
#9324=ORIENTED_EDGE('',*,*,#6740,.T.);
#9325=ORIENTED_EDGE('',*,*,#6791,.T.);
#9326=ORIENTED_EDGE('',*,*,#6668,.T.);
#9327=ORIENTED_EDGE('',*,*,#6881,.F.);
#9328=ORIENTED_EDGE('',*,*,#6603,.T.);
#9329=ORIENTED_EDGE('',*,*,#6512,.T.);
#9330=ORIENTED_EDGE('',*,*,#6820,.T.);
#9331=ORIENTED_EDGE('',*,*,#6604,.T.);
#9332=ORIENTED_EDGE('',*,*,#6881,.T.);
#9333=ORIENTED_EDGE('',*,*,#6667,.T.);
#9334=ORIENTED_EDGE('',*,*,#6878,.F.);
#9335=ORIENTED_EDGE('',*,*,#6275,.T.);
#9336=ORIENTED_EDGE('',*,*,#6879,.F.);
#9337=ORIENTED_EDGE('',*,*,#6741,.T.);
#9338=ORIENTED_EDGE('',*,*,#6880,.T.);
#9339=ORIENTED_EDGE('',*,*,#6278,.T.);
#9340=ORIENTED_EDGE('',*,*,#6371,.T.);
#9341=ORIENTED_EDGE('',*,*,#6882,.F.);
#9342=ORIENTED_EDGE('',*,*,#6506,.T.);
#9343=ORIENTED_EDGE('',*,*,#6599,.T.);
#9344=ORIENTED_EDGE('',*,*,#6883,.T.);
#9345=ORIENTED_EDGE('',*,*,#6662,.T.);
#9346=ORIENTED_EDGE('',*,*,#6788,.T.);
#9347=ORIENTED_EDGE('',*,*,#6734,.T.);
#9348=ORIENTED_EDGE('',*,*,#6884,.T.);
#9349=ORIENTED_EDGE('',*,*,#6372,.T.);
#9350=ORIENTED_EDGE('',*,*,#6276,.T.);
#9351=ORIENTED_EDGE('',*,*,#6885,.F.);
#9352=ORIENTED_EDGE('',*,*,#6736,.T.);
#9353=ORIENTED_EDGE('',*,*,#6789,.T.);
#9354=ORIENTED_EDGE('',*,*,#6664,.T.);
#9355=ORIENTED_EDGE('',*,*,#6886,.F.);
#9356=ORIENTED_EDGE('',*,*,#6600,.T.);
#9357=ORIENTED_EDGE('',*,*,#6504,.T.);
#9358=ORIENTED_EDGE('',*,*,#6822,.T.);
#9359=ORIENTED_EDGE('',*,*,#6601,.T.);
#9360=ORIENTED_EDGE('',*,*,#6886,.T.);
#9361=ORIENTED_EDGE('',*,*,#6663,.T.);
#9362=ORIENTED_EDGE('',*,*,#6883,.F.);
#9363=ORIENTED_EDGE('',*,*,#6279,.T.);
#9364=ORIENTED_EDGE('',*,*,#6884,.F.);
#9365=ORIENTED_EDGE('',*,*,#6737,.T.);
#9366=ORIENTED_EDGE('',*,*,#6885,.T.);
#9367=ORIENTED_EDGE('',*,*,#6282,.T.);
#9368=ORIENTED_EDGE('',*,*,#6365,.T.);
#9369=ORIENTED_EDGE('',*,*,#6887,.F.);
#9370=ORIENTED_EDGE('',*,*,#6498,.T.);
#9371=ORIENTED_EDGE('',*,*,#6596,.T.);
#9372=ORIENTED_EDGE('',*,*,#6888,.T.);
#9373=ORIENTED_EDGE('',*,*,#6658,.T.);
#9374=ORIENTED_EDGE('',*,*,#6786,.T.);
#9375=ORIENTED_EDGE('',*,*,#6730,.T.);
#9376=ORIENTED_EDGE('',*,*,#6889,.T.);
#9377=ORIENTED_EDGE('',*,*,#6366,.T.);
#9378=ORIENTED_EDGE('',*,*,#6280,.T.);
#9379=ORIENTED_EDGE('',*,*,#6890,.F.);
#9380=ORIENTED_EDGE('',*,*,#6732,.T.);
#9381=ORIENTED_EDGE('',*,*,#6787,.T.);
#9382=ORIENTED_EDGE('',*,*,#6660,.T.);
#9383=ORIENTED_EDGE('',*,*,#6891,.F.);
#9384=ORIENTED_EDGE('',*,*,#6597,.T.);
#9385=ORIENTED_EDGE('',*,*,#6496,.T.);
#9386=ORIENTED_EDGE('',*,*,#6824,.T.);
#9387=ORIENTED_EDGE('',*,*,#6598,.T.);
#9388=ORIENTED_EDGE('',*,*,#6891,.T.);
#9389=ORIENTED_EDGE('',*,*,#6659,.T.);
#9390=ORIENTED_EDGE('',*,*,#6888,.F.);
#9391=ORIENTED_EDGE('',*,*,#6283,.T.);
#9392=ORIENTED_EDGE('',*,*,#6889,.F.);
#9393=ORIENTED_EDGE('',*,*,#6733,.T.);
#9394=ORIENTED_EDGE('',*,*,#6890,.T.);
#9395=ORIENTED_EDGE('',*,*,#6286,.T.);
#9396=ORIENTED_EDGE('',*,*,#6359,.T.);
#9397=ORIENTED_EDGE('',*,*,#6892,.F.);
#9398=ORIENTED_EDGE('',*,*,#6490,.T.);
#9399=ORIENTED_EDGE('',*,*,#6593,.T.);
#9400=ORIENTED_EDGE('',*,*,#6893,.T.);
#9401=ORIENTED_EDGE('',*,*,#6654,.T.);
#9402=ORIENTED_EDGE('',*,*,#6784,.T.);
#9403=ORIENTED_EDGE('',*,*,#6726,.T.);
#9404=ORIENTED_EDGE('',*,*,#6894,.T.);
#9405=ORIENTED_EDGE('',*,*,#6360,.T.);
#9406=ORIENTED_EDGE('',*,*,#6284,.T.);
#9407=ORIENTED_EDGE('',*,*,#6895,.F.);
#9408=ORIENTED_EDGE('',*,*,#6728,.T.);
#9409=ORIENTED_EDGE('',*,*,#6785,.T.);
#9410=ORIENTED_EDGE('',*,*,#6656,.T.);
#9411=ORIENTED_EDGE('',*,*,#6896,.F.);
#9412=ORIENTED_EDGE('',*,*,#6594,.T.);
#9413=ORIENTED_EDGE('',*,*,#6488,.T.);
#9414=ORIENTED_EDGE('',*,*,#6826,.T.);
#9415=ORIENTED_EDGE('',*,*,#6595,.T.);
#9416=ORIENTED_EDGE('',*,*,#6896,.T.);
#9417=ORIENTED_EDGE('',*,*,#6655,.T.);
#9418=ORIENTED_EDGE('',*,*,#6893,.F.);
#9419=ORIENTED_EDGE('',*,*,#6287,.T.);
#9420=ORIENTED_EDGE('',*,*,#6894,.F.);
#9421=ORIENTED_EDGE('',*,*,#6729,.T.);
#9422=ORIENTED_EDGE('',*,*,#6895,.T.);
#9423=ORIENTED_EDGE('',*,*,#6290,.T.);
#9424=ORIENTED_EDGE('',*,*,#6353,.T.);
#9425=ORIENTED_EDGE('',*,*,#6897,.F.);
#9426=ORIENTED_EDGE('',*,*,#6482,.T.);
#9427=ORIENTED_EDGE('',*,*,#6590,.T.);
#9428=ORIENTED_EDGE('',*,*,#6898,.T.);
#9429=ORIENTED_EDGE('',*,*,#6650,.T.);
#9430=ORIENTED_EDGE('',*,*,#6782,.T.);
#9431=ORIENTED_EDGE('',*,*,#6722,.T.);
#9432=ORIENTED_EDGE('',*,*,#6899,.T.);
#9433=ORIENTED_EDGE('',*,*,#6354,.T.);
#9434=ORIENTED_EDGE('',*,*,#6288,.T.);
#9435=ORIENTED_EDGE('',*,*,#6900,.F.);
#9436=ORIENTED_EDGE('',*,*,#6724,.T.);
#9437=ORIENTED_EDGE('',*,*,#6783,.T.);
#9438=ORIENTED_EDGE('',*,*,#6652,.T.);
#9439=ORIENTED_EDGE('',*,*,#6901,.F.);
#9440=ORIENTED_EDGE('',*,*,#6591,.T.);
#9441=ORIENTED_EDGE('',*,*,#6480,.T.);
#9442=ORIENTED_EDGE('',*,*,#6828,.T.);
#9443=ORIENTED_EDGE('',*,*,#6592,.T.);
#9444=ORIENTED_EDGE('',*,*,#6901,.T.);
#9445=ORIENTED_EDGE('',*,*,#6651,.T.);
#9446=ORIENTED_EDGE('',*,*,#6898,.F.);
#9447=ORIENTED_EDGE('',*,*,#6291,.T.);
#9448=ORIENTED_EDGE('',*,*,#6899,.F.);
#9449=ORIENTED_EDGE('',*,*,#6725,.T.);
#9450=ORIENTED_EDGE('',*,*,#6900,.T.);
#9451=ORIENTED_EDGE('',*,*,#6294,.T.);
#9452=ORIENTED_EDGE('',*,*,#6347,.T.);
#9453=ORIENTED_EDGE('',*,*,#6902,.F.);
#9454=ORIENTED_EDGE('',*,*,#6474,.T.);
#9455=ORIENTED_EDGE('',*,*,#6587,.T.);
#9456=ORIENTED_EDGE('',*,*,#6903,.T.);
#9457=ORIENTED_EDGE('',*,*,#6646,.T.);
#9458=ORIENTED_EDGE('',*,*,#6780,.T.);
#9459=ORIENTED_EDGE('',*,*,#6718,.T.);
#9460=ORIENTED_EDGE('',*,*,#6904,.T.);
#9461=ORIENTED_EDGE('',*,*,#6348,.T.);
#9462=ORIENTED_EDGE('',*,*,#6292,.T.);
#9463=ORIENTED_EDGE('',*,*,#6905,.F.);
#9464=ORIENTED_EDGE('',*,*,#6720,.T.);
#9465=ORIENTED_EDGE('',*,*,#6781,.T.);
#9466=ORIENTED_EDGE('',*,*,#6648,.T.);
#9467=ORIENTED_EDGE('',*,*,#6906,.F.);
#9468=ORIENTED_EDGE('',*,*,#6588,.T.);
#9469=ORIENTED_EDGE('',*,*,#6472,.T.);
#9470=ORIENTED_EDGE('',*,*,#6830,.T.);
#9471=ORIENTED_EDGE('',*,*,#6589,.T.);
#9472=ORIENTED_EDGE('',*,*,#6906,.T.);
#9473=ORIENTED_EDGE('',*,*,#6647,.T.);
#9474=ORIENTED_EDGE('',*,*,#6903,.F.);
#9475=ORIENTED_EDGE('',*,*,#6295,.T.);
#9476=ORIENTED_EDGE('',*,*,#6904,.F.);
#9477=ORIENTED_EDGE('',*,*,#6721,.T.);
#9478=ORIENTED_EDGE('',*,*,#6905,.T.);
#9479=ORIENTED_EDGE('',*,*,#6298,.T.);
#9480=ORIENTED_EDGE('',*,*,#6341,.T.);
#9481=ORIENTED_EDGE('',*,*,#6907,.F.);
#9482=ORIENTED_EDGE('',*,*,#6466,.T.);
#9483=ORIENTED_EDGE('',*,*,#6584,.T.);
#9484=ORIENTED_EDGE('',*,*,#6908,.T.);
#9485=ORIENTED_EDGE('',*,*,#6642,.T.);
#9486=ORIENTED_EDGE('',*,*,#6778,.T.);
#9487=ORIENTED_EDGE('',*,*,#6714,.T.);
#9488=ORIENTED_EDGE('',*,*,#6909,.T.);
#9489=ORIENTED_EDGE('',*,*,#6342,.T.);
#9490=ORIENTED_EDGE('',*,*,#6296,.T.);
#9491=ORIENTED_EDGE('',*,*,#6910,.F.);
#9492=ORIENTED_EDGE('',*,*,#6716,.T.);
#9493=ORIENTED_EDGE('',*,*,#6779,.T.);
#9494=ORIENTED_EDGE('',*,*,#6644,.T.);
#9495=ORIENTED_EDGE('',*,*,#6911,.F.);
#9496=ORIENTED_EDGE('',*,*,#6585,.T.);
#9497=ORIENTED_EDGE('',*,*,#6464,.T.);
#9498=ORIENTED_EDGE('',*,*,#6832,.T.);
#9499=ORIENTED_EDGE('',*,*,#6586,.T.);
#9500=ORIENTED_EDGE('',*,*,#6911,.T.);
#9501=ORIENTED_EDGE('',*,*,#6643,.T.);
#9502=ORIENTED_EDGE('',*,*,#6908,.F.);
#9503=ORIENTED_EDGE('',*,*,#6299,.T.);
#9504=ORIENTED_EDGE('',*,*,#6909,.F.);
#9505=ORIENTED_EDGE('',*,*,#6717,.T.);
#9506=ORIENTED_EDGE('',*,*,#6910,.T.);
#9507=ORIENTED_EDGE('',*,*,#6302,.T.);
#9508=ORIENTED_EDGE('',*,*,#6335,.T.);
#9509=ORIENTED_EDGE('',*,*,#6912,.F.);
#9510=ORIENTED_EDGE('',*,*,#6458,.T.);
#9511=ORIENTED_EDGE('',*,*,#6581,.T.);
#9512=ORIENTED_EDGE('',*,*,#6913,.T.);
#9513=ORIENTED_EDGE('',*,*,#6638,.T.);
#9514=ORIENTED_EDGE('',*,*,#6776,.T.);
#9515=ORIENTED_EDGE('',*,*,#6710,.T.);
#9516=ORIENTED_EDGE('',*,*,#6914,.T.);
#9517=ORIENTED_EDGE('',*,*,#6336,.T.);
#9518=ORIENTED_EDGE('',*,*,#6300,.T.);
#9519=ORIENTED_EDGE('',*,*,#6915,.F.);
#9520=ORIENTED_EDGE('',*,*,#6712,.T.);
#9521=ORIENTED_EDGE('',*,*,#6777,.T.);
#9522=ORIENTED_EDGE('',*,*,#6640,.T.);
#9523=ORIENTED_EDGE('',*,*,#6916,.F.);
#9524=ORIENTED_EDGE('',*,*,#6582,.T.);
#9525=ORIENTED_EDGE('',*,*,#6456,.T.);
#9526=ORIENTED_EDGE('',*,*,#6834,.T.);
#9527=ORIENTED_EDGE('',*,*,#6583,.T.);
#9528=ORIENTED_EDGE('',*,*,#6916,.T.);
#9529=ORIENTED_EDGE('',*,*,#6639,.T.);
#9530=ORIENTED_EDGE('',*,*,#6913,.F.);
#9531=ORIENTED_EDGE('',*,*,#6303,.T.);
#9532=ORIENTED_EDGE('',*,*,#6914,.F.);
#9533=ORIENTED_EDGE('',*,*,#6713,.T.);
#9534=ORIENTED_EDGE('',*,*,#6915,.T.);
#9535=ORIENTED_EDGE('',*,*,#6306,.T.);
#9536=ORIENTED_EDGE('',*,*,#6329,.T.);
#9537=ORIENTED_EDGE('',*,*,#6917,.F.);
#9538=ORIENTED_EDGE('',*,*,#6450,.T.);
#9539=ORIENTED_EDGE('',*,*,#6578,.T.);
#9540=ORIENTED_EDGE('',*,*,#6918,.T.);
#9541=ORIENTED_EDGE('',*,*,#6634,.T.);
#9542=ORIENTED_EDGE('',*,*,#6774,.T.);
#9543=ORIENTED_EDGE('',*,*,#6706,.T.);
#9544=ORIENTED_EDGE('',*,*,#6919,.T.);
#9545=ORIENTED_EDGE('',*,*,#6330,.T.);
#9546=ORIENTED_EDGE('',*,*,#6304,.T.);
#9547=ORIENTED_EDGE('',*,*,#6920,.F.);
#9548=ORIENTED_EDGE('',*,*,#6708,.T.);
#9549=ORIENTED_EDGE('',*,*,#6775,.T.);
#9550=ORIENTED_EDGE('',*,*,#6636,.T.);
#9551=ORIENTED_EDGE('',*,*,#6921,.F.);
#9552=ORIENTED_EDGE('',*,*,#6579,.T.);
#9553=ORIENTED_EDGE('',*,*,#6448,.T.);
#9554=ORIENTED_EDGE('',*,*,#6836,.T.);
#9555=ORIENTED_EDGE('',*,*,#6580,.T.);
#9556=ORIENTED_EDGE('',*,*,#6921,.T.);
#9557=ORIENTED_EDGE('',*,*,#6635,.T.);
#9558=ORIENTED_EDGE('',*,*,#6918,.F.);
#9559=ORIENTED_EDGE('',*,*,#6307,.T.);
#9560=ORIENTED_EDGE('',*,*,#6919,.F.);
#9561=ORIENTED_EDGE('',*,*,#6709,.T.);
#9562=ORIENTED_EDGE('',*,*,#6920,.T.);
#9563=ORIENTED_EDGE('',*,*,#6310,.T.);
#9564=ORIENTED_EDGE('',*,*,#6323,.T.);
#9565=ORIENTED_EDGE('',*,*,#6922,.F.);
#9566=ORIENTED_EDGE('',*,*,#6442,.T.);
#9567=ORIENTED_EDGE('',*,*,#6575,.T.);
#9568=ORIENTED_EDGE('',*,*,#6923,.T.);
#9569=ORIENTED_EDGE('',*,*,#6630,.T.);
#9570=ORIENTED_EDGE('',*,*,#6772,.T.);
#9571=ORIENTED_EDGE('',*,*,#6702,.T.);
#9572=ORIENTED_EDGE('',*,*,#6924,.T.);
#9573=ORIENTED_EDGE('',*,*,#6324,.T.);
#9574=ORIENTED_EDGE('',*,*,#6308,.T.);
#9575=ORIENTED_EDGE('',*,*,#6925,.F.);
#9576=ORIENTED_EDGE('',*,*,#6704,.T.);
#9577=ORIENTED_EDGE('',*,*,#6773,.T.);
#9578=ORIENTED_EDGE('',*,*,#6632,.T.);
#9579=ORIENTED_EDGE('',*,*,#6926,.F.);
#9580=ORIENTED_EDGE('',*,*,#6576,.T.);
#9581=ORIENTED_EDGE('',*,*,#6440,.T.);
#9582=ORIENTED_EDGE('',*,*,#6838,.T.);
#9583=ORIENTED_EDGE('',*,*,#6577,.T.);
#9584=ORIENTED_EDGE('',*,*,#6926,.T.);
#9585=ORIENTED_EDGE('',*,*,#6631,.T.);
#9586=ORIENTED_EDGE('',*,*,#6923,.F.);
#9587=ORIENTED_EDGE('',*,*,#6311,.T.);
#9588=ORIENTED_EDGE('',*,*,#6924,.F.);
#9589=ORIENTED_EDGE('',*,*,#6705,.T.);
#9590=ORIENTED_EDGE('',*,*,#6925,.T.);
#9591=ORIENTED_EDGE('',*,*,#6314,.T.);
#9592=ORIENTED_EDGE('',*,*,#6419,.T.);
#9593=ORIENTED_EDGE('',*,*,#6927,.F.);
#9594=ORIENTED_EDGE('',*,*,#6434,.T.);
#9595=ORIENTED_EDGE('',*,*,#6572,.T.);
#9596=ORIENTED_EDGE('',*,*,#6928,.T.);
#9597=ORIENTED_EDGE('',*,*,#6626,.T.);
#9598=ORIENTED_EDGE('',*,*,#6770,.T.);
#9599=ORIENTED_EDGE('',*,*,#6698,.T.);
#9600=ORIENTED_EDGE('',*,*,#6929,.T.);
#9601=ORIENTED_EDGE('',*,*,#6420,.T.);
#9602=ORIENTED_EDGE('',*,*,#6312,.T.);
#9603=ORIENTED_EDGE('',*,*,#6930,.F.);
#9604=ORIENTED_EDGE('',*,*,#6700,.T.);
#9605=ORIENTED_EDGE('',*,*,#6771,.T.);
#9606=ORIENTED_EDGE('',*,*,#6628,.T.);
#9607=ORIENTED_EDGE('',*,*,#6931,.F.);
#9608=ORIENTED_EDGE('',*,*,#6573,.T.);
#9609=ORIENTED_EDGE('',*,*,#6432,.T.);
#9610=ORIENTED_EDGE('',*,*,#6840,.T.);
#9611=ORIENTED_EDGE('',*,*,#6574,.T.);
#9612=ORIENTED_EDGE('',*,*,#6931,.T.);
#9613=ORIENTED_EDGE('',*,*,#6627,.T.);
#9614=ORIENTED_EDGE('',*,*,#6928,.F.);
#9615=ORIENTED_EDGE('',*,*,#6315,.T.);
#9616=ORIENTED_EDGE('',*,*,#6929,.F.);
#9617=ORIENTED_EDGE('',*,*,#6701,.T.);
#9618=ORIENTED_EDGE('',*,*,#6930,.T.);
#9619=ORIENTED_EDGE('',*,*,#6422,.T.);
#9620=ORIENTED_EDGE('',*,*,#6807,.F.);
#9621=ORIENTED_EDGE('',*,*,#6566,.T.);
#9622=ORIENTED_EDGE('',*,*,#6932,.F.);
#9623=ORIENTED_EDGE('',*,*,#6933,.F.);
#9624=ORIENTED_EDGE('',*,*,#6177,.F.);
#9625=ORIENTED_EDGE('',*,*,#6424,.T.);
#9626=ORIENTED_EDGE('',*,*,#6934,.F.);
#9627=ORIENTED_EDGE('',*,*,#6571,.T.);
#9628=ORIENTED_EDGE('',*,*,#6842,.T.);
#9629=ORIENTED_EDGE('',*,*,#6423,.T.);
#9630=ORIENTED_EDGE('',*,*,#6247,.F.);
#9631=ORIENTED_EDGE('',*,*,#6935,.F.);
#9632=ORIENTED_EDGE('',*,*,#6936,.T.);
#9633=ORIENTED_EDGE('',*,*,#6564,.T.);
#9634=ORIENTED_EDGE('',*,*,#6934,.T.);
#9635=ORIENTED_EDGE('',*,*,#6933,.T.);
#9636=ORIENTED_EDGE('',*,*,#6937,.T.);
#9637=ORIENTED_EDGE('',*,*,#6938,.T.);
#9638=ORIENTED_EDGE('',*,*,#6178,.F.);
#9639=ORIENTED_EDGE('',*,*,#6935,.T.);
#9640=ORIENTED_EDGE('',*,*,#6246,.F.);
#9641=ORIENTED_EDGE('',*,*,#6939,.T.);
#9642=ORIENTED_EDGE('',*,*,#6940,.T.);
#9643=ORIENTED_EDGE('',*,*,#6411,.T.);
#9644=ORIENTED_EDGE('',*,*,#6243,.F.);
#9645=ORIENTED_EDGE('',*,*,#6941,.F.);
#9646=ORIENTED_EDGE('',*,*,#6942,.T.);
#9647=ORIENTED_EDGE('',*,*,#6556,.T.);
#9648=ORIENTED_EDGE('',*,*,#6943,.T.);
#9649=ORIENTED_EDGE('',*,*,#6410,.T.);
#9650=ORIENTED_EDGE('',*,*,#6809,.F.);
#9651=ORIENTED_EDGE('',*,*,#6558,.T.);
#9652=ORIENTED_EDGE('',*,*,#6944,.F.);
#9653=ORIENTED_EDGE('',*,*,#6939,.F.);
#9654=ORIENTED_EDGE('',*,*,#6245,.F.);
#9655=ORIENTED_EDGE('',*,*,#6412,.T.);
#9656=ORIENTED_EDGE('',*,*,#6943,.F.);
#9657=ORIENTED_EDGE('',*,*,#6563,.T.);
#9658=ORIENTED_EDGE('',*,*,#6847,.T.);
#9659=ORIENTED_EDGE('',*,*,#6404,.T.);
#9660=ORIENTED_EDGE('',*,*,#6811,.F.);
#9661=ORIENTED_EDGE('',*,*,#6550,.T.);
#9662=ORIENTED_EDGE('',*,*,#6945,.F.);
#9663=ORIENTED_EDGE('',*,*,#6946,.F.);
#9664=ORIENTED_EDGE('',*,*,#6241,.F.);
#9665=ORIENTED_EDGE('',*,*,#6405,.T.);
#9666=ORIENTED_EDGE('',*,*,#6239,.F.);
#9667=ORIENTED_EDGE('',*,*,#6947,.F.);
#9668=ORIENTED_EDGE('',*,*,#6948,.T.);
#9669=ORIENTED_EDGE('',*,*,#6548,.T.);
#9670=ORIENTED_EDGE('',*,*,#6949,.T.);
#9671=ORIENTED_EDGE('',*,*,#6406,.T.);
#9672=ORIENTED_EDGE('',*,*,#6949,.F.);
#9673=ORIENTED_EDGE('',*,*,#6555,.T.);
#9674=ORIENTED_EDGE('',*,*,#6852,.T.);
#9675=ORIENTED_EDGE('',*,*,#6565,.T.);
#9676=ORIENTED_EDGE('',*,*,#6936,.F.);
#9677=ORIENTED_EDGE('',*,*,#6940,.F.);
#9678=ORIENTED_EDGE('',*,*,#6944,.T.);
#9679=ORIENTED_EDGE('',*,*,#6557,.T.);
#9680=ORIENTED_EDGE('',*,*,#6942,.F.);
#9681=ORIENTED_EDGE('',*,*,#6950,.F.);
#9682=ORIENTED_EDGE('',*,*,#6945,.T.);
#9683=ORIENTED_EDGE('',*,*,#6549,.T.);
#9684=ORIENTED_EDGE('',*,*,#6948,.F.);
#9685=ORIENTED_EDGE('',*,*,#6951,.F.);
#9686=ORIENTED_EDGE('',*,*,#6952,.T.);
#9687=ORIENTED_EDGE('',*,*,#6541,.T.);
#9688=ORIENTED_EDGE('',*,*,#6953,.F.);
#9689=ORIENTED_EDGE('',*,*,#6954,.F.);
#9690=ORIENTED_EDGE('',*,*,#6955,.T.);
#9691=ORIENTED_EDGE('',*,*,#6533,.T.);
#9692=ORIENTED_EDGE('',*,*,#6956,.F.);
#9693=ORIENTED_EDGE('',*,*,#6957,.F.);
#9694=ORIENTED_EDGE('',*,*,#6958,.T.);
#9695=ORIENTED_EDGE('',*,*,#6525,.T.);
#9696=ORIENTED_EDGE('',*,*,#6959,.F.);
#9697=ORIENTED_EDGE('',*,*,#6960,.F.);
#9698=ORIENTED_EDGE('',*,*,#6961,.T.);
#9699=ORIENTED_EDGE('',*,*,#6517,.T.);
#9700=ORIENTED_EDGE('',*,*,#6962,.F.);
#9701=ORIENTED_EDGE('',*,*,#6963,.F.);
#9702=ORIENTED_EDGE('',*,*,#6964,.T.);
#9703=ORIENTED_EDGE('',*,*,#6509,.T.);
#9704=ORIENTED_EDGE('',*,*,#6965,.F.);
#9705=ORIENTED_EDGE('',*,*,#6966,.F.);
#9706=ORIENTED_EDGE('',*,*,#6967,.T.);
#9707=ORIENTED_EDGE('',*,*,#6501,.T.);
#9708=ORIENTED_EDGE('',*,*,#6968,.F.);
#9709=ORIENTED_EDGE('',*,*,#6969,.F.);
#9710=ORIENTED_EDGE('',*,*,#6970,.T.);
#9711=ORIENTED_EDGE('',*,*,#6493,.T.);
#9712=ORIENTED_EDGE('',*,*,#6971,.F.);
#9713=ORIENTED_EDGE('',*,*,#6972,.F.);
#9714=ORIENTED_EDGE('',*,*,#6973,.T.);
#9715=ORIENTED_EDGE('',*,*,#6485,.T.);
#9716=ORIENTED_EDGE('',*,*,#6974,.F.);
#9717=ORIENTED_EDGE('',*,*,#6975,.F.);
#9718=ORIENTED_EDGE('',*,*,#6976,.T.);
#9719=ORIENTED_EDGE('',*,*,#6477,.T.);
#9720=ORIENTED_EDGE('',*,*,#6977,.F.);
#9721=ORIENTED_EDGE('',*,*,#6978,.F.);
#9722=ORIENTED_EDGE('',*,*,#6979,.T.);
#9723=ORIENTED_EDGE('',*,*,#6469,.T.);
#9724=ORIENTED_EDGE('',*,*,#6980,.F.);
#9725=ORIENTED_EDGE('',*,*,#6981,.F.);
#9726=ORIENTED_EDGE('',*,*,#6982,.T.);
#9727=ORIENTED_EDGE('',*,*,#6461,.T.);
#9728=ORIENTED_EDGE('',*,*,#6983,.F.);
#9729=ORIENTED_EDGE('',*,*,#6984,.F.);
#9730=ORIENTED_EDGE('',*,*,#6985,.T.);
#9731=ORIENTED_EDGE('',*,*,#6453,.T.);
#9732=ORIENTED_EDGE('',*,*,#6986,.F.);
#9733=ORIENTED_EDGE('',*,*,#6987,.F.);
#9734=ORIENTED_EDGE('',*,*,#6988,.T.);
#9735=ORIENTED_EDGE('',*,*,#6445,.T.);
#9736=ORIENTED_EDGE('',*,*,#6989,.F.);
#9737=ORIENTED_EDGE('',*,*,#6990,.F.);
#9738=ORIENTED_EDGE('',*,*,#6991,.T.);
#9739=ORIENTED_EDGE('',*,*,#6437,.T.);
#9740=ORIENTED_EDGE('',*,*,#6992,.F.);
#9741=ORIENTED_EDGE('',*,*,#6993,.F.);
#9742=ORIENTED_EDGE('',*,*,#6994,.T.);
#9743=ORIENTED_EDGE('',*,*,#6429,.T.);
#9744=ORIENTED_EDGE('',*,*,#6995,.F.);
#9745=ORIENTED_EDGE('',*,*,#6937,.F.);
#9746=ORIENTED_EDGE('',*,*,#6932,.T.);
#9747=ORIENTED_EDGE('',*,*,#6175,.T.);
#9748=ORIENTED_EDGE('',*,*,#6174,.T.);
#9749=ORIENTED_EDGE('',*,*,#6161,.T.);
#9750=ORIENTED_EDGE('',*,*,#6172,.T.);
#9751=ORIENTED_EDGE('',*,*,#6105,.T.);
#9752=ORIENTED_EDGE('',*,*,#6947,.T.);
#9753=ORIENTED_EDGE('',*,*,#6238,.F.);
#9754=ORIENTED_EDGE('',*,*,#6996,.T.);
#9755=ORIENTED_EDGE('',*,*,#6951,.T.);
#9756=ORIENTED_EDGE('',*,*,#6398,.T.);
#9757=ORIENTED_EDGE('',*,*,#6813,.F.);
#9758=ORIENTED_EDGE('',*,*,#6542,.T.);
#9759=ORIENTED_EDGE('',*,*,#6952,.F.);
#9760=ORIENTED_EDGE('',*,*,#6996,.F.);
#9761=ORIENTED_EDGE('',*,*,#6237,.F.);
#9762=ORIENTED_EDGE('',*,*,#6400,.T.);
#9763=ORIENTED_EDGE('',*,*,#6997,.F.);
#9764=ORIENTED_EDGE('',*,*,#6547,.T.);
#9765=ORIENTED_EDGE('',*,*,#6857,.T.);
#9766=ORIENTED_EDGE('',*,*,#6399,.T.);
#9767=ORIENTED_EDGE('',*,*,#6235,.F.);
#9768=ORIENTED_EDGE('',*,*,#6998,.F.);
#9769=ORIENTED_EDGE('',*,*,#6953,.T.);
#9770=ORIENTED_EDGE('',*,*,#6540,.T.);
#9771=ORIENTED_EDGE('',*,*,#6997,.T.);
#9772=ORIENTED_EDGE('',*,*,#6941,.T.);
#9773=ORIENTED_EDGE('',*,*,#6242,.F.);
#9774=ORIENTED_EDGE('',*,*,#6946,.T.);
#9775=ORIENTED_EDGE('',*,*,#6950,.T.);
#9776=ORIENTED_EDGE('',*,*,#6998,.T.);
#9777=ORIENTED_EDGE('',*,*,#6234,.F.);
#9778=ORIENTED_EDGE('',*,*,#6999,.T.);
#9779=ORIENTED_EDGE('',*,*,#6954,.T.);
#9780=ORIENTED_EDGE('',*,*,#6393,.T.);
#9781=ORIENTED_EDGE('',*,*,#6231,.F.);
#9782=ORIENTED_EDGE('',*,*,#7000,.F.);
#9783=ORIENTED_EDGE('',*,*,#6956,.T.);
#9784=ORIENTED_EDGE('',*,*,#6532,.T.);
#9785=ORIENTED_EDGE('',*,*,#7001,.T.);
#9786=ORIENTED_EDGE('',*,*,#6392,.T.);
#9787=ORIENTED_EDGE('',*,*,#6815,.F.);
#9788=ORIENTED_EDGE('',*,*,#6534,.T.);
#9789=ORIENTED_EDGE('',*,*,#6955,.F.);
#9790=ORIENTED_EDGE('',*,*,#6999,.F.);
#9791=ORIENTED_EDGE('',*,*,#6233,.F.);
#9792=ORIENTED_EDGE('',*,*,#6394,.T.);
#9793=ORIENTED_EDGE('',*,*,#7001,.F.);
#9794=ORIENTED_EDGE('',*,*,#6539,.T.);
#9795=ORIENTED_EDGE('',*,*,#6862,.T.);
#9796=ORIENTED_EDGE('',*,*,#6386,.T.);
#9797=ORIENTED_EDGE('',*,*,#6817,.F.);
#9798=ORIENTED_EDGE('',*,*,#6526,.T.);
#9799=ORIENTED_EDGE('',*,*,#6958,.F.);
#9800=ORIENTED_EDGE('',*,*,#7002,.F.);
#9801=ORIENTED_EDGE('',*,*,#6229,.F.);
#9802=ORIENTED_EDGE('',*,*,#6387,.T.);
#9803=ORIENTED_EDGE('',*,*,#6227,.F.);
#9804=ORIENTED_EDGE('',*,*,#7003,.F.);
#9805=ORIENTED_EDGE('',*,*,#6959,.T.);
#9806=ORIENTED_EDGE('',*,*,#6524,.T.);
#9807=ORIENTED_EDGE('',*,*,#7004,.T.);
#9808=ORIENTED_EDGE('',*,*,#6388,.T.);
#9809=ORIENTED_EDGE('',*,*,#7004,.F.);
#9810=ORIENTED_EDGE('',*,*,#6531,.T.);
#9811=ORIENTED_EDGE('',*,*,#6867,.T.);
#9812=ORIENTED_EDGE('',*,*,#7003,.T.);
#9813=ORIENTED_EDGE('',*,*,#6226,.F.);
#9814=ORIENTED_EDGE('',*,*,#7005,.T.);
#9815=ORIENTED_EDGE('',*,*,#6960,.T.);
#9816=ORIENTED_EDGE('',*,*,#6380,.T.);
#9817=ORIENTED_EDGE('',*,*,#6819,.F.);
#9818=ORIENTED_EDGE('',*,*,#6518,.T.);
#9819=ORIENTED_EDGE('',*,*,#6961,.F.);
#9820=ORIENTED_EDGE('',*,*,#7005,.F.);
#9821=ORIENTED_EDGE('',*,*,#6225,.F.);
#9822=ORIENTED_EDGE('',*,*,#6382,.T.);
#9823=ORIENTED_EDGE('',*,*,#7006,.F.);
#9824=ORIENTED_EDGE('',*,*,#6523,.T.);
#9825=ORIENTED_EDGE('',*,*,#6872,.T.);
#9826=ORIENTED_EDGE('',*,*,#6381,.T.);
#9827=ORIENTED_EDGE('',*,*,#6223,.F.);
#9828=ORIENTED_EDGE('',*,*,#7007,.F.);
#9829=ORIENTED_EDGE('',*,*,#6962,.T.);
#9830=ORIENTED_EDGE('',*,*,#6516,.T.);
#9831=ORIENTED_EDGE('',*,*,#7006,.T.);
#9832=ORIENTED_EDGE('',*,*,#7000,.T.);
#9833=ORIENTED_EDGE('',*,*,#6230,.F.);
#9834=ORIENTED_EDGE('',*,*,#7002,.T.);
#9835=ORIENTED_EDGE('',*,*,#6957,.T.);
#9836=ORIENTED_EDGE('',*,*,#7007,.T.);
#9837=ORIENTED_EDGE('',*,*,#6222,.F.);
#9838=ORIENTED_EDGE('',*,*,#7008,.T.);
#9839=ORIENTED_EDGE('',*,*,#6963,.T.);
#9840=ORIENTED_EDGE('',*,*,#6375,.T.);
#9841=ORIENTED_EDGE('',*,*,#6219,.F.);
#9842=ORIENTED_EDGE('',*,*,#7009,.F.);
#9843=ORIENTED_EDGE('',*,*,#6965,.T.);
#9844=ORIENTED_EDGE('',*,*,#6508,.T.);
#9845=ORIENTED_EDGE('',*,*,#7010,.T.);
#9846=ORIENTED_EDGE('',*,*,#6374,.T.);
#9847=ORIENTED_EDGE('',*,*,#6821,.F.);
#9848=ORIENTED_EDGE('',*,*,#6510,.T.);
#9849=ORIENTED_EDGE('',*,*,#6964,.F.);
#9850=ORIENTED_EDGE('',*,*,#7008,.F.);
#9851=ORIENTED_EDGE('',*,*,#6221,.F.);
#9852=ORIENTED_EDGE('',*,*,#6376,.T.);
#9853=ORIENTED_EDGE('',*,*,#7010,.F.);
#9854=ORIENTED_EDGE('',*,*,#6515,.T.);
#9855=ORIENTED_EDGE('',*,*,#6877,.T.);
#9856=ORIENTED_EDGE('',*,*,#6368,.T.);
#9857=ORIENTED_EDGE('',*,*,#6823,.F.);
#9858=ORIENTED_EDGE('',*,*,#6502,.T.);
#9859=ORIENTED_EDGE('',*,*,#6967,.F.);
#9860=ORIENTED_EDGE('',*,*,#7011,.F.);
#9861=ORIENTED_EDGE('',*,*,#6217,.F.);
#9862=ORIENTED_EDGE('',*,*,#6369,.T.);
#9863=ORIENTED_EDGE('',*,*,#6215,.F.);
#9864=ORIENTED_EDGE('',*,*,#7012,.F.);
#9865=ORIENTED_EDGE('',*,*,#6968,.T.);
#9866=ORIENTED_EDGE('',*,*,#6500,.T.);
#9867=ORIENTED_EDGE('',*,*,#7013,.T.);
#9868=ORIENTED_EDGE('',*,*,#6370,.T.);
#9869=ORIENTED_EDGE('',*,*,#7013,.F.);
#9870=ORIENTED_EDGE('',*,*,#6507,.T.);
#9871=ORIENTED_EDGE('',*,*,#6882,.T.);
#9872=ORIENTED_EDGE('',*,*,#7012,.T.);
#9873=ORIENTED_EDGE('',*,*,#6214,.F.);
#9874=ORIENTED_EDGE('',*,*,#7014,.T.);
#9875=ORIENTED_EDGE('',*,*,#6969,.T.);
#9876=ORIENTED_EDGE('',*,*,#6362,.T.);
#9877=ORIENTED_EDGE('',*,*,#6825,.F.);
#9878=ORIENTED_EDGE('',*,*,#6494,.T.);
#9879=ORIENTED_EDGE('',*,*,#6970,.F.);
#9880=ORIENTED_EDGE('',*,*,#7014,.F.);
#9881=ORIENTED_EDGE('',*,*,#6213,.F.);
#9882=ORIENTED_EDGE('',*,*,#6364,.T.);
#9883=ORIENTED_EDGE('',*,*,#7015,.F.);
#9884=ORIENTED_EDGE('',*,*,#6499,.T.);
#9885=ORIENTED_EDGE('',*,*,#6887,.T.);
#9886=ORIENTED_EDGE('',*,*,#6363,.T.);
#9887=ORIENTED_EDGE('',*,*,#6211,.F.);
#9888=ORIENTED_EDGE('',*,*,#7016,.F.);
#9889=ORIENTED_EDGE('',*,*,#6971,.T.);
#9890=ORIENTED_EDGE('',*,*,#6492,.T.);
#9891=ORIENTED_EDGE('',*,*,#7015,.T.);
#9892=ORIENTED_EDGE('',*,*,#7009,.T.);
#9893=ORIENTED_EDGE('',*,*,#6218,.F.);
#9894=ORIENTED_EDGE('',*,*,#7011,.T.);
#9895=ORIENTED_EDGE('',*,*,#6966,.T.);
#9896=ORIENTED_EDGE('',*,*,#7016,.T.);
#9897=ORIENTED_EDGE('',*,*,#6210,.F.);
#9898=ORIENTED_EDGE('',*,*,#7017,.T.);
#9899=ORIENTED_EDGE('',*,*,#6972,.T.);
#9900=ORIENTED_EDGE('',*,*,#6357,.T.);
#9901=ORIENTED_EDGE('',*,*,#6207,.F.);
#9902=ORIENTED_EDGE('',*,*,#7018,.F.);
#9903=ORIENTED_EDGE('',*,*,#6974,.T.);
#9904=ORIENTED_EDGE('',*,*,#6484,.T.);
#9905=ORIENTED_EDGE('',*,*,#7019,.T.);
#9906=ORIENTED_EDGE('',*,*,#6356,.T.);
#9907=ORIENTED_EDGE('',*,*,#6827,.F.);
#9908=ORIENTED_EDGE('',*,*,#6486,.T.);
#9909=ORIENTED_EDGE('',*,*,#6973,.F.);
#9910=ORIENTED_EDGE('',*,*,#7017,.F.);
#9911=ORIENTED_EDGE('',*,*,#6209,.F.);
#9912=ORIENTED_EDGE('',*,*,#6358,.T.);
#9913=ORIENTED_EDGE('',*,*,#7019,.F.);
#9914=ORIENTED_EDGE('',*,*,#6491,.T.);
#9915=ORIENTED_EDGE('',*,*,#6892,.T.);
#9916=ORIENTED_EDGE('',*,*,#6350,.T.);
#9917=ORIENTED_EDGE('',*,*,#6829,.F.);
#9918=ORIENTED_EDGE('',*,*,#6478,.T.);
#9919=ORIENTED_EDGE('',*,*,#6976,.F.);
#9920=ORIENTED_EDGE('',*,*,#7020,.F.);
#9921=ORIENTED_EDGE('',*,*,#6205,.F.);
#9922=ORIENTED_EDGE('',*,*,#6351,.T.);
#9923=ORIENTED_EDGE('',*,*,#6203,.F.);
#9924=ORIENTED_EDGE('',*,*,#7021,.F.);
#9925=ORIENTED_EDGE('',*,*,#6977,.T.);
#9926=ORIENTED_EDGE('',*,*,#6476,.T.);
#9927=ORIENTED_EDGE('',*,*,#7022,.T.);
#9928=ORIENTED_EDGE('',*,*,#6352,.T.);
#9929=ORIENTED_EDGE('',*,*,#7022,.F.);
#9930=ORIENTED_EDGE('',*,*,#6483,.T.);
#9931=ORIENTED_EDGE('',*,*,#6897,.T.);
#9932=ORIENTED_EDGE('',*,*,#7021,.T.);
#9933=ORIENTED_EDGE('',*,*,#6202,.F.);
#9934=ORIENTED_EDGE('',*,*,#7023,.T.);
#9935=ORIENTED_EDGE('',*,*,#6978,.T.);
#9936=ORIENTED_EDGE('',*,*,#6344,.T.);
#9937=ORIENTED_EDGE('',*,*,#6831,.F.);
#9938=ORIENTED_EDGE('',*,*,#6470,.T.);
#9939=ORIENTED_EDGE('',*,*,#6979,.F.);
#9940=ORIENTED_EDGE('',*,*,#7023,.F.);
#9941=ORIENTED_EDGE('',*,*,#6201,.F.);
#9942=ORIENTED_EDGE('',*,*,#6346,.T.);
#9943=ORIENTED_EDGE('',*,*,#7024,.F.);
#9944=ORIENTED_EDGE('',*,*,#6475,.T.);
#9945=ORIENTED_EDGE('',*,*,#6902,.T.);
#9946=ORIENTED_EDGE('',*,*,#6345,.T.);
#9947=ORIENTED_EDGE('',*,*,#6199,.F.);
#9948=ORIENTED_EDGE('',*,*,#7025,.F.);
#9949=ORIENTED_EDGE('',*,*,#6980,.T.);
#9950=ORIENTED_EDGE('',*,*,#6468,.T.);
#9951=ORIENTED_EDGE('',*,*,#7024,.T.);
#9952=ORIENTED_EDGE('',*,*,#7018,.T.);
#9953=ORIENTED_EDGE('',*,*,#6206,.F.);
#9954=ORIENTED_EDGE('',*,*,#7020,.T.);
#9955=ORIENTED_EDGE('',*,*,#6975,.T.);
#9956=ORIENTED_EDGE('',*,*,#7025,.T.);
#9957=ORIENTED_EDGE('',*,*,#6198,.F.);
#9958=ORIENTED_EDGE('',*,*,#7026,.T.);
#9959=ORIENTED_EDGE('',*,*,#6981,.T.);
#9960=ORIENTED_EDGE('',*,*,#6339,.T.);
#9961=ORIENTED_EDGE('',*,*,#6195,.F.);
#9962=ORIENTED_EDGE('',*,*,#7027,.F.);
#9963=ORIENTED_EDGE('',*,*,#6983,.T.);
#9964=ORIENTED_EDGE('',*,*,#6460,.T.);
#9965=ORIENTED_EDGE('',*,*,#7028,.T.);
#9966=ORIENTED_EDGE('',*,*,#6338,.T.);
#9967=ORIENTED_EDGE('',*,*,#6833,.F.);
#9968=ORIENTED_EDGE('',*,*,#6462,.T.);
#9969=ORIENTED_EDGE('',*,*,#6982,.F.);
#9970=ORIENTED_EDGE('',*,*,#7026,.F.);
#9971=ORIENTED_EDGE('',*,*,#6197,.F.);
#9972=ORIENTED_EDGE('',*,*,#6340,.T.);
#9973=ORIENTED_EDGE('',*,*,#7028,.F.);
#9974=ORIENTED_EDGE('',*,*,#6467,.T.);
#9975=ORIENTED_EDGE('',*,*,#6907,.T.);
#9976=ORIENTED_EDGE('',*,*,#6332,.T.);
#9977=ORIENTED_EDGE('',*,*,#6835,.F.);
#9978=ORIENTED_EDGE('',*,*,#6454,.T.);
#9979=ORIENTED_EDGE('',*,*,#6985,.F.);
#9980=ORIENTED_EDGE('',*,*,#7029,.F.);
#9981=ORIENTED_EDGE('',*,*,#6193,.F.);
#9982=ORIENTED_EDGE('',*,*,#6333,.T.);
#9983=ORIENTED_EDGE('',*,*,#6191,.F.);
#9984=ORIENTED_EDGE('',*,*,#7030,.F.);
#9985=ORIENTED_EDGE('',*,*,#6986,.T.);
#9986=ORIENTED_EDGE('',*,*,#6452,.T.);
#9987=ORIENTED_EDGE('',*,*,#7031,.T.);
#9988=ORIENTED_EDGE('',*,*,#6334,.T.);
#9989=ORIENTED_EDGE('',*,*,#7031,.F.);
#9990=ORIENTED_EDGE('',*,*,#6459,.T.);
#9991=ORIENTED_EDGE('',*,*,#6912,.T.);
#9992=ORIENTED_EDGE('',*,*,#7030,.T.);
#9993=ORIENTED_EDGE('',*,*,#6190,.F.);
#9994=ORIENTED_EDGE('',*,*,#7032,.T.);
#9995=ORIENTED_EDGE('',*,*,#6987,.T.);
#9996=ORIENTED_EDGE('',*,*,#6326,.T.);
#9997=ORIENTED_EDGE('',*,*,#6837,.F.);
#9998=ORIENTED_EDGE('',*,*,#6446,.T.);
#9999=ORIENTED_EDGE('',*,*,#6988,.F.);
#10000=ORIENTED_EDGE('',*,*,#7032,.F.);
#10001=ORIENTED_EDGE('',*,*,#6189,.F.);
#10002=ORIENTED_EDGE('',*,*,#6328,.T.);
#10003=ORIENTED_EDGE('',*,*,#7033,.F.);
#10004=ORIENTED_EDGE('',*,*,#6451,.T.);
#10005=ORIENTED_EDGE('',*,*,#6917,.T.);
#10006=ORIENTED_EDGE('',*,*,#6327,.T.);
#10007=ORIENTED_EDGE('',*,*,#6187,.F.);
#10008=ORIENTED_EDGE('',*,*,#7034,.F.);
#10009=ORIENTED_EDGE('',*,*,#6989,.T.);
#10010=ORIENTED_EDGE('',*,*,#6444,.T.);
#10011=ORIENTED_EDGE('',*,*,#7033,.T.);
#10012=ORIENTED_EDGE('',*,*,#7027,.T.);
#10013=ORIENTED_EDGE('',*,*,#6194,.F.);
#10014=ORIENTED_EDGE('',*,*,#7029,.T.);
#10015=ORIENTED_EDGE('',*,*,#6984,.T.);
#10016=ORIENTED_EDGE('',*,*,#7034,.T.);
#10017=ORIENTED_EDGE('',*,*,#6186,.F.);
#10018=ORIENTED_EDGE('',*,*,#7035,.T.);
#10019=ORIENTED_EDGE('',*,*,#6990,.T.);
#10020=ORIENTED_EDGE('',*,*,#6321,.T.);
#10021=ORIENTED_EDGE('',*,*,#6183,.F.);
#10022=ORIENTED_EDGE('',*,*,#7036,.F.);
#10023=ORIENTED_EDGE('',*,*,#6992,.T.);
#10024=ORIENTED_EDGE('',*,*,#6436,.T.);
#10025=ORIENTED_EDGE('',*,*,#7037,.T.);
#10026=ORIENTED_EDGE('',*,*,#6320,.T.);
#10027=ORIENTED_EDGE('',*,*,#6839,.F.);
#10028=ORIENTED_EDGE('',*,*,#6438,.T.);
#10029=ORIENTED_EDGE('',*,*,#6991,.F.);
#10030=ORIENTED_EDGE('',*,*,#7035,.F.);
#10031=ORIENTED_EDGE('',*,*,#6185,.F.);
#10032=ORIENTED_EDGE('',*,*,#6322,.T.);
#10033=ORIENTED_EDGE('',*,*,#7037,.F.);
#10034=ORIENTED_EDGE('',*,*,#6443,.T.);
#10035=ORIENTED_EDGE('',*,*,#6922,.T.);
#10036=ORIENTED_EDGE('',*,*,#6416,.T.);
#10037=ORIENTED_EDGE('',*,*,#6841,.F.);
#10038=ORIENTED_EDGE('',*,*,#6430,.T.);
#10039=ORIENTED_EDGE('',*,*,#6994,.F.);
#10040=ORIENTED_EDGE('',*,*,#7038,.F.);
#10041=ORIENTED_EDGE('',*,*,#6181,.F.);
#10042=ORIENTED_EDGE('',*,*,#6417,.T.);
#10043=ORIENTED_EDGE('',*,*,#6179,.F.);
#10044=ORIENTED_EDGE('',*,*,#6938,.F.);
#10045=ORIENTED_EDGE('',*,*,#6995,.T.);
#10046=ORIENTED_EDGE('',*,*,#6428,.T.);
#10047=ORIENTED_EDGE('',*,*,#7039,.T.);
#10048=ORIENTED_EDGE('',*,*,#6418,.T.);
#10049=ORIENTED_EDGE('',*,*,#7039,.F.);
#10050=ORIENTED_EDGE('',*,*,#6435,.T.);
#10051=ORIENTED_EDGE('',*,*,#6927,.T.);
#10052=ORIENTED_EDGE('',*,*,#7036,.T.);
#10053=ORIENTED_EDGE('',*,*,#6182,.F.);
#10054=ORIENTED_EDGE('',*,*,#7038,.T.);
#10055=ORIENTED_EDGE('',*,*,#6993,.T.);
#12120=CYLINDRICAL_SURFACE('',#13129,8.12525);
#12121=CYLINDRICAL_SURFACE('',#13131,8.12525);
#12122=CYLINDRICAL_SURFACE('',#13132,8.12525);
#12123=CYLINDRICAL_SURFACE('',#13133,8.12525);
#12124=CYLINDRICAL_SURFACE('',#13134,8.12525);
#12125=CYLINDRICAL_SURFACE('',#13135,8.12525);
#12126=CYLINDRICAL_SURFACE('',#13136,8.12525);
#12127=CYLINDRICAL_SURFACE('',#13137,8.12525);
#12128=CYLINDRICAL_SURFACE('',#13138,8.12525);
#12129=CYLINDRICAL_SURFACE('',#13139,8.12525);
#12130=CYLINDRICAL_SURFACE('',#13140,8.12525);
#12131=CYLINDRICAL_SURFACE('',#13141,8.12525);
#12132=CYLINDRICAL_SURFACE('',#13143,7.01125);
#12133=CYLINDRICAL_SURFACE('',#13145,7.01125);
#12134=CYLINDRICAL_SURFACE('',#13146,7.01125);
#12135=CYLINDRICAL_SURFACE('',#13147,7.01125);
#12136=CYLINDRICAL_SURFACE('',#13148,7.01125);
#12137=CYLINDRICAL_SURFACE('',#13149,7.01125);
#12138=CYLINDRICAL_SURFACE('',#13150,7.01125);
#12139=CYLINDRICAL_SURFACE('',#13151,7.01125);
#12140=CYLINDRICAL_SURFACE('',#13152,7.01125);
#12141=CYLINDRICAL_SURFACE('',#13153,7.01125);
#12142=CYLINDRICAL_SURFACE('',#13154,7.01125);
#12143=CYLINDRICAL_SURFACE('',#13155,7.01125);
#12144=CYLINDRICAL_SURFACE('',#13157,7.01125);
#12145=CYLINDRICAL_SURFACE('',#13158,8.12525);
#12146=CYLINDRICAL_SURFACE('',#13676,15.5);
#12147=CYLINDRICAL_SURFACE('',#13678,15.5);
#12148=CYLINDRICAL_SURFACE('',#13697,15.5);
#12149=CYLINDRICAL_SURFACE('',#13698,15.5);
#12150=CYLINDRICAL_SURFACE('',#13699,15.5);
#12151=CYLINDRICAL_SURFACE('',#13700,15.5);
#12152=CYLINDRICAL_SURFACE('',#13701,15.5);
#12153=CYLINDRICAL_SURFACE('',#13702,15.5);
#12154=CYLINDRICAL_SURFACE('',#13703,15.5);
#12155=CYLINDRICAL_SURFACE('',#13704,15.5);
#12156=CYLINDRICAL_SURFACE('',#13705,15.5);
#12157=CYLINDRICAL_SURFACE('',#13706,15.5);
#12158=CYLINDRICAL_SURFACE('',#13707,15.5);
#12159=CYLINDRICAL_SURFACE('',#13708,15.5);
#12160=CYLINDRICAL_SURFACE('',#13709,15.5);
#12161=CYLINDRICAL_SURFACE('',#13710,15.5);
#12162=CYLINDRICAL_SURFACE('',#13711,15.5);
#12163=CYLINDRICAL_SURFACE('',#13712,15.5);
#12326=ADVANCED_FACE('',(#796),#12120,.F.);
#12327=ADVANCED_FACE('',(#797),#12121,.F.);
#12328=ADVANCED_FACE('',(#798),#12122,.F.);
#12329=ADVANCED_FACE('',(#799),#12123,.F.);
#12330=ADVANCED_FACE('',(#800),#12124,.F.);
#12331=ADVANCED_FACE('',(#801),#12125,.F.);
#12332=ADVANCED_FACE('',(#802),#12126,.F.);
#12333=ADVANCED_FACE('',(#803),#12127,.F.);
#12334=ADVANCED_FACE('',(#804),#12128,.F.);
#12335=ADVANCED_FACE('',(#805),#12129,.F.);
#12336=ADVANCED_FACE('',(#806),#12130,.F.);
#12337=ADVANCED_FACE('',(#807),#12131,.F.);
#12338=ADVANCED_FACE('',(#808),#12132,.F.);
#12339=ADVANCED_FACE('',(#809),#12133,.F.);
#12340=ADVANCED_FACE('',(#810),#12134,.F.);
#12341=ADVANCED_FACE('',(#811),#12135,.F.);
#12342=ADVANCED_FACE('',(#812),#12136,.F.);
#12343=ADVANCED_FACE('',(#813),#12137,.F.);
#12344=ADVANCED_FACE('',(#814),#12138,.F.);
#12345=ADVANCED_FACE('',(#815),#12139,.F.);
#12346=ADVANCED_FACE('',(#816),#12140,.F.);
#12347=ADVANCED_FACE('',(#817),#12141,.F.);
#12348=ADVANCED_FACE('',(#818),#12142,.F.);
#12349=ADVANCED_FACE('',(#819),#12143,.F.);
#12350=ADVANCED_FACE('',(#820),#12144,.F.);
#12351=ADVANCED_FACE('',(#821),#12145,.F.);
#12352=ADVANCED_FACE('',(#822),#610,.F.);
#12353=ADVANCED_FACE('',(#823),#611,.F.);
#12354=ADVANCED_FACE('',(#824,#347),#440,.T.);
#12355=ADVANCED_FACE('',(#825),#441,.F.);
#12356=ADVANCED_FACE('',(#826),#442,.F.);
#12357=ADVANCED_FACE('',(#827),#443,.F.);
#12358=ADVANCED_FACE('',(#828),#444,.F.);
#12359=ADVANCED_FACE('',(#829),#445,.F.);
#12360=ADVANCED_FACE('',(#830),#446,.F.);
#12361=ADVANCED_FACE('',(#831),#447,.F.);
#12362=ADVANCED_FACE('',(#832),#448,.F.);
#12363=ADVANCED_FACE('',(#833),#449,.F.);
#12364=ADVANCED_FACE('',(#834),#450,.F.);
#12365=ADVANCED_FACE('',(#835),#451,.F.);
#12366=ADVANCED_FACE('',(#836),#452,.F.);
#12367=ADVANCED_FACE('',(#837),#453,.F.);
#12368=ADVANCED_FACE('',(#838),#454,.F.);
#12369=ADVANCED_FACE('',(#839),#455,.F.);
#12370=ADVANCED_FACE('',(#840),#456,.F.);
#12371=ADVANCED_FACE('',(#841),#457,.F.);
#12372=ADVANCED_FACE('',(#842),#458,.F.);
#12373=ADVANCED_FACE('',(#843),#290,.T.);
#12374=ADVANCED_FACE('',(#844),#291,.T.);
#12375=ADVANCED_FACE('',(#845),#292,.T.);
#12376=ADVANCED_FACE('',(#846),#293,.T.);
#12377=ADVANCED_FACE('',(#847),#294,.T.);
#12378=ADVANCED_FACE('',(#848),#295,.T.);
#12379=ADVANCED_FACE('',(#849),#296,.T.);
#12380=ADVANCED_FACE('',(#850),#297,.T.);
#12381=ADVANCED_FACE('',(#851),#298,.T.);
#12382=ADVANCED_FACE('',(#852),#299,.T.);
#12383=ADVANCED_FACE('',(#853),#300,.T.);
#12384=ADVANCED_FACE('',(#854),#301,.T.);
#12385=ADVANCED_FACE('',(#855),#302,.T.);
#12386=ADVANCED_FACE('',(#856),#303,.T.);
#12387=ADVANCED_FACE('',(#857),#304,.T.);
#12388=ADVANCED_FACE('',(#858),#305,.T.);
#12389=ADVANCED_FACE('',(#859),#306,.T.);
#12390=ADVANCED_FACE('',(#860),#307,.T.);
#12391=ADVANCED_FACE('',(#861),#308,.T.);
#12392=ADVANCED_FACE('',(#862),#309,.T.);
#12393=ADVANCED_FACE('',(#863),#310,.T.);
#12394=ADVANCED_FACE('',(#864),#311,.T.);
#12395=ADVANCED_FACE('',(#865),#312,.T.);
#12396=ADVANCED_FACE('',(#866),#313,.T.);
#12397=ADVANCED_FACE('',(#867),#314,.T.);
#12398=ADVANCED_FACE('',(#868),#315,.T.);
#12399=ADVANCED_FACE('',(#869),#316,.T.);
#12400=ADVANCED_FACE('',(#870),#317,.T.);
#12401=ADVANCED_FACE('',(#871),#318,.T.);
#12402=ADVANCED_FACE('',(#872),#319,.T.);
#12403=ADVANCED_FACE('',(#873),#320,.T.);
#12404=ADVANCED_FACE('',(#874),#321,.T.);
#12405=ADVANCED_FACE('',(#875),#322,.T.);
#12406=ADVANCED_FACE('',(#876),#323,.T.);
#12407=ADVANCED_FACE('',(#877),#324,.T.);
#12408=ADVANCED_FACE('',(#878),#325,.T.);
#12409=ADVANCED_FACE('',(#879),#459,.F.);
#12410=ADVANCED_FACE('',(#880),#460,.F.);
#12411=ADVANCED_FACE('',(#881),#461,.F.);
#12412=ADVANCED_FACE('',(#882),#462,.F.);
#12413=ADVANCED_FACE('',(#883),#463,.F.);
#12414=ADVANCED_FACE('',(#884),#464,.F.);
#12415=ADVANCED_FACE('',(#885),#465,.F.);
#12416=ADVANCED_FACE('',(#886),#466,.F.);
#12417=ADVANCED_FACE('',(#887),#467,.F.);
#12418=ADVANCED_FACE('',(#888),#468,.F.);
#12419=ADVANCED_FACE('',(#889),#469,.F.);
#12420=ADVANCED_FACE('',(#890),#470,.F.);
#12421=ADVANCED_FACE('',(#891),#471,.F.);
#12422=ADVANCED_FACE('',(#892),#472,.F.);
#12423=ADVANCED_FACE('',(#893),#473,.F.);
#12424=ADVANCED_FACE('',(#894),#474,.F.);
#12425=ADVANCED_FACE('',(#895),#475,.F.);
#12426=ADVANCED_FACE('',(#896),#476,.F.);
#12427=ADVANCED_FACE('',(#897),#477,.F.);
#12428=ADVANCED_FACE('',(#898),#478,.F.);
#12429=ADVANCED_FACE('',(#899),#479,.F.);
#12430=ADVANCED_FACE('',(#900),#480,.F.);
#12431=ADVANCED_FACE('',(#901),#481,.F.);
#12432=ADVANCED_FACE('',(#902),#482,.F.);
#12433=ADVANCED_FACE('',(#903),#483,.F.);
#12434=ADVANCED_FACE('',(#904),#484,.F.);
#12435=ADVANCED_FACE('',(#905),#485,.F.);
#12436=ADVANCED_FACE('',(#906),#486,.F.);
#12437=ADVANCED_FACE('',(#907),#487,.F.);
#12438=ADVANCED_FACE('',(#908),#488,.F.);
#12439=ADVANCED_FACE('',(#909),#489,.F.);
#12440=ADVANCED_FACE('',(#910),#490,.F.);
#12441=ADVANCED_FACE('',(#911),#491,.F.);
#12442=ADVANCED_FACE('',(#912),#492,.F.);
#12443=ADVANCED_FACE('',(#913),#493,.F.);
#12444=ADVANCED_FACE('',(#914),#494,.F.);
#12445=ADVANCED_FACE('',(#915),#495,.F.);
#12446=ADVANCED_FACE('',(#916),#496,.F.);
#12447=ADVANCED_FACE('',(#917),#497,.F.);
#12448=ADVANCED_FACE('',(#918),#498,.F.);
#12449=ADVANCED_FACE('',(#919),#499,.F.);
#12450=ADVANCED_FACE('',(#920),#500,.F.);
#12451=ADVANCED_FACE('',(#921),#501,.F.);
#12452=ADVANCED_FACE('',(#922),#502,.F.);
#12453=ADVANCED_FACE('',(#923),#503,.F.);
#12454=ADVANCED_FACE('',(#924),#504,.F.);
#12455=ADVANCED_FACE('',(#925),#505,.F.);
#12456=ADVANCED_FACE('',(#926),#506,.F.);
#12457=ADVANCED_FACE('',(#927),#507,.F.);
#12458=ADVANCED_FACE('',(#928),#508,.F.);
#12459=ADVANCED_FACE('',(#929),#509,.F.);
#12460=ADVANCED_FACE('',(#930),#510,.F.);
#12461=ADVANCED_FACE('',(#931),#511,.F.);
#12462=ADVANCED_FACE('',(#932),#512,.F.);
#12463=ADVANCED_FACE('',(#933),#152,.F.);
#12464=ADVANCED_FACE('',(#934),#153,.F.);
#12465=ADVANCED_FACE('',(#935),#154,.F.);
#12466=ADVANCED_FACE('',(#936),#155,.F.);
#12467=ADVANCED_FACE('',(#937),#156,.F.);
#12468=ADVANCED_FACE('',(#938),#157,.F.);
#12469=ADVANCED_FACE('',(#939),#158,.F.);
#12470=ADVANCED_FACE('',(#940),#159,.F.);
#12471=ADVANCED_FACE('',(#941),#160,.F.);
#12472=ADVANCED_FACE('',(#942),#161,.F.);
#12473=ADVANCED_FACE('',(#943),#162,.F.);
#12474=ADVANCED_FACE('',(#944),#163,.F.);
#12475=ADVANCED_FACE('',(#945),#164,.F.);
#12476=ADVANCED_FACE('',(#946),#165,.F.);
#12477=ADVANCED_FACE('',(#947),#166,.F.);
#12478=ADVANCED_FACE('',(#948),#167,.F.);
#12479=ADVANCED_FACE('',(#949),#168,.F.);
#12480=ADVANCED_FACE('',(#950),#169,.F.);
#12481=ADVANCED_FACE('',(#951),#612,.T.);
#12482=ADVANCED_FACE('',(#952),#613,.T.);
#12483=ADVANCED_FACE('',(#953),#614,.T.);
#12484=ADVANCED_FACE('',(#954),#615,.T.);
#12485=ADVANCED_FACE('',(#955),#616,.T.);
#12486=ADVANCED_FACE('',(#956),#617,.T.);
#12487=ADVANCED_FACE('',(#957),#618,.T.);
#12488=ADVANCED_FACE('',(#958),#619,.T.);
#12489=ADVANCED_FACE('',(#959),#620,.T.);
#12490=ADVANCED_FACE('',(#960),#621,.T.);
#12491=ADVANCED_FACE('',(#961),#622,.T.);
#12492=ADVANCED_FACE('',(#962),#623,.T.);
#12493=ADVANCED_FACE('',(#963),#624,.T.);
#12494=ADVANCED_FACE('',(#964),#625,.T.);
#12495=ADVANCED_FACE('',(#965),#626,.T.);
#12496=ADVANCED_FACE('',(#966),#627,.T.);
#12497=ADVANCED_FACE('',(#967),#628,.T.);
#12498=ADVANCED_FACE('',(#968),#629,.T.);
#12499=ADVANCED_FACE('',(#969),#630,.T.);
#12500=ADVANCED_FACE('',(#970),#631,.T.);
#12501=ADVANCED_FACE('',(#971),#632,.T.);
#12502=ADVANCED_FACE('',(#972),#633,.T.);
#12503=ADVANCED_FACE('',(#973),#634,.T.);
#12504=ADVANCED_FACE('',(#974),#635,.T.);
#12505=ADVANCED_FACE('',(#975),#636,.T.);
#12506=ADVANCED_FACE('',(#976),#637,.T.);
#12507=ADVANCED_FACE('',(#977),#638,.T.);
#12508=ADVANCED_FACE('',(#978),#639,.T.);
#12509=ADVANCED_FACE('',(#979),#640,.T.);
#12510=ADVANCED_FACE('',(#980),#641,.T.);
#12511=ADVANCED_FACE('',(#981),#642,.T.);
#12512=ADVANCED_FACE('',(#982),#643,.T.);
#12513=ADVANCED_FACE('',(#983),#644,.T.);
#12514=ADVANCED_FACE('',(#984),#645,.T.);
#12515=ADVANCED_FACE('',(#985),#646,.T.);
#12516=ADVANCED_FACE('',(#986),#647,.T.);
#12517=ADVANCED_FACE('',(#987),#648,.T.);
#12518=ADVANCED_FACE('',(#988),#649,.T.);
#12519=ADVANCED_FACE('',(#989),#650,.T.);
#12520=ADVANCED_FACE('',(#990),#651,.T.);
#12521=ADVANCED_FACE('',(#991),#652,.T.);
#12522=ADVANCED_FACE('',(#992),#653,.T.);
#12523=ADVANCED_FACE('',(#993),#654,.T.);
#12524=ADVANCED_FACE('',(#994),#655,.T.);
#12525=ADVANCED_FACE('',(#995),#656,.T.);
#12526=ADVANCED_FACE('',(#996),#657,.T.);
#12527=ADVANCED_FACE('',(#997),#658,.T.);
#12528=ADVANCED_FACE('',(#998),#659,.T.);
#12529=ADVANCED_FACE('',(#999),#660,.T.);
#12530=ADVANCED_FACE('',(#1000),#661,.T.);
#12531=ADVANCED_FACE('',(#1001),#662,.T.);
#12532=ADVANCED_FACE('',(#1002),#663,.T.);
#12533=ADVANCED_FACE('',(#1003),#664,.T.);
#12534=ADVANCED_FACE('',(#1004),#665,.T.);
#12535=ADVANCED_FACE('',(#1005),#666,.T.);
#12536=ADVANCED_FACE('',(#1006),#667,.T.);
#12537=ADVANCED_FACE('',(#1007),#668,.T.);
#12538=ADVANCED_FACE('',(#1008),#669,.T.);
#12539=ADVANCED_FACE('',(#1009),#670,.T.);
#12540=ADVANCED_FACE('',(#1010),#671,.T.);
#12541=ADVANCED_FACE('',(#1011),#672,.T.);
#12542=ADVANCED_FACE('',(#1012),#673,.T.);
#12543=ADVANCED_FACE('',(#1013),#674,.T.);
#12544=ADVANCED_FACE('',(#1014),#675,.T.);
#12545=ADVANCED_FACE('',(#1015),#676,.T.);
#12546=ADVANCED_FACE('',(#1016),#677,.T.);
#12547=ADVANCED_FACE('',(#1017),#678,.T.);
#12548=ADVANCED_FACE('',(#1018),#679,.T.);
#12549=ADVANCED_FACE('',(#1019),#680,.T.);
#12550=ADVANCED_FACE('',(#1020),#681,.T.);
#12551=ADVANCED_FACE('',(#1021),#682,.T.);
#12552=ADVANCED_FACE('',(#1022),#683,.T.);
#12553=ADVANCED_FACE('',(#1023),#684,.T.);
#12554=ADVANCED_FACE('',(#1024),#685,.T.);
#12555=ADVANCED_FACE('',(#1025),#686,.T.);
#12556=ADVANCED_FACE('',(#1026),#687,.T.);
#12557=ADVANCED_FACE('',(#1027),#688,.T.);
#12558=ADVANCED_FACE('',(#1028),#689,.T.);
#12559=ADVANCED_FACE('',(#1029),#690,.T.);
#12560=ADVANCED_FACE('',(#1030),#691,.T.);
#12561=ADVANCED_FACE('',(#1031),#692,.T.);
#12562=ADVANCED_FACE('',(#1032),#693,.T.);
#12563=ADVANCED_FACE('',(#1033),#694,.T.);
#12564=ADVANCED_FACE('',(#1034),#695,.T.);
#12565=ADVANCED_FACE('',(#1035),#696,.T.);
#12566=ADVANCED_FACE('',(#1036),#697,.T.);
#12567=ADVANCED_FACE('',(#1037),#698,.T.);
#12568=ADVANCED_FACE('',(#1038),#699,.T.);
#12569=ADVANCED_FACE('',(#1039),#700,.T.);
#12570=ADVANCED_FACE('',(#1040),#701,.T.);
#12571=ADVANCED_FACE('',(#1041),#702,.T.);
#12572=ADVANCED_FACE('',(#1042),#703,.T.);
#12573=ADVANCED_FACE('',(#1043),#704,.T.);
#12574=ADVANCED_FACE('',(#1044),#12146,.T.);
#12575=ADVANCED_FACE('',(#1045),#12147,.T.);
#12576=ADVANCED_FACE('',(#1046),#705,.T.);
#12577=ADVANCED_FACE('',(#1047),#706,.T.);
#12578=ADVANCED_FACE('',(#1048),#707,.T.);
#12579=ADVANCED_FACE('',(#1049),#708,.T.);
#12580=ADVANCED_FACE('',(#1050),#709,.T.);
#12581=ADVANCED_FACE('',(#1051),#710,.T.);
#12582=ADVANCED_FACE('',(#1052,#348),#513,.F.);
#12583=ADVANCED_FACE('',(#1053),#12148,.T.);
#12584=ADVANCED_FACE('',(#1054),#711,.T.);
#12585=ADVANCED_FACE('',(#1055),#712,.T.);
#12586=ADVANCED_FACE('',(#1056),#713,.T.);
#12587=ADVANCED_FACE('',(#1057),#12149,.T.);
#12588=ADVANCED_FACE('',(#1058),#12150,.T.);
#12589=ADVANCED_FACE('',(#1059),#714,.T.);
#12590=ADVANCED_FACE('',(#1060),#715,.T.);
#12591=ADVANCED_FACE('',(#1061),#716,.T.);
#12592=ADVANCED_FACE('',(#1062),#717,.T.);
#12593=ADVANCED_FACE('',(#1063),#718,.T.);
#12594=ADVANCED_FACE('',(#1064),#719,.T.);
#12595=ADVANCED_FACE('',(#1065),#12151,.T.);
#12596=ADVANCED_FACE('',(#1066),#720,.T.);
#12597=ADVANCED_FACE('',(#1067),#721,.T.);
#12598=ADVANCED_FACE('',(#1068),#722,.T.);
#12599=ADVANCED_FACE('',(#1069),#12152,.T.);
#12600=ADVANCED_FACE('',(#1070),#12153,.T.);
#12601=ADVANCED_FACE('',(#1071),#723,.T.);
#12602=ADVANCED_FACE('',(#1072),#724,.T.);
#12603=ADVANCED_FACE('',(#1073),#725,.T.);
#12604=ADVANCED_FACE('',(#1074),#726,.T.);
#12605=ADVANCED_FACE('',(#1075),#727,.T.);
#12606=ADVANCED_FACE('',(#1076),#728,.T.);
#12607=ADVANCED_FACE('',(#1077),#12154,.T.);
#12608=ADVANCED_FACE('',(#1078),#729,.T.);
#12609=ADVANCED_FACE('',(#1079),#730,.T.);
#12610=ADVANCED_FACE('',(#1080),#731,.T.);
#12611=ADVANCED_FACE('',(#1081),#12155,.T.);
#12612=ADVANCED_FACE('',(#1082),#12156,.T.);
#12613=ADVANCED_FACE('',(#1083),#732,.T.);
#12614=ADVANCED_FACE('',(#1084),#733,.T.);
#12615=ADVANCED_FACE('',(#1085),#734,.T.);
#12616=ADVANCED_FACE('',(#1086),#735,.T.);
#12617=ADVANCED_FACE('',(#1087),#736,.T.);
#12618=ADVANCED_FACE('',(#1088),#737,.T.);
#12619=ADVANCED_FACE('',(#1089),#12157,.T.);
#12620=ADVANCED_FACE('',(#1090),#738,.T.);
#12621=ADVANCED_FACE('',(#1091),#739,.T.);
#12622=ADVANCED_FACE('',(#1092),#740,.T.);
#12623=ADVANCED_FACE('',(#1093),#12158,.T.);
#12624=ADVANCED_FACE('',(#1094),#12159,.T.);
#12625=ADVANCED_FACE('',(#1095),#741,.T.);
#12626=ADVANCED_FACE('',(#1096),#742,.T.);
#12627=ADVANCED_FACE('',(#1097),#743,.T.);
#12628=ADVANCED_FACE('',(#1098),#744,.T.);
#12629=ADVANCED_FACE('',(#1099),#745,.T.);
#12630=ADVANCED_FACE('',(#1100),#746,.T.);
#12631=ADVANCED_FACE('',(#1101),#12160,.T.);
#12632=ADVANCED_FACE('',(#1102),#747,.T.);
#12633=ADVANCED_FACE('',(#1103),#748,.T.);
#12634=ADVANCED_FACE('',(#1104),#749,.T.);
#12635=ADVANCED_FACE('',(#1105),#12161,.T.);
#12636=ADVANCED_FACE('',(#1106),#12162,.T.);
#12637=ADVANCED_FACE('',(#1107),#750,.T.);
#12638=ADVANCED_FACE('',(#1108),#751,.T.);
#12639=ADVANCED_FACE('',(#1109),#752,.T.);
#12640=ADVANCED_FACE('',(#1110),#753,.T.);
#12641=ADVANCED_FACE('',(#1111),#754,.T.);
#12642=ADVANCED_FACE('',(#1112),#755,.T.);
#12643=ADVANCED_FACE('',(#1113),#12163,.T.);
#12992=CLOSED_SHELL('',(#12326,#12327,#12328,#12329,#12330,#12331,#12332,
#12333,#12334,#12335,#12336,#12337,#12338,#12339,#12340,#12341,#12342,#12343,
#12344,#12345,#12346,#12347,#12348,#12349,#12350,#12351,#12352,#12353,#12354,
#12355,#12356,#12357,#12358,#12359,#12360,#12361,#12362,#12363,#12364,#12365,
#12366,#12367,#12368,#12369,#12370,#12371,#12372,#12373,#12374,#12375,#12376,
#12377,#12378,#12379,#12380,#12381,#12382,#12383,#12384,#12385,#12386,#12387,
#12388,#12389,#12390,#12391,#12392,#12393,#12394,#12395,#12396,#12397,#12398,
#12399,#12400,#12401,#12402,#12403,#12404,#12405,#12406,#12407,#12408,#12409,
#12410,#12411,#12412,#12413,#12414,#12415,#12416,#12417,#12418,#12419,#12420,
#12421,#12422,#12423,#12424,#12425,#12426,#12427,#12428,#12429,#12430,#12431,
#12432,#12433,#12434,#12435,#12436,#12437,#12438,#12439,#12440,#12441,#12442,
#12443,#12444,#12445,#12446,#12447,#12448,#12449,#12450,#12451,#12452,#12453,
#12454,#12455,#12456,#12457,#12458,#12459,#12460,#12461,#12462,#12463,#12464,
#12465,#12466,#12467,#12468,#12469,#12470,#12471,#12472,#12473,#12474,#12475,
#12476,#12477,#12478,#12479,#12480,#12481,#12482,#12483,#12484,#12485,#12486,
#12487,#12488,#12489,#12490,#12491,#12492,#12493,#12494,#12495,#12496,#12497,
#12498,#12499,#12500,#12501,#12502,#12503,#12504,#12505,#12506,#12507,#12508,
#12509,#12510,#12511,#12512,#12513,#12514,#12515,#12516,#12517,#12518,#12519,
#12520,#12521,#12522,#12523,#12524,#12525,#12526,#12527,#12528,#12529,#12530,
#12531,#12532,#12533,#12534,#12535,#12536,#12537,#12538,#12539,#12540,#12541,
#12542,#12543,#12544,#12545,#12546,#12547,#12548,#12549,#12550,#12551,#12552,
#12553,#12554,#12555,#12556,#12557,#12558,#12559,#12560,#12561,#12562,#12563,
#12564,#12565,#12566,#12567,#12568,#12569,#12570,#12571,#12572,#12573,#12574,
#12575,#12576,#12577,#12578,#12579,#12580,#12581,#12582,#12583,#12584,#12585,
#12586,#12587,#12588,#12589,#12590,#12591,#12592,#12593,#12594,#12595,#12596,
#12597,#12598,#12599,#12600,#12601,#12602,#12603,#12604,#12605,#12606,#12607,
#12608,#12609,#12610,#12611,#12612,#12613,#12614,#12615,#12616,#12617,#12618,
#12619,#12620,#12621,#12622,#12623,#12624,#12625,#12626,#12627,#12628,#12629,
#12630,#12631,#12632,#12633,#12634,#12635,#12636,#12637,#12638,#12639,#12640,
#12641,#12642,#12643));
#13128=AXIS2_PLACEMENT_3D('',#17354,#14381,#14382);
#13129=AXIS2_PLACEMENT_3D('',#17355,#14383,#14384);
#13130=AXIS2_PLACEMENT_3D('',#17369,#14386,#14387);
#13131=AXIS2_PLACEMENT_3D('',#17379,#14388,#14389);
#13132=AXIS2_PLACEMENT_3D('',#17749,#14391,#14392);
#13133=AXIS2_PLACEMENT_3D('',#18127,#14394,#14395);
#13134=AXIS2_PLACEMENT_3D('',#18583,#14397,#14398);
#13135=AXIS2_PLACEMENT_3D('',#18967,#14400,#14401);
#13136=AXIS2_PLACEMENT_3D('',#19419,#14403,#14404);
#13137=AXIS2_PLACEMENT_3D('',#19803,#14406,#14407);
#13138=AXIS2_PLACEMENT_3D('',#20101,#14409,#14410);
#13139=AXIS2_PLACEMENT_3D('',#20393,#14412,#14413);
#13140=AXIS2_PLACEMENT_3D('',#20689,#14415,#14416);
#13141=AXIS2_PLACEMENT_3D('',#20986,#14418,#14419);
#13142=AXIS2_PLACEMENT_3D('',#21008,#14421,#14422);
#13143=AXIS2_PLACEMENT_3D('',#21183,#14423,#14424);
#13144=AXIS2_PLACEMENT_3D('',#21197,#14426,#14427);
#13145=AXIS2_PLACEMENT_3D('',#21286,#14428,#14429);
#13146=AXIS2_PLACEMENT_3D('',#21478,#14431,#14432);
#13147=AXIS2_PLACEMENT_3D('',#21770,#14434,#14435);
#13148=AXIS2_PLACEMENT_3D('',#22065,#14437,#14438);
#13149=AXIS2_PLACEMENT_3D('',#22360,#14440,#14441);
#13150=AXIS2_PLACEMENT_3D('',#22656,#14443,#14444);
#13151=AXIS2_PLACEMENT_3D('',#23072,#14446,#14447);
#13152=AXIS2_PLACEMENT_3D('',#23261,#14449,#14450);
#13153=AXIS2_PLACEMENT_3D('',#23675,#14452,#14453);
#13154=AXIS2_PLACEMENT_3D('',#23976,#14455,#14456);
#13155=AXIS2_PLACEMENT_3D('',#24390,#14458,#14459);
#13156=AXIS2_PLACEMENT_3D('',#24562,#14461,#14462);
#13157=AXIS2_PLACEMENT_3D('',#24701,#14463,#14464);
#13158=AXIS2_PLACEMENT_3D('',#24880,#14465,#14466);
#13159=AXIS2_PLACEMENT_3D('',#26894,#14467,#14468);
#13160=AXIS2_PLACEMENT_3D('',#26897,#14469,#14470);
#13161=AXIS2_PLACEMENT_3D('',#26901,#14472,#14473);
#13162=AXIS2_PLACEMENT_3D('',#26905,#14475,#14476);
#13163=AXIS2_PLACEMENT_3D('',#26909,#14478,#14479);
#13164=AXIS2_PLACEMENT_3D('',#26913,#14481,#14482);
#13165=AXIS2_PLACEMENT_3D('',#26917,#14484,#14485);
#13166=AXIS2_PLACEMENT_3D('',#26921,#14487,#14488);
#13167=AXIS2_PLACEMENT_3D('',#26925,#14490,#14491);
#13168=AXIS2_PLACEMENT_3D('',#26929,#14493,#14494);
#13169=AXIS2_PLACEMENT_3D('',#26933,#14496,#14497);
#13170=AXIS2_PLACEMENT_3D('',#26937,#14499,#14500);
#13171=AXIS2_PLACEMENT_3D('',#26941,#14502,#14503);
#13172=AXIS2_PLACEMENT_3D('',#26945,#14505,#14506);
#13173=AXIS2_PLACEMENT_3D('',#26949,#14508,#14509);
#13174=AXIS2_PLACEMENT_3D('',#26953,#14511,#14512);
#13175=AXIS2_PLACEMENT_3D('',#26957,#14514,#14515);
#13176=AXIS2_PLACEMENT_3D('',#26961,#14517,#14518);
#13177=AXIS2_PLACEMENT_3D('',#26965,#14520,#14521);
#13178=AXIS2_PLACEMENT_3D('',#26969,#14523,#14524);
#13179=AXIS2_PLACEMENT_3D('',#26973,#14526,#14527);
#13180=AXIS2_PLACEMENT_3D('',#26977,#14529,#14530);
#13181=AXIS2_PLACEMENT_3D('',#26981,#14532,#14533);
#13182=AXIS2_PLACEMENT_3D('',#26985,#14535,#14536);
#13183=AXIS2_PLACEMENT_3D('',#26989,#14538,#14539);
#13184=AXIS2_PLACEMENT_3D('',#26993,#14541,#14542);
#13185=AXIS2_PLACEMENT_3D('',#26997,#14544,#14545);
#13186=AXIS2_PLACEMENT_3D('',#27001,#14547,#14548);
#13187=AXIS2_PLACEMENT_3D('',#27005,#14550,#14551);
#13188=AXIS2_PLACEMENT_3D('',#27009,#14553,#14554);
#13189=AXIS2_PLACEMENT_3D('',#27013,#14556,#14557);
#13190=AXIS2_PLACEMENT_3D('',#27017,#14559,#14560);
#13191=AXIS2_PLACEMENT_3D('',#27021,#14562,#14563);
#13192=AXIS2_PLACEMENT_3D('',#27025,#14565,#14566);
#13193=AXIS2_PLACEMENT_3D('',#27029,#14568,#14569);
#13194=AXIS2_PLACEMENT_3D('',#27033,#14571,#14572);
#13195=AXIS2_PLACEMENT_3D('',#27037,#14574,#14575);
#13196=AXIS2_PLACEMENT_3D('',#27039,#14577,#14578);
#13197=AXIS2_PLACEMENT_3D('',#27044,#14580,#14581);
#13198=AXIS2_PLACEMENT_3D('',#27047,#14583,#14584);
#13199=AXIS2_PLACEMENT_3D('',#27048,#14585,#14586);
#13200=AXIS2_PLACEMENT_3D('',#27053,#14588,#14589);
#13201=AXIS2_PLACEMENT_3D('',#27056,#14591,#14592);
#13202=AXIS2_PLACEMENT_3D('',#27057,#14593,#14594);
#13203=AXIS2_PLACEMENT_3D('',#27062,#14596,#14597);
#13204=AXIS2_PLACEMENT_3D('',#27065,#14599,#14600);
#13205=AXIS2_PLACEMENT_3D('',#27066,#14601,#14602);
#13206=AXIS2_PLACEMENT_3D('',#27071,#14604,#14605);
#13207=AXIS2_PLACEMENT_3D('',#27074,#14607,#14608);
#13208=AXIS2_PLACEMENT_3D('',#27075,#14609,#14610);
#13209=AXIS2_PLACEMENT_3D('',#27080,#14612,#14613);
#13210=AXIS2_PLACEMENT_3D('',#27083,#14615,#14616);
#13211=AXIS2_PLACEMENT_3D('',#27084,#14617,#14618);
#13212=AXIS2_PLACEMENT_3D('',#27089,#14620,#14621);
#13213=AXIS2_PLACEMENT_3D('',#27092,#14623,#14624);
#13214=AXIS2_PLACEMENT_3D('',#27093,#14625,#14626);
#13215=AXIS2_PLACEMENT_3D('',#27098,#14628,#14629);
#13216=AXIS2_PLACEMENT_3D('',#27101,#14631,#14632);
#13217=AXIS2_PLACEMENT_3D('',#27102,#14633,#14634);
#13218=AXIS2_PLACEMENT_3D('',#27107,#14636,#14637);
#13219=AXIS2_PLACEMENT_3D('',#27110,#14639,#14640);
#13220=AXIS2_PLACEMENT_3D('',#27111,#14641,#14642);
#13221=AXIS2_PLACEMENT_3D('',#27116,#14644,#14645);
#13222=AXIS2_PLACEMENT_3D('',#27119,#14647,#14648);
#13223=AXIS2_PLACEMENT_3D('',#27120,#14649,#14650);
#13224=AXIS2_PLACEMENT_3D('',#27125,#14652,#14653);
#13225=AXIS2_PLACEMENT_3D('',#27128,#14655,#14656);
#13226=AXIS2_PLACEMENT_3D('',#27129,#14657,#14658);
#13227=AXIS2_PLACEMENT_3D('',#27134,#14660,#14661);
#13228=AXIS2_PLACEMENT_3D('',#27137,#14663,#14664);
#13229=AXIS2_PLACEMENT_3D('',#27138,#14665,#14666);
#13230=AXIS2_PLACEMENT_3D('',#27143,#14668,#14669);
#13231=AXIS2_PLACEMENT_3D('',#27146,#14671,#14672);
#13232=AXIS2_PLACEMENT_3D('',#27147,#14673,#14674);
#13233=AXIS2_PLACEMENT_3D('',#27152,#14676,#14677);
#13234=AXIS2_PLACEMENT_3D('',#27155,#14679,#14680);
#13235=AXIS2_PLACEMENT_3D('',#27156,#14681,#14682);
#13236=AXIS2_PLACEMENT_3D('',#27161,#14684,#14685);
#13237=AXIS2_PLACEMENT_3D('',#27164,#14687,#14688);
#13238=AXIS2_PLACEMENT_3D('',#27165,#14689,#14690);
#13239=AXIS2_PLACEMENT_3D('',#27170,#14692,#14693);
#13240=AXIS2_PLACEMENT_3D('',#27173,#14695,#14696);
#13241=AXIS2_PLACEMENT_3D('',#27174,#14697,#14698);
#13242=AXIS2_PLACEMENT_3D('',#27179,#14700,#14701);
#13243=AXIS2_PLACEMENT_3D('',#27182,#14703,#14704);
#13244=AXIS2_PLACEMENT_3D('',#27183,#14705,#14706);
#13245=AXIS2_PLACEMENT_3D('',#27188,#14708,#14709);
#13246=AXIS2_PLACEMENT_3D('',#27191,#14711,#14712);
#13247=AXIS2_PLACEMENT_3D('',#27192,#14713,#14714);
#13248=AXIS2_PLACEMENT_3D('',#27197,#14716,#14717);
#13249=AXIS2_PLACEMENT_3D('',#27200,#14719,#14720);
#13250=AXIS2_PLACEMENT_3D('',#27201,#14721,#14722);
#13251=AXIS2_PLACEMENT_3D('',#27203,#14723,#14724);
#13252=AXIS2_PLACEMENT_3D('',#27205,#14725,#14726);
#13253=AXIS2_PLACEMENT_3D('',#27228,#14729,#14730);
#13254=AXIS2_PLACEMENT_3D('',#27230,#14731,#14732);
#13255=AXIS2_PLACEMENT_3D('',#27232,#14733,#14734);
#13256=AXIS2_PLACEMENT_3D('',#27255,#14737,#14738);
#13257=AXIS2_PLACEMENT_3D('',#27257,#14739,#14740);
#13258=AXIS2_PLACEMENT_3D('',#27259,#14741,#14742);
#13259=AXIS2_PLACEMENT_3D('',#27280,#14745,#14746);
#13260=AXIS2_PLACEMENT_3D('',#27282,#14747,#14748);
#13261=AXIS2_PLACEMENT_3D('',#27284,#14749,#14750);
#13262=AXIS2_PLACEMENT_3D('',#27307,#14753,#14754);
#13263=AXIS2_PLACEMENT_3D('',#27309,#14755,#14756);
#13264=AXIS2_PLACEMENT_3D('',#27311,#14757,#14758);
#13265=AXIS2_PLACEMENT_3D('',#27334,#14761,#14762);
#13266=AXIS2_PLACEMENT_3D('',#27336,#14763,#14764);
#13267=AXIS2_PLACEMENT_3D('',#27338,#14765,#14766);
#13268=AXIS2_PLACEMENT_3D('',#27361,#14769,#14770);
#13269=AXIS2_PLACEMENT_3D('',#27363,#14771,#14772);
#13270=AXIS2_PLACEMENT_3D('',#27365,#14773,#14774);
#13271=AXIS2_PLACEMENT_3D('',#27386,#14777,#14778);
#13272=AXIS2_PLACEMENT_3D('',#27388,#14779,#14780);
#13273=AXIS2_PLACEMENT_3D('',#27390,#14781,#14782);
#13274=AXIS2_PLACEMENT_3D('',#27413,#14785,#14786);
#13275=AXIS2_PLACEMENT_3D('',#27415,#14787,#14788);
#13276=AXIS2_PLACEMENT_3D('',#27417,#14789,#14790);
#13277=AXIS2_PLACEMENT_3D('',#27440,#14793,#14794);
#13278=AXIS2_PLACEMENT_3D('',#27442,#14795,#14796);
#13279=AXIS2_PLACEMENT_3D('',#27444,#14797,#14798);
#13280=AXIS2_PLACEMENT_3D('',#27467,#14801,#14802);
#13281=AXIS2_PLACEMENT_3D('',#27469,#14803,#14804);
#13282=AXIS2_PLACEMENT_3D('',#27471,#14805,#14806);
#13283=AXIS2_PLACEMENT_3D('',#27492,#14809,#14810);
#13284=AXIS2_PLACEMENT_3D('',#27494,#14811,#14812);
#13285=AXIS2_PLACEMENT_3D('',#27496,#14813,#14814);
#13286=AXIS2_PLACEMENT_3D('',#27519,#14817,#14818);
#13287=AXIS2_PLACEMENT_3D('',#27521,#14819,#14820);
#13288=AXIS2_PLACEMENT_3D('',#27523,#14821,#14822);
#13289=AXIS2_PLACEMENT_3D('',#27546,#14825,#14826);
#13290=AXIS2_PLACEMENT_3D('',#27548,#14827,#14828);
#13291=AXIS2_PLACEMENT_3D('',#27550,#14829,#14830);
#13292=AXIS2_PLACEMENT_3D('',#27573,#14833,#14834);
#13293=AXIS2_PLACEMENT_3D('',#27575,#14835,#14836);
#13294=AXIS2_PLACEMENT_3D('',#27577,#14837,#14838);
#13295=AXIS2_PLACEMENT_3D('',#27600,#14841,#14842);
#13296=AXIS2_PLACEMENT_3D('',#27602,#14843,#14844);
#13297=AXIS2_PLACEMENT_3D('',#27604,#14845,#14846);
#13298=AXIS2_PLACEMENT_3D('',#27627,#14849,#14850);
#13299=AXIS2_PLACEMENT_3D('',#27629,#14851,#14852);
#13300=AXIS2_PLACEMENT_3D('',#27631,#14853,#14854);
#13301=AXIS2_PLACEMENT_3D('',#27654,#14857,#14858);
#13302=AXIS2_PLACEMENT_3D('',#27656,#14859,#14860);
#13303=AXIS2_PLACEMENT_3D('',#27658,#14861,#14862);
#13304=AXIS2_PLACEMENT_3D('',#27681,#14865,#14866);
#13305=AXIS2_PLACEMENT_3D('',#27684,#14867,#14868);
#13306=AXIS2_PLACEMENT_3D('',#27686,#14869,#14870);
#13307=AXIS2_PLACEMENT_3D('',#27688,#14871,#14872);
#13308=AXIS2_PLACEMENT_3D('',#27701,#14874,#14875);
#13309=AXIS2_PLACEMENT_3D('',#27714,#14877,#14878);
#13310=AXIS2_PLACEMENT_3D('',#27717,#14879,#14880);
#13311=AXIS2_PLACEMENT_3D('',#27719,#14881,#14882);
#13312=AXIS2_PLACEMENT_3D('',#27721,#14883,#14884);
#13313=AXIS2_PLACEMENT_3D('',#27736,#14886,#14887);
#13314=AXIS2_PLACEMENT_3D('',#27747,#14889,#14890);
#13315=AXIS2_PLACEMENT_3D('',#27750,#14891,#14892);
#13316=AXIS2_PLACEMENT_3D('',#27752,#14893,#14894);
#13317=AXIS2_PLACEMENT_3D('',#27754,#14895,#14896);
#13318=AXIS2_PLACEMENT_3D('',#27769,#14898,#14899);
#13319=AXIS2_PLACEMENT_3D('',#27782,#14901,#14902);
#13320=AXIS2_PLACEMENT_3D('',#27785,#14903,#14904);
#13321=AXIS2_PLACEMENT_3D('',#27787,#14905,#14906);
#13322=AXIS2_PLACEMENT_3D('',#27789,#14907,#14908);
#13323=AXIS2_PLACEMENT_3D('',#27802,#14910,#14911);
#13324=AXIS2_PLACEMENT_3D('',#27813,#14913,#14914);
#13325=AXIS2_PLACEMENT_3D('',#27816,#14915,#14916);
#13326=AXIS2_PLACEMENT_3D('',#27818,#14917,#14918);
#13327=AXIS2_PLACEMENT_3D('',#27820,#14919,#14920);
#13328=AXIS2_PLACEMENT_3D('',#27835,#14922,#14923);
#13329=AXIS2_PLACEMENT_3D('',#27848,#14925,#14926);
#13330=AXIS2_PLACEMENT_3D('',#27851,#14927,#14928);
#13331=AXIS2_PLACEMENT_3D('',#27853,#14929,#14930);
#13332=AXIS2_PLACEMENT_3D('',#27855,#14931,#14932);
#13333=AXIS2_PLACEMENT_3D('',#27870,#14934,#14935);
#13334=AXIS2_PLACEMENT_3D('',#27883,#14937,#14938);
#13335=AXIS2_PLACEMENT_3D('',#27886,#14939,#14940);
#13336=AXIS2_PLACEMENT_3D('',#27888,#14941,#14942);
#13337=AXIS2_PLACEMENT_3D('',#27890,#14943,#14944);
#13338=AXIS2_PLACEMENT_3D('',#27905,#14946,#14947);
#13339=AXIS2_PLACEMENT_3D('',#27916,#14949,#14950);
#13340=AXIS2_PLACEMENT_3D('',#27919,#14951,#14952);
#13341=AXIS2_PLACEMENT_3D('',#27921,#14953,#14954);
#13342=AXIS2_PLACEMENT_3D('',#27923,#14955,#14956);
#13343=AXIS2_PLACEMENT_3D('',#27936,#14958,#14959);
#13344=AXIS2_PLACEMENT_3D('',#27949,#14961,#14962);
#13345=AXIS2_PLACEMENT_3D('',#27952,#14963,#14964);
#13346=AXIS2_PLACEMENT_3D('',#27954,#14965,#14966);
#13347=AXIS2_PLACEMENT_3D('',#27956,#14967,#14968);
#13348=AXIS2_PLACEMENT_3D('',#27971,#14970,#14971);
#13349=AXIS2_PLACEMENT_3D('',#27984,#14973,#14974);
#13350=AXIS2_PLACEMENT_3D('',#27987,#14975,#14976);
#13351=AXIS2_PLACEMENT_3D('',#27989,#14977,#14978);
#13352=AXIS2_PLACEMENT_3D('',#27991,#14979,#14980);
#13353=AXIS2_PLACEMENT_3D('',#28006,#14982,#14983);
#13354=AXIS2_PLACEMENT_3D('',#28019,#14985,#14986);
#13355=AXIS2_PLACEMENT_3D('',#28022,#14987,#14988);
#13356=AXIS2_PLACEMENT_3D('',#28024,#14989,#14990);
#13357=AXIS2_PLACEMENT_3D('',#28026,#14991,#14992);
#13358=AXIS2_PLACEMENT_3D('',#28041,#14994,#14995);
#13359=AXIS2_PLACEMENT_3D('',#28052,#14997,#14998);
#13360=AXIS2_PLACEMENT_3D('',#28055,#14999,#15000);
#13361=AXIS2_PLACEMENT_3D('',#28057,#15001,#15002);
#13362=AXIS2_PLACEMENT_3D('',#28059,#15003,#15004);
#13363=AXIS2_PLACEMENT_3D('',#28072,#15006,#15007);
#13364=AXIS2_PLACEMENT_3D('',#28085,#15009,#15010);
#13365=AXIS2_PLACEMENT_3D('',#28088,#15011,#15012);
#13366=AXIS2_PLACEMENT_3D('',#28090,#15013,#15014);
#13367=AXIS2_PLACEMENT_3D('',#28092,#15015,#15016);
#13368=AXIS2_PLACEMENT_3D('',#28107,#15018,#15019);
#13369=AXIS2_PLACEMENT_3D('',#28118,#15021,#15022);
#13370=AXIS2_PLACEMENT_3D('',#28121,#15023,#15024);
#13371=AXIS2_PLACEMENT_3D('',#28123,#15025,#15026);
#13372=AXIS2_PLACEMENT_3D('',#28125,#15027,#15028);
#13373=AXIS2_PLACEMENT_3D('',#28140,#15030,#15031);
#13374=AXIS2_PLACEMENT_3D('',#28153,#15033,#15034);
#13375=AXIS2_PLACEMENT_3D('',#28156,#15035,#15036);
#13376=AXIS2_PLACEMENT_3D('',#28158,#15037,#15038);
#13377=AXIS2_PLACEMENT_3D('',#28160,#15039,#15040);
#13378=AXIS2_PLACEMENT_3D('',#28175,#15042,#15043);
#13379=AXIS2_PLACEMENT_3D('',#28188,#15045,#15046);
#13380=AXIS2_PLACEMENT_3D('',#28191,#15047,#15048);
#13381=AXIS2_PLACEMENT_3D('',#28193,#15049,#15050);
#13382=AXIS2_PLACEMENT_3D('',#28195,#15051,#15052);
#13383=AXIS2_PLACEMENT_3D('',#28210,#15054,#15055);
#13384=AXIS2_PLACEMENT_3D('',#28221,#15057,#15058);
#13385=AXIS2_PLACEMENT_3D('',#28224,#15059,#15060);
#13386=AXIS2_PLACEMENT_3D('',#28226,#15061,#15062);
#13387=AXIS2_PLACEMENT_3D('',#28228,#15063,#15064);
#13388=AXIS2_PLACEMENT_3D('',#28241,#15066,#15067);
#13389=AXIS2_PLACEMENT_3D('',#28254,#15069,#15070);
#13390=AXIS2_PLACEMENT_3D('',#28257,#15071,#15072);
#13391=AXIS2_PLACEMENT_3D('',#28259,#15073,#15074);
#13392=AXIS2_PLACEMENT_3D('',#28261,#15075,#15076);
#13393=AXIS2_PLACEMENT_3D('',#28274,#15078,#15079);
#13394=AXIS2_PLACEMENT_3D('',#28285,#15081,#15082);
#13395=AXIS2_PLACEMENT_3D('',#28290,#15085,#15086);
#13396=AXIS2_PLACEMENT_3D('',#28291,#15087,#15088);
#13397=AXIS2_PLACEMENT_3D('',#28296,#15091,#15092);
#13398=AXIS2_PLACEMENT_3D('',#28297,#15093,#15094);
#13399=AXIS2_PLACEMENT_3D('',#28302,#15097,#15098);
#13400=AXIS2_PLACEMENT_3D('',#28303,#15099,#15100);
#13401=AXIS2_PLACEMENT_3D('',#28308,#15103,#15104);
#13402=AXIS2_PLACEMENT_3D('',#28309,#15105,#15106);
#13403=AXIS2_PLACEMENT_3D('',#28314,#15109,#15110);
#13404=AXIS2_PLACEMENT_3D('',#28315,#15111,#15112);
#13405=AXIS2_PLACEMENT_3D('',#28320,#15115,#15116);
#13406=AXIS2_PLACEMENT_3D('',#28321,#15117,#15118);
#13407=AXIS2_PLACEMENT_3D('',#28326,#15121,#15122);
#13408=AXIS2_PLACEMENT_3D('',#28327,#15123,#15124);
#13409=AXIS2_PLACEMENT_3D('',#28332,#15127,#15128);
#13410=AXIS2_PLACEMENT_3D('',#28333,#15129,#15130);
#13411=AXIS2_PLACEMENT_3D('',#28338,#15133,#15134);
#13412=AXIS2_PLACEMENT_3D('',#28339,#15135,#15136);
#13413=AXIS2_PLACEMENT_3D('',#28344,#15139,#15140);
#13414=AXIS2_PLACEMENT_3D('',#28345,#15141,#15142);
#13415=AXIS2_PLACEMENT_3D('',#28350,#15145,#15146);
#13416=AXIS2_PLACEMENT_3D('',#28351,#15147,#15148);
#13417=AXIS2_PLACEMENT_3D('',#28356,#15151,#15152);
#13418=AXIS2_PLACEMENT_3D('',#28357,#15153,#15154);
#13419=AXIS2_PLACEMENT_3D('',#28362,#15157,#15158);
#13420=AXIS2_PLACEMENT_3D('',#28363,#15159,#15160);
#13421=AXIS2_PLACEMENT_3D('',#28368,#15163,#15164);
#13422=AXIS2_PLACEMENT_3D('',#28369,#15165,#15166);
#13423=AXIS2_PLACEMENT_3D('',#28374,#15169,#15170);
#13424=AXIS2_PLACEMENT_3D('',#28375,#15171,#15172);
#13425=AXIS2_PLACEMENT_3D('',#28380,#15175,#15176);
#13426=AXIS2_PLACEMENT_3D('',#28381,#15177,#15178);
#13427=AXIS2_PLACEMENT_3D('',#28386,#15181,#15182);
#13428=AXIS2_PLACEMENT_3D('',#28387,#15183,#15184);
#13429=AXIS2_PLACEMENT_3D('',#28392,#15187,#15188);
#13430=AXIS2_PLACEMENT_3D('',#28393,#15189,#15190);
#13431=AXIS2_PLACEMENT_3D('',#28396,#15191,#15192);
#13432=AXIS2_PLACEMENT_3D('',#28398,#15193,#15194);
#13433=AXIS2_PLACEMENT_3D('',#28406,#15195,#15196);
#13434=AXIS2_PLACEMENT_3D('',#28407,#15197,#15198);
#13435=AXIS2_PLACEMENT_3D('',#28410,#15199,#15200);
#13436=AXIS2_PLACEMENT_3D('',#28412,#15201,#15202);
#13437=AXIS2_PLACEMENT_3D('',#28414,#15203,#15204);
#13438=AXIS2_PLACEMENT_3D('',#28415,#15205,#15206);
#13439=AXIS2_PLACEMENT_3D('',#28416,#15207,#15208);
#13440=AXIS2_PLACEMENT_3D('',#28419,#15209,#15210);
#13441=AXIS2_PLACEMENT_3D('',#28421,#15211,#15212);
#13442=AXIS2_PLACEMENT_3D('',#28423,#15213,#15214);
#13443=AXIS2_PLACEMENT_3D('',#28424,#15215,#15216);
#13444=AXIS2_PLACEMENT_3D('',#28425,#15217,#15218);
#13445=AXIS2_PLACEMENT_3D('',#28428,#15219,#15220);
#13446=AXIS2_PLACEMENT_3D('',#28430,#15221,#15222);
#13447=AXIS2_PLACEMENT_3D('',#28438,#15223,#15224);
#13448=AXIS2_PLACEMENT_3D('',#28439,#15225,#15226);
#13449=AXIS2_PLACEMENT_3D('',#28442,#15227,#15228);
#13450=AXIS2_PLACEMENT_3D('',#28444,#15229,#15230);
#13451=AXIS2_PLACEMENT_3D('',#28446,#15231,#15232);
#13452=AXIS2_PLACEMENT_3D('',#28447,#15233,#15234);
#13453=AXIS2_PLACEMENT_3D('',#28448,#15235,#15236);
#13454=AXIS2_PLACEMENT_3D('',#28451,#15237,#15238);
#13455=AXIS2_PLACEMENT_3D('',#28453,#15239,#15240);
#13456=AXIS2_PLACEMENT_3D('',#28455,#15241,#15242);
#13457=AXIS2_PLACEMENT_3D('',#28456,#15243,#15244);
#13458=AXIS2_PLACEMENT_3D('',#28457,#15245,#15246);
#13459=AXIS2_PLACEMENT_3D('',#28460,#15247,#15248);
#13460=AXIS2_PLACEMENT_3D('',#28462,#15249,#15250);
#13461=AXIS2_PLACEMENT_3D('',#28464,#15251,#15252);
#13462=AXIS2_PLACEMENT_3D('',#28465,#15253,#15254);
#13463=AXIS2_PLACEMENT_3D('',#28466,#15255,#15256);
#13464=AXIS2_PLACEMENT_3D('',#28469,#15257,#15258);
#13465=AXIS2_PLACEMENT_3D('',#28471,#15259,#15260);
#13466=AXIS2_PLACEMENT_3D('',#28479,#15261,#15262);
#13467=AXIS2_PLACEMENT_3D('',#28480,#15263,#15264);
#13468=AXIS2_PLACEMENT_3D('',#28483,#15265,#15266);
#13469=AXIS2_PLACEMENT_3D('',#28485,#15267,#15268);
#13470=AXIS2_PLACEMENT_3D('',#28487,#15269,#15270);
#13471=AXIS2_PLACEMENT_3D('',#28488,#15271,#15272);
#13472=AXIS2_PLACEMENT_3D('',#28489,#15273,#15274);
#13473=AXIS2_PLACEMENT_3D('',#28492,#15275,#15276);
#13474=AXIS2_PLACEMENT_3D('',#28494,#15277,#15278);
#13475=AXIS2_PLACEMENT_3D('',#28496,#15279,#15280);
#13476=AXIS2_PLACEMENT_3D('',#28497,#15281,#15282);
#13477=AXIS2_PLACEMENT_3D('',#28498,#15283,#15284);
#13478=AXIS2_PLACEMENT_3D('',#28501,#15285,#15286);
#13479=AXIS2_PLACEMENT_3D('',#28503,#15287,#15288);
#13480=AXIS2_PLACEMENT_3D('',#28505,#15289,#15290);
#13481=AXIS2_PLACEMENT_3D('',#28506,#15291,#15292);
#13482=AXIS2_PLACEMENT_3D('',#28507,#15293,#15294);
#13483=AXIS2_PLACEMENT_3D('',#28510,#15295,#15296);
#13484=AXIS2_PLACEMENT_3D('',#28512,#15297,#15298);
#13485=AXIS2_PLACEMENT_3D('',#28520,#15299,#15300);
#13486=AXIS2_PLACEMENT_3D('',#28521,#15301,#15302);
#13487=AXIS2_PLACEMENT_3D('',#28524,#15303,#15304);
#13488=AXIS2_PLACEMENT_3D('',#28526,#15305,#15306);
#13489=AXIS2_PLACEMENT_3D('',#28528,#15307,#15308);
#13490=AXIS2_PLACEMENT_3D('',#28529,#15309,#15310);
#13491=AXIS2_PLACEMENT_3D('',#28530,#15311,#15312);
#13492=AXIS2_PLACEMENT_3D('',#28533,#15313,#15314);
#13493=AXIS2_PLACEMENT_3D('',#28535,#15315,#15316);
#13494=AXIS2_PLACEMENT_3D('',#28537,#15317,#15318);
#13495=AXIS2_PLACEMENT_3D('',#28538,#15319,#15320);
#13496=AXIS2_PLACEMENT_3D('',#28539,#15321,#15322);
#13497=AXIS2_PLACEMENT_3D('',#28542,#15323,#15324);
#13498=AXIS2_PLACEMENT_3D('',#28544,#15325,#15326);
#13499=AXIS2_PLACEMENT_3D('',#28546,#15327,#15328);
#13500=AXIS2_PLACEMENT_3D('',#28547,#15329,#15330);
#13501=AXIS2_PLACEMENT_3D('',#28548,#15331,#15332);
#13502=AXIS2_PLACEMENT_3D('',#28551,#15333,#15334);
#13503=AXIS2_PLACEMENT_3D('',#28553,#15335,#15336);
#13504=AXIS2_PLACEMENT_3D('',#28555,#15337,#15338);
#13505=AXIS2_PLACEMENT_3D('',#28556,#15339,#15340);
#13506=AXIS2_PLACEMENT_3D('',#28557,#15341,#15342);
#13507=AXIS2_PLACEMENT_3D('',#28560,#15343,#15344);
#13508=AXIS2_PLACEMENT_3D('',#28562,#15345,#15346);
#13509=AXIS2_PLACEMENT_3D('',#28570,#15347,#15348);
#13510=AXIS2_PLACEMENT_3D('',#28571,#15349,#15350);
#13511=AXIS2_PLACEMENT_3D('',#28574,#15351,#15352);
#13512=AXIS2_PLACEMENT_3D('',#28576,#15353,#15354);
#13513=AXIS2_PLACEMENT_3D('',#28584,#15355,#15356);
#13514=AXIS2_PLACEMENT_3D('',#28585,#15357,#15358);
#13515=AXIS2_PLACEMENT_3D('',#28595,#15359,#15360);
#13516=AXIS2_PLACEMENT_3D('',#28597,#15361,#15362);
#13517=AXIS2_PLACEMENT_3D('',#28598,#15363,#15364);
#13518=AXIS2_PLACEMENT_3D('',#28599,#15365,#15366);
#13519=AXIS2_PLACEMENT_3D('',#28609,#15367,#15368);
#13520=AXIS2_PLACEMENT_3D('',#28611,#15369,#15370);
#13521=AXIS2_PLACEMENT_3D('',#28612,#15371,#15372);
#13522=AXIS2_PLACEMENT_3D('',#28613,#15373,#15374);
#13523=AXIS2_PLACEMENT_3D('',#28623,#15375,#15376);
#13524=AXIS2_PLACEMENT_3D('',#28625,#15377,#15378);
#13525=AXIS2_PLACEMENT_3D('',#28626,#15379,#15380);
#13526=AXIS2_PLACEMENT_3D('',#28627,#15381,#15382);
#13527=AXIS2_PLACEMENT_3D('',#28637,#15383,#15384);
#13528=AXIS2_PLACEMENT_3D('',#28639,#15385,#15386);
#13529=AXIS2_PLACEMENT_3D('',#28640,#15387,#15388);
#13530=AXIS2_PLACEMENT_3D('',#28641,#15389,#15390);
#13531=AXIS2_PLACEMENT_3D('',#28651,#15391,#15392);
#13532=AXIS2_PLACEMENT_3D('',#28653,#15393,#15394);
#13533=AXIS2_PLACEMENT_3D('',#28654,#15395,#15396);
#13534=AXIS2_PLACEMENT_3D('',#28655,#15397,#15398);
#13535=AXIS2_PLACEMENT_3D('',#28665,#15399,#15400);
#13536=AXIS2_PLACEMENT_3D('',#28667,#15401,#15402);
#13537=AXIS2_PLACEMENT_3D('',#28668,#15403,#15404);
#13538=AXIS2_PLACEMENT_3D('',#28669,#15405,#15406);
#13539=AXIS2_PLACEMENT_3D('',#28679,#15407,#15408);
#13540=AXIS2_PLACEMENT_3D('',#28681,#15409,#15410);
#13541=AXIS2_PLACEMENT_3D('',#28682,#15411,#15412);
#13542=AXIS2_PLACEMENT_3D('',#28683,#15413,#15414);
#13543=AXIS2_PLACEMENT_3D('',#28693,#15415,#15416);
#13544=AXIS2_PLACEMENT_3D('',#28695,#15417,#15418);
#13545=AXIS2_PLACEMENT_3D('',#28696,#15419,#15420);
#13546=AXIS2_PLACEMENT_3D('',#28697,#15421,#15422);
#13547=AXIS2_PLACEMENT_3D('',#28707,#15423,#15424);
#13548=AXIS2_PLACEMENT_3D('',#28709,#15425,#15426);
#13549=AXIS2_PLACEMENT_3D('',#28710,#15427,#15428);
#13550=AXIS2_PLACEMENT_3D('',#28711,#15429,#15430);
#13551=AXIS2_PLACEMENT_3D('',#28721,#15431,#15432);
#13552=AXIS2_PLACEMENT_3D('',#28723,#15433,#15434);
#13553=AXIS2_PLACEMENT_3D('',#28724,#15435,#15436);
#13554=AXIS2_PLACEMENT_3D('',#28725,#15437,#15438);
#13555=AXIS2_PLACEMENT_3D('',#28735,#15439,#15440);
#13556=AXIS2_PLACEMENT_3D('',#28737,#15441,#15442);
#13557=AXIS2_PLACEMENT_3D('',#28738,#15443,#15444);
#13558=AXIS2_PLACEMENT_3D('',#28739,#15445,#15446);
#13559=AXIS2_PLACEMENT_3D('',#28749,#15447,#15448);
#13560=AXIS2_PLACEMENT_3D('',#28751,#15449,#15450);
#13561=AXIS2_PLACEMENT_3D('',#28752,#15451,#15452);
#13562=AXIS2_PLACEMENT_3D('',#28753,#15453,#15454);
#13563=AXIS2_PLACEMENT_3D('',#28763,#15455,#15456);
#13564=AXIS2_PLACEMENT_3D('',#28765,#15457,#15458);
#13565=AXIS2_PLACEMENT_3D('',#28766,#15459,#15460);
#13566=AXIS2_PLACEMENT_3D('',#28767,#15461,#15462);
#13567=AXIS2_PLACEMENT_3D('',#28777,#15463,#15464);
#13568=AXIS2_PLACEMENT_3D('',#28779,#15465,#15466);
#13569=AXIS2_PLACEMENT_3D('',#28780,#15467,#15468);
#13570=AXIS2_PLACEMENT_3D('',#28781,#15469,#15470);
#13571=AXIS2_PLACEMENT_3D('',#28791,#15471,#15472);
#13572=AXIS2_PLACEMENT_3D('',#28793,#15473,#15474);
#13573=AXIS2_PLACEMENT_3D('',#28794,#15475,#15476);
#13574=AXIS2_PLACEMENT_3D('',#28795,#15477,#15478);
#13575=AXIS2_PLACEMENT_3D('',#28805,#15479,#15480);
#13576=AXIS2_PLACEMENT_3D('',#28807,#15481,#15482);
#13577=AXIS2_PLACEMENT_3D('',#28808,#15483,#15484);
#13578=AXIS2_PLACEMENT_3D('',#28809,#15485,#15486);
#13579=AXIS2_PLACEMENT_3D('',#28819,#15487,#15488);
#13580=AXIS2_PLACEMENT_3D('',#28821,#15489,#15490);
#13581=AXIS2_PLACEMENT_3D('',#28822,#15491,#15492);
#13582=AXIS2_PLACEMENT_3D('',#28823,#15493,#15494);
#13583=AXIS2_PLACEMENT_3D('',#28833,#15495,#15496);
#13584=AXIS2_PLACEMENT_3D('',#28835,#15497,#15498);
#13585=AXIS2_PLACEMENT_3D('',#28836,#15499,#15500);
#13586=AXIS2_PLACEMENT_3D('',#28837,#15501,#15502);
#13587=AXIS2_PLACEMENT_3D('',#28866,#15503,#15504);
#13588=AXIS2_PLACEMENT_3D('',#28895,#15505,#15506);
#13589=AXIS2_PLACEMENT_3D('',#28924,#15507,#15508);
#13590=AXIS2_PLACEMENT_3D('',#28953,#15509,#15510);
#13591=AXIS2_PLACEMENT_3D('',#28982,#15511,#15512);
#13592=AXIS2_PLACEMENT_3D('',#29011,#15513,#15514);
#13593=AXIS2_PLACEMENT_3D('',#29040,#15515,#15516);
#13594=AXIS2_PLACEMENT_3D('',#29069,#15517,#15518);
#13595=AXIS2_PLACEMENT_3D('',#29098,#15519,#15520);
#13596=AXIS2_PLACEMENT_3D('',#29127,#15521,#15522);
#13597=AXIS2_PLACEMENT_3D('',#29156,#15523,#15524);
#13598=AXIS2_PLACEMENT_3D('',#29185,#15525,#15526);
#13599=AXIS2_PLACEMENT_3D('',#29214,#15527,#15528);
#13600=AXIS2_PLACEMENT_3D('',#29243,#15529,#15530);
#13601=AXIS2_PLACEMENT_3D('',#29272,#15531,#15532);
#13602=AXIS2_PLACEMENT_3D('',#29301,#15533,#15534);
#13603=AXIS2_PLACEMENT_3D('',#29330,#15535,#15536);
#13604=AXIS2_PLACEMENT_3D('',#29823,#15537,#15538);
#13605=AXIS2_PLACEMENT_3D('',#29824,#15539,#15540);
#13606=AXIS2_PLACEMENT_3D('',#29849,#15541,#15542);
#13607=AXIS2_PLACEMENT_3D('',#29850,#15543,#15544);
#13608=AXIS2_PLACEMENT_3D('',#29911,#15545,#15546);
#13609=AXIS2_PLACEMENT_3D('',#29912,#15547,#15548);
#13610=AXIS2_PLACEMENT_3D('',#29937,#15549,#15550);
#13611=AXIS2_PLACEMENT_3D('',#29938,#15551,#15552);
#13612=AXIS2_PLACEMENT_3D('',#30003,#15553,#15554);
#13613=AXIS2_PLACEMENT_3D('',#30004,#15555,#15556);
#13614=AXIS2_PLACEMENT_3D('',#30033,#15557,#15558);
#13615=AXIS2_PLACEMENT_3D('',#30034,#15559,#15560);
#13616=AXIS2_PLACEMENT_3D('',#30095,#15561,#15562);
#13617=AXIS2_PLACEMENT_3D('',#30096,#15563,#15564);
#13618=AXIS2_PLACEMENT_3D('',#30125,#15565,#15566);
#13619=AXIS2_PLACEMENT_3D('',#30126,#15567,#15568);
#13620=AXIS2_PLACEMENT_3D('',#30187,#15569,#15570);
#13621=AXIS2_PLACEMENT_3D('',#30188,#15571,#15572);
#13622=AXIS2_PLACEMENT_3D('',#30217,#15573,#15574);
#13623=AXIS2_PLACEMENT_3D('',#30218,#15575,#15576);
#13624=AXIS2_PLACEMENT_3D('',#30283,#15577,#15578);
#13625=AXIS2_PLACEMENT_3D('',#30284,#15579,#15580);
#13626=AXIS2_PLACEMENT_3D('',#30313,#15581,#15582);
#13627=AXIS2_PLACEMENT_3D('',#30314,#15583,#15584);
#13628=AXIS2_PLACEMENT_3D('',#30375,#15585,#15586);
#13629=AXIS2_PLACEMENT_3D('',#30376,#15587,#15588);
#13630=AXIS2_PLACEMENT_3D('',#30405,#15589,#15590);
#13631=AXIS2_PLACEMENT_3D('',#30406,#15591,#15592);
#13632=AXIS2_PLACEMENT_3D('',#30471,#15593,#15594);
#13633=AXIS2_PLACEMENT_3D('',#30472,#15595,#15596);
#13634=AXIS2_PLACEMENT_3D('',#30501,#15597,#15598);
#13635=AXIS2_PLACEMENT_3D('',#30502,#15599,#15600);
#13636=AXIS2_PLACEMENT_3D('',#30563,#15601,#15602);
#13637=AXIS2_PLACEMENT_3D('',#30564,#15603,#15604);
#13638=AXIS2_PLACEMENT_3D('',#30593,#15605,#15606);
#13639=AXIS2_PLACEMENT_3D('',#30594,#15607,#15608);
#13640=AXIS2_PLACEMENT_3D('',#30655,#15609,#15610);
#13641=AXIS2_PLACEMENT_3D('',#30656,#15611,#15612);
#13642=AXIS2_PLACEMENT_3D('',#30685,#15613,#15614);
#13643=AXIS2_PLACEMENT_3D('',#30686,#15615,#15616);
#13644=AXIS2_PLACEMENT_3D('',#30747,#15617,#15618);
#13645=AXIS2_PLACEMENT_3D('',#30748,#15619,#15620);
#13646=AXIS2_PLACEMENT_3D('',#30777,#15621,#15622);
#13647=AXIS2_PLACEMENT_3D('',#30778,#15623,#15624);
#13648=AXIS2_PLACEMENT_3D('',#30843,#15625,#15626);
#13649=AXIS2_PLACEMENT_3D('',#30844,#15627,#15628);
#13650=AXIS2_PLACEMENT_3D('',#30873,#15629,#15630);
#13651=AXIS2_PLACEMENT_3D('',#30874,#15631,#15632);
#13652=AXIS2_PLACEMENT_3D('',#30935,#15633,#15634);
#13653=AXIS2_PLACEMENT_3D('',#30936,#15635,#15636);
#13654=AXIS2_PLACEMENT_3D('',#30965,#15637,#15638);
#13655=AXIS2_PLACEMENT_3D('',#30966,#15639,#15640);
#13656=AXIS2_PLACEMENT_3D('',#31027,#15641,#15642);
#13657=AXIS2_PLACEMENT_3D('',#31028,#15643,#15644);
#13658=AXIS2_PLACEMENT_3D('',#31057,#15645,#15646);
#13659=AXIS2_PLACEMENT_3D('',#31058,#15647,#15648);
#13660=AXIS2_PLACEMENT_3D('',#31123,#15649,#15650);
#13661=AXIS2_PLACEMENT_3D('',#31124,#15651,#15652);
#13662=AXIS2_PLACEMENT_3D('',#31153,#15653,#15654);
#13663=AXIS2_PLACEMENT_3D('',#31154,#15655,#15656);
#13664=AXIS2_PLACEMENT_3D('',#31215,#15657,#15658);
#13665=AXIS2_PLACEMENT_3D('',#31216,#15659,#15660);
#13666=AXIS2_PLACEMENT_3D('',#31245,#15661,#15662);
#13667=AXIS2_PLACEMENT_3D('',#31246,#15663,#15664);
#13668=AXIS2_PLACEMENT_3D('',#31311,#15665,#15666);
#13669=AXIS2_PLACEMENT_3D('',#31312,#15667,#15668);
#13670=AXIS2_PLACEMENT_3D('',#31341,#15669,#15670);
#13671=AXIS2_PLACEMENT_3D('',#31342,#15671,#15672);
#13672=AXIS2_PLACEMENT_3D('',#31403,#15673,#15674);
#13673=AXIS2_PLACEMENT_3D('',#31404,#15675,#15676);
#13674=AXIS2_PLACEMENT_3D('',#31429,#15677,#15678);
#13675=AXIS2_PLACEMENT_3D('',#31430,#15679,#15680);
#13676=AXIS2_PLACEMENT_3D('',#31545,#15683,#15684);
#13677=AXIS2_PLACEMENT_3D('',#31547,#15685,#15686);
#13678=AXIS2_PLACEMENT_3D('',#31561,#15687,#15688);
#13679=AXIS2_PLACEMENT_3D('',#31576,#15689,#15690);
#13680=AXIS2_PLACEMENT_3D('',#31727,#15695,#15696);
#13681=AXIS2_PLACEMENT_3D('',#31728,#15697,#15698);
#13682=AXIS2_PLACEMENT_3D('',#31730,#15699,#15700);
#13683=AXIS2_PLACEMENT_3D('',#31735,#15703,#15704);
#13684=AXIS2_PLACEMENT_3D('',#31740,#15707,#15708);
#13685=AXIS2_PLACEMENT_3D('',#31745,#15711,#15712);
#13686=AXIS2_PLACEMENT_3D('',#31750,#15715,#15716);
#13687=AXIS2_PLACEMENT_3D('',#31755,#15719,#15720);
#13688=AXIS2_PLACEMENT_3D('',#31760,#15723,#15724);
#13689=AXIS2_PLACEMENT_3D('',#31765,#15727,#15728);
#13690=AXIS2_PLACEMENT_3D('',#31770,#15731,#15732);
#13691=AXIS2_PLACEMENT_3D('',#31775,#15735,#15736);
#13692=AXIS2_PLACEMENT_3D('',#31780,#15739,#15740);
#13693=AXIS2_PLACEMENT_3D('',#31785,#15743,#15744);
#13694=AXIS2_PLACEMENT_3D('',#31790,#15747,#15748);
#13695=AXIS2_PLACEMENT_3D('',#31795,#15751,#15752);
#13696=AXIS2_PLACEMENT_3D('',#31800,#15755,#15756);
#13697=AXIS2_PLACEMENT_3D('',#31803,#15759,#15760);
#13698=AXIS2_PLACEMENT_3D('',#31882,#15761,#15762);
#13699=AXIS2_PLACEMENT_3D('',#31883,#15763,#15764);
#13700=AXIS2_PLACEMENT_3D('',#32040,#15765,#15766);
#13701=AXIS2_PLACEMENT_3D('',#32119,#15767,#15768);
#13702=AXIS2_PLACEMENT_3D('',#32120,#15769,#15770);
#13703=AXIS2_PLACEMENT_3D('',#32277,#15771,#15772);
#13704=AXIS2_PLACEMENT_3D('',#32356,#15773,#15774);
#13705=AXIS2_PLACEMENT_3D('',#32357,#15775,#15776);
#13706=AXIS2_PLACEMENT_3D('',#32514,#15777,#15778);
#13707=AXIS2_PLACEMENT_3D('',#32593,#15779,#15780);
#13708=AXIS2_PLACEMENT_3D('',#32594,#15781,#15782);
#13709=AXIS2_PLACEMENT_3D('',#32751,#15783,#15784);
#13710=AXIS2_PLACEMENT_3D('',#32830,#15785,#15786);
#13711=AXIS2_PLACEMENT_3D('',#32831,#15787,#15788);
#13712=AXIS2_PLACEMENT_3D('',#32975,#15789,#15790);
#14381=DIRECTION('axis',(0.,0.,1.));
#14382=DIRECTION('refdir',(1.,0.,0.));
#14383=DIRECTION('center_axis',(0.,0.,1.));
#14384=DIRECTION('ref_axis',(-0.608812046626718,0.793314497461244,0.));
#14385=DIRECTION('',(0.,0.,1.));
#14386=DIRECTION('center_axis',(0.,0.,-1.));
#14387=DIRECTION('ref_axis',(1.,6.43162402581532E-14,0.));
#14388=DIRECTION('center_axis',(0.,0.,1.));
#14389=DIRECTION('ref_axis',(-0.608812046626718,0.793314497461244,0.));
#14390=DIRECTION('',(0.,0.,1.));
#14391=DIRECTION('center_axis',(0.,0.,1.));
#14392=DIRECTION('ref_axis',(-0.608812046626718,0.793314497461244,0.));
#14393=DIRECTION('',(0.,0.,1.));
#14394=DIRECTION('center_axis',(0.,0.,1.));
#14395=DIRECTION('ref_axis',(-0.608812046626718,0.793314497461244,0.));
#14396=DIRECTION('',(0.,0.,1.));
#14397=DIRECTION('center_axis',(0.,0.,1.));
#14398=DIRECTION('ref_axis',(-0.608812046626718,0.793314497461244,0.));
#14399=DIRECTION('',(0.,0.,1.));
#14400=DIRECTION('center_axis',(0.,0.,1.));
#14401=DIRECTION('ref_axis',(-0.608812046626718,0.793314497461244,0.));
#14402=DIRECTION('',(0.,0.,1.));
#14403=DIRECTION('center_axis',(0.,0.,1.));
#14404=DIRECTION('ref_axis',(-0.608812046626718,0.793314497461244,0.));
#14405=DIRECTION('',(0.,0.,1.));
#14406=DIRECTION('center_axis',(0.,0.,1.));
#14407=DIRECTION('ref_axis',(-0.608812046626718,0.793314497461244,0.));
#14408=DIRECTION('',(0.,0.,1.));
#14409=DIRECTION('center_axis',(0.,0.,1.));
#14410=DIRECTION('ref_axis',(-0.608812046626718,0.793314497461244,0.));
#14411=DIRECTION('',(0.,0.,1.));
#14412=DIRECTION('center_axis',(0.,0.,1.));
#14413=DIRECTION('ref_axis',(-0.608812046626718,0.793314497461244,0.));
#14414=DIRECTION('',(0.,0.,1.));
#14415=DIRECTION('center_axis',(0.,0.,1.));
#14416=DIRECTION('ref_axis',(-0.608812046626718,0.793314497461244,0.));
#14417=DIRECTION('',(0.,0.,1.));
#14418=DIRECTION('center_axis',(0.,0.,1.));
#14419=DIRECTION('ref_axis',(-0.608812046626718,0.793314497461244,0.));
#14420=DIRECTION('',(0.,0.,1.));
#14421=DIRECTION('center_axis',(0.,0.,1.));
#14422=DIRECTION('ref_axis',(1.,6.43162402581532E-14,0.));
#14423=DIRECTION('center_axis',(0.,0.,1.));
#14424=DIRECTION('ref_axis',(0.93738942346349,0.348283029702549,0.));
#14425=DIRECTION('',(0.,0.,1.));
#14426=DIRECTION('center_axis',(0.,0.,-1.));
#14427=DIRECTION('ref_axis',(1.,0.,0.));
#14428=DIRECTION('center_axis',(0.,0.,1.));
#14429=DIRECTION('ref_axis',(0.93738942346349,0.348283029702549,0.));
#14430=DIRECTION('',(0.,0.,1.));
#14431=DIRECTION('center_axis',(0.,0.,1.));
#14432=DIRECTION('ref_axis',(0.93738942346349,0.348283029702549,0.));
#14433=DIRECTION('',(0.,0.,1.));
#14434=DIRECTION('center_axis',(0.,0.,1.));
#14435=DIRECTION('ref_axis',(0.93738942346349,0.348283029702549,0.));
#14436=DIRECTION('',(0.,0.,1.));
#14437=DIRECTION('center_axis',(0.,0.,1.));
#14438=DIRECTION('ref_axis',(0.93738942346349,0.348283029702549,0.));
#14439=DIRECTION('',(0.,0.,1.));
#14440=DIRECTION('center_axis',(0.,0.,1.));
#14441=DIRECTION('ref_axis',(0.93738942346349,0.348283029702549,0.));
#14442=DIRECTION('',(0.,0.,1.));
#14443=DIRECTION('center_axis',(0.,0.,1.));
#14444=DIRECTION('ref_axis',(0.93738942346349,0.348283029702549,0.));
#14445=DIRECTION('',(0.,0.,1.));
#14446=DIRECTION('center_axis',(0.,0.,1.));
#14447=DIRECTION('ref_axis',(0.93738942346349,0.348283029702549,0.));
#14448=DIRECTION('',(0.,0.,1.));
#14449=DIRECTION('center_axis',(0.,0.,1.));
#14450=DIRECTION('ref_axis',(0.93738942346349,0.348283029702549,0.));
#14451=DIRECTION('',(0.,0.,1.));
#14452=DIRECTION('center_axis',(0.,0.,1.));
#14453=DIRECTION('ref_axis',(0.93738942346349,0.348283029702549,0.));
#14454=DIRECTION('',(0.,0.,1.));
#14455=DIRECTION('center_axis',(0.,0.,1.));
#14456=DIRECTION('ref_axis',(0.93738942346349,0.348283029702549,0.));
#14457=DIRECTION('',(0.,0.,1.));
#14458=DIRECTION('center_axis',(0.,0.,1.));
#14459=DIRECTION('ref_axis',(0.93738942346349,0.348283029702549,0.));
#14460=DIRECTION('',(0.,0.,1.));
#14461=DIRECTION('center_axis',(0.,0.,-1.));
#14462=DIRECTION('ref_axis',(1.,0.,0.));
#14463=DIRECTION('center_axis',(0.,0.,1.));
#14464=DIRECTION('ref_axis',(0.93738942346349,0.348283029702549,0.));
#14465=DIRECTION('center_axis',(0.,0.,1.));
#14466=DIRECTION('ref_axis',(-0.608812046626718,0.793314497461244,0.));
#14467=DIRECTION('center_axis',(0.,0.,1.));
#14468=DIRECTION('ref_axis',(1.,0.,0.));
#14469=DIRECTION('center_axis',(0.,0.,1.));
#14470=DIRECTION('ref_axis',(0.,-1.,0.));
#14471=DIRECTION('',(-0.990431813260487,0.138002982871906,0.));
#14472=DIRECTION('center_axis',(0.,0.,1.));
#14473=DIRECTION('ref_axis',(1.,0.,0.));
#14474=DIRECTION('',(0.999687555793007,0.0249958155018767,0.));
#14475=DIRECTION('center_axis',(0.,0.,1.));
#14476=DIRECTION('ref_axis',(0.,-1.,0.));
#14477=DIRECTION('',(-0.977901266293703,-0.209067246074493,0.));
#14478=DIRECTION('center_axis',(0.,0.,1.));
#14479=DIRECTION('ref_axis',(1.,0.,0.));
#14480=DIRECTION('',(0.930849946869696,0.365401664490851,0.));
#14481=DIRECTION('center_axis',(0.,0.,1.));
#14482=DIRECTION('ref_axis',(0.,-1.,0.));
#14483=DIRECTION('',(-0.847421394326308,-0.530920879640325,0.));
#14484=DIRECTION('center_axis',(0.,0.,1.));
#14485=DIRECTION('ref_axis',(1.,0.,0.));
#14486=DIRECTION('',(0.749738096471781,0.661734679988038,0.));
#14487=DIRECTION('center_axis',(0.,0.,1.));
#14488=DIRECTION('ref_axis',(0.,-1.,0.));
#14489=DIRECTION('',(-0.614729995595327,-0.788737619563926,0.));
#14490=DIRECTION('center_axis',(0.,0.,1.));
#14491=DIRECTION('ref_axis',(1.,0.,0.));
#14492=DIRECTION('',(0.478196766683598,0.87825272691484,0.));
#14493=DIRECTION('center_axis',(0.,0.,1.));
#14494=DIRECTION('ref_axis',(0.,-1.,0.));
#14495=DIRECTION('',(-0.307893086947081,-0.951420962040567,0.));
#14496=DIRECTION('center_axis',(0.,0.,1.));
#14497=DIRECTION('ref_axis',(1.,0.,0.));
#14498=DIRECTION('',(0.148977849400632,0.98884053334598,0.));
#14499=DIRECTION('center_axis',(0.,0.,1.));
#14500=DIRECTION('ref_axis',(0.,-1.,0.));
#14501=DIRECTION('',(0.0360802720049828,-0.999348895017174,0.));
#14502=DIRECTION('center_axis',(0.,0.,1.));
#14503=DIRECTION('ref_axis',(1.,0.,0.));
#14504=DIRECTION('',(-0.198209995198882,0.980159577723576,0.));
#14505=DIRECTION('center_axis',(0.,0.,1.));
#14506=DIRECTION('ref_axis',(0.,-1.,0.));
#14507=DIRECTION('',(0.375701817665145,-0.92674060243582,0.));
#14508=DIRECTION('center_axis',(0.,0.,1.));
#14509=DIRECTION('ref_axis',(1.,0.,0.));
#14510=DIRECTION('',(-0.521490789109412,0.853256911412994,0.));
#14511=DIRECTION('center_axis',(0.,0.,1.));
#14512=DIRECTION('ref_axis',(0.,-1.,0.));
#14513=DIRECTION('',(0.670008179346718,-0.742353715965978,0.));
#14514=DIRECTION('center_axis',(0.,0.,1.));
#14515=DIRECTION('ref_axis',(1.,0.,0.));
#14516=DIRECTION('',(-0.781872097469079,0.623438868855081,0.));
#14517=DIRECTION('center_axis',(0.,0.,1.));
#14518=DIRECTION('ref_axis',(0.,-1.,0.));
#14519=DIRECTION('',(0.883501666331281,-0.468428015376802,0.));
#14520=DIRECTION('center_axis',(0.,0.,1.));
#14521=DIRECTION('ref_axis',(1.,0.,0.));
#14522=DIRECTION('',(-0.947948091670679,0.318424897735586,0.));
#14523=DIRECTION('center_axis',(0.,0.,1.));
#14524=DIRECTION('ref_axis',(0.,-1.,0.));
#14525=DIRECTION('',(0.990431813260487,-0.138002982871907,0.));
#14526=DIRECTION('center_axis',(0.,0.,1.));
#14527=DIRECTION('ref_axis',(1.,0.,0.));
#14528=DIRECTION('',(-0.999687555793007,-0.0249958155018767,0.));
#14529=DIRECTION('center_axis',(0.,0.,1.));
#14530=DIRECTION('ref_axis',(0.,-1.,0.));
#14531=DIRECTION('',(0.977901266293703,0.209067246074493,0.));
#14532=DIRECTION('center_axis',(0.,0.,1.));
#14533=DIRECTION('ref_axis',(1.,0.,0.));
#14534=DIRECTION('',(-0.930849946869696,-0.365401664490851,0.));
#14535=DIRECTION('center_axis',(0.,0.,1.));
#14536=DIRECTION('ref_axis',(0.,-1.,0.));
#14537=DIRECTION('',(0.847421394326308,0.530920879640325,0.));
#14538=DIRECTION('center_axis',(0.,0.,1.));
#14539=DIRECTION('ref_axis',(1.,0.,0.));
#14540=DIRECTION('',(-0.749738096471781,-0.661734679988038,0.));
#14541=DIRECTION('center_axis',(0.,0.,1.));
#14542=DIRECTION('ref_axis',(0.,-1.,0.));
#14543=DIRECTION('',(0.614729995595327,0.788737619563926,0.));
#14544=DIRECTION('center_axis',(0.,0.,1.));
#14545=DIRECTION('ref_axis',(1.,0.,0.));
#14546=DIRECTION('',(-0.478196766683598,-0.87825272691484,0.));
#14547=DIRECTION('center_axis',(0.,0.,1.));
#14548=DIRECTION('ref_axis',(0.,-1.,0.));
#14549=DIRECTION('',(0.307893086947081,0.951420962040567,0.));
#14550=DIRECTION('center_axis',(0.,0.,1.));
#14551=DIRECTION('ref_axis',(1.,0.,0.));
#14552=DIRECTION('',(-0.148977849400632,-0.98884053334598,0.));
#14553=DIRECTION('center_axis',(0.,0.,1.));
#14554=DIRECTION('ref_axis',(0.,-1.,0.));
#14555=DIRECTION('',(-0.0360802720049828,0.999348895017174,0.));
#14556=DIRECTION('center_axis',(0.,0.,1.));
#14557=DIRECTION('ref_axis',(1.,0.,0.));
#14558=DIRECTION('',(0.198209995198882,-0.980159577723576,0.));
#14559=DIRECTION('center_axis',(0.,0.,1.));
#14560=DIRECTION('ref_axis',(0.,-1.,0.));
#14561=DIRECTION('',(-0.375701817665128,0.926740602435827,0.));
#14562=DIRECTION('center_axis',(0.,0.,1.));
#14563=DIRECTION('ref_axis',(1.,0.,0.));
#14564=DIRECTION('',(0.521490789109416,-0.853256911412992,0.));
#14565=DIRECTION('center_axis',(0.,0.,1.));
#14566=DIRECTION('ref_axis',(0.,-1.,0.));
#14567=DIRECTION('',(-0.670008179346718,0.742353715965978,0.));
#14568=DIRECTION('center_axis',(0.,0.,1.));
#14569=DIRECTION('ref_axis',(1.,0.,0.));
#14570=DIRECTION('',(0.781872097469079,-0.623438868855081,0.));
#14571=DIRECTION('center_axis',(0.,0.,1.));
#14572=DIRECTION('ref_axis',(0.,-1.,0.));
#14573=DIRECTION('',(-0.883501666331281,0.468428015376802,0.));
#14574=DIRECTION('center_axis',(0.,0.,1.));
#14575=DIRECTION('ref_axis',(1.,0.,0.));
#14576=DIRECTION('',(0.947948091670678,-0.318424897735588,0.));
#14577=DIRECTION('center_axis',(0.,0.,-1.));
#14578=DIRECTION('ref_axis',(-1.,0.,0.));
#14579=DIRECTION('',(0.474277008002355,-0.880375669632194,0.));
#14580=DIRECTION('center_axis',(0.,0.,1.));
#14581=DIRECTION('ref_axis',(1.,0.,0.));
#14582=DIRECTION('',(-0.990722494271237,0.13590047588209,0.));
#14583=DIRECTION('center_axis',(0.,0.,-1.));
#14584=DIRECTION('ref_axis',(0.796664686286605,-0.60442152313089,0.));
#14585=DIRECTION('center_axis',(0.,0.,-1.));
#14586=DIRECTION('ref_axis',(-1.,0.,0.));
#14587=DIRECTION('',(0.144555196347935,-0.98949673835178,0.));
#14588=DIRECTION('center_axis',(0.,0.,1.));
#14589=DIRECTION('ref_axis',(1.,0.,0.));
#14590=DIRECTION('',(-0.884491140557834,0.466556987167379,0.));
#14591=DIRECTION('center_axis',(0.,0.,-1.));
#14592=DIRECTION('ref_axis',(0.541895590973931,-0.840445815316499,0.));
#14593=DIRECTION('center_axis',(0.,0.,-1.));
#14594=DIRECTION('ref_axis',(-1.,0.,0.));
#14595=DIRECTION('',(-0.202590371288481,-0.979263570986481,0.));
#14596=DIRECTION('center_axis',(0.,0.,1.));
#14597=DIRECTION('ref_axis',(1.,0.,0.));
#14598=DIRECTION('',(-0.671582337664226,0.74092993173272,0.));
#14599=DIRECTION('center_axis',(0.,0.,-1.));
#14600=DIRECTION('ref_axis',(0.221765889862626,-0.975099938515759,0.));
#14601=DIRECTION('center_axis',(0.,0.,-1.));
#14602=DIRECTION('ref_axis',(-1.,0.,0.));
#14603=DIRECTION('',(-0.525300549059025,-0.850916760416838,-1.44557603741106E-12));
#14604=DIRECTION('center_axis',(0.,0.,1.));
#14605=DIRECTION('ref_axis',(1.,0.,0.));
#14606=DIRECTION('',(-0.377668004938845,0.92594107698358,0.));
#14607=DIRECTION('center_axis',(0.,0.,-1.));
#14608=DIRECTION('ref_axis',(-0.125112050482103,-0.992142618187609,0.));
#14609=DIRECTION('center_axis',(0.,0.,-1.));
#14610=DIRECTION('ref_axis',(-1.,0.,0.));
#14611=DIRECTION('',(-0.78465171542998,-0.619936839906123,0.));
#14612=DIRECTION('center_axis',(0.,0.,1.));
#14613=DIRECTION('ref_axis',(1.,0.,0.));
#14614=DIRECTION('',(-0.0381953670132134,0.999270290731555,0.));
#14615=DIRECTION('center_axis',(0.,0.,-1.));
#14616=DIRECTION('ref_axis',(-0.456899631081401,-0.889518255640479,0.));
#14617=DIRECTION('center_axis',(0.,0.,-1.));
#14618=DIRECTION('ref_axis',(-1.,0.,0.));
#14619=DIRECTION('',(-0.949362313354307,-0.314183382728237,0.));
#14620=DIRECTION('center_axis',(0.,0.,1.));
#14621=DIRECTION('ref_axis',(1.,0.,0.));
#14622=DIRECTION('',(0.305872997935251,0.952072323478685,0.));
#14623=DIRECTION('center_axis',(0.,0.,-1.));
#14624=DIRECTION('ref_axis',(-0.733578373052014,-0.679604863571738,0.));
#14625=DIRECTION('center_axis',(0.,0.,-1.));
#14626=DIRECTION('ref_axis',(-1.,0.,0.));
#14627=DIRECTION('',(-0.999565805862472,0.0294652295173026,-1.4455760374657E-12));
#14628=DIRECTION('center_axis',(0.,0.,1.));
#14629=DIRECTION('ref_axis',(1.,0.,0.));
#14630=DIRECTION('',(0.613059210435848,0.790036964008504,0.));
#14631=DIRECTION('center_axis',(0.,0.,-1.));
#14632=DIRECTION('ref_axis',(-0.921776736768698,-0.387721095056807,0.));
#14633=DIRECTION('center_axis',(0.,0.,-1.));
#14634=DIRECTION('ref_axis',(-1.,0.,0.));
#14635=DIRECTION('',(-0.929206905711275,0.36955990905194,0.));
#14636=DIRECTION('center_axis',(0.,0.,1.));
#14637=DIRECTION('ref_axis',(1.,0.,0.));
#14638=DIRECTION('',(0.846292579865157,0.532718377067262,0.));
#14639=DIRECTION('center_axis',(0.,0.,-1.));
#14640=DIRECTION('ref_axis',(-0.998795222055377,-0.049072440323971,0.));
#14641=DIRECTION('center_axis',(0.,0.,-1.));
#14642=DIRECTION('ref_axis',(-1.,0.,0.));
#14643=DIRECTION('',(-0.746771944067323,0.66508019332552,0.));
#14644=DIRECTION('center_axis',(0.,0.,1.));
#14645=DIRECTION('ref_axis',(1.,0.,0.));
#14646=DIRECTION('',(0.977455315104272,0.211142385546837,0.));
#14647=DIRECTION('center_axis',(0.,0.,-1.));
#14648=DIRECTION('ref_axis',(-0.955344262914612,0.295495074943961,0.));
#14649=DIRECTION('center_axis',(0.,0.,-1.));
#14650=DIRECTION('ref_axis',(-1.,0.,0.));
#14651=DIRECTION('',(-0.474265266635988,0.880381994853765,0.));
#14652=DIRECTION('center_axis',(0.,0.,1.));
#14653=DIRECTION('ref_axis',(1.,0.,0.));
#14654=DIRECTION('',(0.990722494271013,-0.135900475883722,0.));
#14655=DIRECTION('center_axis',(0.,0.,-1.));
#14656=DIRECTION('ref_axis',(-0.796664686286608,0.604421523130886,0.));
#14657=DIRECTION('center_axis',(0.,0.,-1.));
#14658=DIRECTION('ref_axis',(-1.,0.,0.));
#14659=DIRECTION('',(-0.144555196349004,0.989496738351623,0.));
#14660=DIRECTION('center_axis',(0.,0.,1.));
#14661=DIRECTION('ref_axis',(1.,0.,0.));
#14662=DIRECTION('',(0.884491140558253,-0.466556987166584,0.));
#14663=DIRECTION('center_axis',(0.,0.,-1.));
#14664=DIRECTION('ref_axis',(-0.541895590973931,0.840445815316499,0.));
#14665=DIRECTION('center_axis',(0.,0.,-1.));
#14666=DIRECTION('ref_axis',(-1.,0.,0.));
#14667=DIRECTION('',(0.202590371280164,0.979263570988202,0.));
#14668=DIRECTION('center_axis',(0.,0.,1.));
#14669=DIRECTION('ref_axis',(1.,0.,0.));
#14670=DIRECTION('',(0.671582337664788,-0.740929931732211,1.44548415250913E-12));
#14671=DIRECTION('center_axis',(0.,0.,-1.));
#14672=DIRECTION('ref_axis',(-0.221765889862635,0.975099938515757,0.));
#14673=DIRECTION('center_axis',(0.,0.,-1.));
#14674=DIRECTION('ref_axis',(-1.,0.,0.));
#14675=DIRECTION('',(0.525300549057258,0.850916760417929,0.));
#14676=DIRECTION('center_axis',(0.,0.,1.));
#14677=DIRECTION('ref_axis',(1.,0.,0.));
#14678=DIRECTION('',(0.377668004939932,-0.925941076983137,0.));
#14679=DIRECTION('center_axis',(0.,0.,-1.));
#14680=DIRECTION('ref_axis',(0.125112050482093,0.99214261818761,0.));
#14681=DIRECTION('center_axis',(0.,0.,-1.));
#14682=DIRECTION('ref_axis',(-1.,0.,0.));
#14683=DIRECTION('',(0.784651716122117,0.619936839030088,1.4455738977615E-12));
#14684=DIRECTION('center_axis',(0.,0.,1.));
#14685=DIRECTION('ref_axis',(1.,0.,0.));
#14686=DIRECTION('',(0.0381953670132134,-0.999270290731555,0.));
#14687=DIRECTION('center_axis',(0.,0.,-1.));
#14688=DIRECTION('ref_axis',(0.456899631081495,0.88951825564043,0.));
#14689=DIRECTION('center_axis',(0.,0.,-1.));
#14690=DIRECTION('ref_axis',(-1.,0.,0.));
#14691=DIRECTION('',(0.949362313026162,0.314183383719787,-1.44557603741564E-12));
#14692=DIRECTION('center_axis',(0.,0.,1.));
#14693=DIRECTION('ref_axis',(1.,0.,0.));
#14694=DIRECTION('',(-0.305872997971906,-0.952072323466909,1.44548415256294E-12));
#14695=DIRECTION('center_axis',(0.,0.,-1.));
#14696=DIRECTION('ref_axis',(0.733578373052045,0.679604863571704,0.));
#14697=DIRECTION('center_axis',(0.,0.,-1.));
#14698=DIRECTION('ref_axis',(-1.,0.,0.));
#14699=DIRECTION('',(0.999565805862573,-0.0294652295138758,0.));
#14700=DIRECTION('center_axis',(0.,0.,1.));
#14701=DIRECTION('ref_axis',(1.,0.,0.));
#14702=DIRECTION('',(-0.613059210433514,-0.790036964010315,0.));
#14703=DIRECTION('center_axis',(0.,0.,-1.));
#14704=DIRECTION('ref_axis',(0.921776736768698,0.387721095056807,0.));
#14705=DIRECTION('center_axis',(0.,0.,-1.));
#14706=DIRECTION('ref_axis',(-1.,0.,0.));
#14707=DIRECTION('',(0.92921182631369,-0.36954753664282,0.));
#14708=DIRECTION('center_axis',(0.,0.,1.));
#14709=DIRECTION('ref_axis',(1.,0.,0.));
#14710=DIRECTION('',(-0.846292579863551,-0.532718377069813,0.));
#14711=DIRECTION('center_axis',(0.,0.,-1.));
#14712=DIRECTION('ref_axis',(0.998795222055378,0.0490724403239548,0.));
#14713=DIRECTION('center_axis',(0.,0.,-1.));
#14714=DIRECTION('ref_axis',(-1.,0.,0.));
#14715=DIRECTION('',(0.746780806816249,-0.665070241832298,-1.44557391839046E-12));
#14716=DIRECTION('center_axis',(0.,0.,1.));
#14717=DIRECTION('ref_axis',(1.,0.,0.));
#14718=DIRECTION('',(-0.977456573143307,-0.211136561540019,0.));
#14719=DIRECTION('center_axis',(0.,0.,-1.));
#14720=DIRECTION('ref_axis',(0.955344262914614,-0.295495074943952,0.));
#14721=DIRECTION('center_axis',(0.,0.,-1.));
#14722=DIRECTION('ref_axis',(0.,-1.,0.));
#14723=DIRECTION('center_axis',(-0.619032382875318,-0.33848017230615,-0.708681932821279));
#14724=DIRECTION('ref_axis',(-0.451228736779563,0.891841105362626,-0.0318130459071304));
#14725=DIRECTION('center_axis',(0.67086774319136,0.218417923344258,0.708681932821286));
#14726=DIRECTION('ref_axis',(-0.287922260464996,0.957389170141623,-0.0225110822543487));
#14727=DIRECTION('',(-0.685495936603333,-0.181409993675129,0.705113987306385));
#14728=DIRECTION('',(0.645329675210074,0.295341295811932,-0.70450204348986));
#14729=DIRECTION('center_axis',(0.,0.,-1.));
#14730=DIRECTION('ref_axis',(0.,-1.,0.));
#14731=DIRECTION('center_axis',(-0.465933125170307,-0.529788864512786,-0.708681932821265));
#14732=DIRECTION('ref_axis',(-0.729043936918215,0.683727188396728,-0.0318130459072231));
#14733=DIRECTION('center_axis',(0.555706138352604,0.43469599249356,0.708681932821259));
#14734=DIRECTION('ref_axis',(-0.598004804709664,0.8011763256112,-0.0225110822550398));
#14735=DIRECTION('',(-0.582109601172995,-0.404923050876555,0.7051139873035));
#14736=DIRECTION('',(0.505398861452357,0.498245784270093,-0.704502043502885));
#14737=DIRECTION('center_axis',(0.,0.,-1.));
#14738=DIRECTION('ref_axis',(0.,-1.,0.));
#14739=DIRECTION('center_axis',(-0.256635456129185,-0.657197200808165,-0.70868193282126));
#14740=DIRECTION('ref_axis',(-0.918925678721932,0.393145681771461,-0.0318130459071376));
#14741=DIRECTION('center_axis',(0.37351817187998,0.598543309517481,0.708681932821276));
#14742=DIRECTION('ref_axis',(-0.83595914389466,0.548329792109296,-0.0225110822547992));
#14743=DIRECTION('',(-0.408512256818674,-0.579596412148449,0.705113987276922));
#14744=DIRECTION('',(0.304509486091619,0.641054477849826,-0.704502043509389));
#14745=DIRECTION('center_axis',(0.,0.,-1.));
#14746=DIRECTION('ref_axis',(0.0617633245521631,0.998090823392473,0.));
#14747=DIRECTION('center_axis',(-0.0163837635432463,-0.705337855488318,
-0.708681932821276));
#14748=DIRECTION('ref_axis',(-0.997971421773015,0.0551450037126303,-0.0318130459070098));
#14749=DIRECTION('center_axis',(0.146278401337234,0.6901974698555,0.708681932821269));
#14750=DIRECTION('ref_axis',(-0.973084472883285,0.229346593192864,-0.022511082254869));
#14751=DIRECTION('',(-0.185642305292501,-0.684361892155193,0.705113987275426));
#14752=DIRECTION('',(0.0668917726419952,0.70654254045347,-0.704502043490556));
#14753=DIRECTION('center_axis',(0.,0.,-1.));
#14754=DIRECTION('ref_axis',(0.,-1.,0.));
#14755=DIRECTION('center_axis',(0.225844052724809,-0.668404355118618,-0.708681932821275));
#14756=DIRECTION('ref_axis',(-0.95664708286883,-0.289506975647697,-0.0318130459070163));
#14757=DIRECTION('center_axis',(-0.0986047032458038,0.69860362909915,0.708681932821279));
#14758=DIRECTION('ref_axis',(-0.992841453244872,-0.117299189657614,-0.0225110822546955));
#14759=DIRECTION('',(0.0596188480477669,-0.706583227868191,0.705113987276402));
#14760=DIRECTION('',(-0.1787940758072,0.686811145215674,-0.704502043477365));
#14761=DIRECTION('center_axis',(0.,0.,-1.));
#14762=DIRECTION('ref_axis',(0.,-1.,0.));
#14763=DIRECTION('center_axis',(0.440831743130997,-0.550851424923984,-0.708681932821279));
#14764=DIRECTION('ref_axis',(-0.799936987163271,-0.599240141077255,-0.0318130459066631));
#14765=DIRECTION('center_axis',(-0.331594625366901,0.622747880382156,0.708681932821288));
#14766=DIRECTION('ref_axis',(-0.892847101565944,-0.449796959083795,-0.0225110822543812));
#14767=DIRECTION('',(0.297689088430308,-0.643580198230555,0.705113987292163));
#14768=DIRECTION('',(-0.402914719960345,0.584240189604372,-0.704502043496202));
#14769=DIRECTION('center_axis',(0.,0.,-1.));
#14770=DIRECTION('ref_axis',(0.,-1.,0.));
#14771=DIRECTION('center_axis',(0.60264861933197,-0.366857683182414,-0.708681932821278));
#14772=DIRECTION('ref_axis',(-0.546742684993606,-0.836696101649882,-0.0318130459068674));
#14773=DIRECTION('center_axis',(-0.524589341853953,0.471779546510804,0.708681932821274));
#14774=DIRECTION('ref_axis',(-0.685162212418179,-0.728042576948589,-0.0225110822548518));
#14775=DIRECTION('',(0.499853631303652,-0.502951898509268,0.705113987280408));
#14776=DIRECTION('',(-0.578437902573191,0.411201244629492,-0.704502043490212));
#14777=DIRECTION('center_axis',(0.,0.,-1.));
#14778=DIRECTION('ref_axis',(0.,-1.,0.));
#14779=DIRECTION('center_axis',(0.691777177895169,-0.138615490606495,-0.708681932821288));
#14780=DIRECTION('ref_axis',(-0.227603145951143,-0.973234164044439,-0.0318130459067542));
#14781=DIRECTION('center_axis',(-0.654310841598713,0.263907636606227,0.708681932821276));
#14782=DIRECTION('ref_axis',(-0.394836648535736,-0.918475515269075,-0.0225110822546137));
#14783=DIRECTION('',(0.641728449228522,-0.301660176976957,0.705113987293535));
#14784=DIRECTION('',(-0.684192937232473,0.188565360909515,-0.704502043507516));
#14785=DIRECTION('center_axis',(0.,0.,-1.));
#14786=DIRECTION('ref_axis',(0.,-1.,0.));
#14787=DIRECTION('center_axis',(0.697467199260489,0.106345775884312,-0.708681932821271));
#14788=DIRECTION('ref_axis',(0.118988691558466,-0.992385822848809,-0.0318130459072569));
#14789=DIRECTION('center_axis',(-0.705112797247349,0.0242045708643797,0.70868193282127));
#14790=DIRECTION('ref_axis',(-0.0568879576711038,-0.998126751193317,-0.0225110822548537));
#14791=DIRECTION('',(0.706201345226432,-0.0639837860996167,0.705113987321721));
#14792=DIRECTION('',(-0.707424206095769,-0.056814288281615,-0.704502043486621));
#14793=DIRECTION('center_axis',(0.,0.,-1.));
#14794=DIRECTION('ref_axis',(0.,-1.,0.));
#14795=DIRECTION('center_axis',(0.61903238287525,0.338480172306288,-0.708681932821273));
#14796=DIRECTION('ref_axis',(0.451228736779656,-0.891841105362575,-0.0318130459072342));
#14797=DIRECTION('center_axis',(-0.670867743191319,-0.218417923344399,0.708681932821281));
#14798=DIRECTION('ref_axis',(0.287922260465025,-0.957389170141609,-0.0225110822545478));
#14799=DIRECTION('',(0.685495936588057,0.181409993663856,0.705113987324136));
#14800=DIRECTION('',(-0.645329675209038,-0.295341295816895,-0.704502043488729));
#14801=DIRECTION('center_axis',(0.,0.,-1.));
#14802=DIRECTION('ref_axis',(0.,-1.,0.));
#14803=DIRECTION('center_axis',(0.465933125169797,0.529788864513252,-0.708681932821252));
#14804=DIRECTION('ref_axis',(0.729043936918548,-0.683727188396351,-0.031813045907688));
#14805=DIRECTION('center_axis',(-0.55570613835297,-0.434695992493057,0.70868193282128));
#14806=DIRECTION('ref_axis',(0.598004804709207,-0.80117632561155,-0.0225110822547272));
#14807=DIRECTION('',(0.58210960117426,0.404923050894126,0.705113987292365));
#14808=DIRECTION('',(-0.505398861452357,-0.498245784270093,-0.704502043502885));
#14809=DIRECTION('center_axis',(0.,0.,-1.));
#14810=DIRECTION('ref_axis',(0.,-1.,0.));
#14811=DIRECTION('center_axis',(0.256635456129172,0.657197200808164,-0.708681932821267));
#14812=DIRECTION('ref_axis',(0.918925678721868,-0.393145681771596,-0.0318130459073145));
#14813=DIRECTION('center_axis',(-0.373518171879956,-0.598543309517493,0.708681932821278));
#14814=DIRECTION('ref_axis',(0.835959143894646,-0.548329792109316,-0.0225110822548671));
#14815=DIRECTION('',(0.408512256819533,0.579596412136736,0.705113987286052));
#14816=DIRECTION('',(-0.304509486097168,-0.641054477848632,-0.704502043508077));
#14817=DIRECTION('center_axis',(0.,0.,-1.));
#14818=DIRECTION('ref_axis',(0.,-1.,0.));
#14819=DIRECTION('center_axis',(0.0163837635434838,0.705337855488308,-0.708681932821281));
#14820=DIRECTION('ref_axis',(0.997971421773012,-0.0551450037127905,-0.0318130459068232));
#14821=DIRECTION('center_axis',(-0.146278401337369,-0.690197469855462,0.708681932821278));
#14822=DIRECTION('ref_axis',(0.973084472883258,-0.229346593192995,-0.0225110822547478));
#14823=DIRECTION('',(0.185642305292172,0.684361892155236,0.705113987275471));
#14824=DIRECTION('',(-0.0668917726414032,-0.706542540453498,-0.704502043490584));
#14825=DIRECTION('center_axis',(0.,0.,-1.));
#14826=DIRECTION('ref_axis',(0.,-1.,0.));
#14827=DIRECTION('center_axis',(-0.225844052724565,0.668404355118693,-0.708681932821282));
#14828=DIRECTION('ref_axis',(0.956647082868877,0.289506975647566,-0.0318130459067811));
#14829=DIRECTION('center_axis',(0.0986047032463636,-0.698603629099088,0.708681932821262));
#14830=DIRECTION('ref_axis',(0.992841453244803,0.117299189658157,-0.0225110822549345));
#14831=DIRECTION('',(-0.0596188480500861,0.706583227852509,0.70511398729192));
#14832=DIRECTION('',(0.178794075800621,-0.686811145216509,-0.704502043478221));
#14833=DIRECTION('center_axis',(0.,0.,-1.));
#14834=DIRECTION('ref_axis',(0.,-1.,0.));
#14835=DIRECTION('center_axis',(-0.440831743131266,0.550851424923786,-0.708681932821265));
#14836=DIRECTION('ref_axis',(0.799936987163221,0.599240141077298,-0.031813045907131));
#14837=DIRECTION('center_axis',(0.331594625366664,-0.622747880382285,0.708681932821286));
#14838=DIRECTION('ref_axis',(0.892847101566032,0.449796959083631,-0.0225110822541639));
#14839=DIRECTION('',(-0.297689088430928,0.643580198230424,0.70511398729202));
#14840=DIRECTION('',(0.402914719960345,-0.584240189604372,-0.704502043496202));
#14841=DIRECTION('center_axis',(0.,0.,-1.));
#14842=DIRECTION('ref_axis',(0.,-1.,0.));
#14843=DIRECTION('center_axis',(-0.602648619332025,0.366857683182321,-0.70868193282128));
#14844=DIRECTION('ref_axis',(0.546742684993566,0.836696101649904,-0.0318130459069726));
#14845=DIRECTION('center_axis',(0.524589341854173,-0.471779546510578,0.708681932821261));
#14846=DIRECTION('ref_axis',(0.685162212417927,0.728042576948822,-0.022511082254977));
#14847=DIRECTION('',(-0.499853631345304,0.502951898491402,0.705113987263625));
#14848=DIRECTION('',(0.578437902573191,-0.411201244629492,-0.704502043490212));
#14849=DIRECTION('center_axis',(0.,0.,-1.));
#14850=DIRECTION('ref_axis',(0.,-1.,0.));
#14851=DIRECTION('center_axis',(-0.697467199260449,-0.106345775884652,-0.70868193282126));
#14852=DIRECTION('ref_axis',(-0.118988691558859,0.992385822848759,-0.0318130459073474));
#14853=DIRECTION('center_axis',(0.705112797247378,-0.0242045708638981,0.708681932821257));
#14854=DIRECTION('ref_axis',(0.0568879576706311,0.998126751193339,-0.0225110822550593));
#14855=DIRECTION('',(-0.706201345257537,0.0639837861036678,0.7051139872902));
#14856=DIRECTION('',(0.707424206095769,0.056814288281615,-0.704502043486621));
#14857=DIRECTION('center_axis',(0.,0.,-1.));
#14858=DIRECTION('ref_axis',(0.,-1.,0.));
#14859=DIRECTION('center_axis',(-0.691777177895279,0.138615490606009,-0.708681932821276));
#14860=DIRECTION('ref_axis',(0.227603145950679,0.97323416404454,-0.0318130459069853));
#14861=DIRECTION('center_axis',(0.654310841598881,-0.263907636605812,0.708681932821276));
#14862=DIRECTION('ref_axis',(0.394836648535391,0.918475515269218,-0.0225110822548663));
#14863=DIRECTION('',(-0.641728449232441,0.3016601769701,0.705113987292902));
#14864=DIRECTION('',(0.684192937233218,-0.188565360903944,-0.704502043508283));
#14865=DIRECTION('center_axis',(0.,0.,1.));
#14866=DIRECTION('ref_axis',(0.,-1.,0.));
#14867=DIRECTION('center_axis',(-0.703660934063436,0.0512953015946455,0.708681932821268));
#14868=DIRECTION('ref_axis',(-0.040760194859215,-0.998662373690501,0.031813045907198));
#14869=DIRECTION('center_axis',(0.,0.,-1.));
#14870=DIRECTION('ref_axis',(0.,-1.,0.));
#14871=DIRECTION('center_axis',(0.701040101070486,0.0794524687080656,-0.70868193282126));
#14872=DIRECTION('ref_axis',(0.135024713403112,-0.990586481810706,0.0225110822551012));
#14873=DIRECTION('',(-0.699004252188757,-0.119194464416953,-0.705113987291694));
#14874=DIRECTION('center_axis',(0.,0.,1.));
#14875=DIRECTION('ref_axis',(1.,0.,0.));
#14876=DIRECTION('',(0.709701051035535,-0.00113528531252956,0.704502043493358));
#14877=DIRECTION('center_axis',(0.,0.,1.));
#14878=DIRECTION('ref_axis',(0.,-1.,0.));
#14879=DIRECTION('center_axis',(-0.678769013677884,-0.19246439713213,0.708681932821289));
#14880=DIRECTION('ref_axis',(0.303260593853006,-0.952376470901111,0.0318130459067882));
#14881=DIRECTION('center_axis',(0.,0.,-1.));
#14882=DIRECTION('ref_axis',(0.,-1.,0.));
#14883=DIRECTION('center_axis',(0.631587865115614,0.314430734393761,-0.708681932821277));
#14884=DIRECTION('ref_axis',(0.465682257294193,-0.884665635377067,0.0225110822546476));
#14885=DIRECTION('',(-0.616082229859789,-0.351079693163982,-0.705113987309055));
#14886=DIRECTION('center_axis',(0.,0.,1.));
#14887=DIRECTION('ref_axis',(1.,0.,0.));
#14888=DIRECTION('',(0.66728913109891,0.241665235964873,0.704502043462831));
#14889=DIRECTION('center_axis',(0.,0.,1.));
#14890=DIRECTION('ref_axis',(0.,-1.,0.));
#14891=DIRECTION('center_axis',(-0.572007532679314,-0.413010049091819,0.708681932821274));
#14892=DIRECTION('ref_axis',(0.610703679296142,-0.791219910141464,0.0318130459071324));
#14893=DIRECTION('center_axis',(0.,0.,-1.));
#14894=DIRECTION('ref_axis',(0.,-1.,0.));
#14895=DIRECTION('center_axis',(0.485956811383988,0.511484013007474,-0.708681932821261));
#14896=DIRECTION('ref_axis',(0.740171648217135,-0.672041057042826,0.0225110822550047));
#14897=DIRECTION('',(-0.458851598246782,-0.540619529544785,-0.705113987282304));
#14898=DIRECTION('center_axis',(0.,0.,1.));
#14899=DIRECTION('ref_axis',(1.,0.,0.));
#14900=DIRECTION('',(0.544392293801187,0.455317363180238,0.704502043457986));
#14901=DIRECTION('center_axis',(0.,0.,1.));
#14902=DIRECTION('ref_axis',(0.,-1.,0.));
#14903=DIRECTION('center_axis',(-0.396253501306999,-0.583740593752603,0.708681932821279));
#14904=DIRECTION('ref_axis',(0.844486887990209,-0.534630551056288,0.0318130459067074));
#14905=DIRECTION('center_axis',(0.,0.,-1.));
#14906=DIRECTION('ref_axis',(0.,-1.,0.));
#14907=DIRECTION('center_axis',(0.281712194240451,0.646844770952772,-0.708681932821267));
#14908=DIRECTION('ref_axis',(0.925385414595141,-0.378358408959404,0.0225110822549279));
#14909=DIRECTION('',(-0.24627669192658,-0.664952671929248,-0.705113987315423));
#14910=DIRECTION('center_axis',(0.,0.,1.));
#14911=DIRECTION('ref_axis',(1.,0.,0.));
#14912=DIRECTION('',(0.355833711437326,0.614051496670459,0.704502043461555));
#14913=DIRECTION('center_axis',(0.,0.,1.));
#14914=DIRECTION('ref_axis',(0.,-1.,0.));
#14915=DIRECTION('center_axis',(-0.172705449598815,-0.684063407712745,0.708681932821276));
#14916=DIRECTION('ref_axis',(0.976412514693378,-0.21355685720732,0.0318130459070931));
#14917=DIRECTION('center_axis',(0.,0.,-1.));
#14918=DIRECTION('ref_axis',(0.,-1.,0.));
#14919=DIRECTION('center_axis',(0.0434889288417849,0.704186503109001,-0.708681932821284));
#14920=DIRECTION('ref_axis',(0.998984042738759,-0.0390401527796353,0.0225110822545011));
#14921=DIRECTION('',(-0.0039971818986142,-0.70908270844906,-0.705113987320784));
#14922=DIRECTION('center_axis',(0.,0.,1.));
#14923=DIRECTION('ref_axis',(1.,0.,0.));
#14924=DIRECTION('',(0.124356331985472,0.698721957173194,0.704502043474098));
#14925=DIRECTION('center_axis',(0.,0.,1.));
#14926=DIRECTION('ref_axis',(0.,-1.,0.));
#14927=DIRECTION('center_axis',(0.0716734281918473,-0.701878079002291,0.708681932821264));
#14928=DIRECTION('ref_axis',(0.990568381810636,0.133274945384173,0.0318130459073441));
#14929=DIRECTION('center_axis',(0.,0.,-1.));
#14930=DIRECTION('ref_axis',(0.,-1.,0.));
#14931=DIRECTION('center_axis',(-0.199979743202182,0.676592950304318,-0.708681932821268));
#14932=DIRECTION('ref_axis',(0.952090451893775,0.304986921995709,0.022511082254978));
#14933=DIRECTION('',(0.238764447245934,-0.667686905404276,-0.705113987297802));
#14934=DIRECTION('center_axis',(0.,0.,1.));
#14935=DIRECTION('ref_axis',(1.,0.,0.));
#14936=DIRECTION('',(-0.122120256424646,0.699116237642577,0.704502043457126));
#14937=DIRECTION('center_axis',(0.,0.,1.));
#14938=DIRECTION('ref_axis',(0.,-1.,0.));
#14939=DIRECTION('center_axis',(0.307407432756173,-0.635035895346844,0.708681932821271));
#14940=DIRECTION('ref_axis',(0.885247082849198,0.464031822634076,0.0318130459070229));
#14941=DIRECTION('center_axis',(0.,0.,-1.));
#14942=DIRECTION('ref_axis',(0.,-1.,0.));
#14943=DIRECTION('center_axis',(-0.419327906830114,0.567392302244386,-0.70868193282127));
#14944=DIRECTION('ref_axis',(0.790360701191827,0.612228072851353,0.0225110822547893));
#14945=DIRECTION('',(0.452727560264035,-0.545758207516331,-0.705113987314063));
#14946=DIRECTION('center_axis',(0.,0.,1.));
#14947=DIRECTION('ref_axis',(1.,0.,0.));
#14948=DIRECTION('',(-0.35386733960517,0.615186781972065,0.704502043465889));
#14949=DIRECTION('center_axis',(0.,0.,1.));
#14950=DIRECTION('ref_axis',(0.,-1.,0.));
#14951=DIRECTION('center_axis',(0.5060635640791,-0.49159901058105,0.70868193282127));
#14952=DIRECTION('ref_axis',(0.673151920840624,0.738819613693819,0.0318130459072238));
#14953=DIRECTION('center_axis',(0.,0.,-1.));
#14954=DIRECTION('ref_axis',(0.,-1.,0.));
#14955=DIRECTION('center_axis',(-0.588098936273544,0.389755768714997,-0.708681932821282));
#14956=DIRECTION('ref_axis',(0.533301785444319,0.845625482597132,0.0225110822545249));
#14957=DIRECTION('',(0.612085047945861,-0.358003015318079,-0.705113987312885));
#14958=DIRECTION('center_axis',(0.,0.,1.));
#14959=DIRECTION('ref_axis',(1.,0.,0.));
#14960=DIRECTION('',(-0.542932799114604,0.45705672118749,0.704502043476754));
#14961=DIRECTION('center_axis',(0.,0.,1.));
#14962=DIRECTION('ref_axis',(0.,-1.,0.));
#14963=DIRECTION('center_axis',(0.643680960871656,-0.288868029909898,0.708681932821287));
#14964=DIRECTION('ref_axis',(0.379864702514146,0.924494855525966,0.0318130459067162));
#14965=DIRECTION('center_axis',(0.,0.,-1.));
#14966=DIRECTION('ref_axis',(0.,-1.,0.));
#14967=DIRECTION('center_axis',(-0.685936554586207,0.165108937296249,-0.708681932821281));
#14968=DIRECTION('ref_axis',(0.211918803676205,0.97702797903856,0.0225110822545819));
#14969=DIRECTION('',(0.697616045442606,-0.12706737586408,-0.705113987332571));
#14970=DIRECTION('center_axis',(0.,0.,1.));
#14971=DIRECTION('ref_axis',(1.,0.,0.));
#14972=DIRECTION('',(-0.666512550211308,0.243798874435375,0.70450204345684));
#14973=DIRECTION('center_axis',(0.,0.,1.));
#14974=DIRECTION('ref_axis',(0.,-1.,0.));
#14975=DIRECTION('center_axis',(0.703660934063412,-0.0512953015951689,0.708681932821253));
#14976=DIRECTION('ref_axis',(0.0407601948595917,0.998662373690474,0.031813045907557));
#14977=DIRECTION('center_axis',(0.,0.,-1.));
#14978=DIRECTION('ref_axis',(0.,-1.,0.));
#14979=DIRECTION('center_axis',(-0.701040101070454,-0.0794524687082925,
-0.708681932821266));
#14980=DIRECTION('ref_axis',(-0.135024713403322,0.99058648181068,0.0225110822549792));
#14981=DIRECTION('',(0.699004252188757,0.119194464416953,-0.705113987291694));
#14982=DIRECTION('center_axis',(0.,0.,1.));
#14983=DIRECTION('ref_axis',(1.,0.,0.));
#14984=DIRECTION('',(-0.709701051066567,0.00113528531247919,0.704502043462096));
#14985=DIRECTION('center_axis',(0.,0.,1.));
#14986=DIRECTION('ref_axis',(0.,-1.,0.));
#14987=DIRECTION('center_axis',(0.678769013677966,0.192464397131867,0.708681932821283));
#14988=DIRECTION('ref_axis',(-0.303260593852791,0.952376470901174,0.0318130459069519));
#14989=DIRECTION('center_axis',(0.,0.,-1.));
#14990=DIRECTION('ref_axis',(0.,-1.,0.));
#14991=DIRECTION('center_axis',(-0.631587865115661,-0.314430734393692,-0.708681932821265));
#14992=DIRECTION('ref_axis',(-0.465682257294258,0.884665635377028,0.0225110822548306));
#14993=DIRECTION('',(0.616082229859789,0.351079693163982,-0.705113987309055));
#14994=DIRECTION('center_axis',(0.,0.,1.));
#14995=DIRECTION('ref_axis',(1.,0.,0.));
#14996=DIRECTION('',(-0.667289131086675,-0.241665235966725,0.704502043473784));
#14997=DIRECTION('center_axis',(0.,0.,1.));
#14998=DIRECTION('ref_axis',(0.,-1.,0.));
#14999=DIRECTION('center_axis',(0.572007532679451,0.413010049091652,0.708681932821261));
#15000=DIRECTION('ref_axis',(-0.61070367929613,0.79121991014146,0.0318130459074592));
#15001=DIRECTION('center_axis',(0.,0.,-1.));
#15002=DIRECTION('ref_axis',(0.,-1.,0.));
#15003=DIRECTION('center_axis',(-0.485956811383784,-0.511484013007649,-0.708681932821274));
#15004=DIRECTION('ref_axis',(-0.740171648217328,0.672041057042616,0.0225110822549303));
#15005=DIRECTION('',(0.458851598226975,0.540619529521448,-0.705113987313086));
#15006=DIRECTION('center_axis',(0.,0.,1.));
#15007=DIRECTION('ref_axis',(1.,0.,0.));
#15008=DIRECTION('',(-0.544392293794381,-0.455317363180406,0.704502043463136));
#15009=DIRECTION('center_axis',(0.,0.,1.));
#15010=DIRECTION('ref_axis',(0.,-1.,0.));
#15011=DIRECTION('center_axis',(0.396253501307373,0.583740593752364,0.708681932821266));
#15012=DIRECTION('ref_axis',(-0.844486887990119,0.534630551056402,0.0318130459071614));
#15013=DIRECTION('center_axis',(0.,0.,-1.));
#15014=DIRECTION('ref_axis',(0.,-1.,0.));
#15015=DIRECTION('center_axis',(-0.281712194240633,-0.646844770952699,-0.708681932821261));
#15016=DIRECTION('ref_axis',(-0.925385414595083,0.378358408959537,0.0225110822550412));
#15017=DIRECTION('',(0.246276691905924,0.664952671934695,-0.705113987317501));
#15018=DIRECTION('center_axis',(0.,0.,1.));
#15019=DIRECTION('ref_axis',(1.,0.,0.));
#15020=DIRECTION('',(-0.355833711481152,-0.614051496661014,0.704502043447652));
#15021=DIRECTION('center_axis',(0.,0.,1.));
#15022=DIRECTION('ref_axis',(0.,-1.,0.));
#15023=DIRECTION('center_axis',(0.172705449598441,0.68406340771283,0.708681932821284));
#15024=DIRECTION('ref_axis',(-0.976412514693421,0.21355685720718,0.0318130459067133));
#15025=DIRECTION('center_axis',(0.,0.,-1.));
#15026=DIRECTION('ref_axis',(0.,-1.,0.));
#15027=DIRECTION('center_axis',(-0.0434889288422669,-0.704186503108984,
-0.708681932821272));
#15028=DIRECTION('ref_axis',(-0.998984042738736,0.0390401527801138,0.0225110822546889));
#15029=DIRECTION('',(0.00399718189249243,0.709082708449077,-0.705113987320802));
#15030=DIRECTION('center_axis',(0.,0.,1.));
#15031=DIRECTION('ref_axis',(1.,0.,0.));
#15032=DIRECTION('',(-0.124356331985472,-0.698721957173194,0.704502043474098));
#15033=DIRECTION('center_axis',(0.,0.,1.));
#15034=DIRECTION('ref_axis',(0.,-1.,0.));
#15035=DIRECTION('center_axis',(-0.071673428192519,0.701878079002203,0.708681932821282));
#15036=DIRECTION('ref_axis',(-0.990568381810588,-0.13327494538465,0.0318130459068612));
#15037=DIRECTION('center_axis',(0.,0.,-1.));
#15038=DIRECTION('ref_axis',(0.,-1.,0.));
#15039=DIRECTION('center_axis',(0.199979743201945,-0.676592950304395,-0.708681932821262));
#15040=DIRECTION('ref_axis',(-0.952090451893826,-0.304986921995541,0.0225110822550975));
#15041=DIRECTION('',(-0.23876444723984,0.667686905405306,-0.70511398729889));
#15042=DIRECTION('center_axis',(0.,0.,1.));
#15043=DIRECTION('ref_axis',(1.,0.,0.));
#15044=DIRECTION('',(0.122120256422062,-0.699116237636338,0.704502043463766));
#15045=DIRECTION('center_axis',(0.,0.,1.));
#15046=DIRECTION('ref_axis',(0.,-1.,0.));
#15047=DIRECTION('center_axis',(-0.307407432755953,0.63503589534695,0.708681932821271));
#15048=DIRECTION('ref_axis',(-0.885247082849227,-0.464031822634005,0.0318130459072588));
#15049=DIRECTION('center_axis',(0.,0.,-1.));
#15050=DIRECTION('ref_axis',(0.,-1.,0.));
#15051=DIRECTION('center_axis',(0.419327906830362,-0.567392302244193,-0.708681932821278));
#15052=DIRECTION('ref_axis',(-0.790360701191684,-0.612228072851546,0.0225110822545551));
#15053=DIRECTION('',(-0.452727560269443,0.54575820751465,-0.705113987311891));
#15054=DIRECTION('center_axis',(0.,0.,1.));
#15055=DIRECTION('ref_axis',(1.,0.,0.));
#15056=DIRECTION('',(0.35386733960517,-0.615186781972065,0.704502043465889));
#15057=DIRECTION('center_axis',(0.,0.,1.));
#15058=DIRECTION('ref_axis',(0.,-1.,0.));
#15059=DIRECTION('center_axis',(-0.506063564078916,0.491599010581241,0.708681932821269));
#15060=DIRECTION('ref_axis',(-0.673151920840782,-0.73881961369367,0.0318130459073368));
#15061=DIRECTION('center_axis',(0.,0.,-1.));
#15062=DIRECTION('ref_axis',(0.,-1.,0.));
#15063=DIRECTION('center_axis',(0.588098936273506,-0.389755768715068,-0.708681932821275));
#15064=DIRECTION('ref_axis',(-0.533301785444285,-0.845625482597149,0.022511082254684));
#15065=DIRECTION('',(-0.612085047945861,0.358003015318079,-0.705113987312885));
#15066=DIRECTION('center_axis',(0.,0.,1.));
#15067=DIRECTION('ref_axis',(1.,0.,0.));
#15068=DIRECTION('',(0.542932799116209,-0.457056721221068,0.704502043453732));
#15069=DIRECTION('center_axis',(0.,0.,1.));
#15070=DIRECTION('ref_axis',(0.,-1.,0.));
#15071=DIRECTION('center_axis',(-0.643680960871258,0.288868029910839,0.708681932821265));
#15072=DIRECTION('ref_axis',(-0.379864702514675,-0.92449485552572,0.0318130459075584));
#15073=DIRECTION('center_axis',(0.,0.,-1.));
#15074=DIRECTION('ref_axis',(0.,-1.,0.));
#15075=DIRECTION('center_axis',(0.685936554586071,-0.165108937296882,-0.708681932821266));
#15076=DIRECTION('ref_axis',(-0.21191880367663,-0.977027979038457,0.022511082255061));
#15077=DIRECTION('',(-0.697616045443148,0.127067375858057,-0.705113987333119));
#15078=DIRECTION('center_axis',(0.,0.,1.));
#15079=DIRECTION('ref_axis',(1.,0.,0.));
#15080=DIRECTION('',(0.666512550199835,-0.243798874428091,0.704502043470215));
#15081=DIRECTION('center_axis',(0.,0.,1.));
#15082=DIRECTION('ref_axis',(1.,0.,0.));
#15083=DIRECTION('',(0.897353006349151,0.44131347361727,0.));
#15084=DIRECTION('',(-0.885480349083443,0.464676824671798,0.));
#15085=DIRECTION('center_axis',(0.,0.,1.));
#15086=DIRECTION('ref_axis',(0.999566449009809,0.0294434035722917,0.));
#15087=DIRECTION('center_axis',(0.,0.,1.));
#15088=DIRECTION('ref_axis',(1.,0.,0.));
#15089=DIRECTION('',(0.69228830556049,0.72162102379586,0.));
#15090=DIRECTION('',(-0.991008984713935,0.133795337049747,0.));
#15091=DIRECTION('center_axis',(0.,0.,1.));
#15092=DIRECTION('ref_axis',(0.929214979009912,0.369539609221539,0.));
#15093=DIRECTION('center_axis',(0.,0.,1.));
#15094=DIRECTION('ref_axis',(1.,0.,0.));
#15095=DIRECTION('',(0.403741491998108,0.914873110130111,0.));
#15096=DIRECTION('',(-0.977004529914168,-0.213218546395934,-1.44547855409531E-12));
#15097=DIRECTION('center_axis',(0.,0.,1.));
#15098=DIRECTION('ref_axis',(0.746786468788826,0.665063884174983,0.));
#15099=DIRECTION('center_axis',(0.,0.,1.));
#15100=DIRECTION('ref_axis',(1.,0.,0.));
#15101=DIRECTION('',(0.0664745597242861,0.997788120248714,0.));
#15102=DIRECTION('',(-0.845158910852611,-0.534515121775268,0.));
#15103=DIRECTION('center_axis',(0.,0.,1.));
#15104=DIRECTION('ref_axis',(0.474284489037475,0.880371639399215,0.));
#15105=DIRECTION('center_axis',(0.,0.,1.));
#15106=DIRECTION('ref_axis',(1.,0.,0.));
#15107=DIRECTION('',(-0.278785196504122,0.960353483989181,0.));
#15108=DIRECTION('',(-0.611374661297878,-0.79134128132109,0.));
#15109=DIRECTION('center_axis',(0.,0.,1.));
#15110=DIRECTION('ref_axis',(0.144576800214518,0.989493582010379,0.));
#15111=DIRECTION('center_axis',(0.,0.,1.));
#15112=DIRECTION('ref_axis',(1.,0.,0.));
#15113=DIRECTION('',(-0.590432628680576,0.807086929016537,0.));
#15114=DIRECTION('',(-0.303849593520484,-0.952720013706774,-1.44547855411804E-12));
#15115=DIRECTION('center_axis',(0.,0.,1.));
#15116=DIRECTION('ref_axis',(-0.202568984440614,0.979267995261102,0.));
#15117=DIRECTION('center_axis',(0.,0.,1.));
#15118=DIRECTION('ref_axis',(1.,0.,0.));
#15119=DIRECTION('',(-0.830872579903455,0.556462717497387,0.));
#15120=DIRECTION('',(0.040324221163864,-0.999186647822882,0.));
#15121=DIRECTION('center_axis',(0.,0.,1.));
#15122=DIRECTION('ref_axis',(-0.525281959972336,0.850928235826983,0.));
#15123=DIRECTION('center_axis',(0.,0.,1.));
#15124=DIRECTION('ref_axis',(1.,0.,0.));
#15125=DIRECTION('',(-0.97108310621034,0.238741703170764,0.));
#15126=DIRECTION('',(0.379634333178067,-0.92513662400342,0.));
#15127=DIRECTION('center_axis',(0.,0.,1.));
#15128=DIRECTION('ref_axis',(-0.784638178795358,0.61995397278887,0.));
#15129=DIRECTION('center_axis',(0.,0.,1.));
#15130=DIRECTION('ref_axis',(1.,0.,0.));
#15131=DIRECTION('',(-0.994174099458657,-0.107786177061661,0.));
#15132=DIRECTION('',(0.673154938045335,-0.739501473551731,1.44547855411289E-12));
#15133=DIRECTION('center_axis',(0.,0.,1.));
#15134=DIRECTION('ref_axis',(-0.949355453229469,0.3142041110862,0.));
#15135=DIRECTION('center_axis',(0.,0.,1.));
#15136=DIRECTION('ref_axis',(1.,0.,0.));
#15137=DIRECTION('',(-0.897353006349151,-0.44131347361727,0.));
#15138=DIRECTION('',(0.885483124695737,-0.464671535473257,0.));
#15139=DIRECTION('center_axis',(0.,0.,1.));
#15140=DIRECTION('ref_axis',(-0.999566449009809,-0.0294434035723091,0.));
#15141=DIRECTION('center_axis',(0.,0.,1.));
#15142=DIRECTION('ref_axis',(1.,0.,0.));
#15143=DIRECTION('',(-0.692288305561494,-0.721621023794897,0.));
#15144=DIRECTION('',(0.9910089847142,-0.133795337047783,0.));
#15145=DIRECTION('center_axis',(0.,0.,1.));
#15146=DIRECTION('ref_axis',(-0.929214979009907,-0.369539609221553,0.));
#15147=DIRECTION('center_axis',(0.,0.,1.));
#15148=DIRECTION('ref_axis',(1.,0.,0.));
#15149=DIRECTION('',(-0.403741491998464,-0.914873110129953,0.));
#15150=DIRECTION('',(0.977004530010046,0.213218545956606,0.));
#15151=DIRECTION('center_axis',(0.,0.,1.));
#15152=DIRECTION('ref_axis',(-0.746786468788919,-0.665063884174879,0.));
#15153=DIRECTION('center_axis',(0.,0.,1.));
#15154=DIRECTION('ref_axis',(1.,0.,0.));
#15155=DIRECTION('',(-0.0664745597243501,-0.99778812024871,1.44557389775539E-12));
#15156=DIRECTION('',(0.845158910606238,0.534515122164824,0.));
#15157=DIRECTION('center_axis',(0.,0.,1.));
#15158=DIRECTION('ref_axis',(-0.474284489037501,-0.880371639399201,0.));
#15159=DIRECTION('center_axis',(0.,0.,1.));
#15160=DIRECTION('ref_axis',(1.,0.,0.));
#15161=DIRECTION('',(0.278785196503829,-0.960353483989266,0.));
#15162=DIRECTION('',(0.611374661295944,0.791341281322585,0.));
#15163=DIRECTION('center_axis',(0.,0.,1.));
#15164=DIRECTION('ref_axis',(-0.144576800214509,-0.989493582010381,0.));
#15165=DIRECTION('center_axis',(0.,0.,1.));
#15166=DIRECTION('ref_axis',(1.,0.,0.));
#15167=DIRECTION('',(0.590432628680576,-0.807086929016537,0.));
#15168=DIRECTION('',(0.303849593506657,0.952720013711184,0.));
#15169=DIRECTION('center_axis',(0.,0.,1.));
#15170=DIRECTION('ref_axis',(0.202568984440597,-0.979267995261106,0.));
#15171=DIRECTION('center_axis',(0.,0.,1.));
#15172=DIRECTION('ref_axis',(1.,0.,0.));
#15173=DIRECTION('',(0.830872579905544,-0.556462717494268,1.44557389777932E-12));
#15174=DIRECTION('',(-0.0403242211638251,0.999186647822883,0.));
#15175=DIRECTION('center_axis',(0.,0.,1.));
#15176=DIRECTION('ref_axis',(0.525281959972335,-0.850928235826983,0.));
#15177=DIRECTION('center_axis',(0.,0.,1.));
#15178=DIRECTION('ref_axis',(1.,0.,0.));
#15179=DIRECTION('',(0.971083106210285,-0.238741703170988,0.));
#15180=DIRECTION('',(-0.37962882645773,0.925138883693863,0.));
#15181=DIRECTION('center_axis',(0.,0.,1.));
#15182=DIRECTION('ref_axis',(0.784638178795358,-0.61995397278887,0.));
#15183=DIRECTION('center_axis',(0.,0.,1.));
#15184=DIRECTION('ref_axis',(1.,0.,0.));
#15185=DIRECTION('',(0.994172662512016,0.107799430025248,0.));
#15186=DIRECTION('',(-0.673150528894382,0.739505487098786,1.44548415247993E-12));
#15187=DIRECTION('center_axis',(0.,0.,1.));
#15188=DIRECTION('ref_axis',(0.949355453229467,-0.314204111086206,0.));
#15189=DIRECTION('center_axis',(0.,0.,-1.));
#15190=DIRECTION('ref_axis',(-1.,0.,0.));
#15191=DIRECTION('center_axis',(0.,0.,-1.));
#15192=DIRECTION('ref_axis',(0.850763965251217,0.525547976335203,0.));
#15193=DIRECTION('center_axis',(0.,0.,-1.));
#15194=DIRECTION('ref_axis',(0.999566449009811,-0.0294434035722236,0.));
#15195=DIRECTION('center_axis',(0.,0.,1.));
#15196=DIRECTION('ref_axis',(1.,0.,0.));
#15197=DIRECTION('center_axis',(0.,0.,-1.));
#15198=DIRECTION('ref_axis',(-1.,0.,0.));
#15199=DIRECTION('center_axis',(0.,0.,-1.));
#15200=DIRECTION('ref_axis',(0.599889878870626,0.800082579005808,0.));
#15201=DIRECTION('center_axis',(0.,0.,-1.));
#15202=DIRECTION('ref_axis',(0.949355453229486,0.314204111086149,0.));
#15203=DIRECTION('center_axis',(0.,0.,-1.));
#15204=DIRECTION('ref_axis',(0.979411716378758,-0.201872954652214,0.));
#15205=DIRECTION('center_axis',(0.,0.,1.));
#15206=DIRECTION('ref_axis',(1.,0.,0.));
#15207=DIRECTION('center_axis',(0.,0.,-1.));
#15208=DIRECTION('ref_axis',(-1.,0.,0.));
#15209=DIRECTION('center_axis',(0.,0.,-1.));
#15210=DIRECTION('ref_axis',(0.314028052635586,0.949413704429161,0.));
#15211=DIRECTION('center_axis',(0.,0.,-1.));
#15212=DIRECTION('ref_axis',(0.784638178795399,0.619953972788819,0.));
#15213=DIRECTION('center_axis',(0.,0.,-1.));
#15214=DIRECTION('ref_axis',(0.989389291469206,0.145288781143156,0.));
#15215=DIRECTION('center_axis',(0.,0.,1.));
#15216=DIRECTION('ref_axis',(1.,0.,0.));
#15217=DIRECTION('center_axis',(0.,0.,-1.));
#15218=DIRECTION('ref_axis',(-1.,0.,0.));
#15219=DIRECTION('center_axis',(-1.32132775915598E-13,-9.56797466456895E-14,
-1.));
#15220=DIRECTION('ref_axis',(-0.0547306874098733,0.998501152656141,-8.8304619656333E-14));
#15221=DIRECTION('center_axis',(0.,0.,-1.));
#15222=DIRECTION('ref_axis',(0.525281959972367,0.850928235826964,0.));
#15223=DIRECTION('center_axis',(0.,0.,1.));
#15224=DIRECTION('ref_axis',(1.,0.,0.));
#15225=DIRECTION('center_axis',(0.,0.,-1.));
#15226=DIRECTION('ref_axis',(-1.,0.,0.));
#15227=DIRECTION('center_axis',(0.,0.,-1.));
#15228=DIRECTION('ref_axis',(-0.36977560838049,0.929121089765397,0.));
#15229=DIRECTION('center_axis',(0.,0.,-1.));
#15230=DIRECTION('ref_axis',(0.20256898444057,0.979267995261112,0.));
#15231=DIRECTION('center_axis',(-5.28974998245161E-12,3.849896247492E-12,
-1.));
#15232=DIRECTION('ref_axis',(0.664558246712093,0.747236466406016,-6.38564105877661E-13));
#15233=DIRECTION('center_axis',(0.,0.,1.));
#15234=DIRECTION('ref_axis',(1.,0.,0.));
#15235=DIRECTION('center_axis',(0.,0.,-1.));
#15236=DIRECTION('ref_axis',(-1.,0.,0.));
#15237=DIRECTION('center_axis',(0.,0.,-1.));
#15238=DIRECTION('ref_axis',(-0.665255506900887,0.746615771691199,0.));
#15239=DIRECTION('center_axis',(0.,0.,-1.));
#15240=DIRECTION('ref_axis',(-0.144576800214448,0.98949358201039,0.));
#15241=DIRECTION('center_axis',(0.,0.,-1.));
#15242=DIRECTION('ref_axis',(0.368892007453974,0.929472262542878,0.));
#15243=DIRECTION('center_axis',(0.,0.,1.));
#15244=DIRECTION('ref_axis',(1.,0.,0.));
#15245=DIRECTION('center_axis',(0.,0.,-1.));
#15246=DIRECTION('ref_axis',(-1.,0.,0.));
#15247=DIRECTION('center_axis',(0.,0.,-1.));
#15248=DIRECTION('ref_axis',(0.892093090490583,-0.451851654748504,0.));
#15249=DIRECTION('center_axis',(0.,0.,-1.));
#15250=DIRECTION('ref_axis',(-0.474284489037421,0.880371639399244,0.));
#15251=DIRECTION('center_axis',(0.,0.,-1.));
#15252=DIRECTION('ref_axis',(0.0287254060179531,0.999587340380571,0.));
#15253=DIRECTION('center_axis',(0.,0.,1.));
#15254=DIRECTION('ref_axis',(1.,0.,0.));
#15255=DIRECTION('center_axis',(0.,0.,-1.));
#15256=DIRECTION('ref_axis',(-1.,0.,0.));
#15257=DIRECTION('center_axis',(0.,0.,-1.));
#15258=DIRECTION('ref_axis',(0.989520239095182,-0.144394239570053,0.));
#15259=DIRECTION('center_axis',(0.,0.,-1.));
#15260=DIRECTION('ref_axis',(-0.746786468788856,0.66506388417495,0.));
#15261=DIRECTION('center_axis',(0.,0.,1.));
#15262=DIRECTION('ref_axis',(1.,0.,0.));
#15263=DIRECTION('center_axis',(0.,0.,-1.));
#15264=DIRECTION('ref_axis',(-1.,0.,0.));
#15265=DIRECTION('center_axis',(-8.27850864256961E-13,6.25380161775213E-12,
-1.));
#15266=DIRECTION('ref_axis',(0.97922431753446,0.202780018614189,4.57494310884885E-13));
#15267=DIRECTION('center_axis',(0.,0.,-1.));
#15268=DIRECTION('ref_axis',(-0.92921497900993,0.369539609221494,0.));
#15269=DIRECTION('center_axis',(-4.70972287661959E-12,-4.54062894276413E-12,
-1.));
#15270=DIRECTION('ref_axis',(-0.620501753965407,0.784205058212362,-6.38392878747627E-13));
#15271=DIRECTION('center_axis',(0.,0.,1.));
#15272=DIRECTION('ref_axis',(1.,0.,0.));
#15273=DIRECTION('center_axis',(0.,0.,-1.));
#15274=DIRECTION('ref_axis',(-1.,0.,0.));
#15275=DIRECTION('center_axis',(0.,0.,-1.));
#15276=DIRECTION('ref_axis',(0.85076379978476,0.52554824419438,0.));
#15277=DIRECTION('center_axis',(0.,0.,-1.));
#15278=DIRECTION('ref_axis',(-0.99956644900981,0.0294434035722665,0.));
#15279=DIRECTION('center_axis',(0.,0.,-1.));
#15280=DIRECTION('ref_axis',(0.851282603118517,-0.524707470527876,0.));
#15281=DIRECTION('center_axis',(0.,0.,1.));
#15282=DIRECTION('ref_axis',(1.,0.,0.));
#15283=DIRECTION('center_axis',(0.,0.,-1.));
#15284=DIRECTION('ref_axis',(-1.,0.,0.));
#15285=DIRECTION('center_axis',(4.82728718843136E-12,-4.41615259808489E-12,
-1.));
#15286=DIRECTION('ref_axis',(0.59988968881684,0.800082721505242,-6.37447579960598E-13));
#15287=DIRECTION('center_axis',(1.42286553678981E-14,5.73968510871457E-15,
-1.));
#15288=DIRECTION('ref_axis',(-0.949355453229486,-0.314204111086149,-1.53187688370636E-14));
#15289=DIRECTION('center_axis',(0.,0.,-1.));
#15290=DIRECTION('ref_axis',(0.979411667303631,-0.201873192746145,0.));
#15291=DIRECTION('center_axis',(0.,0.,1.));
#15292=DIRECTION('ref_axis',(1.,0.,0.));
#15293=DIRECTION('center_axis',(0.,0.,-1.));
#15294=DIRECTION('ref_axis',(-1.,0.,0.));
#15295=DIRECTION('center_axis',(0.,0.,-1.));
#15296=DIRECTION('ref_axis',(0.314028299832077,0.94941362266642,0.));
#15297=DIRECTION('center_axis',(0.,0.,-1.));
#15298=DIRECTION('ref_axis',(-0.784638178795399,-0.619953972788819,0.));
#15299=DIRECTION('center_axis',(0.,0.,1.));
#15300=DIRECTION('ref_axis',(1.,0.,0.));
#15301=DIRECTION('center_axis',(0.,0.,-1.));
#15302=DIRECTION('ref_axis',(-1.,0.,0.));
#15303=DIRECTION('center_axis',(0.,0.,-1.));
#15304=DIRECTION('ref_axis',(-0.0547311918692556,0.99850112500516,0.));
#15305=DIRECTION('center_axis',(0.,0.,-1.));
#15306=DIRECTION('ref_axis',(-0.525281959972365,-0.850928235826965,0.));
#15307=DIRECTION('center_axis',(0.,0.,-1.));
#15308=DIRECTION('ref_axis',(0.88003414096249,0.474910423912145,0.));
#15309=DIRECTION('center_axis',(0.,0.,1.));
#15310=DIRECTION('ref_axis',(1.,0.,0.));
#15311=DIRECTION('center_axis',(0.,0.,-1.));
#15312=DIRECTION('ref_axis',(-1.,0.,0.));
#15313=DIRECTION('center_axis',(-6.01566800664695E-12,-1.90143638812626E-12,
-1.));
#15314=DIRECTION('ref_axis',(-0.369775977307563,0.929120942938128,4.57785146442974E-13));
#15315=DIRECTION('center_axis',(0.,0.,-1.));
#15316=DIRECTION('ref_axis',(-0.202568984440568,-0.979267995261112,0.));
#15317=DIRECTION('center_axis',(-3.47775045046998E-12,2.39197982760852E-12,
-1.));
#15318=DIRECTION('ref_axis',(0.664558447941313,0.747236287441819,-5.23794315673617E-13));
#15319=DIRECTION('center_axis',(0.,0.,1.));
#15320=DIRECTION('ref_axis',(1.,0.,0.));
#15321=DIRECTION('center_axis',(0.,0.,-1.));
#15322=DIRECTION('ref_axis',(-1.,0.,0.));
#15323=DIRECTION('center_axis',(0.,0.,-1.));
#15324=DIRECTION('ref_axis',(-0.665255256778492,0.746615994557164,0.));
#15325=DIRECTION('center_axis',(0.,0.,-1.));
#15326=DIRECTION('ref_axis',(0.144576800214612,-0.989493582010366,0.));
#15327=DIRECTION('center_axis',(0.,0.,-1.));
#15328=DIRECTION('ref_axis',(0.368891975145543,0.929472275365554,0.));
#15329=DIRECTION('center_axis',(0.,0.,1.));
#15330=DIRECTION('ref_axis',(1.,0.,0.));
#15331=DIRECTION('center_axis',(0.,0.,-1.));
#15332=DIRECTION('ref_axis',(-1.,0.,0.));
#15333=DIRECTION('center_axis',(0.,0.,-1.));
#15334=DIRECTION('ref_axis',(0.892092990260699,-0.451851852632834,0.));
#15335=DIRECTION('center_axis',(0.,0.,-1.));
#15336=DIRECTION('ref_axis',(0.47428448903741,-0.88037163939925,0.));
#15337=DIRECTION('center_axis',(-6.52620372287673E-12,-4.50951246938111E-13,
-1.));
#15338=DIRECTION('ref_axis',(0.0287256757183184,0.999587332630084,-6.38234765888116E-13));
#15339=DIRECTION('center_axis',(0.,0.,1.));
#15340=DIRECTION('ref_axis',(1.,0.,0.));
#15341=DIRECTION('center_axis',(0.,0.,-1.));
#15342=DIRECTION('ref_axis',(-1.,0.,0.));
#15343=DIRECTION('center_axis',(0.,0.,-1.));
#15344=DIRECTION('ref_axis',(0.989520246610118,-0.144394188070888,0.));
#15345=DIRECTION('center_axis',(0.,0.,-1.));
#15346=DIRECTION('ref_axis',(0.746786468788917,-0.665063884174881,0.));
#15347=DIRECTION('center_axis',(0.,0.,1.));
#15348=DIRECTION('ref_axis',(1.,0.,0.));
#15349=DIRECTION('center_axis',(0.,0.,-1.));
#15350=DIRECTION('ref_axis',(-1.,0.,0.));
#15351=DIRECTION('center_axis',(0.,0.,-1.));
#15352=DIRECTION('ref_axis',(0.973825526449741,0.22729681923618,0.));
#15353=DIRECTION('center_axis',(0.,0.,-1.));
#15354=DIRECTION('ref_axis',(0.92921497900996,-0.369539609221419,0.));
#15355=DIRECTION('center_axis',(0.,0.,1.));
#15356=DIRECTION('ref_axis',(1.,0.,0.));
#15357=DIRECTION('center_axis',(0.,0.,1.));
#15358=DIRECTION('ref_axis',(1.,0.,0.));
#15359=DIRECTION('center_axis',(0.,0.,1.));
#15360=DIRECTION('ref_axis',(1.,0.,0.));
#15361=DIRECTION('center_axis',(0.,0.,1.));
#15362=DIRECTION('ref_axis',(0.889388506695126,-0.457152145525549,0.));
#15363=DIRECTION('center_axis',(0.,0.,1.));
#15364=DIRECTION('ref_axis',(0.99417501641652,0.107777719094496,0.));
#15365=DIRECTION('center_axis',(0.,0.,1.));
#15366=DIRECTION('ref_axis',(1.,0.,0.));
#15367=DIRECTION('center_axis',(0.,0.,1.));
#15368=DIRECTION('ref_axis',(1.,0.,0.));
#15369=DIRECTION('center_axis',(0.,0.,1.));
#15370=DIRECTION('ref_axis',(0.988657810802218,-0.150185662231007,0.));
#15371=DIRECTION('center_axis',(0.,0.,1.));
#15372=DIRECTION('ref_axis',(0.897356775764319,0.441305808923773,0.));
#15373=DIRECTION('center_axis',(0.,0.,1.));
#15374=DIRECTION('ref_axis',(1.,0.,0.));
#15375=DIRECTION('center_axis',(0.,0.,1.));
#15376=DIRECTION('ref_axis',(1.,0.,0.));
#15377=DIRECTION('center_axis',(0.,0.,1.));
#15378=DIRECTION('ref_axis',(0.98039945695656,0.197020061920814,0.));
#15379=DIRECTION('center_axis',(0.,0.,1.));
#15380=DIRECTION('ref_axis',(0.692304064379401,0.721605905216803,0.));
#15381=DIRECTION('center_axis',(0.,0.,1.));
#15382=DIRECTION('ref_axis',(1.,0.,0.));
#15383=DIRECTION('center_axis',(0.,0.,1.));
#15384=DIRECTION('ref_axis',(1.,0.,0.));
#15385=DIRECTION('center_axis',(0.,0.,1.));
#15386=DIRECTION('ref_axis',(0.853892973276138,0.520448643181666,0.));
#15387=DIRECTION('center_axis',(0.,0.,1.));
#15388=DIRECTION('ref_axis',(0.403749265510609,0.91486967957171,0.));
#15389=DIRECTION('center_axis',(0.,0.,1.));
#15390=DIRECTION('ref_axis',(1.,0.,0.));
#15391=DIRECTION('center_axis',(0.,0.,1.));
#15392=DIRECTION('ref_axis',(1.,0.,0.));
#15393=DIRECTION('center_axis',(0.,0.,1.));
#15394=DIRECTION('ref_axis',(-0.624419851739997,-0.7810888865891,0.));
#15395=DIRECTION('center_axis',(0.,0.,1.));
#15396=DIRECTION('ref_axis',(0.0664963465165425,0.997786668531882,0.));
#15397=DIRECTION('center_axis',(0.,0.,1.));
#15398=DIRECTION('ref_axis',(1.,0.,0.));
#15399=DIRECTION('center_axis',(0.,0.,1.));
#15400=DIRECTION('ref_axis',(1.,0.,0.));
#15401=DIRECTION('center_axis',(0.,0.,1.));
#15402=DIRECTION('ref_axis',(-0.319595441725534,-0.947554090080488,0.));
#15403=DIRECTION('center_axis',(0.,0.,1.));
#15404=DIRECTION('ref_axis',(-0.278777013248851,0.9603558595042,0.));
#15405=DIRECTION('center_axis',(0.,0.,1.));
#15406=DIRECTION('ref_axis',(1.,0.,0.));
#15407=DIRECTION('center_axis',(0.,0.,1.));
#15408=DIRECTION('ref_axis',(1.,0.,0.));
#15409=DIRECTION('center_axis',(0.,0.,1.));
#15410=DIRECTION('ref_axis',(0.0237812816597838,-0.99971718532924,0.));
#15411=DIRECTION('center_axis',(0.,0.,1.));
#15412=DIRECTION('ref_axis',(-0.590425750906046,0.807091960477263,0.));
#15413=DIRECTION('center_axis',(0.,0.,1.));
#15414=DIRECTION('ref_axis',(1.,0.,0.));
#15415=DIRECTION('center_axis',(0.,0.,1.));
#15416=DIRECTION('ref_axis',(1.,0.,0.));
#15417=DIRECTION('center_axis',(0.,0.,1.));
#15418=DIRECTION('ref_axis',(0.364271227124465,-0.93129290402603,0.));
#15419=DIRECTION('center_axis',(0.,0.,1.));
#15420=DIRECTION('ref_axis',(-0.830860429247751,0.556480859608165,0.));
#15421=DIRECTION('center_axis',(0.,0.,1.));
#15422=DIRECTION('ref_axis',(1.,0.,0.));
#15423=DIRECTION('center_axis',(0.,0.,1.));
#15424=DIRECTION('ref_axis',(1.,0.,0.));
#15425=DIRECTION('center_axis',(0.,0.,1.));
#15426=DIRECTION('ref_axis',(0.66080906094452,-0.750554052000002,0.));
#15427=DIRECTION('center_axis',(0.,0.,1.));
#15428=DIRECTION('ref_axis',(-0.971081077628326,0.238749954287344,0.));
#15429=DIRECTION('center_axis',(0.,0.,1.));
#15430=DIRECTION('ref_axis',(1.,0.,0.));
#15431=DIRECTION('center_axis',(0.,0.,1.));
#15432=DIRECTION('ref_axis',(1.,0.,0.));
#15433=DIRECTION('center_axis',(0.,0.,1.));
#15434=DIRECTION('ref_axis',(0.877651349637868,-0.479299602001534,0.));
#15435=DIRECTION('center_axis',(0.,0.,1.));
#15436=DIRECTION('ref_axis',(-0.99417501641652,-0.107777719094496,0.));
#15437=DIRECTION('center_axis',(0.,0.,1.));
#15438=DIRECTION('ref_axis',(1.,0.,0.));
#15439=DIRECTION('center_axis',(0.,0.,1.));
#15440=DIRECTION('ref_axis',(1.,0.,0.));
#15441=DIRECTION('center_axis',(-3.47737300407025E-13,-6.53322053534217E-12,
1.));
#15442=DIRECTION('ref_axis',(0.988657789032747,-0.150185805537277,-6.37403798268417E-13));
#15443=DIRECTION('center_axis',(0.,0.,1.));
#15444=DIRECTION('ref_axis',(-0.897356775764326,-0.441305808923759,0.));
#15445=DIRECTION('center_axis',(0.,0.,1.));
#15446=DIRECTION('ref_axis',(1.,0.,0.));
#15447=DIRECTION('center_axis',(0.,0.,1.));
#15448=DIRECTION('ref_axis',(1.,0.,0.));
#15449=DIRECTION('center_axis',(0.,0.,1.));
#15450=DIRECTION('ref_axis',(0.980399405327247,0.197020318835346,0.));
#15451=DIRECTION('center_axis',(0.,0.,1.));
#15452=DIRECTION('ref_axis',(-0.692304064379401,-0.721605905216803,0.));
#15453=DIRECTION('center_axis',(0.,0.,1.));
#15454=DIRECTION('ref_axis',(1.,0.,0.));
#15455=DIRECTION('center_axis',(0.,0.,1.));
#15456=DIRECTION('ref_axis',(1.,0.,0.));
#15457=DIRECTION('center_axis',(3.9330849286785E-12,-5.22825041966026E-12,
1.));
#15458=DIRECTION('ref_axis',(0.853893037802406,0.520448537314285,-6.37398554059169E-13));
#15459=DIRECTION('center_axis',(0.,0.,1.));
#15460=DIRECTION('ref_axis',(-0.403749265510619,-0.914869679571706,0.));
#15461=DIRECTION('center_axis',(0.,0.,1.));
#15462=DIRECTION('ref_axis',(1.,0.,0.));
#15463=DIRECTION('center_axis',(0.,0.,1.));
#15464=DIRECTION('ref_axis',(1.,0.,0.));
#15465=DIRECTION('center_axis',(-5.48451776394876E-12,3.56805502485972E-12,
1.));
#15466=DIRECTION('ref_axis',(-0.624419281297108,-0.781089342613509,-6.37668886649601E-13));
#15467=DIRECTION('center_axis',(0.,0.,1.));
#15468=DIRECTION('ref_axis',(-0.0664963465165425,-0.997786668531882,0.));
#15469=DIRECTION('center_axis',(0.,0.,1.));
#15470=DIRECTION('ref_axis',(1.,0.,0.));
#15471=DIRECTION('center_axis',(0.,0.,1.));
#15472=DIRECTION('ref_axis',(1.,0.,0.));
#15473=DIRECTION('center_axis',(0.,0.,1.));
#15474=DIRECTION('ref_axis',(-0.319595564366664,-0.947554048715509,0.));
#15475=DIRECTION('center_axis',(0.,0.,1.));
#15476=DIRECTION('ref_axis',(0.278777013248859,-0.960355859504197,0.));
#15477=DIRECTION('center_axis',(0.,0.,1.));
#15478=DIRECTION('ref_axis',(1.,0.,0.));
#15479=DIRECTION('center_axis',(0.,0.,1.));
#15480=DIRECTION('ref_axis',(1.,0.,0.));
#15481=DIRECTION('center_axis',(-6.49423776379365E-12,-7.9201404422884E-13,
1.));
#15482=DIRECTION('ref_axis',(0.0237818414100777,-0.999717172013738,-6.37345107913742E-13));
#15483=DIRECTION('center_axis',(0.,0.,1.));
#15484=DIRECTION('ref_axis',(0.590425750905992,-0.807091960477302,0.));
#15485=DIRECTION('center_axis',(0.,0.,1.));
#15486=DIRECTION('ref_axis',(1.,0.,0.));
#15487=DIRECTION('center_axis',(0.,0.,1.));
#15488=DIRECTION('ref_axis',(1.,0.,0.));
#15489=DIRECTION('center_axis',(0.,0.,1.));
#15490=DIRECTION('ref_axis',(0.387549166087966,-0.921849035289685,0.));
#15491=DIRECTION('center_axis',(0.,0.,1.));
#15492=DIRECTION('ref_axis',(0.830860429247751,-0.556480859608165,0.));
#15493=DIRECTION('center_axis',(0.,0.,1.));
#15494=DIRECTION('ref_axis',(1.,0.,0.));
#15495=DIRECTION('center_axis',(0.,0.,1.));
#15496=DIRECTION('ref_axis',(1.,0.,0.));
#15497=DIRECTION('center_axis',(-4.30576259291751E-12,-4.61078946408106E-12,
1.));
#15498=DIRECTION('ref_axis',(0.679434606802726,-0.733736066360939,-4.57618409888508E-13));
#15499=DIRECTION('center_axis',(0.,0.,1.));
#15500=DIRECTION('ref_axis',(0.971081077628323,-0.238749954287355,0.));
#15501=DIRECTION('center_axis',(0.,0.,1.));
#15502=DIRECTION('ref_axis',(1.,0.,0.));
#15503=DIRECTION('center_axis',(0.,0.,1.));
#15504=DIRECTION('ref_axis',(1.,0.,0.));
#15505=DIRECTION('center_axis',(0.,0.,1.));
#15506=DIRECTION('ref_axis',(1.,0.,0.));
#15507=DIRECTION('center_axis',(0.,0.,1.));
#15508=DIRECTION('ref_axis',(1.,0.,0.));
#15509=DIRECTION('center_axis',(0.,0.,1.));
#15510=DIRECTION('ref_axis',(1.,0.,0.));
#15511=DIRECTION('center_axis',(0.,0.,1.));
#15512=DIRECTION('ref_axis',(1.,0.,0.));
#15513=DIRECTION('center_axis',(0.,0.,1.));
#15514=DIRECTION('ref_axis',(1.,0.,0.));
#15515=DIRECTION('center_axis',(0.,0.,1.));
#15516=DIRECTION('ref_axis',(1.,0.,0.));
#15517=DIRECTION('center_axis',(0.,0.,1.));
#15518=DIRECTION('ref_axis',(1.,0.,0.));
#15519=DIRECTION('center_axis',(0.,0.,1.));
#15520=DIRECTION('ref_axis',(-0.999229036240747,-0.0392598157584637,0.));
#15521=DIRECTION('center_axis',(0.,0.,1.));
#15522=DIRECTION('ref_axis',(1.,0.,0.));
#15523=DIRECTION('center_axis',(0.,0.,1.));
#15524=DIRECTION('ref_axis',(1.,0.,0.));
#15525=DIRECTION('center_axis',(0.,0.,1.));
#15526=DIRECTION('ref_axis',(1.,0.,0.));
#15527=DIRECTION('center_axis',(0.,0.,1.));
#15528=DIRECTION('ref_axis',(1.,0.,0.));
#15529=DIRECTION('center_axis',(0.,0.,1.));
#15530=DIRECTION('ref_axis',(1.,0.,0.));
#15531=DIRECTION('center_axis',(0.,0.,1.));
#15532=DIRECTION('ref_axis',(1.,0.,0.));
#15533=DIRECTION('center_axis',(0.,0.,1.));
#15534=DIRECTION('ref_axis',(1.,0.,0.));
#15535=DIRECTION('center_axis',(0.,0.,1.));
#15536=DIRECTION('ref_axis',(1.,0.,0.));
#15537=DIRECTION('center_axis',(-0.378441568052335,-0.916480699435958,0.129788701863713));
#15538=DIRECTION('ref_axis',(0.924381621172865,-0.381465300242715,0.00168616385949415));
#15539=DIRECTION('center_axis',(-0.305383147490373,-0.943343005537968,0.129788701863709));
#15540=DIRECTION('ref_axis',(0.951456650156171,-0.307778183945461,0.00168296192234297));
#15541=DIRECTION('center_axis',(-0.224107897665031,-0.965883296818355,0.129788701863708));
#15542=DIRECTION('ref_axis',(0.974171131086531,-0.225804727578402,0.00168296192248745));
#15543=DIRECTION('center_axis',(-0.299184912142572,-0.945327076315269,0.129788701863708));
#15544=DIRECTION('ref_axis',(0.953456387284282,-0.30152624164116,0.00168616385952863));
#15545=DIRECTION('center_axis',(-0.66907360907623,-0.731775511004736,0.129788701863704));
#15546=DIRECTION('ref_axis',(0.738165771541167,-0.674617262287642,0.00168616385934017));
#15547=DIRECTION('center_axis',(-0.609608600176635,-0.782005273293741,0.129788701863704));
#15548=DIRECTION('ref_axis',(0.788810454557559,-0.614634228155136,0.00168296192406015));
#15549=DIRECTION('center_axis',(-0.540944081297966,-0.830983991288178,0.129788701863717));
#15550=DIRECTION('ref_axis',(0.838191657982016,-0.545373186110699,0.00168296192002916));
#15551=DIRECTION('center_axis',(-0.604462756307606,-0.785989611321642,0.129788701863707));
#15552=DIRECTION('ref_axis',(0.792827883000484,-0.609443274463194,0.00168616385667629));
#15553=DIRECTION('center_axis',(-0.879005498371115,-0.458807396084543,0.129788701863717));
#15554=DIRECTION('ref_axis',(0.462916235689704,-0.886400426210586,0.0016861638606374));
#15555=DIRECTION('center_axis',(-0.840306258803425,-0.526346163930475,0.129788701863704));
#15556=DIRECTION('ref_axis',(0.531022076545678,-0.847356313400851,0.00168296192311816));
#15557=DIRECTION('center_axis',(-0.792529856525827,-0.595861809126773,0.129788793581421));
#15558=DIRECTION('ref_axis',(0.601120180867897,-0.799156862206045,0.00168455998250973));
#15559=DIRECTION('center_axis',(-0.83683754017856,-0.531843783212709,0.129788757625188));
#15560=DIRECTION('ref_axis',(0.536565993516091,-0.843856680285777,0.00168455904000648));
#15561=DIRECTION('center_axis',(-0.98291635181688,-0.130500337928791,0.129788701863707));
#15562=DIRECTION('ref_axis',(0.131832169906145,-0.991270616849543,0.00168616386006647));
#15563=DIRECTION('center_axis',(-0.969650581024334,-0.207201939150445,0.129788701863711));
#15564=DIRECTION('ref_axis',(0.209184599046497,-0.97787472160851,0.001682961923121));
#15565=DIRECTION('center_axis',(-0.948531199288248,-0.288865769930391,0.129788793581421));
#15566=DIRECTION('ref_axis',(0.291540453620295,-0.956557016680417,0.00168455998226241));
#15567=DIRECTION('center_axis',(-0.968271348267041,-0.213554383048539,0.129788757625165));
#15568=DIRECTION('ref_axis',(0.215591121919023,-0.976482273474809,0.00168455904166718));
#15569=DIRECTION('center_axis',(-0.968272986935159,0.213546986961178,0.129788701863713));
#15570=DIRECTION('ref_axis',(-0.215152801203895,-0.9765789415022,0.00168616385887264));
#15571=DIRECTION('center_axis',(-0.982040732655837,0.136933897459027,0.129788701863709));
#15572=DIRECTION('ref_axis',(-0.137883628326555,-0.990447006496901,0.00168296192237585));
#15573=DIRECTION('center_axis',(-0.990125680589725,0.052971744330466,0.129788793581421));
#15574=DIRECTION('ref_axis',(-0.0532033550188353,-0.998582277667897,0.00168455998277433));
#15575=DIRECTION('center_axis',(-0.982917341583731,0.130492827420077,0.129788757625168));
#15576=DIRECTION('ref_axis',(-0.131387220749492,-0.991329693131685,0.00168455904115533));
#15577=DIRECTION('center_axis',(-0.836841609645931,0.531837393602351,0.129788701863704));
#15578=DIRECTION('ref_axis',(-0.53618716916805,-0.844097433043719,0.00168616385845728));
#15579=DIRECTION('center_axis',(-0.875982278548042,0.464553485121265,0.129788701863712));
#15580=DIRECTION('ref_axis',(-0.468321055193095,-0.883556764957403,0.00168296192337288));
#15581=DIRECTION('center_axis',(-0.912296392111608,0.388420084445723,0.129788793581425));
#15582=DIRECTION('ref_axis',(-0.391530053845128,-0.920163778462124,0.00168455998354657));
#15583=DIRECTION('center_axis',(-0.879008997189149,0.458800677042487,0.129788757625161));
#15584=DIRECTION('ref_axis',(-0.462518325536303,-0.886608121327528,0.00168455904187875));
#15585=DIRECTION('center_axis',(-0.60447478375946,0.785980361502429,0.129788701863699));
#15586=DIRECTION('ref_axis',(-0.792549451262032,-0.609805316601694,0.00168616385909342));
#15587=DIRECTION('center_axis',(-0.664267433537108,0.736141066379643,0.129788701863703));
#15588=DIRECTION('ref_axis',(-0.742272051101889,-0.670096537666153,0.00168296192149378));
#15589=DIRECTION('center_axis',(-0.724425523284778,0.677024780995576,0.129788701863712));
#15590=DIRECTION('ref_axis',(-0.682638195940333,-0.730754583346887,0.0016829619261111));
#15591=DIRECTION('center_axis',(-0.669084806894506,0.731765272509891,0.129788701863711));
#15592=DIRECTION('ref_axis',(-0.737857578818759,-0.674954331959692,0.00168616386059911));
#15593=DIRECTION('center_axis',(-0.299199377858597,0.945322497964352,0.12978870186371));
#15594=DIRECTION('ref_axis',(-0.953318572743403,-0.301961679214298,0.00168616385977842));
#15595=DIRECTION('center_axis',(-0.372432132484037,0.918939170762639,0.129788701863704));
#15596=DIRECTION('ref_axis',(-0.926694082893931,-0.375812778346535,0.00168296192305547));
#15597=DIRECTION('center_axis',(-0.449187964027621,0.883959864492387,0.129788793581425));
#15598=DIRECTION('ref_axis',(-0.891399297735882,-0.453215681826704,0.00168455998165862));
#15599=DIRECTION('center_axis',(-0.37844856723093,0.916477801343259,0.129788757625163));
#15600=DIRECTION('ref_axis',(-0.924210308154052,-0.381880175660676,0.00168455904140337));
#15601=DIRECTION('center_axis',(0.0421638887274789,0.990644789698058,0.12978870186371));
#15602=DIRECTION('ref_axis',(-0.999103404868771,0.0423029931691144,0.00168616385986293));
#15603=DIRECTION('center_axis',(-0.035676019747098,0.990899649048045,0.12978870186371));
#15604=DIRECTION('ref_axis',(-0.99934313173509,-0.0362004515589168,0.0016829619223935));
#15605=DIRECTION('center_axis',(-0.119766535590606,0.984281893571808,0.129788793581421));
#15606=DIRECTION('ref_axis',(-0.992650234712453,-0.121006916260922,0.00168455998244488));
#15607=DIRECTION('center_axis',(-0.0421714570058776,0.990644460241976,0.129788757625168));
#15608=DIRECTION('ref_axis',(-0.999084319039234,-0.0427514410370733,0.00168455904153955));
#15609=DIRECTION('center_axis',(0.378441568051778,0.916480699436188,0.129788701863713));
#15610=DIRECTION('ref_axis',(-0.924381621173083,0.381465300242189,0.00168616385911061));
#15611=DIRECTION('center_axis',(0.305383147489853,0.943343005538136,0.129788701863713));
#15612=DIRECTION('ref_axis',(-0.951456650156345,0.307778183944919,0.00168296192291583));
#15613=DIRECTION('center_axis',(0.22410050459774,0.965884999831614,0.129788793581424));
#15614=DIRECTION('ref_axis',(-0.974172903424311,0.225797069271315,0.00168455998189598));
#15615=DIRECTION('center_axis',(0.299192153321727,0.945324776880847,0.129788757625169));
#15616=DIRECTION('ref_axis',(-0.953454016134601,0.30153374832286,0.00168455904205274));
#15617=DIRECTION('center_axis',(0.669073609076934,0.731775511004093,0.129788701863703));
#15618=DIRECTION('ref_axis',(-0.738165771540547,0.674617262288319,0.0016861638597269));
#15619=DIRECTION('center_axis',(0.609608600175811,0.782005273294383,0.129788701863703));
#15620=DIRECTION('ref_axis',(-0.788810454558216,0.614634228154292,0.00168296192405618));
#15621=DIRECTION('center_axis',(0.540944081288723,0.830983991294197,0.129788701863706));
#15622=DIRECTION('ref_axis',(-0.838191657988026,0.545373186101464,0.00168296191918214));
#15623=DIRECTION('center_axis',(0.604462756308468,0.785989611320978,0.129788701863709));
#15624=DIRECTION('ref_axis',(-0.792827882999811,0.60944327446407,0.0016861638564983));
#15625=DIRECTION('center_axis',(0.879005498370731,0.458807396085279,0.129788701863717));
#15626=DIRECTION('ref_axis',(-0.462916235690331,0.886400426210261,0.00168616385968331));
#15627=DIRECTION('center_axis',(0.84030625880358,0.526346163930226,0.129788701863705));
#15628=DIRECTION('ref_axis',(-0.531022076545447,0.847356313400996,0.00168296192330928));
#15629=DIRECTION('center_axis',(0.792529856523363,0.595861809130046,0.129788793581438));
#15630=DIRECTION('ref_axis',(-0.601120180871209,0.799156862203554,0.00168455998284762));
#15631=DIRECTION('center_axis',(0.83683754017869,0.531843783212505,0.129788757625188));
#15632=DIRECTION('ref_axis',(-0.5365659935158,0.843856680285963,0.00168455903923744));
#15633=DIRECTION('center_axis',(0.98291635181687,0.130500337928863,0.129788701863709));
#15634=DIRECTION('ref_axis',(-0.131832169906245,0.99127061684953,0.00168616385986865));
#15635=DIRECTION('center_axis',(0.969650581024497,0.20720193914968,0.129788701863711));
#15636=DIRECTION('ref_axis',(-0.209184599045755,0.977874721608669,0.00168296192350968));
#15637=DIRECTION('center_axis',(0.948531199288787,0.288865769928619,0.129788793581424));
#15638=DIRECTION('ref_axis',(-0.291540453618539,0.956557016680951,0.00168455998264496));
#15639=DIRECTION('center_axis',(0.968271348265747,0.213554383054406,0.12978875762517));
#15640=DIRECTION('ref_axis',(-0.215591121924833,0.976482273473528,0.00168455904061127));
#15641=DIRECTION('center_axis',(0.968272986934853,-0.213546986962567,0.129788701863712));
#15642=DIRECTION('ref_axis',(0.215152801205168,0.976578941501918,0.00168616385981979));
#15643=DIRECTION('center_axis',(0.982040732655296,-0.136933897462913,0.129788701863709));
#15644=DIRECTION('ref_axis',(0.137883628330465,0.990447006496357,0.00168296192237878));
#15645=DIRECTION('center_axis',(0.990125680589855,-0.0529717443280386,0.129788793581422));
#15646=DIRECTION('ref_axis',(0.0532033550164054,0.998582277668026,0.00168455998277367));
#15647=DIRECTION('center_axis',(0.982917341583747,-0.130492827419958,0.129788757625171));
#15648=DIRECTION('ref_axis',(0.131387220749417,0.991329693131696,0.00168455904058849));
#15649=DIRECTION('center_axis',(0.836841609645931,-0.531837393602351,0.129788701863704));
#15650=DIRECTION('ref_axis',(0.53618716916805,0.844097433043719,0.00168616385845728));
#15651=DIRECTION('center_axis',(0.875982278548042,-0.464553485121265,0.129788701863712));
#15652=DIRECTION('ref_axis',(0.468321055193095,0.883556764957403,0.00168296192337288));
#15653=DIRECTION('center_axis',(0.912293431178322,-0.38842706947047,0.129788701863712));
#15654=DIRECTION('ref_axis',(0.391537288042102,0.920160703199067,0.00168296192312245));
#15655=DIRECTION('center_axis',(0.879012519102615,-0.458793945175181,0.129788701863713));
#15656=DIRECTION('ref_axis',(0.46251134465318,0.886611759970813,0.00168616386051783));
#15657=DIRECTION('center_axis',(0.60447478375946,-0.785980361502429,0.129788701863699));
#15658=DIRECTION('ref_axis',(0.792549451262032,0.609805316601694,0.00168616385909342));
#15659=DIRECTION('center_axis',(0.664267433536779,-0.736141066379941,0.129788701863701));
#15660=DIRECTION('ref_axis',(0.742272051102183,0.670096537665826,0.00168296192169911));
#15661=DIRECTION('center_axis',(0.724430694688769,-0.677019229899289,0.129788793581426));
#15662=DIRECTION('ref_axis',(0.682632449802081,0.730759947407406,0.00168455998210372));
#15663=DIRECTION('center_axis',(0.669079194957684,-0.731770393818234,0.129788757625171));
#15664=DIRECTION('ref_axis',(0.737862894201601,0.674948525164164,0.0016845590394145));
#15665=DIRECTION('center_axis',(0.29919937785432,-0.945322497965705,0.12978870186371));
#15666=DIRECTION('ref_axis',(0.953318572744759,0.301961679210016,0.00168616386027698));
#15667=DIRECTION('center_axis',(0.372432132484241,-0.918939170762557,0.129788701863703));
#15668=DIRECTION('ref_axis',(0.926694082893838,0.375812778346763,0.00168296192307007));
#15669=DIRECTION('center_axis',(0.449187964027621,-0.883959864492387,0.129788793581425));
#15670=DIRECTION('ref_axis',(0.891399297735882,0.453215681826704,0.00168455998165862));
#15671=DIRECTION('center_axis',(0.378448567230374,-0.916477801343488,0.129788757625164));
#15672=DIRECTION('ref_axis',(0.924210308154263,0.381880175660163,0.00168455904178805));
#15673=DIRECTION('center_axis',(-0.0421638887269278,-0.990644789698082,
0.12978870186371));
#15674=DIRECTION('ref_axis',(0.999103404868793,-0.0423029931685897,0.0016861638598628));
#15675=DIRECTION('center_axis',(0.0356760197477962,-0.990899649048019,0.129788701863709));
#15676=DIRECTION('ref_axis',(0.999343131735064,0.036200451559631,0.00168296192257817));
#15677=DIRECTION('center_axis',(0.119759005916489,-0.984282821840566,0.12978870186371));
#15678=DIRECTION('ref_axis',(0.992651188554834,0.120999113632468,0.00168296192272656));
#15679=DIRECTION('center_axis',(0.0421790479366033,-0.990644144374606,0.12978870186371));
#15680=DIRECTION('ref_axis',(0.999083979754942,0.0427593059867003,0.00168616385957026));
#15681=DIRECTION('',(-0.956649531312375,0.291241608016117,0.));
#15682=DIRECTION('',(0.886464649099777,-0.462796311455061,0.));
#15683=DIRECTION('center_axis',(0.,0.,1.));
#15684=DIRECTION('ref_axis',(1.,0.,0.));
#15685=DIRECTION('center_axis',(0.,0.,1.));
#15686=DIRECTION('ref_axis',(1.,0.,0.));
#15687=DIRECTION('center_axis',(0.,0.,1.));
#15688=DIRECTION('ref_axis',(1.,0.,0.));
#15689=DIRECTION('center_axis',(0.,0.,1.));
#15690=DIRECTION('ref_axis',(1.,0.,0.));
#15691=DIRECTION('',(0.674718628572079,-0.738075045139593,0.));
#15692=DIRECTION('',(-0.799346008736428,0.600870999730511,0.));
#15693=DIRECTION('',(-0.54562956041628,0.838026480965809,0.));
#15694=DIRECTION('',(0.381591583652422,-0.924331035552543,0.));
#15695=DIRECTION('center_axis',(0.,0.,1.));
#15696=DIRECTION('ref_axis',(1.,0.,0.));
#15697=DIRECTION('center_axis',(0.,0.,1.));
#15698=DIRECTION('ref_axis',(1.,0.,0.));
#15699=DIRECTION('center_axis',(0.,0.,1.));
#15700=DIRECTION('ref_axis',(1.,0.,0.));
#15701=DIRECTION('',(-0.226102134475161,0.974103600643061,0.));
#15702=DIRECTION('',(0.0424389620521028,-0.999099061404794,0.));
#15703=DIRECTION('center_axis',(0.,0.,1.));
#15704=DIRECTION('ref_axis',(1.,0.,0.));
#15705=DIRECTION('',(0.120696545795735,0.992689449844703,0.));
#15706=DIRECTION('',(-0.301832424704053,-0.953360995319859,0.));
#15707=DIRECTION('center_axis',(0.,0.,1.));
#15708=DIRECTION('ref_axis',(1.,0.,0.));
#15709=DIRECTION('',(0.452937441352379,0.891542300859113,0.));
#15710=DIRECTION('',(-0.609698366468669,-0.792633523089604,0.));
#15711=DIRECTION('center_axis',(0.,0.,1.));
#15712=DIRECTION('ref_axis',(1.,0.,0.));
#15713=DIRECTION('',(0.73054739683727,0.682861992626833,0.));
#15714=DIRECTION('',(-0.844025687047658,-0.536302749949811,0.));
#15715=DIRECTION('center_axis',(0.,0.,1.));
#15716=DIRECTION('ref_axis',(1.,0.,0.));
#15717=DIRECTION('',(0.920042554532171,0.391818450114231,0.));
#15718=DIRECTION('',(-0.976551053276238,-0.215285950180383,0.));
#15719=DIRECTION('center_axis',(0.,0.,1.));
#15720=DIRECTION('ref_axis',(1.,0.,0.));
#15721=DIRECTION('',(0.998567001768609,0.0535158198932806,0.));
#15722=DIRECTION('',(-0.991289950121085,0.131697512462977,0.));
#15723=DIRECTION('center_axis',(0.,0.,1.));
#15724=DIRECTION('ref_axis',(1.,0.,0.));
#15725=DIRECTION('',(0.956649531312375,-0.291241608016117,0.));
#15726=DIRECTION('',(-0.886464649099777,0.462796311455061,0.));
#15727=DIRECTION('center_axis',(0.,0.,1.));
#15728=DIRECTION('ref_axis',(1.,0.,0.));
#15729=DIRECTION('',(0.799346008736428,-0.600870999730511,0.));
#15730=DIRECTION('',(-0.674718628572181,0.7380750451395,0.));
#15731=DIRECTION('center_axis',(0.,0.,1.));
#15732=DIRECTION('ref_axis',(1.,0.,0.));
#15733=DIRECTION('',(0.545629560416191,-0.838026480965866,0.));
#15734=DIRECTION('',(-0.381591583652368,0.924331035552565,0.));
#15735=DIRECTION('center_axis',(0.,0.,1.));
#15736=DIRECTION('ref_axis',(1.,0.,0.));
#15737=DIRECTION('',(0.226102134475161,-0.974103600643061,0.));
#15738=DIRECTION('',(-0.0424389620521028,0.999099061404794,0.));
#15739=DIRECTION('center_axis',(0.,0.,1.));
#15740=DIRECTION('ref_axis',(1.,0.,0.));
#15741=DIRECTION('',(-0.120696545795755,-0.9926894498447,0.));
#15742=DIRECTION('',(0.301832424704055,0.953360995319859,0.));
#15743=DIRECTION('center_axis',(0.,0.,1.));
#15744=DIRECTION('ref_axis',(1.,0.,0.));
#15745=DIRECTION('',(-0.452937441352379,-0.891542300859113,0.));
#15746=DIRECTION('',(0.609698366468669,0.792633523089604,0.));
#15747=DIRECTION('center_axis',(0.,0.,1.));
#15748=DIRECTION('ref_axis',(1.,0.,0.));
#15749=DIRECTION('',(-0.730547396837178,-0.68286199262693,0.));
#15750=DIRECTION('',(0.844025687047666,0.536302749949798,0.));
#15751=DIRECTION('center_axis',(0.,0.,1.));
#15752=DIRECTION('ref_axis',(1.,0.,0.));
#15753=DIRECTION('',(-0.920042554532177,-0.391818450114216,0.));
#15754=DIRECTION('',(0.976551053276238,0.215285950180383,0.));
#15755=DIRECTION('center_axis',(0.,0.,1.));
#15756=DIRECTION('ref_axis',(1.,0.,0.));
#15757=DIRECTION('',(-0.998567001768609,-0.0535158198932787,0.));
#15758=DIRECTION('',(0.991289950121088,-0.131697512462957,0.));
#15759=DIRECTION('center_axis',(0.,0.,1.));
#15760=DIRECTION('ref_axis',(1.,0.,0.));
#15761=DIRECTION('center_axis',(0.,0.,1.));
#15762=DIRECTION('ref_axis',(1.,0.,0.));
#15763=DIRECTION('center_axis',(0.,0.,1.));
#15764=DIRECTION('ref_axis',(1.,0.,0.));
#15765=DIRECTION('center_axis',(0.,0.,1.));
#15766=DIRECTION('ref_axis',(1.,0.,0.));
#15767=DIRECTION('center_axis',(0.,0.,1.));
#15768=DIRECTION('ref_axis',(1.,0.,0.));
#15769=DIRECTION('center_axis',(0.,0.,1.));
#15770=DIRECTION('ref_axis',(1.,0.,0.));
#15771=DIRECTION('center_axis',(0.,0.,1.));
#15772=DIRECTION('ref_axis',(-0.990865895863231,0.134850941469303,0.));
#15773=DIRECTION('center_axis',(0.,0.,1.));
#15774=DIRECTION('ref_axis',(1.,0.,0.));
#15775=DIRECTION('center_axis',(0.,0.,1.));
#15776=DIRECTION('ref_axis',(1.,0.,0.));
#15777=DIRECTION('center_axis',(0.,0.,1.));
#15778=DIRECTION('ref_axis',(1.,0.,0.));
#15779=DIRECTION('center_axis',(0.,0.,1.));
#15780=DIRECTION('ref_axis',(1.,0.,0.));
#15781=DIRECTION('center_axis',(0.,0.,1.));
#15782=DIRECTION('ref_axis',(1.,0.,0.));
#15783=DIRECTION('center_axis',(0.,0.,1.));
#15784=DIRECTION('ref_axis',(1.,0.,0.));
#15785=DIRECTION('center_axis',(0.,0.,1.));
#15786=DIRECTION('ref_axis',(1.,0.,0.));
#15787=DIRECTION('center_axis',(0.,0.,1.));
#15788=DIRECTION('ref_axis',(1.,0.,0.));
#15789=DIRECTION('center_axis',(0.,0.,1.));
#15790=DIRECTION('ref_axis',(1.,0.,0.));
#17354=CARTESIAN_POINT('',(0.,0.,0.));
#17355=CARTESIAN_POINT('Origin',(0.,0.,-16.4167025567876));
#17356=CARTESIAN_POINT('',(4.94641461892554,-6.44544214322681,11.1250611305836));
#17357=CARTESIAN_POINT('',(4.94634499595658,-6.44535064078879,11.2916505155556));
#17358=CARTESIAN_POINT('',(4.94675008185374,-6.44587862049697,-16.4167025567876));
#17359=CARTESIAN_POINT('',(2.10208451021607,7.84862588447237,12.));
#17360=CARTESIAN_POINT('Ctrl Pts',(4.94634499595713,-6.44535064078836,11.2916505155556));
#17361=CARTESIAN_POINT('Ctrl Pts',(5.46269818329968,-6.04916543688375,11.3171416411407));
#17362=CARTESIAN_POINT('Ctrl Pts',(6.90127424538504,-4.64649602035922,11.3952891090332));
#17363=CARTESIAN_POINT('Ctrl Pts',(8.32999914323059,-1.51322275430053,11.5260929192331));
#17364=CARTESIAN_POINT('Ctrl Pts',(8.04577806167976,2.63534640472438,11.6840619461554));
#17365=CARTESIAN_POINT('Ctrl Pts',(5.82000697965989,6.14913288471192,11.8420309730777));
#17366=CARTESIAN_POINT('Ctrl Pts',(3.40044170599962,7.5008890207006,11.9473436576926));
#17367=CARTESIAN_POINT('Ctrl Pts',(2.10208451021619,7.84862588447234,12.));
#17368=CARTESIAN_POINT('',(-2.10232310766211,7.84918820146781,12.));
#17369=CARTESIAN_POINT('Origin',(0.,0.,12.));
#17370=CARTESIAN_POINT('Ctrl Pts',(4.94641461892554,-6.44544214322681,11.1250611305836));
#17371=CARTESIAN_POINT('Ctrl Pts',(5.59685733717957,-5.94568272231727,11.1571897395813));
#17372=CARTESIAN_POINT('Ctrl Pts',(7.11589899816117,-4.3690230073217,11.2419746908865));
#17373=CARTESIAN_POINT('Ctrl Pts',(8.40836897789325,-0.989475114550315,
11.3794159844989));
#17374=CARTESIAN_POINT('Ctrl Pts',(7.86514495884525,3.13354651991988,11.5373850114212));
#17375=CARTESIAN_POINT('Ctrl Pts',(5.42427178070265,6.50055875679946,11.6953540383435));
#17376=CARTESIAN_POINT('Ctrl Pts',(1.76398188025238,8.25622587257004,11.8495590345364));
#17377=CARTESIAN_POINT('Ctrl Pts',(-0.896857186010099,8.17128250291834,
11.9511076884219));
#17378=CARTESIAN_POINT('Ctrl Pts',(-2.10232310766211,7.84918820146781,12.));
#17379=CARTESIAN_POINT('Origin',(0.,0.,-16.4167025567876));
#17380=CARTESIAN_POINT('',(4.94675008185374,-6.44587862049698,9.12505123879043));
#17381=CARTESIAN_POINT('',(4.94675008185378,-6.44587862049694,9.29164626296918));
#17382=CARTESIAN_POINT('',(4.94675008185374,-6.44587862049697,-16.4167025567876));
#17383=CARTESIAN_POINT('',(-8.12531051676223,4.45465981452085E-5,10.5832974437648));
#17384=CARTESIAN_POINT('Ctrl Pts',(4.94675008185378,-6.44587862049695,9.29164626296917));
#17385=CARTESIAN_POINT('Ctrl Pts',(5.10118068104462,-6.32736419846628,9.29927302275314));
#17386=CARTESIAN_POINT('Ctrl Pts',(5.25133360162953,-6.20331023734921,9.3068997825371));
#17387=CARTESIAN_POINT('Ctrl Pts',(5.39681829916228,-6.07404641144,9.31452654232107));
#17388=CARTESIAN_POINT('Ctrl Pts',(5.55368691362083,-5.93466792274758,9.32275008239372));
#17389=CARTESIAN_POINT('Ctrl Pts',(5.70517872870825,-5.78918660410757,9.33097362246638));
#17390=CARTESIAN_POINT('Ctrl Pts',(5.85082702241694,-5.63804139008004,9.33919716253903));
#17391=CARTESIAN_POINT('Ctrl Pts',(5.99644883481933,-5.48692365679126,9.34741920743397));
#17392=CARTESIAN_POINT('Ctrl Pts',(6.13622904182113,-5.3301442957319,9.35564125232891));
#17393=CARTESIAN_POINT('Ctrl Pts',(6.26973810288252,-5.16817875888239,9.36386329722384));
#17394=CARTESIAN_POINT('Ctrl Pts',(6.40323242351307,-5.00623110427828,9.37208443434156));
#17395=CARTESIAN_POINT('Ctrl Pts',(6.53045679299592,-4.83909864454014,9.38030557145927));
#17396=CARTESIAN_POINT('Ctrl Pts',(6.65102172662004,-4.66729017252282,9.38852670857699));
#17397=CARTESIAN_POINT('Ctrl Pts',(6.77159622277953,-4.49546807361966,9.39674849774927));
#17398=CARTESIAN_POINT('Ctrl Pts',(6.8855100561201,-4.31896946130181,9.40497028692155));
#17399=CARTESIAN_POINT('Ctrl Pts',(6.9924162780203,-4.13833325837549,9.41319207609382));
#17400=CARTESIAN_POINT('Ctrl Pts',(7.09932220321884,-3.95769755677698,9.42141384244779));
#17401=CARTESIAN_POINT('Ctrl Pts',(7.19922040798751,-3.77292454272602,9.42963560880176));
#17402=CARTESIAN_POINT('Ctrl Pts',(7.29180896211549,-3.58457942058929,9.43785737515573));
#17403=CARTESIAN_POINT('Ctrl Pts',(7.38441681926181,-3.39619503194298,9.44608085559746));
#17404=CARTESIAN_POINT('Ctrl Pts',(7.46971185125825,-3.20423731220333,9.45430433603919));
#17405=CARTESIAN_POINT('Ctrl Pts',(7.54743903387266,-3.00929420171497,9.46252781648091));
#17406=CARTESIAN_POINT('Ctrl Pts',(7.57884363377462,-2.93053011709735,9.46585040073506));
#17407=CARTESIAN_POINT('Ctrl Pts',(7.60901336428037,-2.8512789138126,9.46917298498921));
#17408=CARTESIAN_POINT('Ctrl Pts',(7.63793365164409,-2.77158025241607,9.47249556924336));
#17409=CARTESIAN_POINT('Ctrl Pts',(7.70951258681434,-2.5743226925063,9.48071910588856));
#17410=CARTESIAN_POINT('Ctrl Pts',(7.77345749340724,-2.37425871081297,9.48894264253376));
#17411=CARTESIAN_POINT('Ctrl Pts',(7.82956695341158,-2.17199652038058,9.49716617917896));
#17412=CARTESIAN_POINT('Ctrl Pts',(7.88566621167817,-1.96977110495586,9.50538822063308));
#17413=CARTESIAN_POINT('Ctrl Pts',(7.93393278795164,-1.76534856255913,9.5136102620872));
#17414=CARTESIAN_POINT('Ctrl Pts',(7.97421534807755,-1.55935151424699,9.52183230354132));
#17415=CARTESIAN_POINT('Ctrl Pts',(8.01449346068486,-1.35337720966573,9.53005343721594));
#17416=CARTESIAN_POINT('Ctrl Pts',(8.0467892604458,-1.14582903557047,9.53827457089056));
#17417=CARTESIAN_POINT('Ctrl Pts',(8.07100251214971,-0.937339859054906,
9.54649570456517));
#17418=CARTESIAN_POINT('Ctrl Pts',(8.09521768437924,-0.728834145776361,
9.55471749031651));
#17419=CARTESIAN_POINT('Ctrl Pts',(8.11134899094865,-0.519387573613384,
9.56293927606786));
#17420=CARTESIAN_POINT('Ctrl Pts',(8.11934794775107,-0.309639251146375,
9.5711610618192));
#17421=CARTESIAN_POINT('Ctrl Pts',(8.1273468823722,-0.0998915103161628,
9.57938282477134));
#17422=CARTESIAN_POINT('Ctrl Pts',(8.127213503792,0.11015768432331,9.58760458772348));
#17423=CARTESIAN_POINT('Ctrl Pts',(8.11895142944701,0.319867548807802,9.59582635067563));
#17424=CARTESIAN_POINT('Ctrl Pts',(8.11068763255972,0.529621135255785,9.60404982776564));
#17425=CARTESIAN_POINT('Ctrl Pts',(8.09429176592694,0.739034955460716,9.61227330485565));
#17426=CARTESIAN_POINT('Ctrl Pts',(8.06981952014667,0.947470566698362,9.62049678194566));
#17427=CARTESIAN_POINT('Ctrl Pts',(8.05993178057643,1.03168666437841,9.62381938668566));
#17428=CARTESIAN_POINT('Ctrl Pts',(8.04872618389744,1.11574312782325,9.62714199142565));
#17429=CARTESIAN_POINT('Ctrl Pts',(8.03620879910646,1.19959814090547,9.63046459616564));
#17430=CARTESIAN_POINT('Ctrl Pts',(8.00522790680143,1.40714174309708,9.63868813976847));
#17431=CARTESIAN_POINT('Ctrl Pts',(7.96619763652384,1.61351824172196,9.6469116833713));
#17432=CARTESIAN_POINT('Ctrl Pts',(7.91923047146385,1.81809689025048,9.65513522697413));
#17433=CARTESIAN_POINT('Ctrl Pts',(7.87227184577047,2.02263834317481,9.66335727540786));
#17434=CARTESIAN_POINT('Ctrl Pts',(7.81737927142266,2.22538231109902,9.6715793238416));
#17435=CARTESIAN_POINT('Ctrl Pts',(7.75471613389214,2.42570922520672,9.67980137227533));
#17436=CARTESIAN_POINT('Ctrl Pts',(7.6920599148738,2.62601402161889,9.68802251292907));
#17437=CARTESIAN_POINT('Ctrl Pts',(7.62163493351841,2.82390201562019,9.69624365358282));
#17438=CARTESIAN_POINT('Ctrl Pts',(7.54365438847455,3.01876895931911,9.70446479423656));
#17439=CARTESIAN_POINT('Ctrl Pts',(7.46566765874121,3.21365135804645,9.7126865869145));
#17440=CARTESIAN_POINT('Ctrl Pts',(7.38012427510874,3.40551195291009,9.72090837959244));
#17441=CARTESIAN_POINT('Ctrl Pts',(7.28728591611064,3.59376564891974,9.72913017227038));
#17442=CARTESIAN_POINT('Ctrl Pts',(7.19444781504218,3.78201882191059,9.737351942106));
#17443=CARTESIAN_POINT('Ctrl Pts',(7.09431491201529,3.96666485277055,9.74557371194161));
#17444=CARTESIAN_POINT('Ctrl Pts',(6.98719549945698,4.14714198151788,9.75379548177722));
#17445=CARTESIAN_POINT('Ctrl Pts',(6.88005375522472,4.32765673515784,9.76201896564281));
#17446=CARTESIAN_POINT('Ctrl Pts',(6.76592274233344,4.50400059678417,9.77024244950839));
#17447=CARTESIAN_POINT('Ctrl Pts',(6.64515542962041,4.67563865997859,9.77846593337397));
#17448=CARTESIAN_POINT('Ctrl Pts',(6.59636138562037,4.74498619301089,9.78178849661196));
#17449=CARTESIAN_POINT('Ctrl Pts',(6.54648450469863,4.8135658675388,9.78511105984995));
#17450=CARTESIAN_POINT('Ctrl Pts',(6.49555003357664,4.88134380307334,9.78843362308793));
#17451=CARTESIAN_POINT('Ctrl Pts',(6.36948432400681,5.04909804392677,9.79665715585387));
#17452=CARTESIAN_POINT('Ctrl Pts',(6.23689602737285,5.21199325894114,9.80488068861981));
#17453=CARTESIAN_POINT('Ctrl Pts',(6.09818438755089,5.36952835339665,9.81310422138575));
#17454=CARTESIAN_POINT('Ctrl Pts',(5.95949796812527,5.5270348049962,9.82132625895809));
#17455=CARTESIAN_POINT('Ctrl Pts',(5.81469062241994,5.67918285992319,9.82954829653043));
#17456=CARTESIAN_POINT('Ctrl Pts',(5.66420103359679,5.82550548995544,9.83777033410278));
#17457=CARTESIAN_POINT('Ctrl Pts',(5.51372805986296,5.97181196495939,9.84599146390542));
#17458=CARTESIAN_POINT('Ctrl Pts',(5.3575743068858,6.11229409360518,9.85421259370807));
#17459=CARTESIAN_POINT('Ctrl Pts',(5.19621496658465,6.24652203898631,9.86243372351071));
#17460=CARTESIAN_POINT('Ctrl Pts',(5.03484282687037,6.3807606316527,9.87065550543326));
#17461=CARTESIAN_POINT('Ctrl Pts',(4.86826449983262,6.50874385914892,9.8788772873558));
#17462=CARTESIAN_POINT('Ctrl Pts',(4.69698868909341,6.63008181073421,9.88709906927834));
#17463=CARTESIAN_POINT('Ctrl Pts',(4.52571335263917,6.75141942631895,9.8953208284337));
#17464=CARTESIAN_POINT('Ctrl Pts',(4.34974080072379,6.86611163451026,9.90354258758907));
#17465=CARTESIAN_POINT('Ctrl Pts',(4.16960961644487,6.97381123984228,9.91176434674443));
#17466=CARTESIAN_POINT('Ctrl Pts',(3.98944087541279,7.08153330018401,9.91998782010925));
#17467=CARTESIAN_POINT('Ctrl Pts',(3.80511202306167,7.1822596937542,9.92821129347406));
#17468=CARTESIAN_POINT('Ctrl Pts',(3.61718814284456,7.27568811190836,9.93643476683888));
#17469=CARTESIAN_POINT('Ctrl Pts',(3.54125902303476,7.31343710659426,9.93975739456266));
#17470=CARTESIAN_POINT('Ctrl Pts',(3.46474329176694,7.34999523346899,9.94308002228644));
#17471=CARTESIAN_POINT('Ctrl Pts',(3.38767928464742,7.38534471956934,9.94640265001022));
#17472=CARTESIAN_POINT('Ctrl Pts',(3.19694494112705,7.47283512238055,9.9546261935469));
#17473=CARTESIAN_POINT('Ctrl Pts',(3.00278850872504,7.55294691300247,9.96284973708356));
#17474=CARTESIAN_POINT('Ctrl Pts',(2.80579966671456,7.62542954808216,9.97107328062024));
#17475=CARTESIAN_POINT('Ctrl Pts',(2.60884664093059,7.69789900447391,9.97929532896411));
#17476=CARTESIAN_POINT('Ctrl Pts',(2.40906251004286,7.76274197206463,9.98751737730799));
#17477=CARTESIAN_POINT('Ctrl Pts',(2.20705541388873,7.81975664343363,9.99573942565187));
#17478=CARTESIAN_POINT('Ctrl Pts',(2.00507062150387,7.87676501976597,10.0039605661926));
#17479=CARTESIAN_POINT('Ctrl Pts',(1.800863637598,7.92594674539523,10.0121817067334));
#17480=CARTESIAN_POINT('Ctrl Pts',(1.59505699769923,7.96715010129662,10.0204028472742));
#17481=CARTESIAN_POINT('Ctrl Pts',(1.38923403596426,8.00835672489834,10.0286246398061));
#17482=CARTESIAN_POINT('Ctrl Pts',(1.18181145343513,8.04158365400576,10.036846432338));
#17483=CARTESIAN_POINT('Ctrl Pts',(0.97342224362766,8.06673023585832,10.04506822487));
#17484=CARTESIAN_POINT('Ctrl Pts',(0.76503361325674,8.09187674778957,10.0532899945408));
#17485=CARTESIAN_POINT('Ctrl Pts',(0.555678654114234,8.10894292475295,10.0615117642116));
#17486=CARTESIAN_POINT('Ctrl Pts',(0.345996295648056,8.11787990339213,10.0697335338824));
#17487=CARTESIAN_POINT('Ctrl Pts',(0.136270224418411,8.12681874513528,10.0779570175566));
#17488=CARTESIAN_POINT('Ctrl Pts',(-0.0737830877680571,8.12762499045848,
10.0861805012309));
#17489=CARTESIAN_POINT('Ctrl Pts',(-0.283522780993305,8.12030186601199,
10.0944039849051));
#17490=CARTESIAN_POINT('Ctrl Pts',(-0.368264671852043,8.11734307741529,
10.0977265489142));
#17491=CARTESIAN_POINT('Ctrl Pts',(-0.452955373840572,8.11305781836599,
10.1010491129234));
#17492=CARTESIAN_POINT('Ctrl Pts',(-0.537552715890539,8.10744871338319,
10.1043716769325));
#17493=CARTESIAN_POINT('Ctrl Pts',(-0.746936273138496,8.09356583803725,
10.1125952245589));
#17494=CARTESIAN_POINT('Ctrl Pts',(-0.95581573925282,8.07156504140797,10.1208187721854));
#17495=CARTESIAN_POINT('Ctrl Pts',(-1.16355327480506,8.04150678288531,10.1290423198118));
#17496=CARTESIAN_POINT('Ctrl Pts',(-1.37125304209956,8.01145398918175,10.137264372335));
#17497=CARTESIAN_POINT('Ctrl Pts',(-1.57781100145189,7.97334669958723,10.1454864248582));
#17498=CARTESIAN_POINT('Ctrl Pts',(-1.78259628568773,7.92729702009154,10.1537084773814));
#17499=CARTESIAN_POINT('Ctrl Pts',(-1.98735896129443,7.88125242455553,10.1619296221766));
#17500=CARTESIAN_POINT('Ctrl Pts',(-2.19034906486886,7.82726725440287,10.1701507669718));
#17501=CARTESIAN_POINT('Ctrl Pts',(-2.39094691996103,7.76550451602656,10.1783719117669));
#17502=CARTESIAN_POINT('Ctrl Pts',(-2.59156068571871,7.70373687886271,10.1865937086323));
#17503=CARTESIAN_POINT('Ctrl Pts',(-2.78978154120482,7.63419052513503,10.1948155054977));
#17504=CARTESIAN_POINT('Ctrl Pts',(-2.98500492896638,7.55707834659311,10.2030373023631));
#17505=CARTESIAN_POINT('Ctrl Pts',(-3.18022777478683,7.47996638211498,10.2112590764048));
#17506=CARTESIAN_POINT('Ctrl Pts',(-3.37245289621099,7.39528874569337,10.2194808504464));
#17507=CARTESIAN_POINT('Ctrl Pts',(-3.56109517563416,7.30330669714583,10.227702624488));
#17508=CARTESIAN_POINT('Ctrl Pts',(-3.74977678216303,7.2113054726863,10.23592611256));
#17509=CARTESIAN_POINT('Ctrl Pts',(-3.93487378939249,7.11199692330008,10.2441496006319));
#17510=CARTESIAN_POINT('Ctrl Pts',(-4.11582418494491,7.00568903400105,10.2523730887038));
#17511=CARTESIAN_POINT('Ctrl Pts',(-4.18893362822572,6.96273742519532,10.2556956270875));
#17512=CARTESIAN_POINT('Ctrl Pts',(-4.26136646570056,6.91864375934967,10.2590181654711));
#17513=CARTESIAN_POINT('Ctrl Pts',(-4.33308686423123,6.87343042370597,10.2623407038548));
#17514=CARTESIAN_POINT('Ctrl Pts',(-4.51059939498032,6.76152455315659,10.2705641968788));
#17515=CARTESIAN_POINT('Ctrl Pts',(-4.68380334479664,6.64272019540365,10.2787876899029));
#17516=CARTESIAN_POINT('Ctrl Pts',(-4.85216661490309,6.51737421848093,10.2870111829269));
#17517=CARTESIAN_POINT('Ctrl Pts',(-5.02049926876101,6.39205103526837,10.2952331805386));
#17518=CARTESIAN_POINT('Ctrl Pts',(-5.1839927633476,6.26018878317385,10.3034551781503));
#17519=CARTESIAN_POINT('Ctrl Pts',(-5.34214572251453,6.12218642658974,10.311677175762));
#17520=CARTESIAN_POINT('Ctrl Pts',(-5.50028121871459,5.98419930797901,10.3198982655155));
#17521=CARTESIAN_POINT('Ctrl Pts',(-5.65307713464885,5.84007363228023,10.3281193552689));
#17522=CARTESIAN_POINT('Ctrl Pts',(-5.80006617113131,5.69024779539504,10.3363404450223));
#17523=CARTESIAN_POINT('Ctrl Pts',(-5.94706687016392,5.54041007087948,10.3445621870617));
#17524=CARTESIAN_POINT('Ctrl Pts',(-6.08825956070333,5.3848714901936,10.352783929101));
#17525=CARTESIAN_POINT('Ctrl Pts',(-6.223213991623,5.2241071176774,10.3610056711403));
#17526=CARTESIAN_POINT('Ctrl Pts',(-6.35816805162263,5.06334318701944,10.3692273905823));
#17527=CARTESIAN_POINT('Ctrl Pts',(-6.48688369873636,4.89735372089354,10.3774491100243));
#17528=CARTESIAN_POINT('Ctrl Pts',(-6.60897080711255,4.72664706036257,10.3856708294663));
#17529=CARTESIAN_POINT('Ctrl Pts',(-6.73108337788995,4.55590479737089,10.3938942636243));
#17530=CARTESIAN_POINT('Ctrl Pts',(-6.84656447660069,4.38044361453761,10.4021176977823));
#17531=CARTESIAN_POINT('Ctrl Pts',(-6.95506654361545,4.20080193967545,10.4103411319402));
#17532=CARTESIAN_POINT('Ctrl Pts',(-6.99890928045173,4.12821362046178,10.4136639982192));
#17533=CARTESIAN_POINT('Ctrl Pts',(-7.04161301819278,4.05494305048928,10.4169868644981));
#17534=CARTESIAN_POINT('Ctrl Pts',(-7.08315690008883,3.98102698951213,10.4203097307771));
#17535=CARTESIAN_POINT('Ctrl Pts',(-7.18597263275045,3.7980943020025,10.4285333948984));
#17536=CARTESIAN_POINT('Ctrl Pts',(-7.28171451842812,3.61114674844409,10.4367570590196));
#17537=CARTESIAN_POINT('Ctrl Pts',(-7.37008456692655,3.42075153129413,10.4449807231409));
#17538=CARTESIAN_POINT('Ctrl Pts',(-7.45843855370341,3.23039091947729,10.4532028925679));
#17539=CARTESIAN_POINT('Ctrl Pts',(-7.53942325343114,3.03658416212785,10.4614250619949));
#17540=CARTESIAN_POINT('Ctrl Pts',(-7.61278773679275,2.83992085048825,10.4696472314219));
#17541=CARTESIAN_POINT('Ctrl Pts',(-7.68614412099281,2.6432792497346,10.4778684931525));
#17542=CARTESIAN_POINT('Ctrl Pts',(-7.7518818652997,2.44378200048974,10.4860897548832));
#17543=CARTESIAN_POINT('Ctrl Pts',(-7.80979878193991,2.24203714244655,10.4943110166138));
#17544=CARTESIAN_POINT('Ctrl Pts',(-7.86772028649138,2.04027630310532,10.5025329295948));
#17545=CARTESIAN_POINT('Ctrl Pts',(-7.91781964157207,1.83626778195898,10.5107548425759));
#17546=CARTESIAN_POINT('Ctrl Pts',(-7.95994469791944,1.63063422279928,10.518976755557));
#17547=CARTESIAN_POINT('Ctrl Pts',(-8.00206963380308,1.42500125168357,10.5271986450261));
#17548=CARTESIAN_POINT('Ctrl Pts',(-8.03622026002123,1.21774354130453,10.5354205344952));
#17549=CARTESIAN_POINT('Ctrl Pts',(-8.06229555673676,1.00949389216715,10.5436424239643));
#17550=CARTESIAN_POINT('Ctrl Pts',(-8.08837628383372,0.801200873435803,
10.5518660257053));
#17551=CARTESIAN_POINT('Ctrl Pts',(-8.10637828512661,0.591915795942659,
10.5600896274462));
#17552=CARTESIAN_POINT('Ctrl Pts',(-8.11625229777714,0.382277649526231,
10.5683132291872));
#17553=CARTESIAN_POINT('Ctrl Pts',(-8.12024080782819,0.297596387342468,
10.5716350720246));
#17554=CARTESIAN_POINT('Ctrl Pts',(-8.12290368527564,0.212857557078161,
10.574956914862));
#17555=CARTESIAN_POINT('Ctrl Pts',(-8.12424009294534,0.128103374972905,
10.5782787576994));
#17556=CARTESIAN_POINT('Ctrl Pts',(-8.12491311392995,0.0854207831386196,
10.5799516528704));
#17557=CARTESIAN_POINT('Ctrl Pts',(-8.12524976576722,0.0427328788580502,
10.5816245480414));
#17558=CARTESIAN_POINT('Ctrl Pts',(-8.12524999987781,4.45603647705344E-5,
10.5832974432124));
#17559=CARTESIAN_POINT('Ctrl Pts',(-8.12591305058771,4.44095313166514E-5,
10.5832974492654));
#17560=CARTESIAN_POINT('Ctrl Pts',(-8.12552057083844,-1.30103839990057,
10.6342808943841));
#17561=CARTESIAN_POINT('Ctrl Pts',(-7.47833086458203,-3.94627513751248,
10.7379206818104));
#17562=CARTESIAN_POINT('Ctrl Pts',(-4.73857352870345,-7.01609149949043,
10.894216811544));
#17563=CARTESIAN_POINT('Ctrl Pts',(-0.826182671114257,-8.42599612481989,
11.0521858384663));
#17564=CARTESIAN_POINT('Ctrl Pts',(2.62202662826466,-7.90340622427413,11.1846637398034));
#17565=CARTESIAN_POINT('Ctrl Pts',(4.3960810936187,-6.86755470903723,11.2644852988333));
#17566=CARTESIAN_POINT('Ctrl Pts',(4.94634499595713,-6.44535064078836,11.2916505155556));
#17567=CARTESIAN_POINT('',(-8.125249999086,-0.000121872618778703,10.4167025567876));
#17568=CARTESIAN_POINT('Ctrl Pts',(-8.12577597885438,-0.000121880508085447,
10.4167025567876));
#17569=CARTESIAN_POINT('Ctrl Pts',(-8.12586828455546,-0.126869683330212,
10.4216689788468));
#17570=CARTESIAN_POINT('Ctrl Pts',(-8.09216383980146,-1.59740819601278,
10.4792917432134));
#17571=CARTESIAN_POINT('Ctrl Pts',(-7.24824502833796,-4.37523271893839,
10.5895708498875));
#17572=CARTESIAN_POINT('Ctrl Pts',(-4.29055725454787,-7.29868675118837,
10.7475398768098));
#17573=CARTESIAN_POINT('Ctrl Pts',(-0.297666946508737,-8.46115357972005,
10.9055089037321));
#17574=CARTESIAN_POINT('Ctrl Pts',(2.94034048028108,-7.76093097353364,11.0313493216566));
#17575=CARTESIAN_POINT('Ctrl Pts',(4.53083127840292,-6.76475033712395,11.1045333972739));
#17576=CARTESIAN_POINT('Ctrl Pts',(4.94641461892554,-6.44544214322681,11.1250611305836));
#17577=CARTESIAN_POINT('Ctrl Pts',(4.94675008185374,-6.44587862049698,9.12505123879043));
#17578=CARTESIAN_POINT('Ctrl Pts',(5.11329136906744,-6.31807011297456,9.13327483954532));
#17579=CARTESIAN_POINT('Ctrl Pts',(5.27486419726295,-6.18381344106902,9.14149844030021));
#17580=CARTESIAN_POINT('Ctrl Pts',(5.43097866278426,-6.04352201343572,9.1497220410551));
#17581=CARTESIAN_POINT('Ctrl Pts',(5.5456881614843,-5.94043893729674,9.15576456323235));
#17582=CARTESIAN_POINT('Ctrl Pts',(5.65745135058914,-5.83409856845521,9.16180708540961));
#17583=CARTESIAN_POINT('Ctrl Pts',(5.76608602502051,-5.7246781144937,9.16784960758686));
#17584=CARTESIAN_POINT('Ctrl Pts',(5.91393181999677,-5.57576291695406,9.1760731467067));
#17585=CARTESIAN_POINT('Ctrl Pts',(6.05602971023113,-5.42109306343681,9.18429668582654));
#17586=CARTESIAN_POINT('Ctrl Pts',(6.19194133522727,-5.26113581497418,9.19252022494639));
#17587=CARTESIAN_POINT('Ctrl Pts',(6.32782824913167,-5.10120764951486,9.20074226888412));
#17588=CARTESIAN_POINT('Ctrl Pts',(6.4575309518339,-4.93599423248227,9.20896431282186));
#17589=CARTESIAN_POINT('Ctrl Pts',(6.58065047508811,-4.76599694578402,9.2171863567596));
#17590=CARTESIAN_POINT('Ctrl Pts',(6.70375640497549,-4.59601842812757,9.22540749291881));
#17591=CARTESIAN_POINT('Ctrl Pts',(6.82028043358262,-4.42125733406629,9.23362862907802));
#17592=CARTESIAN_POINT('Ctrl Pts',(6.92986565501094,-4.24224581631001,9.24184976523723));
#17593=CARTESIAN_POINT('Ctrl Pts',(7.0394595681963,-4.0632201002467,9.25007155345625));
#17594=CARTESIAN_POINT('Ctrl Pts',(7.14211341829752,-3.87994353705425,9.25829334167527));
#17595=CARTESIAN_POINT('Ctrl Pts',(7.23751463638086,-3.69297569050661,9.26651512989428));
#17596=CARTESIAN_POINT('Ctrl Pts',(7.33291558974847,-3.50600836275037,9.27473689529979));
#17597=CARTESIAN_POINT('Ctrl Pts',(7.4210638197075,-3.31535003606191,9.28295866070529));
#17598=CARTESIAN_POINT('Ctrl Pts',(7.50169333110056,-3.12158368919069,9.2911804261108));
#17599=CARTESIAN_POINT('Ctrl Pts',(7.58233965240079,-2.92777694527071,9.29940390561715));
#17600=CARTESIAN_POINT('Ctrl Pts',(7.65546401033655,-2.73086115905672,9.3076273851235));
#17601=CARTESIAN_POINT('Ctrl Pts',(7.72084864568379,-2.53143906759433,9.31585086462984));
#17602=CARTESIAN_POINT('Ctrl Pts',(7.74726645736075,-2.45086516474235,9.31917345458962));
#17603=CARTESIAN_POINT('Ctrl Pts',(7.77242135098286,-2.36988231555596,9.32249604454938));
#17604=CARTESIAN_POINT('Ctrl Pts',(7.79630126137023,-2.28853101452808,9.32581863450915));
#17605=CARTESIAN_POINT('Ctrl Pts',(7.85540496560554,-2.08718338980453,9.33404217350456));
#17606=CARTESIAN_POINT('Ctrl Pts',(7.90671408272067,-1.88351221563601,9.34226571249997));
#17607=CARTESIAN_POINT('Ctrl Pts',(7.95006562244418,-1.67813711040879,9.35048925149539));
#17608=CARTESIAN_POINT('Ctrl Pts',(7.99340928010374,-1.47279934594789,9.35871129530838));
#17609=CARTESIAN_POINT('Ctrl Pts',(8.02879818718711,-1.26575855719513,9.36693333912137));
#17610=CARTESIAN_POINT('Ctrl Pts',(8.05612024024124,-1.0576456104364,9.37515538293436));
#17611=CARTESIAN_POINT('Ctrl Pts',(8.08343927672539,-0.849555640987154,
9.38337651896891));
#17612=CARTESIAN_POINT('Ctrl Pts',(8.10269319894266,-0.640394042174207,
9.39159765500347));
#17613=CARTESIAN_POINT('Ctrl Pts',(8.11382154309571,-0.430798710880048,
9.39981879103802));
#17614=CARTESIAN_POINT('Ctrl Pts',(8.12495076989518,-0.221186755498332,
9.4080405791333));
#17615=CARTESIAN_POINT('Ctrl Pts',(8.12795311261308,-0.0111412932857755,
9.41626236722859));
#17616=CARTESIAN_POINT('Ctrl Pts',(8.12282014757337,0.198696785772053,9.42448415532387));
#17617=CARTESIAN_POINT('Ctrl Pts',(8.11768719677593,0.408534282598971,9.43270592060643));
#17618=CARTESIAN_POINT('Ctrl Pts',(8.10441899328247,0.618164102644243,9.44092768588898));
#17619=CARTESIAN_POINT('Ctrl Pts',(8.08305921775857,0.826946941894175,9.44914945117154));
#17620=CARTESIAN_POINT('Ctrl Pts',(8.06169498907283,1.03577330893178,9.45737293055691));
#17621=CARTESIAN_POINT('Ctrl Pts',(8.0322358483172,1.24375204896069,9.46559640994228));
#17622=CARTESIAN_POINT('Ctrl Pts',(7.99477730100009,1.45024945092688,9.47381988932766));
#17623=CARTESIAN_POINT('Ctrl Pts',(7.97964265845209,1.53368206083007,9.47714248002892));
#17624=CARTESIAN_POINT('Ctrl Pts',(7.96320273148207,1.61687294099377,9.48046507073018));
#17625=CARTESIAN_POINT('Ctrl Pts',(7.94546619198763,1.69978073717804,9.48378766143144));
#17626=CARTESIAN_POINT('Ctrl Pts',(7.90156757781221,1.90498070631346,9.49201120060057));
#17627=CARTESIAN_POINT('Ctrl Pts',(7.84970833035457,2.10851250470891,9.50023473976971));
#17628=CARTESIAN_POINT('Ctrl Pts',(7.79004015499954,2.30975365482873,9.50845827893885));
#17629=CARTESIAN_POINT('Ctrl Pts',(7.73038282835455,2.5109582158142,9.51668032292581));
#17630=CARTESIAN_POINT('Ctrl Pts',(7.66291949136707,2.70987267714272,9.52490236691278));
#17631=CARTESIAN_POINT('Ctrl Pts',(7.58785195310618,2.90588890018918,9.53312441089974));
#17632=CARTESIAN_POINT('Ctrl Pts',(7.51279270289526,3.10188348149425,9.54134554710802));
#17633=CARTESIAN_POINT('Ctrl Pts',(7.43013103300787,3.29498018804166,9.54956668331629));
#17634=CARTESIAN_POINT('Ctrl Pts',(7.34011751013447,3.48458928712085,9.55778781952457));
#17635=CARTESIAN_POINT('Ctrl Pts',(7.25009684784155,3.67421342503929,9.56600960779198));
#17636=CARTESIAN_POINT('Ctrl Pts',(7.15272329154659,3.86034913519876,9.5742313960594));
#17637=CARTESIAN_POINT('Ctrl Pts',(7.04829459525269,4.04242883190684,9.58245318432682));
#17638=CARTESIAN_POINT('Ctrl Pts',(6.94386618872948,4.22450802337678,9.59067494978027));
#17639=CARTESIAN_POINT('Ctrl Pts',(6.83238283043981,4.40253096940976,9.59889671523371));
#17640=CARTESIAN_POINT('Ctrl Pts',(6.71418733783394,4.57595628857733,9.60711848068715));
#17641=CARTESIAN_POINT('Ctrl Pts',(6.59596720345582,4.74941776400707,9.61534196024041));
#17642=CARTESIAN_POINT('Ctrl Pts',(6.47103230535662,4.91827945395025,9.62356543979366));
#17643=CARTESIAN_POINT('Ctrl Pts',(6.33976837071526,5.08202957175363,9.63178891934692));
#17644=CARTESIAN_POINT('Ctrl Pts',(6.28673288977089,5.14819067134376,9.63511150901586));
#17645=CARTESIAN_POINT('Ctrl Pts',(6.23266469135999,5.21351768872211,9.6384340986848));
#17646=CARTESIAN_POINT('Ctrl Pts',(6.17759109212934,5.27797838769204,9.64175668835373));
#17647=CARTESIAN_POINT('Ctrl Pts',(6.0412817856079,5.43752113225969,9.64998022739884));
#17648=CARTESIAN_POINT('Ctrl Pts',(5.89876649961063,5.59180647339974,9.65820376644395));
#17649=CARTESIAN_POINT('Ctrl Pts',(5.75047503249476,5.74035926255094,9.66642730548906));
#17650=CARTESIAN_POINT('Ctrl Pts',(5.60221052733612,5.88888504223203,9.67464934935233));
#17651=CARTESIAN_POINT('Ctrl Pts',(5.44817214542095,6.03168014155998,9.6828713932156));
#17652=CARTESIAN_POINT('Ctrl Pts',(5.28882691690482,6.1683058780773,9.69109343707887));
#17653=CARTESIAN_POINT('Ctrl Pts',(5.12949928134886,6.30491653004416,9.69931457316416));
#17654=CARTESIAN_POINT('Ctrl Pts',(4.96486619276775,6.43535898718115,9.70753570924944));
#17655=CARTESIAN_POINT('Ctrl Pts',(4.79542879292314,6.55923396857466,9.71575684533473));
#17656=CARTESIAN_POINT('Ctrl Pts',(4.62597795411924,6.68311877513566,9.72397863348098));
#17657=CARTESIAN_POINT('Ctrl Pts',(4.45172227920275,6.8004348889347,9.73220042162723));
#17658=CARTESIAN_POINT('Ctrl Pts',(4.27319385933427,6.91082497268219,9.74042220977348));
#17659=CARTESIAN_POINT('Ctrl Pts',(4.09466593482349,7.02121475013348,9.74864397510696));
#17660=CARTESIAN_POINT('Ctrl Pts',(3.91186554134461,7.12467838315912,9.75686574044044));
#17661=CARTESIAN_POINT('Ctrl Pts',(3.72535191994056,7.22090303459998,9.76508750577393));
#17662=CARTESIAN_POINT('Ctrl Pts',(3.53879941351825,7.31714774729588,9.77331098521008));
#17663=CARTESIAN_POINT('Ctrl Pts',(3.34853239480094,7.40615032819317,9.78153446464623));
#17664=CARTESIAN_POINT('Ctrl Pts',(3.15513374641341,7.48764439625329,9.78975794408238));
#17665=CARTESIAN_POINT('Ctrl Pts',(3.07699352643903,7.52057101936011,9.79308053448026));
#17666=CARTESIAN_POINT('Ctrl Pts',(2.9983423235223,7.55227245004202,9.79640312487814));
#17667=CARTESIAN_POINT('Ctrl Pts',(2.91921950827881,7.58273334787558,9.79972571527602));
#17668=CARTESIAN_POINT('Ctrl Pts',(2.7233875024442,7.6581252396316,9.80794925408946));
#17669=CARTESIAN_POINT('Ctrl Pts',(2.5246015167032,7.72593897414762,9.8161727929029));
#17670=CARTESIAN_POINT('Ctrl Pts',(2.32346574288007,7.78596137314865,9.82439633171635));
#17671=CARTESIAN_POINT('Ctrl Pts',(2.12236653907767,7.84597285902202,9.83261837534582));
#17672=CARTESIAN_POINT('Ctrl Pts',(1.91891868238004,7.89819575245895,9.84084041897529));
#17673=CARTESIAN_POINT('Ctrl Pts',(1.71374174143379,7.94246667013262,9.84906246260476));
#17674=CARTESIAN_POINT('Ctrl Pts',(1.50858745366323,7.9867326999428,9.85728359845484));
#17675=CARTESIAN_POINT('Ctrl Pts',(1.30170475096606,8.02304844462583,9.86550473430492));
#17676=CARTESIAN_POINT('Ctrl Pts',(1.09372443731284,8.05130141143186,9.873725870155));
#17677=CARTESIAN_POINT('Ctrl Pts',(0.885727627668747,8.07955661912634,9.88194765806574));
#17678=CARTESIAN_POINT('Ctrl Pts',(0.676633325022578,8.09974772883555,9.89016944597649));
#17679=CARTESIAN_POINT('Ctrl Pts',(0.467079577523585,8.11181386810375,9.89839123388723));
#17680=CARTESIAN_POINT('Ctrl Pts',(0.257526411458404,8.12387997389291,9.90661299898557));
#17681=CARTESIAN_POINT('Ctrl Pts',(0.0475140976898377,8.12782114007451,
9.91483476408391));
#17682=CARTESIAN_POINT('Ctrl Pts',(-0.162316629894777,8.12362855343347,
9.92305652918225));
#17683=CARTESIAN_POINT('Ctrl Pts',(-0.372191103778895,8.11943509270619,
9.93128000838511));
#17684=CARTESIAN_POINT('Ctrl Pts',(-0.581883620923186,8.10710449741623,
9.93950348758796));
#17685=CARTESIAN_POINT('Ctrl Pts',(-0.79075477812074,8.08668006312722,9.94772696679081));
#17686=CARTESIAN_POINT('Ctrl Pts',(-0.875146503029868,8.07842783116245,
9.95104955859331));
#17687=CARTESIAN_POINT('Ctrl Pts',(-0.959404188540645,8.06885490375017,
9.95437215039581));
#17688=CARTESIAN_POINT('Ctrl Pts',(-1.04348590916689,8.05796653752484,9.95769474219831));
#17689=CARTESIAN_POINT('Ctrl Pts',(-1.25159134012213,8.03101742029885,9.96591828227097));
#17690=CARTESIAN_POINT('Ctrl Pts',(-1.45868603051667,7.99599780690685,9.97414182234363));
#17691=CARTESIAN_POINT('Ctrl Pts',(-1.66413717105161,7.95300792395081,9.98236536241628));
#17692=CARTESIAN_POINT('Ctrl Pts',(-1.86955095712071,7.91002585727707,9.99058740731132));
#17693=CARTESIAN_POINT('Ctrl Pts',(-2.07332150121117,7.85907647371045,9.99880945220635));
#17694=CARTESIAN_POINT('Ctrl Pts',(-2.27482618222162,7.80031110938397,10.0070314971014));
#17695=CARTESIAN_POINT('Ctrl Pts',(-2.47630861555574,7.74155223320853,10.015252634219));
#17696=CARTESIAN_POINT('Ctrl Pts',(-2.6755254022331,7.67497918165133,10.0234737713367));
#17697=CARTESIAN_POINT('Ctrl Pts',(-2.87186827291337,7.60079339184625,10.0316949084543));
#17698=CARTESIAN_POINT('Ctrl Pts',(-3.06822671641337,7.52660171803872,10.0399166976267));
#17699=CARTESIAN_POINT('Ctrl Pts',(-3.26171051162318,7.44479620130437,10.048138486799));
#17700=CARTESIAN_POINT('Ctrl Pts',(-3.45172959808347,7.35562712106959,10.0563602759713));
#17701=CARTESIAN_POINT('Ctrl Pts',(-3.64174815717429,7.26645828831022,10.0645820423253));
#17702=CARTESIAN_POINT('Ctrl Pts',(-3.82830176090006,7.16992606066323,10.0728038086793));
#17703=CARTESIAN_POINT('Ctrl Pts',(-4.0108227752078,7.06632777532817,10.0810255750332));
#17704=CARTESIAN_POINT('Ctrl Pts',(-4.19338184180514,6.96270789164746,10.089249055475));
#17705=CARTESIAN_POINT('Ctrl Pts',(-4.37190638292323,6.85201915297229,10.0974725359167));
#17706=CARTESIAN_POINT('Ctrl Pts',(-4.54585474639135,6.73460408540927,10.1056960163584));
#17707=CARTESIAN_POINT('Ctrl Pts',(-4.61613619201214,6.68716414104035,10.1090186006125));
#17708=CARTESIAN_POINT('Ctrl Pts',(-4.68567091912808,6.63862665464677,10.1123411848665));
#17709=CARTESIAN_POINT('Ctrl Pts',(-4.75442456323019,6.58901621147296,10.1156637691206));
#17710=CARTESIAN_POINT('Ctrl Pts',(-4.92459274213244,6.46622826503502,10.1238873057658));
#17711=CARTESIAN_POINT('Ctrl Pts',(-5.09002932993603,6.33682469759667,10.1321108424109));
#17712=CARTESIAN_POINT('Ctrl Pts',(-5.25022558127162,6.20119495809164,10.1403343790561));
#17713=CARTESIAN_POINT('Ctrl Pts',(-5.41039270596633,6.06558987858133,10.1485564205103));
#17714=CARTESIAN_POINT('Ctrl Pts',(-5.56532117086996,5.92376107689451,10.1567784619644));
#17715=CARTESIAN_POINT('Ctrl Pts',(-5.71453552566292,5.77613809464736,10.1650005034185));
#17716=CARTESIAN_POINT('Ctrl Pts',(-5.86373340599093,5.62853141116482,10.1732216370932));
#17717=CARTESIAN_POINT('Ctrl Pts',(-6.00721822616031,5.47513203165639,10.1814427707678));
#17718=CARTESIAN_POINT('Ctrl Pts',(-6.14455101197339,5.31640672106233,10.1896639044424));
#17719=CARTESIAN_POINT('Ctrl Pts',(-6.28189469062889,5.1576688208322,10.1978856901938));
#17720=CARTESIAN_POINT('Ctrl Pts',(-6.41308516494823,4.99360436675842,10.2061074759451));
#17721=CARTESIAN_POINT('Ctrl Pts',(-6.53772272932725,4.82471440366555,10.2143292616965));
#17722=CARTESIAN_POINT('Ctrl Pts',(-6.66235994808432,4.65582490890724,10.2225510246487));
#17723=CARTESIAN_POINT('Ctrl Pts',(-6.78044412029115,4.48211017080621,10.2307727876009));
#17724=CARTESIAN_POINT('Ctrl Pts',(-6.89161766797295,4.3041019366394,10.2389945505531));
#17725=CARTESIAN_POINT('Ctrl Pts',(-7.00281439398958,4.12605658991714,10.2472180276431));
#17726=CARTESIAN_POINT('Ctrl Pts',(-7.10709746095352,3.94371620909176,10.2554415047331));
#17727=CARTESIAN_POINT('Ctrl Pts',(-7.20415365520637,3.75763990753195,10.263664981823));
#17728=CARTESIAN_POINT('Ctrl Pts',(-7.2433681343784,3.68245784101783,10.266987586563));
#17729=CARTESIAN_POINT('Ctrl Pts',(-7.28140336517111,3.6066661814362,10.2703101913029));
#17730=CARTESIAN_POINT('Ctrl Pts',(-7.31824083470849,3.53030291160762,10.2736327960429));
#17731=CARTESIAN_POINT('Ctrl Pts',(-7.40911983224593,3.34191273449019,10.2818297485419));
#17732=CARTESIAN_POINT('Ctrl Pts',(-7.49273708782956,3.14997699955855,10.2900267010408));
#17733=CARTESIAN_POINT('Ctrl Pts',(-7.56883154281126,2.9550764184781,10.2982236535398));
#17734=CARTESIAN_POINT('Ctrl Pts',(-7.64491133611954,2.76021339031354,10.3064190266722));
#17735=CARTESIAN_POINT('Ctrl Pts',(-7.71347111297681,2.56238693425361,10.3146143998045));
#17736=CARTESIAN_POINT('Ctrl Pts',(-7.77429815698699,2.36219722478219,10.3228097729369));
#17737=CARTESIAN_POINT('Ctrl Pts',(-7.83512569348692,2.16200589446299,10.3310052124236));
#17738=CARTESIAN_POINT('Ctrl Pts',(-7.8882202811252,1.95945155713435,10.3392006519102));
#17739=CARTESIAN_POINT('Ctrl Pts',(-7.93341893815651,1.75514999763543,10.3473960913969));
#17740=CARTESIAN_POINT('Ctrl Pts',(-7.97861499566341,1.55086018819557,10.3555910595368));
#17741=CARTESIAN_POINT('Ctrl Pts',(-8.01591596665708,1.34482364940534,10.3637860276766));
#17742=CARTESIAN_POINT('Ctrl Pts',(-8.04520979307792,1.13766732741303,10.3719809958164));
#17743=CARTESIAN_POINT('Ctrl Pts',(-8.07451001198787,0.930465799836723,
10.3801777522595));
#17744=CARTESIAN_POINT('Ctrl Pts',(-8.09579955145645,0.722144296566263,
10.3883745087025));
#17745=CARTESIAN_POINT('Ctrl Pts',(-8.10901798322321,0.513337033792121,
10.3965712651456));
#17746=CARTESIAN_POINT('Ctrl Pts',(-8.11983950377611,0.342392997043054,
10.4032816956929));
#17747=CARTESIAN_POINT('Ctrl Pts',(-8.12525256763878,0.171123594131868,
10.4099921262403));
#17748=CARTESIAN_POINT('Ctrl Pts',(-8.125249999086,-0.000121872618778703,
10.4167025567876));
#17749=CARTESIAN_POINT('Origin',(0.,0.,-16.4167025567876));
#17750=CARTESIAN_POINT('',(4.94675008185378,-6.44587862049694,7.1250592150305));
#17751=CARTESIAN_POINT('',(4.94684221335274,-6.44599857519204,7.2916588140437));
#17752=CARTESIAN_POINT('',(4.94675008185374,-6.44587862049697,-16.4167025567876));
#17753=CARTESIAN_POINT('',(-8.12524999873121,0.000143591189764823,8.58329744321241));
#17754=CARTESIAN_POINT('Ctrl Pts',(4.94684221335274,-6.44599857519204,7.2916588140437));
#17755=CARTESIAN_POINT('Ctrl Pts',(5.8049765999933,-5.78602921714794,7.33407194911367));
#17756=CARTESIAN_POINT('Ctrl Pts',(7.43356999167247,-3.92084680041933,7.42914142649105));
#17757=CARTESIAN_POINT('Ctrl Pts',(8.46465994169792,-0.171018365282867,
7.57686724617588));
#17758=CARTESIAN_POINT('Ctrl Pts',(7.52493661231736,3.8800830133467,7.73483627309817));
#17759=CARTESIAN_POINT('Ctrl Pts',(4.76963640343018,6.99501849808588,7.89280530002046));
#17760=CARTESIAN_POINT('Ctrl Pts',(0.863543566747498,8.42223294139058,8.05077432694274));
#17761=CARTESIAN_POINT('Ctrl Pts',(-3.25090049128004,7.81737559566535,8.20874335386504));
#17762=CARTESIAN_POINT('Ctrl Pts',(-6.58098448454454,5.32638324072316,8.36671238078732));
#17763=CARTESIAN_POINT('Ctrl Pts',(-7.95798473996769,2.34191872576517,8.49156374016535));
#17764=CARTESIAN_POINT('Ctrl Pts',(-8.12506463397728,0.498971488914468,
8.56375875723593));
#17765=CARTESIAN_POINT('Ctrl Pts',(-8.12474591487583,0.000143868560570458,
8.58329743199909));
#17766=CARTESIAN_POINT('Ctrl Pts',(-8.12524999873121,0.000143591189764823,
8.58329744321241));
#17767=CARTESIAN_POINT('Ctrl Pts',(-8.12525373444067,-0.211245236214326,
8.59157685916403));
#17768=CARTESIAN_POINT('Ctrl Pts',(-8.11700370973027,-0.422638087073884,
8.59985627511566));
#17769=CARTESIAN_POINT('Ctrl Pts',(-8.10052557183335,-0.633382208918111,
8.60813569106728));
#17770=CARTESIAN_POINT('Ctrl Pts',(-8.08412976794414,-0.843073335074187,
8.61637373841882));
#17771=CARTESIAN_POINT('Ctrl Pts',(-8.05958793823209,-1.05212190871435,
8.62461178577036));
#17772=CARTESIAN_POINT('Ctrl Pts',(-8.0269774401061,-1.25988917708176,8.6328498331219));
#17773=CARTESIAN_POINT('Ctrl Pts',(-7.99412130416121,-1.46922144756729,
8.64114993337356));
#17774=CARTESIAN_POINT('Ctrl Pts',(-7.95307447349202,-1.67725273047273,
8.64945003362523));
#17775=CARTESIAN_POINT('Ctrl Pts',(-7.90396883610218,-1.88333857827675,
8.6577501338769));
#17776=CARTESIAN_POINT('Ctrl Pts',(-7.85486319871234,-2.08942442608081,
8.66605023412856));
#17777=CARTESIAN_POINT('Ctrl Pts',(-7.79769883263737,-2.29356454561377,
8.67435033438023));
#17778=CARTESIAN_POINT('Ctrl Pts',(-7.73265961988368,-2.49512780544812,
8.6826504346319));
#17779=CARTESIAN_POINT('Ctrl Pts',(-7.66822033769495,-2.6948318182955,8.69087397362733));
#17780=CARTESIAN_POINT('Ctrl Pts',(-7.59603010807265,-2.89207061628817,
8.69909751262277));
#17781=CARTESIAN_POINT('Ctrl Pts',(-7.51630285168063,-3.08624027002397,
8.7073210516182));
#17782=CARTESIAN_POINT('Ctrl Pts',(-7.43659009109071,-3.28037462033905,
8.71554309543119));
#17783=CARTESIAN_POINT('Ctrl Pts',(-7.3493431507886,-3.47144066745328,8.72376513924418));
#17784=CARTESIAN_POINT('Ctrl Pts',(-7.2548243468166,-3.65885381770537,8.73198718305717));
#17785=CARTESIAN_POINT('Ctrl Pts',(-7.16031597846581,-3.84624627606796,
8.7402083190917));
#17786=CARTESIAN_POINT('Ctrl Pts',(-7.058537482107,-4.02998637952217,8.74842945512621));
#17787=CARTESIAN_POINT('Ctrl Pts',(-6.94979781843153,-4.20951278005239,
8.75665059116074));
#17788=CARTESIAN_POINT('Ctrl Pts',(-6.84104953005183,-4.38905341974846,
8.76487237925602));
#17789=CARTESIAN_POINT('Ctrl Pts',(-6.72533912169375,-4.56437943508953,
8.77309416735129));
#17790=CARTESIAN_POINT('Ctrl Pts',(-6.60302025785466,-4.73495628668956,
8.78131595544657));
#17791=CARTESIAN_POINT('Ctrl Pts',(-6.48070173341022,-4.90553266499488,
8.78953772072908));
#17792=CARTESIAN_POINT('Ctrl Pts',(-6.35177496422567,-5.07135966781209,
8.79775948601159));
#17793=CARTESIAN_POINT('Ctrl Pts',(-6.21663579505286,-5.2319333858687,8.80598125129411));
#17794=CARTESIAN_POINT('Ctrl Pts',(-6.08146845158538,-5.39254058090519,
8.81420473067949));
#17795=CARTESIAN_POINT('Ctrl Pts',(-5.94008631066937,-5.54789207754479,
8.82242821006488));
#17796=CARTESIAN_POINT('Ctrl Pts',(-5.79292491153289,-5.69751775177942,
8.83065168945026));
#17797=CARTESIAN_POINT('Ctrl Pts',(-5.73346624769379,-5.75797207416436,
8.83397428015158));
#17798=CARTESIAN_POINT('Ctrl Pts',(-5.67306457586728,-5.81749208577385,
8.83729687085289));
#17799=CARTESIAN_POINT('Ctrl Pts',(-5.611750334763,-5.87604848029587,8.8406194615542));
#17800=CARTESIAN_POINT('Ctrl Pts',(-5.45999524102061,-6.02097779818127,
8.84884300072332));
#17801=CARTESIAN_POINT('Ctrl Pts',(-5.30259807197871,-6.16004866386615,
8.85706653989244));
#17802=CARTESIAN_POINT('Ctrl Pts',(-5.14003450407988,-6.29283186326858,
8.86529007906155));
#17803=CARTESIAN_POINT('Ctrl Pts',(-4.97750049305847,-6.42559092038131,
8.87351212304855));
#17804=CARTESIAN_POINT('Ctrl Pts',(-4.80980218630475,-6.55206440643836,
8.88173416703556));
#17805=CARTESIAN_POINT('Ctrl Pts',(-4.63744861058498,-6.67186315407349,
8.88995621102256));
#17806=CARTESIAN_POINT('Ctrl Pts',(-4.46511406406289,-6.79164867497955,
8.89817734723088));
#17807=CARTESIAN_POINT('Ctrl Pts',(-4.28812551679848,-6.90476076047794,
8.9063984834392));
#17808=CARTESIAN_POINT('Ctrl Pts',(-4.10702194464438,-7.01085289452784,
8.91461961964752));
#17809=CARTESIAN_POINT('Ctrl Pts',(-3.92590400826825,-7.11695344327079,
8.92284140791492));
#17810=CARTESIAN_POINT('Ctrl Pts',(-3.74067064801074,-7.21603277668371,
8.93106319618231));
#17811=CARTESIAN_POINT('Ctrl Pts',(-3.55188738558178,-7.30778923906848,
8.9392849844497));
#17812=CARTESIAN_POINT('Ctrl Pts',(-3.36310464699317,-7.3995454468452,8.94750674990307));
#17813=CARTESIAN_POINT('Ctrl Pts',(-3.17077229237575,-7.4839786977384,8.95572851535645));
#17814=CARTESIAN_POINT('Ctrl Pts',(-2.97547835057054,-7.56083435526702,
8.96395028080983));
#17815=CARTESIAN_POINT('Ctrl Pts',(-2.78014369326115,-7.63770603590836,
8.9721737603631));
#17816=CARTESIAN_POINT('Ctrl Pts',(-2.58184648978833,-7.70699685917193,
8.98039723991638));
#17817=CARTESIAN_POINT('Ctrl Pts',(-2.38119358789019,-7.76850079870567,
8.98862071946965));
#17818=CARTESIAN_POINT('Ctrl Pts',(-2.30012239964538,-7.79335066338527,
8.9919433091386));
#17819=CARTESIAN_POINT('Ctrl Pts',(-2.21866684018557,-7.81692991511405,
8.99526589880754));
#17820=CARTESIAN_POINT('Ctrl Pts',(-2.13686763041389,-7.83922727649794,
8.99858848847649));
#17821=CARTESIAN_POINT('Ctrl Pts',(-1.93441139523571,-7.8944141157448,9.0068120275216));
#17822=CARTESIAN_POINT('Ctrl Pts',(-1.72978324732373,-7.94176276214306,
9.01503556656671));
#17823=CARTESIAN_POINT('Ctrl Pts',(-1.52360585017358,-7.98112227545831,
9.02325910561183));
#17824=CARTESIAN_POINT('Ctrl Pts',(-1.31746593964419,-8.02047463253253,
9.03148114947515));
#17825=CARTESIAN_POINT('Ctrl Pts',(-1.10977763163798,-8.05184070039555,
9.03970319333847));
#17826=CARTESIAN_POINT('Ctrl Pts',(-0.901173848330154,-8.07512063424354,
9.04792523720179));
#17827=CARTESIAN_POINT('Ctrl Pts',(-0.692593096515015,-8.09839799780437,
9.05614637328703));
#17828=CARTESIAN_POINT('Ctrl Pts',(-0.483097364193052,-8.11359097703911,
9.06436750937227));
#17829=CARTESIAN_POINT('Ctrl Pts',(-0.273325601106056,-8.12065149346282,
9.07258864545751));
#17830=CARTESIAN_POINT('Ctrl Pts',(-0.0635371999307712,-8.12771256989277,
9.08081043360376));
#17831=CARTESIAN_POINT('Ctrl Pts',(0.146526981067496,-8.1266398821167,9.08903222175));
#17832=CARTESIAN_POINT('Ctrl Pts',(0.356226009082313,-8.11743744003939,
9.09725400989625));
#17833=CARTESIAN_POINT('Ctrl Pts',(0.565924455252275,-8.10823502349579,
9.10547577522978));
#17834=CARTESIAN_POINT('Ctrl Pts',(0.775257455935232,-8.09090291339795,
9.11369754056332));
#17835=CARTESIAN_POINT('Ctrl Pts',(0.983586674719125,-8.06549718342366,
9.12191930589685));
#17836=CARTESIAN_POINT('Ctrl Pts',(1.19195932671374,-8.04008615677312,9.13014278533304));
#17837=CARTESIAN_POINT('Ctrl Pts',(1.39932748592745,-8.00659818337073,9.13836626476921));
#17838=CARTESIAN_POINT('Ctrl Pts',(1.60505941315471,-7.96514104349342,9.14658974420539));
#17839=CARTESIAN_POINT('Ctrl Pts',(1.68818273476456,-7.94839082286656,9.14991233460318));
#17840=CARTESIAN_POINT('Ctrl Pts',(1.7710390522369,-7.93034025273445,9.15323492500098));
#17841=CARTESIAN_POINT('Ctrl Pts',(1.85358718734214,-7.91099880555047,9.15655751539878));
#17842=CARTESIAN_POINT('Ctrl Pts',(2.05789534233786,-7.86312836748343,9.16478098783841));
#17843=CARTESIAN_POINT('Ctrl Pts',(2.26038124965037,-7.80733128189522,9.17300446027803));
#17844=CARTESIAN_POINT('Ctrl Pts',(2.46042550664494,-7.74377129625811,9.18122793271765));
#17845=CARTESIAN_POINT('Ctrl Pts',(2.66043274840183,-7.68022307145837,9.18944988352506));
#17846=CARTESIAN_POINT('Ctrl Pts',(2.85799896066828,-7.60891490290157,9.19767183433247));
#17847=CARTESIAN_POINT('Ctrl Pts',(3.05252005421146,-7.53006035043126,9.20589378513987));
#17848=CARTESIAN_POINT('Ctrl Pts',(3.24703585258523,-7.4512079445056,9.21411551213287));
#17849=CARTESIAN_POINT('Ctrl Pts',(3.43850642331368,-7.36480967276742,9.22233723912587));
#17850=CARTESIAN_POINT('Ctrl Pts',(3.62634687940736,-7.27112755167398,9.23055896611887));
#17851=CARTESIAN_POINT('Ctrl Pts',(3.81417466180681,-7.17745175136246,9.23878013838763));
#17852=CARTESIAN_POINT('Ctrl Pts',(3.99837255546468,-7.07649321608515,9.2470013106564));
#17853=CARTESIAN_POINT('Ctrl Pts',(4.17837898390298,-6.96856058518385,9.25522248292517));
#17854=CARTESIAN_POINT('Ctrl Pts',(4.35840773699178,-6.86061456832582,9.26344467479528));
#17855=CARTESIAN_POINT('Ctrl Pts',(4.53424373298925,-6.74569287891959,9.27166686666539));
#17856=CARTESIAN_POINT('Ctrl Pts',(4.70535225921246,-6.62414882677195,9.2798890585355));
#17857=CARTESIAN_POINT('Ctrl Pts',(4.78691031392296,-6.56621543985316,9.28380812668006));
#17858=CARTESIAN_POINT('Ctrl Pts',(4.86739475154616,-6.50677815177985,9.28772719482462));
#17859=CARTESIAN_POINT('Ctrl Pts',(4.94675008185378,-6.44587862049695,9.29164626296917));
#17860=CARTESIAN_POINT('',(-8.12524999739701,0.000205669423076638,8.41670255675951));
#17861=CARTESIAN_POINT('Ctrl Pts',(-8.12524999739703,0.000205668705097187,
8.41670255678763));
#17862=CARTESIAN_POINT('Ctrl Pts',(-8.12525529312676,-0.209010060191446,
8.42489859465923));
#17863=CARTESIAN_POINT('Ctrl Pts',(-8.11717565384267,-0.418248871417476,
8.43309463253084));
#17864=CARTESIAN_POINT('Ctrl Pts',(-8.10103180470332,-0.626874199249931,
8.44129067040245));
#17865=CARTESIAN_POINT('Ctrl Pts',(-8.08488735073895,-0.835507343174935,
8.44948701533644));
#17866=CARTESIAN_POINT('Ctrl Pts',(-8.06067810215077,-1.04352665968774,
8.45768336027043));
#17867=CARTESIAN_POINT('Ctrl Pts',(-8.02847678956486,-1.25029916496744,
8.46587970520442));
#17868=CARTESIAN_POINT('Ctrl Pts',(-7.99627686368355,-1.45706276587775,
8.47407569717425));
#17869=CARTESIAN_POINT('Ctrl Pts',(-7.95608560916812,-1.6625793679671,8.48227168914408));
#17870=CARTESIAN_POINT('Ctrl Pts',(-7.90802724461236,-1.86622417221745,
8.49046768111391));
#17871=CARTESIAN_POINT('Ctrl Pts',(-7.85995700677275,-2.06991928888659,
8.49866569798284));
#17872=CARTESIAN_POINT('Ctrl Pts',(-7.80401584222756,-2.27174139244837,
8.50686371485177));
#17873=CARTESIAN_POINT('Ctrl Pts',(-7.74037870259076,-2.47107772095079,
8.5150617317207));
#17874=CARTESIAN_POINT('Ctrl Pts',(-7.68626947378545,-2.64056891853931,
8.52203232111304));
#17875=CARTESIAN_POINT('Ctrl Pts',(-7.62659715252873,-2.80826308622982,
8.52900291050538));
#17876=CARTESIAN_POINT('Ctrl Pts',(-7.56149739431627,-2.97379298510308,
8.53597349989771));
#17877=CARTESIAN_POINT('Ctrl Pts',(-7.48469608310022,-3.16907655647114,
8.54419703897036));
#17878=CARTESIAN_POINT('Ctrl Pts',(-7.40031315177781,-3.36141504559831,
8.552420578043));
#17879=CARTESIAN_POINT('Ctrl Pts',(-7.30859986802793,-3.55021908219227,
8.56064411711565));
#17880=CARTESIAN_POINT('Ctrl Pts',(-7.21690325934615,-3.73898879093273,
8.56886616100604));
#17881=CARTESIAN_POINT('Ctrl Pts',(-7.1178790871281,-3.92422506458559,8.57708820489644));
#17882=CARTESIAN_POINT('Ctrl Pts',(-7.0118257105885,-4.10536085707822,8.58531024878684));
#17883=CARTESIAN_POINT('Ctrl Pts',(-6.90578404317839,-4.28647665075028,
8.59353138489872));
#17884=CARTESIAN_POINT('Ctrl Pts',(-6.79271486982163,-4.46349261269185,
8.60175252101061));
#17885=CARTESIAN_POINT('Ctrl Pts',(-6.67296164946673,-4.63586781382367,
8.60997365712249));
#17886=CARTESIAN_POINT('Ctrl Pts',(-6.55319893087479,-4.80825668690949,
8.61819544529449));
#17887=CARTESIAN_POINT('Ctrl Pts',(-6.42675127210854,-4.97600381998557,
8.62641723346649));
#17888=CARTESIAN_POINT('Ctrl Pts',(-6.29400507200062,-5.13859783560948,
8.63463902163849));
#17889=CARTESIAN_POINT('Ctrl Pts',(-6.16125924022752,-5.30119140007895,
8.64286078699726));
#17890=CARTESIAN_POINT('Ctrl Pts',(-6.02221509068316,-5.45863164894251,
8.65108255235602));
#17891=CARTESIAN_POINT('Ctrl Pts',(-5.87729920450196,-5.61044041259335,
8.65930431771478));
#17892=CARTESIAN_POINT('Ctrl Pts',(-5.73235310576378,-5.76228082585171,
8.66752779717516));
#17893=CARTESIAN_POINT('Ctrl Pts',(-5.58153302855493,-5.90848719506552,
8.67575127663554));
#17894=CARTESIAN_POINT('Ctrl Pts',(-5.42530305809643,-6.04861755199562,
8.68397475609592));
#17895=CARTESIAN_POINT('Ctrl Pts',(-5.36218036438097,-6.10523540563009,
8.68729734633727));
#17896=CARTESIAN_POINT('Ctrl Pts',(-5.29817493400528,-6.16086180795296,
8.69061993657863));
#17897=CARTESIAN_POINT('Ctrl Pts',(-5.23331897871228,-6.2154694134514,8.69394252681999));
#17898=CARTESIAN_POINT('Ctrl Pts',(-5.07279798642728,-6.35062534448837,
8.70216606589345));
#17899=CARTESIAN_POINT('Ctrl Pts',(-4.9070123093046,-6.47958147178438,8.71038960496692));
#17900=CARTESIAN_POINT('Ctrl Pts',(-4.7364635329758,-6.60193916688804,8.71861314404039));
#17901=CARTESIAN_POINT('Ctrl Pts',(-4.56594576537733,-6.72427461523712,
8.72683518793159));
#17902=CARTESIAN_POINT('Ctrl Pts',(-4.39066686656009,-6.84001385403544,
8.73505723182279));
#17903=CARTESIAN_POINT('Ctrl Pts',(-4.21115920295708,-6.94880030867558,
8.74327927571399));
#17904=CARTESIAN_POINT('Ctrl Pts',(-4.03167135841674,-7.05757475243263,
8.75150041182666));
#17905=CARTESIAN_POINT('Ctrl Pts',(-3.84795593335041,-7.15939779180149,
8.75972154793934));
#17906=CARTESIAN_POINT('Ctrl Pts',(-3.66057251753701,-7.25395729284042,
8.76794268405202));
#17907=CARTESIAN_POINT('Ctrl Pts',(-3.47317423939208,-7.34852429387421,
8.7761644722248));
#17908=CARTESIAN_POINT('Ctrl Pts',(-3.28210765132299,-7.43582647021802,
8.78438626039758));
#17909=CARTESIAN_POINT('Ctrl Pts',(-3.08795603174893,-7.51559812047487,
8.79260804857036));
#17910=CARTESIAN_POINT('Ctrl Pts',(-2.89380495089375,-7.5953695493867,8.80082981392988));
#17911=CARTESIAN_POINT('Ctrl Pts',(-2.6965691294845,-7.66761038441627,8.80905157928939));
#17912=CARTESIAN_POINT('Ctrl Pts',(-2.49685136875701,-7.73210325880586,
8.81727334464891));
#17913=CARTESIAN_POINT('Ctrl Pts',(-2.29709197019225,-7.79660957888901,
8.82549682411));
#17914=CARTESIAN_POINT('Ctrl Pts',(-2.09484987931887,-7.85336462073605,
8.83372030357109));
#17915=CARTESIAN_POINT('Ctrl Pts',(-1.89074363968878,-7.90220070938953,
8.84194378303218));
#17916=CARTESIAN_POINT('Ctrl Pts',(-1.80827716035315,-7.9219322977186,8.84526637326888));
#17917=CARTESIAN_POINT('Ctrl Pts',(-1.72550651753203,-7.9403717234113,8.84858896350558));
#17918=CARTESIAN_POINT('Ctrl Pts',(-1.64247305766683,-7.95751027755155,
8.85191155374228));
#17919=CARTESIAN_POINT('Ctrl Pts',(-1.43696203959017,-7.99992886055946,
8.86013509282285));
#17920=CARTESIAN_POINT('Ctrl Pts',(-1.22977350723855,-8.0343887741463,8.86835863190342));
#17921=CARTESIAN_POINT('Ctrl Pts',(-1.02153834427083,-8.06077831066482,
8.87658217098399));
#17922=CARTESIAN_POINT('Ctrl Pts',(-0.813341042072039,-8.08716304910731,
8.88480421488234));
#17923=CARTESIAN_POINT('Ctrl Pts',(-0.604097781515014,-8.10548030205177,
8.89302625878069));
#17924=CARTESIAN_POINT('Ctrl Pts',(-0.394446489696768,-8.11566999879036,
8.90124830267904));
#17925=CARTESIAN_POINT('Ctrl Pts',(-0.184818345032949,-8.12585857050614,
8.90946943879896));
#17926=CARTESIAN_POINT('Ctrl Pts',(0.0252174464794002,-8.12792136322245,
8.91769057491888));
#17927=CARTESIAN_POINT('Ctrl Pts',(0.23502017909011,-8.12185034816084,8.9259117110388));
#17928=CARTESIAN_POINT('Ctrl Pts',(0.444839552220188,-8.11577885157623,
8.93413349921875));
#17929=CARTESIAN_POINT('Ctrl Pts',(0.654425534617284,-8.10157226405988,
8.9423552873987));
#17930=CARTESIAN_POINT('Ctrl Pts',(0.863138698604562,-8.07927466728736,
8.95057707557865));
#17931=CARTESIAN_POINT('Ctrl Pts',(1.07185128346766,-8.05697713238481,8.9587988409453));
#17932=CARTESIAN_POINT('Ctrl Pts',(1.27969076178868,-8.02658866714655,8.96702060631194));
#17933=CARTESIAN_POINT('Ctrl Pts',(1.48602355292116,-7.98820515276514,8.97524237167858));
#17934=CARTESIAN_POINT('Ctrl Pts',(1.69239936101312,-7.94981363605858,8.98346585114673));
#17935=CARTESIAN_POINT('Ctrl Pts',(1.89726756438602,-7.90342379430053,8.99168933061488));
#17936=CARTESIAN_POINT('Ctrl Pts',(2.10000440007057,-7.84918270154188,8.99991281008302));
#17937=CARTESIAN_POINT('Ctrl Pts',(2.18191758837314,-7.82726729169603,9.00323540027687));
#17938=CARTESIAN_POINT('Ctrl Pts',(2.26348298004169,-7.80407077408141,9.00655799047072));
#17939=CARTESIAN_POINT('Ctrl Pts',(2.34466006978829,-7.77960517761926,9.00988058066456));
#17940=CARTESIAN_POINT('Ctrl Pts',(2.54557448666919,-7.71905248889661,9.01810403722619));
#17941=CARTESIAN_POINT('Ctrl Pts',(2.74417455196863,-7.65070264728471,9.02632749378782));
#17942=CARTESIAN_POINT('Ctrl Pts',(2.93985231848861,-7.57475781183644,9.03455095034945));
#17943=CARTESIAN_POINT('Ctrl Pts',(3.13550499087003,-7.49882271571756,9.04277335231728));
#17944=CARTESIAN_POINT('Ctrl Pts',(3.32823583684251,-7.41529467444085,9.05099575428512));
#17945=CARTESIAN_POINT('Ctrl Pts',(3.51745520753185,-7.32442464808718,9.05921815625295));
#17946=CARTESIAN_POINT('Ctrl Pts',(3.70664939863717,-7.2335667138859,9.0674394640587));
#17947=CARTESIAN_POINT('Ctrl Pts',(3.89233278190311,-7.13536887353303,9.07566077186445));
#17948=CARTESIAN_POINT('Ctrl Pts',(4.07393808722629,-7.03012916125635,9.0838820796702));
#17949=CARTESIAN_POINT('Ctrl Pts',(4.25555288501596,-6.92488394812473,9.09210381720177));
#17950=CARTESIAN_POINT('Ctrl Pts',(4.43308892276975,-6.81259627380045,9.10032555473332));
#17951=CARTESIAN_POINT('Ctrl Pts',(4.606004912716,-6.69360936315648,9.10854729226489));
#17952=CARTESIAN_POINT('Ctrl Pts',(4.72170617580161,-6.61399303700617,9.1140486077734));
#17953=CARTESIAN_POINT('Ctrl Pts',(4.83533949743165,-6.53137826299053,9.11954992328192));
#17954=CARTESIAN_POINT('Ctrl Pts',(4.94675008185374,-6.44587862049698,9.12505123879043));
#17955=CARTESIAN_POINT('Ctrl Pts',(4.94675008185378,-6.44587862049694,7.1250592150305));
#17956=CARTESIAN_POINT('Ctrl Pts',(5.11322900588198,-6.31811797225193,7.1332820268424));
#17957=CARTESIAN_POINT('Ctrl Pts',(5.27477905707631,-6.18388645837806,7.1415048386543));
#17958=CARTESIAN_POINT('Ctrl Pts',(5.43090386575413,-6.04358922854928,7.1497276504662));
#17959=CARTESIAN_POINT('Ctrl Pts',(5.5870051723591,-5.90331311820653,7.15794922446635));
#17960=CARTESIAN_POINT('Ctrl Pts',(5.73768264733383,-5.75697331156837,7.16617079846651));
#17961=CARTESIAN_POINT('Ctrl Pts',(5.88247446602308,-5.60501398027574,7.17439237246666));
#17962=CARTESIAN_POINT('Ctrl Pts',(6.02727483851187,-5.45304567175172,7.18261443216895));
#17963=CARTESIAN_POINT('Ctrl Pts',(6.16618865358631,-5.29545738600774,7.19083649187124));
#17964=CARTESIAN_POINT('Ctrl Pts',(6.29879154616042,-5.13272954874091,7.19905855157353));
#17965=CARTESIAN_POINT('Ctrl Pts',(6.4313887281217,-4.97000871943337,7.20728025718852));
#17966=CARTESIAN_POINT('Ctrl Pts',(6.55767534570129,-4.80214901067917,7.21550196280352));
#17967=CARTESIAN_POINT('Ctrl Pts',(6.67726755981736,-4.62966364837779,7.22372366841851));
#17968=CARTESIAN_POINT('Ctrl Pts',(6.79688947185335,-4.45713545338438,7.23194741570116));
#17969=CARTESIAN_POINT('Ctrl Pts',(6.90981348869871,-4.27997955088766,7.24017116298381));
#17970=CARTESIAN_POINT('Ctrl Pts',(7.01569862192865,-4.09873888028604,7.24839491026646));
#17971=CARTESIAN_POINT('Ctrl Pts',(7.11795771483149,-3.92370480319253,7.25633703501743));
#17972=CARTESIAN_POINT('Ctrl Pts',(7.21365187453952,-3.74486129647251,7.26427915976841));
#17973=CARTESIAN_POINT('Ctrl Pts',(7.3025141739088,-3.56272007072702,7.27222128451938));
#17974=CARTESIAN_POINT('Ctrl Pts',(7.39452514250719,-3.37412501161318,7.28044482359336));
#17975=CARTESIAN_POINT('Ctrl Pts',(7.47924115530385,-3.18193299646193,7.28866836266734));
#17976=CARTESIAN_POINT('Ctrl Pts',(7.55639768745436,-2.98672756567021,7.29689190174131));
#17977=CARTESIAN_POINT('Ctrl Pts',(7.63354019120711,-2.79155762661658,7.30511394563304));
#17978=CARTESIAN_POINT('Ctrl Pts',(7.70312584918836,-2.59337563960125,7.31333598952476));
#17979=CARTESIAN_POINT('Ctrl Pts',(7.76493841870277,-2.39278476178984,7.32155803341648));
#17980=CARTESIAN_POINT('Ctrl Pts',(7.82674416362197,-2.19221603079347,7.32977916952971));
#17981=CARTESIAN_POINT('Ctrl Pts',(7.88077844663869,-1.98923922172765,7.33800030564295));
#17982=CARTESIAN_POINT('Ctrl Pts',(7.92687475615988,-1.78447307703291,7.34622144175618));
#17983=CARTESIAN_POINT('Ctrl Pts',(7.97297472181362,-1.57969069129466,7.35444322992949));
#17984=CARTESIAN_POINT('Ctrl Pts',(8.01113538861028,-1.37311897351596,7.3626650181028));
#17985=CARTESIAN_POINT('Ctrl Pts',(8.04124104749046,-1.16538833813218,7.37088680627611));
#17986=CARTESIAN_POINT('Ctrl Pts',(8.07134662283547,-0.957658279145457,
7.37910857163616));
#17987=CARTESIAN_POINT('Ctrl Pts',(8.09339719534004,-0.748769601255617,
7.38733033699621));
#17988=CARTESIAN_POINT('Ctrl Pts',(8.10732868918165,-0.539359887340692,
7.39555210235626));
#17989=CARTESIAN_POINT('Ctrl Pts',(8.12126308750845,-0.32990651497671,7.4037755818179));
#17990=CARTESIAN_POINT('Ctrl Pts',(8.12707500607554,-0.119932183916431,
7.41199906127953));
#17991=CARTESIAN_POINT('Ctrl Pts',(8.12475239826843,0.0899223516781355,
7.42022254074117));
#17992=CARTESIAN_POINT('Ctrl Pts',(8.1238139787038,0.17471135536876,7.42354513097467));
#17993=CARTESIAN_POINT('Ctrl Pts',(8.12154822459675,0.259480796073226,7.42686772120818));
#17994=CARTESIAN_POINT('Ctrl Pts',(8.11795675478785,0.344188451134322,7.43019031144168));
#17995=CARTESIAN_POINT('Ctrl Pts',(8.10906772838656,0.553843166974015,7.43841385051562));
#17996=CARTESIAN_POINT('Ctrl Pts',(8.0920510902348,0.763187399131707,7.44663738958956));
#17997=CARTESIAN_POINT('Ctrl Pts',(8.06695208136577,0.971582049776792,7.45486092866349));
#17998=CARTESIAN_POINT('Ctrl Pts',(8.04185763593252,1.17993881065456,7.46308297255518));
#17999=CARTESIAN_POINT('Ctrl Pts',(8.0086837880162,1.38734604193663,7.47130501644687));
#18000=CARTESIAN_POINT('Ctrl Pts',(7.96752757674456,1.59317038521149,7.47952706033857));
#18001=CARTESIAN_POINT('Ctrl Pts',(7.92637590944327,1.79897200385541,7.48774819645176));
#18002=CARTESIAN_POINT('Ctrl Pts',(7.87724369610853,2.00319079430361,7.49596933256495));
#18003=CARTESIAN_POINT('Ctrl Pts',(7.82027912851159,2.20520337263164,7.50419046867814));
#18004=CARTESIAN_POINT('Ctrl Pts',(7.7633100427653,2.40723197360391,7.51241225685142));
#18005=CARTESIAN_POINT('Ctrl Pts',(7.69850743899205,2.60705372822604,7.5206340450247));
#18006=CARTESIAN_POINT('Ctrl Pts',(7.62606974046467,2.80405917841781,7.52885583319798));
#18007=CARTESIAN_POINT('Ctrl Pts',(7.55363224293257,3.00106408197203,7.53707759855799));
#18008=CARTESIAN_POINT('Ctrl Pts',(7.47355979733775,3.19525242084551,7.545299363918));
#18009=CARTESIAN_POINT('Ctrl Pts',(7.38609964456578,3.38603301859938,7.55352112927801));
#18010=CARTESIAN_POINT('Ctrl Pts',(7.29862125780382,3.57685339094087,7.56174460873961));
#18011=CARTESIAN_POINT('Ctrl Pts',(7.20375220988757,3.7642643347215,7.56996808820122));
#18012=CARTESIAN_POINT('Ctrl Pts',(7.10178700425989,3.94769665863847,7.57819156766283));
#18013=CARTESIAN_POINT('Ctrl Pts',(7.06058928521914,4.02181011035177,7.58151415789654));
#18014=CARTESIAN_POINT('Ctrl Pts',(7.01823367273,4.09527434525954,7.58483674813025));
#18015=CARTESIAN_POINT('Ctrl Pts',(6.97474169477012,4.16805300514942,7.58815933836396));
#18016=CARTESIAN_POINT('Ctrl Pts',(6.86709737061338,4.34818299749209,7.59638287743793));
#18017=CARTESIAN_POINT('Ctrl Pts',(6.75245376590448,4.52416997829286,7.6046064165119));
#18018=CARTESIAN_POINT('Ctrl Pts',(6.63115497203716,4.69547349042957,7.61282995558587));
#18019=CARTESIAN_POINT('Ctrl Pts',(6.50987823239749,4.86674585661227,7.6210519994776));
#18020=CARTESIAN_POINT('Ctrl Pts',(6.38194888903332,5.03333621311725,7.62927404336933));
#18021=CARTESIAN_POINT('Ctrl Pts',(6.24775384980835,5.19473381365253,7.63749608726106));
#18022=CARTESIAN_POINT('Ctrl Pts',(6.11357362677427,5.35611359461956,7.64571722337428));
#18023=CARTESIAN_POINT('Ctrl Pts',(5.97312927748498,5.51230153753551,7.65393835948751));
#18024=CARTESIAN_POINT('Ctrl Pts',(5.82684794214979,5.66282002376597,7.66215949560073));
#18025=CARTESIAN_POINT('Ctrl Pts',(5.68055500449834,5.81335044838265,7.67038128377405));
#18026=CARTESIAN_POINT('Ctrl Pts',(5.52842435941999,5.95821030446604,7.67860307194737));
#18027=CARTESIAN_POINT('Ctrl Pts',(5.37092068800271,6.09695813711104,7.68682486012069));
#18028=CARTESIAN_POINT('Ctrl Pts',(5.21341745361613,6.23570558476779,7.69504662548074));
#18029=CARTESIAN_POINT('Ctrl Pts',(5.05054144580448,6.3683408499792,7.70326839084078));
#18030=CARTESIAN_POINT('Ctrl Pts',(4.88279156918908,6.49446179866785,7.71149015620083));
#18031=CARTESIAN_POINT('Ctrl Pts',(4.7150067195091,6.62060904148066,7.71971363566247));
#18032=CARTESIAN_POINT('Ctrl Pts',(4.54234620688782,6.74023907735389,7.72793711512412));
#18033=CARTESIAN_POINT('Ctrl Pts',(4.36534002859345,6.85299160930901,7.73616059458576));
#18034=CARTESIAN_POINT('Ctrl Pts',(4.293822977689,6.89854780765837,7.73948318481926));
#18035=CARTESIAN_POINT('Ctrl Pts',(4.22159684483345,6.94298177497777,7.74280577505276));
#18036=CARTESIAN_POINT('Ctrl Pts',(4.14869787298499,6.98627178981678,7.74612836528626));
#18037=CARTESIAN_POINT('Ctrl Pts',(3.96827010388932,7.09341624746095,7.75435190436024));
#18038=CARTESIAN_POINT('Ctrl Pts',(3.78366013480724,7.19358476960094,7.76257544343422));
#18039=CARTESIAN_POINT('Ctrl Pts',(3.59542788694271,7.28646593845704,7.77079898250821));
#18040=CARTESIAN_POINT('Ctrl Pts',(3.40722986297049,7.37933021990327,7.77902102639995));
#18041=CARTESIAN_POINT('Ctrl Pts',(3.21541113904964,7.46490966210488,7.78724307029169));
#18042=CARTESIAN_POINT('Ctrl Pts',(3.02055514069819,7.54293936105161,7.79546511418343));
#18043=CARTESIAN_POINT('Ctrl Pts',(2.82572065598566,7.62096044490422,7.80368625029668));
#18044=CARTESIAN_POINT('Ctrl Pts',(2.62784984002567,7.6914333400571,7.81190738640993));
#18045=CARTESIAN_POINT('Ctrl Pts',(2.42754572333658,7.75414143046219,7.82012852252318));
#18046=CARTESIAN_POINT('Ctrl Pts',(2.22722571951015,7.81685449456459,7.82835031069651));
#18047=CARTESIAN_POINT('Ctrl Pts',(2.02447231000839,7.87180143271431,7.83657209886984));
#18048=CARTESIAN_POINT('Ctrl Pts',(1.8199043179409,7.91881530508447,7.84479388704317));
#18049=CARTESIAN_POINT('Ctrl Pts',(1.61533689349503,7.96582904700367,7.85301565240323));
#18050=CARTESIAN_POINT('Ctrl Pts',(1.40895518459802,8.00490970374414,7.8612374177633));
#18051=CARTESIAN_POINT('Ctrl Pts',(1.20138938654037,8.03594120837181,7.86945918312336));
#18052=CARTESIAN_POINT('Ctrl Pts',(0.993780314459552,8.06697918255304,7.87768266258501));
#18053=CARTESIAN_POINT('Ctrl Pts',(0.78498695180016,8.08996460861358,7.88590614204666));
#18054=CARTESIAN_POINT('Ctrl Pts',(0.575646914719905,8.10483301444721,7.89412962150832));
#18055=CARTESIAN_POINT('Ctrl Pts',(0.491065787484527,8.11084040100901,7.89745221174172));
#18056=CARTESIAN_POINT('Ctrl Pts',(0.406395473335491,8.11552330827984,7.90077480197513));
#18057=CARTESIAN_POINT('Ctrl Pts',(0.321678185702375,8.11887989240777,7.90409739220854));
#18058=CARTESIAN_POINT('Ctrl Pts',(0.11199962887258,8.12718756768263,7.91232093128234));
#18059=CARTESIAN_POINT('Ctrl Pts',(-0.0980349882997524,8.12736950028921,
7.92054447035614));
#18060=CARTESIAN_POINT('Ctrl Pts',(-0.307785009625147,8.11941844902392,
7.92876800942994));
#18061=CARTESIAN_POINT('Ctrl Pts',(-0.517496894753254,8.11146884339787,
7.93699005332149));
#18062=CARTESIAN_POINT('Ctrl Pts',(-0.726923992733384,8.09538921641806,
7.94521209721304));
#18063=CARTESIAN_POINT('Ctrl Pts',(-0.935427126214352,8.07122442099353,
7.95343414110459));
#18064=CARTESIAN_POINT('Ctrl Pts',(-1.14390723930476,8.04706229355302,7.96165527721765));
#18065=CARTESIAN_POINT('Ctrl Pts',(-1.35146329870153,8.01481681378467,7.9698764133307));
#18066=CARTESIAN_POINT('Ctrl Pts',(-1.55746187958918,7.97458463220038,7.97809754944375));
#18067=CARTESIAN_POINT('Ctrl Pts',(-1.76347679927134,7.93434925959728,7.9863193376169));
#18068=CARTESIAN_POINT('Ctrl Pts',(-1.96793370363497,7.88612597338955,7.99454112579004));
#18069=CARTESIAN_POINT('Ctrl Pts',(-2.17020893391364,7.83006262718642,8.00276291396318));
#18070=CARTESIAN_POINT('Ctrl Pts',(-2.37248360293232,7.77399943654416,8.01098467932305));
#18071=CARTESIAN_POINT('Ctrl Pts',(-2.57257632647824,7.71009631079563,8.01920644468292));
#18072=CARTESIAN_POINT('Ctrl Pts',(-2.76987766877603,7.63855125416566,8.02742821004279));
#18073=CARTESIAN_POINT('Ctrl Pts',(-2.96722014512873,7.56699128157895,8.03565168950427));
#18074=CARTESIAN_POINT('Ctrl Pts',(-3.16176980033458,7.48778629588259,8.04387516896574));
#18075=CARTESIAN_POINT('Ctrl Pts',(-3.35293523999828,7.40118320533127,8.05209864842722));
#18076=CARTESIAN_POINT('Ctrl Pts',(-3.43017315686592,7.36619234966065,8.05542123866176));
#18077=CARTESIAN_POINT('Ctrl Pts',(-3.50685884706295,7.32999432979059,8.0587438288963));
#18078=CARTESIAN_POINT('Ctrl Pts',(-3.58295431172122,7.2926076243425,8.06206641913084));
#18079=CARTESIAN_POINT('Ctrl Pts',(-3.77129352384996,7.20007408532274,8.07028995820521));
#18080=CARTESIAN_POINT('Ctrl Pts',(-3.95607674832197,7.10022553265419,8.07851349727958));
#18081=CARTESIAN_POINT('Ctrl Pts',(-4.13673716809682,6.99336064882874,8.08673703635396));
#18082=CARTESIAN_POINT('Ctrl Pts',(-4.31736474066964,6.88651519489519,8.0949590802461));
#18083=CARTESIAN_POINT('Ctrl Pts',(-4.49387075093313,6.77265610602097,8.10318112413823));
#18084=CARTESIAN_POINT('Ctrl Pts',(-4.66571448703126,6.65212717016193,8.11140316803037));
#18085=CARTESIAN_POINT('Ctrl Pts',(-4.83753925022554,6.53161154164806,8.11962430414402));
#18086=CARTESIAN_POINT('Ctrl Pts',(-5.00470252556901,6.40442770564491,8.12784544025766));
#18087=CARTESIAN_POINT('Ctrl Pts',(-5.16669332333603,6.27096225990038,8.13606657637131));
#18088=CARTESIAN_POINT('Ctrl Pts',(-5.32869696941604,6.13748622833342,8.14428836454502));
#18089=CARTESIAN_POINT('Ctrl Pts',(-5.48552708887313,5.99772777702664,8.15251015271874));
#18090=CARTESIAN_POINT('Ctrl Pts',(-5.63670566037028,5.85211387968909,8.16073194089245));
#18091=CARTESIAN_POINT('Ctrl Pts',(-5.78788381238767,5.70650038639083,8.16895370625292));
#18092=CARTESIAN_POINT('Ctrl Pts',(-5.9334102372631,5.55503168610662,8.17717547161338));
#18093=CARTESIAN_POINT('Ctrl Pts',(-6.07284330017465,5.39817208080882,8.18539723697385));
#18094=CARTESIAN_POINT('Ctrl Pts',(-6.21230543256481,5.24127977288767,8.19362071643588));
#18095=CARTESIAN_POINT('Ctrl Pts',(-6.34567146918689,5.0789945351682,8.20184419589792));
#18096=CARTESIAN_POINT('Ctrl Pts',(-6.47253892591764,4.91181508354914,8.21006767535996));
#18097=CARTESIAN_POINT('Ctrl Pts',(-6.52379807653848,4.8442683941768,8.21339026559101));
#18098=CARTESIAN_POINT('Ctrl Pts',(-6.57399682523498,4.77592311388816,8.21671285582206));
#18099=CARTESIAN_POINT('Ctrl Pts',(-6.62311055586632,4.70681358535391,8.22003544605311));
#18100=CARTESIAN_POINT('Ctrl Pts',(-6.74466893495809,4.53576483461904,8.22825898512622));
#18101=CARTESIAN_POINT('Ctrl Pts',(-6.85961724827754,4.35997672703516,8.23648252419932));
#18102=CARTESIAN_POINT('Ctrl Pts',(-6.96759927654907,4.17998180425858,8.24470606327243));
#18103=CARTESIAN_POINT('Ctrl Pts',(-7.07556167181243,4.00001960768513,8.25292810716331));
#18104=CARTESIAN_POINT('Ctrl Pts',(-7.17656015834777,3.81585237530458,8.26115015105419));
#18105=CARTESIAN_POINT('Ctrl Pts',(-7.27028294988928,3.62803988278096,8.26937219494506));
#18106=CARTESIAN_POINT('Ctrl Pts',(-7.36399539369519,3.4402481262382,8.27759333105743));
#18107=CARTESIAN_POINT('Ctrl Pts',(-7.45043361461306,3.24881217685777,8.2858144671698));
#18108=CARTESIAN_POINT('Ctrl Pts',(-7.52933234690375,3.05431530336488,8.29403560328216));
#18109=CARTESIAN_POINT('Ctrl Pts',(-7.60823733705397,2.85980300333624,8.30225739145462));
#18110=CARTESIAN_POINT('Ctrl Pts',(-7.67960153040176,2.662229566419,8.31047917962708));
#18111=CARTESIAN_POINT('Ctrl Pts',(-7.74320787749797,2.46219806846511,8.31870096779955));
#18112=CARTESIAN_POINT('Ctrl Pts',(-7.80681404810367,2.26216712554486,8.32692273315876));
#18113=CARTESIAN_POINT('Ctrl Pts',(-7.86266232871362,2.05967841711304,8.33514449851796));
#18114=CARTESIAN_POINT('Ctrl Pts',(-7.91058544077199,1.85535051856683,8.34336626387717));
#18115=CARTESIAN_POINT('Ctrl Pts',(-7.95851854400361,1.65098002104596,8.35158974333796));
#18116=CARTESIAN_POINT('Ctrl Pts',(-7.99852311057174,1.44476985459871,8.35981322279876));
#18117=CARTESIAN_POINT('Ctrl Pts',(-8.03048267586436,1.23735021523509,8.36803670225956));
#18118=CARTESIAN_POINT('Ctrl Pts',(-8.04339552378697,1.15354499965283,8.37135929249818));
#18119=CARTESIAN_POINT('Ctrl Pts',(-8.05499564268842,1.06954244622362,8.3746818827368));
#18120=CARTESIAN_POINT('Ctrl Pts',(-8.06527773840728,0.985384475649966,
8.37800447297542));
#18121=CARTESIAN_POINT('Ctrl Pts',(-8.09203917827196,0.766344648534784,
8.38665225269826));
#18122=CARTESIAN_POINT('Ctrl Pts',(-8.10987423995967,0.546205259409921,
8.3953000324211));
#18123=CARTESIAN_POINT('Ctrl Pts',(-8.11872063627548,0.325672830636386,
8.40394781214395));
#18124=CARTESIAN_POINT('Ctrl Pts',(-8.12306986537984,0.217250595927776,
8.40819939368247));
#18125=CARTESIAN_POINT('Ctrl Pts',(-8.1252472503007,0.108733441558642,8.41245097522098));
#18126=CARTESIAN_POINT('Ctrl Pts',(-8.12524999739701,0.000205669423076638,
8.4167025567595));
#18127=CARTESIAN_POINT('Origin',(0.,0.,-16.4167025567876));
#18128=CARTESIAN_POINT('',(4.94675008185377,-6.44587862049696,5.12505864308909));
#18129=CARTESIAN_POINT('',(4.94675008185375,-6.44587862049697,5.29165016466231));
#18130=CARTESIAN_POINT('',(4.94675008185374,-6.44587862049697,-16.4167025567876));
#18131=CARTESIAN_POINT('',(-8.12524999762747,-0.000196353792745782,6.58329744321239));
#18132=CARTESIAN_POINT('Ctrl Pts',(4.94675008185375,-6.44587862049697,5.29165016466231));
#18133=CARTESIAN_POINT('Ctrl Pts',(5.11327081011718,-6.31808589049612,5.29987187156593));
#18134=CARTESIAN_POINT('Ctrl Pts',(5.27483491075145,-6.18383844836398,5.30809357846955));
#18135=CARTESIAN_POINT('Ctrl Pts',(5.43095059073167,-6.04354724011746,5.31631528537316));
#18136=CARTESIAN_POINT('Ctrl Pts',(5.58710529693372,-5.90322096149353,5.32453904756141));
#18137=CARTESIAN_POINT('Ctrl Pts',(5.73780863988046,-5.75684809339947,5.33276280974965));
#18138=CARTESIAN_POINT('Ctrl Pts',(5.88260367082485,-5.60487837642335,5.3409865719379));
#18139=CARTESIAN_POINT('Ctrl Pts',(6.0253035427776,-5.45510763490172,5.3490913377132));
#18140=CARTESIAN_POINT('Ctrl Pts',(6.16226475094292,-5.29990113350262,5.35719610348851));
#18141=CARTESIAN_POINT('Ctrl Pts',(6.29308631040871,-5.13972297427074,5.36530086926381));
#18142=CARTESIAN_POINT('Ctrl Pts',(6.42582502683911,-4.97719744450756,5.37352440833777));
#18143=CARTESIAN_POINT('Ctrl Pts',(6.55228585150901,-4.80950059499723,5.38174794741173));
#18144=CARTESIAN_POINT('Ctrl Pts',(6.67207770646967,-4.63713992039602,5.38997148648569));
#18145=CARTESIAN_POINT('Ctrl Pts',(6.79184778119074,-4.46481058395874,5.39819353037743));
#18146=CARTESIAN_POINT('Ctrl Pts',(6.90495113804472,-4.2878193569373,5.40641557426917));
#18147=CARTESIAN_POINT('Ctrl Pts',(7.01103920883055,-4.10670388203735,5.41463761816091));
#18148=CARTESIAN_POINT('Ctrl Pts',(7.11711556665462,-3.92560840371775,5.422858754274));
#18149=CARTESIAN_POINT('Ctrl Pts',(7.21617803574784,-3.74038984099968,5.4310798903871));
#18150=CARTESIAN_POINT('Ctrl Pts',(7.30792289097652,-3.55161239186391,5.43930102650019));
#18151=CARTESIAN_POINT('Ctrl Pts',(7.3996750229574,-3.36281996982626,5.4475228146735));
#18152=CARTESIAN_POINT('Ctrl Pts',(7.48410825008128,-3.17046836147892,5.4557446028468));
#18153=CARTESIAN_POINT('Ctrl Pts',(7.56096562904357,-2.97514475596091,5.46396639102011));
#18154=CARTESIAN_POINT('Ctrl Pts',(7.63782279474688,-2.77982169241446,5.47218815638012));
#18155=CARTESIAN_POINT('Ctrl Pts',(7.70710404885484,-2.58152692363019,5.48040992174014));
#18156=CARTESIAN_POINT('Ctrl Pts',(7.76860106943491,-2.38086643608471,5.48863168710015));
#18157=CARTESIAN_POINT('Ctrl Pts',(7.83011091112316,-2.18016411415777,5.49685516656179));
#18158=CARTESIAN_POINT('Ctrl Pts',(7.88383319079082,-1.97709537020895,5.50507864602343));
#18159=CARTESIAN_POINT('Ctrl Pts',(7.92960950831404,-1.77228118766622,5.51330212548507));
#18160=CARTESIAN_POINT('Ctrl Pts',(7.94810483577805,-1.68952867325787,5.51662471571875));
#18161=CARTESIAN_POINT('Ctrl Pts',(7.96530359370538,-1.60649136570547,5.51994730595243));
#18162=CARTESIAN_POINT('Ctrl Pts',(7.98119769287488,-1.52321073714334,5.52326989618611));
#18163=CARTESIAN_POINT('Ctrl Pts',(8.020536201801,-1.31708796698015,5.53149343526006));
#18164=CARTESIAN_POINT('Ctrl Pts',(8.05189182966708,-1.10940696613294,5.539716974334));
#18165=CARTESIAN_POINT('Ctrl Pts',(8.07516232205342,-0.900800219243289,
5.54794051340795));
#18166=CARTESIAN_POINT('Ctrl Pts',(8.0984285834601,-0.69223140068324,5.55616255729967));
#18167=CARTESIAN_POINT('Ctrl Pts',(8.11361261069341,-0.482737464993099,
5.56438460119139));
#18168=CARTESIAN_POINT('Ctrl Pts',(8.12066388589119,-0.272957166754323,
5.57260664508311));
#18169=CARTESIAN_POINT('Ctrl Pts',(8.12771438257256,-0.0632000299157026,
5.58082778119631));
#18170=CARTESIAN_POINT('Ctrl Pts',(8.12663390997845,0.146843111696508,5.58904891730951));
#18171=CARTESIAN_POINT('Ctrl Pts',(8.11742402792945,0.356531503928758,5.59727005342272));
#18172=CARTESIAN_POINT('Ctrl Pts',(8.10821341539789,0.566236527612974,5.605491841596));
#18173=CARTESIAN_POINT('Ctrl Pts',(8.0908721153668,0.775586450921568,5.61371362976927));
#18174=CARTESIAN_POINT('Ctrl Pts',(8.06545377315046,0.983942577426666,5.62193541794256));
#18175=CARTESIAN_POINT('Ctrl Pts',(8.04003550146333,1.1922981257983,5.63015718330254));
#18176=CARTESIAN_POINT('Ctrl Pts',(8.00654027081425,1.39965959044746,5.63837894866252));
#18177=CARTESIAN_POINT('Ctrl Pts',(7.96507343273785,1.60539489646433,5.6466007140225));
#18178=CARTESIAN_POINT('Ctrl Pts',(7.92359794951369,1.8111730948791,5.65482419348415));
#18179=CARTESIAN_POINT('Ctrl Pts',(7.87414759705053,2.01532416821216,5.66304767294581));
#18180=CARTESIAN_POINT('Ctrl Pts',(7.81687876709476,2.21722662419589,5.67127115240746));
#18181=CARTESIAN_POINT('Ctrl Pts',(7.79374003901856,2.29880269324658,5.6745937426411));
#18182=CARTESIAN_POINT('Ctrl Pts',(7.7693255511162,2.38001183374261,5.67791633287475));
#18183=CARTESIAN_POINT('Ctrl Pts',(7.74364793709499,2.46081372493419,5.6812389231084));
#18184=CARTESIAN_POINT('Ctrl Pts',(7.68009485128538,2.66080152443282,5.68946246218234));
#18185=CARTESIAN_POINT('Ctrl Pts',(7.60877996240833,2.85835850389997,5.69768600125629));
#18186=CARTESIAN_POINT('Ctrl Pts',(7.52991451097841,3.0528797912556,5.70590954033023));
#18187=CARTESIAN_POINT('Ctrl Pts',(7.4510633986569,3.2473657112637,5.71413158422198));
#18188=CARTESIAN_POINT('Ctrl Pts',(7.36466457454118,3.43881676758294,5.72235362811374));
#18189=CARTESIAN_POINT('Ctrl Pts',(7.2709777597904,3.62664720908078,5.73057567200549));
#18190=CARTESIAN_POINT('Ctrl Pts',(7.17730128880249,3.81445691261722,5.73879680811878));
#18191=CARTESIAN_POINT('Ctrl Pts',(7.07633856522753,3.99864653558411,5.74701794423208));
#18192=CARTESIAN_POINT('Ctrl Pts',(6.96839605749512,4.17865336542605,5.75523908034537));
#18193=CARTESIAN_POINT('Ctrl Pts',(6.8604449882947,4.35867447252305,5.76346086851869));
#18194=CARTESIAN_POINT('Ctrl Pts',(6.74551317819972,4.53451186929834,5.77168265669199));
#18195=CARTESIAN_POINT('Ctrl Pts',(6.62395191788581,4.70562945332895,5.77990444486531));
#18196=CARTESIAN_POINT('Ctrl Pts',(6.50239099487288,4.87674656255263,5.78812621022529));
#18197=CARTESIAN_POINT('Ctrl Pts',(6.37420083144179,5.0431436463528,5.79634797558527));
#18198=CARTESIAN_POINT('Ctrl Pts',(6.23977503393361,5.20431504507546,5.80456974094526));
#18199=CARTESIAN_POINT('Ctrl Pts',(6.10532121087724,5.36552004536035,5.81279322040689));
#18200=CARTESIAN_POINT('Ctrl Pts',(5.96462934560591,5.52149695758798,5.82101669986853));
#18201=CARTESIAN_POINT('Ctrl Pts',(5.81813288836337,5.67177373101612,5.82924017933016));
#18202=CARTESIAN_POINT('Ctrl Pts',(5.75894289459634,5.73249111251439,5.83256276956367));
#18203=CARTESIAN_POINT('Ctrl Pts',(5.69880575929252,5.79227837433905,5.83588535979718));
#18204=CARTESIAN_POINT('Ctrl Pts',(5.63775179089365,5.85110607550191,5.83920795003068));
#18205=CARTESIAN_POINT('Ctrl Pts',(5.4866408625328,5.99670690652375,5.84743148910464));
#18206=CARTESIAN_POINT('Ctrl Pts',(5.32986193586128,6.13647436219046,5.85565502817858));
#18207=CARTESIAN_POINT('Ctrl Pts',(5.16788877933457,6.26997712331774,5.86387856725254));
#18208=CARTESIAN_POINT('Ctrl Pts',(5.00594507234165,6.40345561132373,5.87210061114422));
#18209=CARTESIAN_POINT('Ctrl Pts',(4.83880924788867,6.53067149067059,5.8803226550359));
#18210=CARTESIAN_POINT('Ctrl Pts',(4.66698860200944,6.65123334060789,5.88854469892759));
#18211=CARTESIAN_POINT('Ctrl Pts',(4.49518692648261,6.77178187956752,5.89676583504087));
#18212=CARTESIAN_POINT('Ctrl Pts',(4.31870170351852,6.88567768649474,5.90498697115416));
#18213=CARTESIAN_POINT('Ctrl Pts',(4.13807036707505,6.99257185873948,5.91320810726745));
#18214=CARTESIAN_POINT('Ctrl Pts',(3.95742470384393,7.09947450930331,5.92142989544075));
#18215=CARTESIAN_POINT('Ctrl Pts',(3.77263252254023,7.19937426308323,5.92965168361405));
#18216=CARTESIAN_POINT('Ctrl Pts',(3.58425800164598,7.29196695961637,5.93787347178735));
#18217=CARTESIAN_POINT('Ctrl Pts',(3.3958840034416,7.38455939922907,5.94609523714734));
#18218=CARTESIAN_POINT('Ctrl Pts',(3.20392795140517,7.46984469447034,5.95431700250735));
#18219=CARTESIAN_POINT('Ctrl Pts',(3.00897673942943,7.54756560382701,5.96253876786734));
#18220=CARTESIAN_POINT('Ctrl Pts',(2.8139848833609,7.62530271670363,5.97076224732899));
#18221=CARTESIAN_POINT('Ctrl Pts',(2.61599689391173,7.69547218396382,5.97898572679063));
#18222=CARTESIAN_POINT('Ctrl Pts',(2.41561869924228,7.75786529029546,5.98720920625227));
#18223=CARTESIAN_POINT('Ctrl Pts',(2.33465848821067,7.78307441578868,5.99053179648584));
#18224=CARTESIAN_POINT('Ctrl Pts',(2.2533082752287,7.80701464484136,5.99385438671941));
#18225=CARTESIAN_POINT('Ctrl Pts',(2.17160873081213,7.82967451959278,5.99717697695298));
#18226=CARTESIAN_POINT('Ctrl Pts',(1.96939920492885,7.88575858423208,6.00540051602693));
#18227=CARTESIAN_POINT('Ctrl Pts',(1.76498303012576,7.93401416412474,6.0136240551009));
#18228=CARTESIAN_POINT('Ctrl Pts',(1.55898219445379,7.97428755939213,6.02184759417486));
#18229=CARTESIAN_POINT('Ctrl Pts',(1.35301881331104,8.01455363225689,6.03006963806661));
#18230=CARTESIAN_POINT('Ctrl Pts',(1.14547163566338,8.04684036056402,6.03829168195836));
#18231=CARTESIAN_POINT('Ctrl Pts',(0.936973134717045,8.0710450938722,6.04651372585011));
#18232=CARTESIAN_POINT('Ctrl Pts',(0.728497653651553,8.0952471547867,6.05473486196329));
#18233=CARTESIAN_POINT('Ctrl Pts',(0.519071351836212,8.11136896818083,6.06295599807648));
#18234=CARTESIAN_POINT('Ctrl Pts',(0.309332959536304,8.11935962269467,6.07117713418966));
#18235=CARTESIAN_POINT('Ctrl Pts',(0.0995779318177861,8.12735091098795,
6.07939892236296));
#18236=CARTESIAN_POINT('Ctrl Pts',(-0.110488941216562,8.12720973790773,
6.08762071053625));
#18237=CARTESIAN_POINT('Ctrl Pts',(-0.320226715276507,8.11893727117799,
6.09584249870955));
#18238=CARTESIAN_POINT('Ctrl Pts',(-0.529963907372128,8.11066482740207,
6.10406426406966));
#18239=CARTESIAN_POINT('Ctrl Pts',(-0.739371707723339,8.09426114942689,
6.11228602942977));
#18240=CARTESIAN_POINT('Ctrl Pts',(-0.947811537538,8.06977947975097,6.12050779478988));
#18241=CARTESIAN_POINT('Ctrl Pts',(-1.15629482359629,8.04529270605341,6.12873127425156));
#18242=CARTESIAN_POINT('Ctrl Pts',(-1.36380944299606,8.01272461066221,6.13695475371323));
#18243=CARTESIAN_POINT('Ctrl Pts',(-1.56972318479993,7.97218017142121,6.14517823317491));
#18244=CARTESIAN_POINT('Ctrl Pts',(-1.65291996186244,7.95579871653089,6.14850082340836));
#18245=CARTESIAN_POINT('Ctrl Pts',(-1.7358555036824,7.93811574105068,6.15182341364181));
#18246=CARTESIAN_POINT('Ctrl Pts',(-1.81848859043681,7.91914053473931,6.15514600387527));
#18247=CARTESIAN_POINT('Ctrl Pts',(-2.02300866964623,7.87217616670896,6.16336954294922));
#18248=CARTESIAN_POINT('Ctrl Pts',(-2.22574163981204,7.81727701990729,6.17159308202317));
#18249=CARTESIAN_POINT('Ctrl Pts',(-2.42606736327293,7.75460409765463,6.17981662109712));
#18250=CARTESIAN_POINT('Ctrl Pts',(-2.62635666403652,7.6919425704282,6.18803866498878));
#18251=CARTESIAN_POINT('Ctrl Pts',(-2.82423931031158,7.62151017676951,6.19626070888043));
#18252=CARTESIAN_POINT('Ctrl Pts',(-3.01911025150712,7.54351780350153,6.20448275277209));
#18253=CARTESIAN_POINT('Ctrl Pts',(-3.21395967741587,7.46553404120587,6.21270388888535));
#18254=CARTESIAN_POINT('Ctrl Pts',(-3.40579778838885,7.37999207525797,6.22092502499861));
#18255=CARTESIAN_POINT('Ctrl Pts',(-3.59403866731135,7.28715126921151,6.22914616111186));
#18256=CARTESIAN_POINT('Ctrl Pts',(-3.78229447657336,7.1943030994895,6.23736794928514));
#18257=CARTESIAN_POINT('Ctrl Pts',(-3.96695221800712,7.09415506104298,6.24558973745842));
#18258=CARTESIAN_POINT('Ctrl Pts',(-4.14744882516031,6.98701336804048,6.25381152563171));
#18259=CARTESIAN_POINT('Ctrl Pts',(-4.32794493148387,6.87987197232742,6.26203329099174));
#18260=CARTESIAN_POINT('Ctrl Pts',(-4.50427967438332,6.76573711374006,6.27025505635178));
#18261=CARTESIAN_POINT('Ctrl Pts',(-4.67591686307836,6.64495967272033,6.27847682171181));
#18262=CARTESIAN_POINT('Ctrl Pts',(-4.84758983527764,6.52415705160934,6.28670030117342));
#18263=CARTESIAN_POINT('Ctrl Pts',(-5.01456305554396,6.39670925125489,6.29492378063502));
#18264=CARTESIAN_POINT('Ctrl Pts',(-5.17633056667184,6.26300961415826,6.30314726009662));
#18265=CARTESIAN_POINT('Ctrl Pts',(-5.24169063172759,6.20899000961815,6.30646985033027));
#18266=CARTESIAN_POINT('Ctrl Pts',(-5.30620125380452,6.15395028433812,6.30979244056392));
#18267=CARTESIAN_POINT('Ctrl Pts',(-5.36983060907314,6.09791823431253,6.31311503079757));
#18268=CARTESIAN_POINT('Ctrl Pts',(-5.52731571933501,5.95923674776865,6.32133856987151));
#18269=CARTESIAN_POINT('Ctrl Pts',(-5.67945114680157,5.8144286498553,6.32956210894545));
#18270=CARTESIAN_POINT('Ctrl Pts',(-5.82576822773381,5.66393080106274,6.33778564801939));
#18271=CARTESIAN_POINT('Ctrl Pts',(-5.97205870568036,5.51346031539206,6.34600769191115));
#18272=CARTESIAN_POINT('Ctrl Pts',(-6.11253274300237,5.35730235493905,6.3542297358029));
#18273=CARTESIAN_POINT('Ctrl Pts',(-6.24675869512846,5.19593046213448,6.36245177969466));
#18274=CARTESIAN_POINT('Ctrl Pts',(-6.38096982765176,5.03457638605846,6.37067291580799));
#18275=CARTESIAN_POINT('Ctrl Pts',(-6.50893406368367,4.86800975357322,6.37889405192132));
#18276=CARTESIAN_POINT('Ctrl Pts',(-6.63025966624038,4.69673762528056,6.38711518803465));
#18277=CARTESIAN_POINT('Ctrl Pts',(-6.75159489174576,4.52545191252702,6.39533697620796));
#18278=CARTESIAN_POINT('Ctrl Pts',(-6.8662902590413,4.34946019738865,6.40355876438126));
#18279=CARTESIAN_POINT('Ctrl Pts',(-6.97399643320615,4.16929985874461,6.41178055255457));
#18280=CARTESIAN_POINT('Ctrl Pts',(-7.08170230851493,3.98914001999775,6.42000231791461));
#18281=CARTESIAN_POINT('Ctrl Pts',(-7.18241888046251,3.80481183541026,6.42822408327464));
#18282=CARTESIAN_POINT('Ctrl Pts',(-7.27584171555407,3.61687916479154,6.43644584863467));
#18283=CARTESIAN_POINT('Ctrl Pts',(-7.36928402775632,3.4289073133299,6.44466932809633));
#18284=CARTESIAN_POINT('Ctrl Pts',(-7.45542943402357,3.23732973875257,6.45289280755799));
#18285=CARTESIAN_POINT('Ctrl Pts',(-7.53402030555906,3.04273324462132,6.46111628701965));
#18286=CARTESIAN_POINT('Ctrl Pts',(-7.56577392802695,2.9641090547187,6.46443887725305));
#18287=CARTESIAN_POINT('Ctrl Pts',(-7.59629484888616,2.88499227325942,6.46776146748644));
#18288=CARTESIAN_POINT('Ctrl Pts',(-7.62556831858584,2.80542249600304,6.47108405771984));
#18289=CARTESIAN_POINT('Ctrl Pts',(-7.69788746847904,2.60884796256347,6.47929240827029));
#18290=CARTESIAN_POINT('Ctrl Pts',(-7.76261427768914,2.40944077562039,6.48750075882073));
#18291=CARTESIAN_POINT('Ctrl Pts',(-7.81954479118166,2.2078058839499,6.49570910937118));
#18292=CARTESIAN_POINT('Ctrl Pts',(-7.87646704650205,2.00620024084121,6.50391626924254));
#18293=CARTESIAN_POINT('Ctrl Pts',(-7.92559518063946,1.80236782324838,6.5121234291139));
#18294=CARTESIAN_POINT('Ctrl Pts',(-7.96677522118852,1.59692834452788,6.52033058898526));
#18295=CARTESIAN_POINT('Ctrl Pts',(-8.00794972966339,1.39151646428526,6.52853664631721));
#18296=CARTESIAN_POINT('Ctrl Pts',(-8.04117821850922,1.18449824532056,6.53674270364917));
#18297=CARTESIAN_POINT('Ctrl Pts',(-8.06635777565389,0.976503864635504,
6.54494876098113));
#18298=CARTESIAN_POINT('Ctrl Pts',(-8.09153848603434,0.768499957708096,
6.55315519415444));
#18299=CARTESIAN_POINT('Ctrl Pts',(-8.10866949080331,0.55952009450846,6.56136162732775));
#18300=CARTESIAN_POINT('Ctrl Pts',(-8.11769960763622,0.350200860482541,
6.56956806050107));
#18301=CARTESIAN_POINT('Ctrl Pts',(-8.12273541013038,0.233470330824207,
6.57414452140484));
#18302=CARTESIAN_POINT('Ctrl Pts',(-8.12525282094382,0.116634346959204,
6.57872098230862));
#18303=CARTESIAN_POINT('Ctrl Pts',(-8.12524999762747,-0.000196353792745782,
6.58329744321239));
#18304=CARTESIAN_POINT('Ctrl Pts',(-8.12501235669361,-0.00019654038003419,
6.58329745074651));
#18305=CARTESIAN_POINT('Ctrl Pts',(-8.12536948861794,-0.389544456400672,
6.59854932871172));
#18306=CARTESIAN_POINT('Ctrl Pts',(-8.00298129759573,-2.1228738540623,6.66645754898436));
#18307=CARTESIAN_POINT('Ctrl Pts',(-6.79075267338643,-5.05622322872534,
6.78702211156442));
#18308=CARTESIAN_POINT('Ctrl Pts',(-3.56400020377475,-7.67968864976366,
6.94499113848673));
#18309=CARTESIAN_POINT('Ctrl Pts',(0.522655372263073,-8.4502394387162,7.102960165409));
#18310=CARTESIAN_POINT('Ctrl Pts',(3.41983802727889,-7.52248145840713,7.21851605726134));
#18311=CARTESIAN_POINT('Ctrl Pts',(4.73959395534349,-6.60538794581216,7.28141560680623));
#18312=CARTESIAN_POINT('Ctrl Pts',(4.94684221335274,-6.44599857519204,7.2916588140437));
#18313=CARTESIAN_POINT('',(-8.12524999939286,-9.93290792602784E-5,6.41670255680724));
#18314=CARTESIAN_POINT('Ctrl Pts',(-8.12524999939286,-9.93290792612735E-5,
6.41670255680723));
#18315=CARTESIAN_POINT('Ctrl Pts',(-8.12524737621332,-0.214678883336293,
6.42510654393496));
#18316=CARTESIAN_POINT('Ctrl Pts',(-8.11674017324388,-0.429227910625565,
6.43351053106269));
#18317=CARTESIAN_POINT('Ctrl Pts',(-8.09976162698335,-0.643077871294042,
6.44191451819041));
#18318=CARTESIAN_POINT('Ctrl Pts',(-8.08277759880984,-0.856996878325916,
6.45032121873808));
#18319=CARTESIAN_POINT('Ctrl Pts',(-8.05731678308044,-1.0702161025105,6.45872791928576));
#18320=CARTESIAN_POINT('Ctrl Pts',(-8.02346435712921,-1.28207147709367,
6.46713461983344));
#18321=CARTESIAN_POINT('Ctrl Pts',(-8.00300596344256,-1.41010427049229,
6.47221512985827));
#18322=CARTESIAN_POINT('Ctrl Pts',(-7.97948372510071,-1.53763906534455,
6.4772956398831));
#18323=CARTESIAN_POINT('Ctrl Pts',(-7.95292554614784,-1.6645308107479,6.48237614990793));
#18324=CARTESIAN_POINT('Ctrl Pts',(-7.90993729865206,-1.86992342318004,
6.49059968898189));
#18325=CARTESIAN_POINT('Ctrl Pts',(-7.85898109901696,-2.07368318179469,
6.49882322805586));
#18326=CARTESIAN_POINT('Ctrl Pts',(-7.80020589082835,-2.27518694247015,
6.50704676712982));
#18327=CARTESIAN_POINT('Ctrl Pts',(-7.7414413689935,-2.47665406626185,6.51526881102154));
#18328=CARTESIAN_POINT('Ctrl Pts',(-7.67486075856426,-2.67586572779008,
6.52349085491326));
#18329=CARTESIAN_POINT('Ctrl Pts',(-7.6006631699023,-2.87221289952377,6.53171289880498));
#18330=CARTESIAN_POINT('Ctrl Pts',(-7.52647377323958,-3.06853839298042,
6.53993403491818));
#18331=CARTESIAN_POINT('Ctrl Pts',(-7.44466918153527,-3.26199975226291,
6.54815517103138));
#18332=CARTESIAN_POINT('Ctrl Pts',(-7.35549734391185,-3.45200613936385,
6.55637630714458));
#18333=CARTESIAN_POINT('Ctrl Pts',(-7.26631843361666,-3.64202759683729,
6.56459809531788));
#18334=CARTESIAN_POINT('Ctrl Pts',(-7.16977123275741,-3.82859326646194,
6.57281988349117));
#18335=CARTESIAN_POINT('Ctrl Pts',(-7.06615097551361,-4.0111342477843,6.58104167166447));
#18336=CARTESIAN_POINT('Ctrl Pts',(-6.96253100578854,-4.19367472260383,
6.58926343702449));
#18337=CARTESIAN_POINT('Ctrl Pts',(-6.85183816687966,-4.37219027630242,
6.5974852023845));
#18338=CARTESIAN_POINT('Ctrl Pts',(-6.73441287217018,-4.54613801260462,
6.60570696774452));
#18339=CARTESIAN_POINT('Ctrl Pts',(-6.6169630962361,-4.72012201412216,6.61393044720613));
#18340=CARTESIAN_POINT('Ctrl Pts',(-6.49277822554736,-4.88953605130122,
6.62215392666773));
#18341=CARTESIAN_POINT('Ctrl Pts',(-6.36224171402828,-5.05386663207276,
6.63037740612934));
#18342=CARTESIAN_POINT('Ctrl Pts',(-6.30950012935843,-5.12026227217948,
6.63369999636296));
#18343=CARTESIAN_POINT('Ctrl Pts',(-6.25572213838534,-5.18582841745631,
6.63702258659659));
#18344=CARTESIAN_POINT('Ctrl Pts',(-6.20093491455415,-5.25053271087452,
6.64034517683022));
#18345=CARTESIAN_POINT('Ctrl Pts',(-6.06533442088806,-5.41067833454873,
6.64856871590418));
#18346=CARTESIAN_POINT('Ctrl Pts',(-5.92350469539871,-5.56559412612467,
6.65679225497815));
#18347=CARTESIAN_POINT('Ctrl Pts',(-5.77587342523036,-5.71480303582002,
6.66501579405212));
#18348=CARTESIAN_POINT('Ctrl Pts',(-5.62826899699123,-5.86398481674387,
6.67323783794384));
#18349=CARTESIAN_POINT('Ctrl Pts',(-5.47486533671266,-6.0074615771866,6.68145988183557));
#18350=CARTESIAN_POINT('Ctrl Pts',(-5.31612752467578,-6.14479256801111,
6.68968192572729));
#18351=CARTESIAN_POINT('Ctrl Pts',(-5.15740723854511,-6.28210839641128,
6.69790306184053));
#18352=CARTESIAN_POINT('Ctrl Pts',(-4.99335419939815,-6.41327961698362,
6.70612419795378));
#18353=CARTESIAN_POINT('Ctrl Pts',(-4.82446777350828,-6.53790473048361,
6.71434533406702));
#18354=CARTESIAN_POINT('Ctrl Pts',(-4.65556795237824,-6.6625397286343,6.72256712224032));
#18355=CARTESIAN_POINT('Ctrl Pts',(-4.48183421426568,-6.78062740503495,
6.73078891041362));
#18356=CARTESIAN_POINT('Ctrl Pts',(-4.30379706053266,-6.8918080664112,6.73901069858692));
#18357=CARTESIAN_POINT('Ctrl Pts',(-4.12576040080534,-7.00298841929072,
6.74723246394694));
#18358=CARTESIAN_POINT('Ctrl Pts',(-3.94342060093207,-7.10726164154992,
6.75545422930696));
#18359=CARTESIAN_POINT('Ctrl Pts',(-3.75733550922104,-7.20431241921439,
6.76367599466699));
#18360=CARTESIAN_POINT('Ctrl Pts',(-3.57121162185707,-7.30138343035512,
6.77189947412863));
#18361=CARTESIAN_POINT('Ctrl Pts',(-3.38134114432983,-7.39122885241546,
6.78012295359026));
#18362=CARTESIAN_POINT('Ctrl Pts',(-3.18830577230109,-7.47357972224901,
6.7883464330519));
#18363=CARTESIAN_POINT('Ctrl Pts',(-3.11031233353567,-7.5068525232706,6.79166902328544));
#18364=CARTESIAN_POINT('Ctrl Pts',(-3.03180248393373,-7.53890240992644,
6.79499161351897));
#18365=CARTESIAN_POINT('Ctrl Pts',(-2.95281552569253,-7.56971386736178,
6.79831420375251));
#18366=CARTESIAN_POINT('Ctrl Pts',(-2.7573197552922,-7.6459734137806,6.80653774282647));
#18367=CARTESIAN_POINT('Ctrl Pts',(-2.55883642947032,-7.71466797602978,
6.81476128190043));
#18368=CARTESIAN_POINT('Ctrl Pts',(-2.35796878883899,-7.77558169871304,
6.82298482097439));
#18369=CARTESIAN_POINT('Ctrl Pts',(-2.15713766943384,-7.83648434622343,
6.8312068648661));
#18370=CARTESIAN_POINT('Ctrl Pts',(-1.95392338255781,-7.88960889218248,
6.83942890875781));
#18371=CARTESIAN_POINT('Ctrl Pts',(-1.74894476630273,-7.93478920746621,
6.84765095264953));
#18372=CARTESIAN_POINT('Ctrl Pts',(-1.5439887813034,-7.97996453448684,6.85587208876275));
#18373=CARTESIAN_POINT('Ctrl Pts',(-1.33726914373695,-8.01719731848192,
6.86409322487598));
#18374=CARTESIAN_POINT('Ctrl Pts',(-1.12941615257612,-8.04637227058257,
6.87231436098921));
#18375=CARTESIAN_POINT('Ctrl Pts',(-0.921546675538772,-8.07554953669688,
6.8805361491625));
#18376=CARTESIAN_POINT('Ctrl Pts',(-0.712543957006131,-8.09666765029956,
6.88875793733578));
#18377=CARTESIAN_POINT('Ctrl Pts',(-0.503045768961866,-8.10966291018496,
6.89697972550907));
#18378=CARTESIAN_POINT('Ctrl Pts',(-0.293548162218716,-8.12265813401201,
6.90520149086911));
#18379=CARTESIAN_POINT('Ctrl Pts',(-0.0835553832472526,-8.12753053363892,
6.91342325622916));
#18380=CARTESIAN_POINT('Ctrl Pts',(0.126291879406771,-8.12426845467922,
6.9216450215892));
#18381=CARTESIAN_POINT('Ctrl Pts',(0.336182891731384,-8.12100569563021,
6.92986850105082));
#18382=CARTESIAN_POINT('Ctrl Pts',(0.545928032182363,-8.10960507465031,
6.93809198051246));
#18383=CARTESIAN_POINT('Ctrl Pts',(0.754887711811087,-8.09010705152019,
6.94631545997408));
#18384=CARTESIAN_POINT('Ctrl Pts',(0.839315160555174,-8.08222912812676,
6.94963805020766));
#18385=CARTESIAN_POINT('Ctrl Pts',(0.923614427795624,-8.07302992913747,
6.95296064044122));
#18386=CARTESIAN_POINT('Ctrl Pts',(1.00774356520921,-8.06251452521355,6.95628323067479));
#18387=CARTESIAN_POINT('Ctrl Pts',(1.21596642753791,-8.03648849462657,6.96450676974876));
#18388=CARTESIAN_POINT('Ctrl Pts',(1.4232143473262,-8.00238756714075,6.97273030882273));
#18389=CARTESIAN_POINT('Ctrl Pts',(1.62885407719636,-7.96030916219344,6.98095384789669));
#18390=CARTESIAN_POINT('Ctrl Pts',(1.83445641819157,-7.91823840783107,6.98917589178841));
#18391=CARTESIAN_POINT('Ctrl Pts',(2.03845086405484,-7.86819313002325,6.99739793568012));
#18392=CARTESIAN_POINT('Ctrl Pts',(2.24021412886317,-7.81032190241489,7.00561997957184));
#18393=CARTESIAN_POINT('Ctrl Pts',(2.44195511741554,-7.75245706424656,7.01384111568505));
#18394=CARTESIAN_POINT('Ctrl Pts',(2.64146513332877,-7.68676808259966,7.02206225179827));
#18395=CARTESIAN_POINT('Ctrl Pts',(2.83813502013096,-7.61345369526907,7.03028338791148));
#18396=CARTESIAN_POINT('Ctrl Pts',(3.03482050582152,-7.54013349300177,7.03850517608479));
#18397=CARTESIAN_POINT('Ctrl Pts',(3.22866513500992,-7.45918677712556,7.0467269642581));
#18398=CARTESIAN_POINT('Ctrl Pts',(3.41907774333964,-7.37086120799323,7.0549487524314));
#18399=CARTESIAN_POINT('Ctrl Pts',(3.60948982332529,-7.28253588394074,7.06317051779145));
#18400=CARTESIAN_POINT('Ctrl Pts',(3.79646963508711,-7.18683187414066,7.07139228315149));
#18401=CARTESIAN_POINT('Ctrl Pts',(3.97944823178316,-7.08404399570315,7.07961404851153));
#18402=CARTESIAN_POINT('Ctrl Pts',(4.16246497647897,-6.98123468769939,7.08783752797316));
#18403=CARTESIAN_POINT('Ctrl Pts',(4.34147858245787,-6.87133870517064,7.09606100743479));
#18404=CARTESIAN_POINT('Ctrl Pts',(4.51594588412085,-6.75469616890293,7.10428448689642));
#18405=CARTESIAN_POINT('Ctrl Pts',(4.5864371348482,-6.70756826475614,7.10760707712998));
#18406=CARTESIAN_POINT('Ctrl Pts',(4.65618653868655,-6.65933951416623,7.11092966736354));
#18407=CARTESIAN_POINT('Ctrl Pts',(4.7251596222561,-6.6100343498881,7.1142522575971));
#18408=CARTESIAN_POINT('Ctrl Pts',(4.79993955054399,-6.55657818324849,7.11785457674156));
#18409=CARTESIAN_POINT('Ctrl Pts',(4.87381758274083,-6.50184908894628,7.12145689588603));
#18410=CARTESIAN_POINT('Ctrl Pts',(4.94675008185378,-6.44587862049694,7.1250592150305));
#18411=CARTESIAN_POINT('Ctrl Pts',(4.94675008185377,-6.44587862049696,5.12505864308909));
#18412=CARTESIAN_POINT('Ctrl Pts',(5.11327330421413,-6.31808397645537,5.13328059944019));
#18413=CARTESIAN_POINT('Ctrl Pts',(5.27484659373271,-6.18382917332942,5.1415025557913));
#18414=CARTESIAN_POINT('Ctrl Pts',(5.43097679848903,-6.04352368877411,5.1497245121424));
#18415=CARTESIAN_POINT('Ctrl Pts',(5.58710221449753,-5.90322250759869,5.15794621631375));
#18416=CARTESIAN_POINT('Ctrl Pts',(5.73778466133417,-5.75687121453366,5.16616792048511));
#18417=CARTESIAN_POINT('Ctrl Pts',(5.8825659940448,-5.60491791984572,5.17438962465647));
#18418=CARTESIAN_POINT('Ctrl Pts',(6.02738129098646,-5.45292897845727,5.18261325755616));
#18419=CARTESIAN_POINT('Ctrl Pts',(6.16629250319627,-5.29533562228945,5.19083689045586));
#18420=CARTESIAN_POINT('Ctrl Pts',(6.29887929555683,-5.1326218624116,5.19906052335556));
#18421=CARTESIAN_POINT('Ctrl Pts',(6.40401733559483,-5.00359388386116,5.20558166041357));
#18422=CARTESIAN_POINT('Ctrl Pts',(6.50517923101827,-4.87134688198783,5.2121027974716));
#18423=CARTESIAN_POINT('Ctrl Pts',(6.60217363942672,-4.73613669538359,5.21862393452961));
#18424=CARTESIAN_POINT('Ctrl Pts',(6.72448931848791,-4.56562866237569,5.22684747360358));
#18425=CARTESIAN_POINT('Ctrl Pts',(6.84021601287271,-4.39035200757339,5.23507101267753));
#18426=CARTESIAN_POINT('Ctrl Pts',(6.94899514531588,-4.21083768778568,5.24329455175149));
#18427=CARTESIAN_POINT('Ctrl Pts',(7.05775449982326,-4.03135600681953,5.2515165956432));
#18428=CARTESIAN_POINT('Ctrl Pts',(7.15956866079511,-3.8476384507736,5.25973863953492));
#18429=CARTESIAN_POINT('Ctrl Pts',(7.25412336277317,-3.66024340722969,5.26796068342663));
#18430=CARTESIAN_POINT('Ctrl Pts',(7.34866762516637,-3.47286905357661,5.27618181953985));
#18431=CARTESIAN_POINT('Ctrl Pts',(7.43595389592423,-3.2818182862483,5.28440295565307));
#18432=CARTESIAN_POINT('Ctrl Pts',(7.51571432548066,-3.08767319194646,5.29262409176629));
#18433=CARTESIAN_POINT('Ctrl Pts',(7.59548108124206,-2.89351269901063,5.30084587993959));
#18434=CARTESIAN_POINT('Ctrl Pts',(7.6677206885832,-2.69625766052627,5.30906766811289));
#18435=CARTESIAN_POINT('Ctrl Pts',(7.73221342592157,-2.49651018393641,5.31728945628619));
#18436=CARTESIAN_POINT('Ctrl Pts',(7.79670598430982,-2.29676326159246,5.32551122164622));
#18437=CARTESIAN_POINT('Ctrl Pts',(7.85345162764113,-2.09452419647121,5.33373298700625));
#18438=CARTESIAN_POINT('Ctrl Pts',(7.90228033600609,-1.89041081611153,5.34195475236629));
#18439=CARTESIAN_POINT('Ctrl Pts',(7.95111922434617,-1.68625488150042,5.35017823182791));
#18440=CARTESIAN_POINT('Ctrl Pts',(7.99203781176432,-1.48022413790811,5.35840171128954));
#18441=CARTESIAN_POINT('Ctrl Pts',(8.02491684026517,-1.2729482587004,5.36662519075116));
#18442=CARTESIAN_POINT('Ctrl Pts',(8.03820118535247,-1.18920112768048,5.36994778098474));
#18443=CARTESIAN_POINT('Ctrl Pts',(8.05017368940018,-1.10525083961553,5.37327037121832));
#18444=CARTESIAN_POINT('Ctrl Pts',(8.06082887240659,-1.02113929131937,5.37659296145191));
#18445=CARTESIAN_POINT('Ctrl Pts',(8.08720086161786,-0.812959962735982,
5.38481650052586));
#18446=CARTESIAN_POINT('Ctrl Pts',(8.10550815197252,-0.603724648719067,
5.39304003959982));
#18447=CARTESIAN_POINT('Ctrl Pts',(8.11568824050388,-0.394070990364645,
5.40126357867378));
#18448=CARTESIAN_POINT('Ctrl Pts',(8.12586647811832,-0.184455450687011,
5.40948562256549));
#18449=CARTESIAN_POINT('Ctrl Pts',(8.12792044886564,0.0255779870747951,
5.41770766645721));
#18450=CARTESIAN_POINT('Ctrl Pts',(8.12183967716184,0.235388659411679,5.42592971034892));
#18451=CARTESIAN_POINT('Ctrl Pts',(8.1157595768232,0.445176166995444,5.43415084646213));
#18452=CARTESIAN_POINT('Ctrl Pts',(8.10154653567723,0.654740663561258,5.44237198257534));
#18453=CARTESIAN_POINT('Ctrl Pts',(8.07924217894022,0.863442746528816,5.45059311868856));
#18454=CARTESIAN_POINT('Ctrl Pts',(8.05693605313133,1.07216138271922,5.45881490686185));
#18455=CARTESIAN_POINT('Ctrl Pts',(8.02653735813692,1.28001717508234,5.46703669503515));
#18456=CARTESIAN_POINT('Ctrl Pts',(7.98813957405315,1.48637603181224,5.47525848320845));
#18457=CARTESIAN_POINT('Ctrl Pts',(7.94974189651298,1.69273431595145,5.48348024856849));
#18458=CARTESIAN_POINT('Ctrl Pts',(7.90334523088579,1.89759538330417,5.49170201392852));
#18459=CARTESIAN_POINT('Ctrl Pts',(7.84909424822766,2.10033498398221,5.49992377928855));
#18460=CARTESIAN_POINT('Ctrl Pts',(7.79483195514024,2.30311685250138,5.50814725875018));
#18461=CARTESIAN_POINT('Ctrl Pts',(7.73271215002935,2.50377608581617,5.5163707382118));
#18462=CARTESIAN_POINT('Ctrl Pts',(7.66292978250387,2.70170218768004,5.52459421767343));
#18463=CARTESIAN_POINT('Ctrl Pts',(7.63473512184973,2.7816716624132,5.52791680790702));
#18464=CARTESIAN_POINT('Ctrl Pts',(7.60529014342423,2.86119514928919,5.5312393981406));
#18465=CARTESIAN_POINT('Ctrl Pts',(7.57460997759708,2.94023319649765,5.53456198837419));
#18466=CARTESIAN_POINT('Ctrl Pts',(7.49867538297727,3.13585541406091,5.54278552744815));
#18467=CARTESIAN_POINT('Ctrl Pts',(7.41514618317771,3.32856619812029,5.55100906652211));
#18468=CARTESIAN_POINT('Ctrl Pts',(7.32427102991529,3.51777506996164,5.55923260559608));
#18469=CARTESIAN_POINT('Ctrl Pts',(7.23341239933428,3.70694954034342,5.56745464948779));
#18470=CARTESIAN_POINT('Ctrl Pts',(7.13521060866594,3.89262310357579,5.5756766933795));
#18471=CARTESIAN_POINT('Ctrl Pts',(7.02996149969404,4.07422739612304,5.58389873727121));
#18472=CARTESIAN_POINT('Ctrl Pts',(6.92472401105381,4.25581163812419,5.59211987338444));
#18473=CARTESIAN_POINT('Ctrl Pts',(6.81244090534801,4.43332725133232,5.60034100949766));
#18474=CARTESIAN_POINT('Ctrl Pts',(6.69345323946345,4.60623178895898,5.60856214561088));
#18475=CARTESIAN_POINT('Ctrl Pts',(6.57445613606251,4.77915004052309,5.61678393378418));
#18476=CARTESIAN_POINT('Ctrl Pts',(6.44875357497336,4.94745624127609,5.62500572195748));
#18477=CARTESIAN_POINT('Ctrl Pts',(6.31672968358794,5.11063730536407,5.63322751013078));
#18478=CARTESIAN_POINT('Ctrl Pts',(6.18470615853356,5.2738179166682,5.64144927549082));
#18479=CARTESIAN_POINT('Ctrl Pts',(6.04636152587247,5.43187319216415,5.64967104085084));
#18480=CARTESIAN_POINT('Ctrl Pts',(5.9021202421595,5.58432307532355,5.65789280621088));
#18481=CARTESIAN_POINT('Ctrl Pts',(5.7578488865334,5.73680474175279,5.6661162856725));
#18482=CARTESIAN_POINT('Ctrl Pts',(5.60767862669683,5.88367846697999,5.67433976513413));
#18483=CARTESIAN_POINT('Ctrl Pts',(5.45207158345308,6.02450022918112,5.68256324459576));
#18484=CARTESIAN_POINT('Ctrl Pts',(5.389200575558,6.08139743600792,5.68588583482933));
#18485=CARTESIAN_POINT('Ctrl Pts',(5.32544244321428,6.1373071156651,5.6892084250629));
#18486=CARTESIAN_POINT('Ctrl Pts',(5.26082927658751,6.19220178006981,5.69253101529648));
#18487=CARTESIAN_POINT('Ctrl Pts',(5.10090919523702,6.32806819330439,5.70075455437044));
#18488=CARTESIAN_POINT('Ctrl Pts',(4.93569698852641,6.45775820936455,5.70897809344439));
#18489=CARTESIAN_POINT('Ctrl Pts',(4.76569246948587,6.58087097949698,5.71720163251835));
#18490=CARTESIAN_POINT('Ctrl Pts',(4.59571886022002,6.70396136558925,5.72542367641005));
#18491=CARTESIAN_POINT('Ctrl Pts',(4.42095491644826,6.82047671964672,5.73364572030177));
#18492=CARTESIAN_POINT('Ctrl Pts',(4.24193141818231,6.93005810985289,5.74186776419347));
#18493=CARTESIAN_POINT('Ctrl Pts',(4.06292768552231,7.03962740140945,5.75008890030669));
#18494=CARTESIAN_POINT('Ctrl Pts',(3.87966558873464,7.14226410361958,5.75831003641991));
#18495=CARTESIAN_POINT('Ctrl Pts',(3.69270332797605,7.23765360417688,5.76653117253313));
#18496=CARTESIAN_POINT('Ctrl Pts',(3.50572623829061,7.33305067056014,5.77475296070643));
#18497=CARTESIAN_POINT('Ctrl Pts',(3.31504865975612,7.42119925035857,5.78297474887973));
#18498=CARTESIAN_POINT('Ctrl Pts',(3.12125268683624,7.50183105830953,5.79119653705303));
#18499=CARTESIAN_POINT('Ctrl Pts',(2.92745725164848,7.58246264252875,5.79941830241306));
#18500=CARTESIAN_POINT('Ctrl Pts',(2.73054371272274,7.6555773858157,5.80764006777308));
#18501=CARTESIAN_POINT('Ctrl Pts',(2.53111390148152,7.72095525050023,5.81586183313311));
#18502=CARTESIAN_POINT('Ctrl Pts',(2.33164251243531,7.78634674538423,5.82408531259473));
#18503=CARTESIAN_POINT('Ctrl Pts',(2.12965408337915,7.8439980474413,5.83230879205635));
#18504=CARTESIAN_POINT('Ctrl Pts',(1.92576640824912,7.89373874050562,5.84053227151798));
#18505=CARTESIAN_POINT('Ctrl Pts',(1.84338823714769,7.9138358224962,5.84385486175158));
#18506=CARTESIAN_POINT('Ctrl Pts',(1.76070017561212,7.93264210333362,5.84717745198518));
#18507=CARTESIAN_POINT('Ctrl Pts',(1.67774353105856,7.95014869084165,5.85050004221878));
#18508=CARTESIAN_POINT('Ctrl Pts',(1.47242263381648,7.9934781706457,5.85872358129273));
#18509=CARTESIAN_POINT('Ctrl Pts',(1.26538894703182,8.02885649802595,5.86694712036669));
#18510=CARTESIAN_POINT('Ctrl Pts',(1.05727285280546,8.05616916885567,5.87517065944065));
#18511=CARTESIAN_POINT('Ctrl Pts',(0.849194597700014,8.0834768737674,5.88339270333236));
#18512=CARTESIAN_POINT('Ctrl Pts',(0.64003462022648,8.10272181068945,5.89161474722407));
#18513=CARTESIAN_POINT('Ctrl Pts',(0.430430574832467,8.1138410806935,5.89983679111578));
#18514=CARTESIAN_POINT('Ctrl Pts',(0.220849671378751,8.12495912304241,5.90805792722898));
#18515=CARTESIAN_POINT('Ctrl Pts',(0.0108250922942836,8.12795327395779,
5.91627906334217));
#18516=CARTESIAN_POINT('Ctrl Pts',(-0.19900249857376,8.12281266360744,5.92450019945537));
#18517=CARTESIAN_POINT('Ctrl Pts',(-0.40884673193482,8.11767164552915,5.93272198762866));
#18518=CARTESIAN_POINT('Ctrl Pts',(-0.618493650941377,8.10439458157231,
5.94094377580196));
#18519=CARTESIAN_POINT('Ctrl Pts',(-0.827303638729489,8.08302271751385,
5.94916556397526));
#18520=CARTESIAN_POINT('Ctrl Pts',(-1.03611304712544,8.06165091275662,5.95738732933529));
#18521=CARTESIAN_POINT('Ctrl Pts',(-1.24408523582356,8.03218438553973,5.96560909469531));
#18522=CARTESIAN_POINT('Ctrl Pts',(-1.45058620523406,7.99471620657573,5.97383086005534));
#18523=CARTESIAN_POINT('Ctrl Pts',(-1.65713022666894,7.95724021611836,5.98205433951696));
#18524=CARTESIAN_POINT('Ctrl Pts',(-1.86220212582129,7.91175929396889,5.99027781897859));
#18525=CARTESIAN_POINT('Ctrl Pts',(-2.06517749367339,7.85841774673024,5.99850129844022));
#18526=CARTESIAN_POINT('Ctrl Pts',(-2.14718705885023,7.83686578630671,6.00182388867383));
#18527=CARTESIAN_POINT('Ctrl Pts',(-2.22885451172286,7.81403118841705,6.00514647890743));
#18528=CARTESIAN_POINT('Ctrl Pts',(-2.31013929405932,7.7899258022489,6.00846906914104));
#18529=CARTESIAN_POINT('Ctrl Pts',(-2.51132226778267,7.73026404105987,6.016692608215));
#18530=CARTESIAN_POINT('Ctrl Pts',(-2.71022544243532,7.66279478417243,6.02491614728895));
#18531=CARTESIAN_POINT('Ctrl Pts',(-2.90623996210263,7.58771749903604,6.0331396863629));
#18532=CARTESIAN_POINT('Ctrl Pts',(-3.10221884292558,7.51265386425415,6.04136173025461));
#18533=CARTESIAN_POINT('Ctrl Pts',(-3.29530984173093,7.42998506751543,6.04958377414633));
#18534=CARTESIAN_POINT('Ctrl Pts',(-3.48492227952547,7.33995941870028,6.05780581803804));
#18535=CARTESIAN_POINT('Ctrl Pts',(-3.67451378261095,7.24994370942702,6.06602695415124));
#18536=CARTESIAN_POINT('Ctrl Pts',(-3.86062722512228,7.15257289616183,6.07424809026443));
#18537=CARTESIAN_POINT('Ctrl Pts',(-4.04269405550415,7.04814247416235,6.08246922637763));
#18538=CARTESIAN_POINT('Ctrl Pts',(-4.22477532653196,6.94370376925518,6.09069101455093));
#18539=CARTESIAN_POINT('Ctrl Pts',(-4.40280908696486,6.83220448126467,6.09891280272423));
#18540=CARTESIAN_POINT('Ctrl Pts',(-4.57625252091034,6.71398543544456,6.10713459089753));
#18541=CARTESIAN_POINT('Ctrl Pts',(-4.74969547359642,6.59576671765087,6.11535635625755));
#18542=CARTESIAN_POINT('Ctrl Pts',(-4.91854788308649,6.47082844766323,6.12357812161758));
#18543=CARTESIAN_POINT('Ctrl Pts',(-5.08229654968902,6.339554348968,6.1317998869776));
#18544=CARTESIAN_POINT('Ctrl Pts',(-5.24607935517029,6.20825288180235,6.14002336643922));
#18545=CARTESIAN_POINT('Ctrl Pts',(-5.40475606194957,6.07061313163142,6.14824684590084));
#18546=CARTESIAN_POINT('Ctrl Pts',(-5.55784630003058,5.92705931029346,6.15647032536246));
#18547=CARTESIAN_POINT('Ctrl Pts',(-5.61970042543883,5.86905825040111,6.15979291559608));
#18548=CARTESIAN_POINT('Ctrl Pts',(-5.68064297885062,5.81009218470904,6.16311550582971));
#18549=CARTESIAN_POINT('Ctrl Pts',(-5.74064393689372,5.75019084485945,6.16643809606334));
#18550=CARTESIAN_POINT('Ctrl Pts',(-5.8891486239747,5.60193271665247,6.1746616351373));
#18551=CARTESIAN_POINT('Ctrl Pts',(-6.03193098122543,5.4478945007128,6.18288517421126));
#18552=CARTESIAN_POINT('Ctrl Pts',(-6.16855058045022,5.2885415096156,6.19110871328523));
#18553=CARTESIAN_POINT('Ctrl Pts',(-6.30514533985905,5.12921749165983,6.19933075717696));
#18554=CARTESIAN_POINT('Ctrl Pts',(-6.43557938575343,4.96458085100612,6.2075528010687));
#18555=CARTESIAN_POINT('Ctrl Pts',(-6.5594515304958,4.79513119544985,6.21577484496043));
#18556=CARTESIAN_POINT('Ctrl Pts',(-6.68330999877533,4.62570024847347,6.2239959810736));
#18557=CARTESIAN_POINT('Ctrl Pts',(-6.80060783832332,4.45145758551055,6.23221711718678));
#18558=CARTESIAN_POINT('Ctrl Pts',(-6.91098578698644,4.27293377137669,6.24043825329995));
#18559=CARTESIAN_POINT('Ctrl Pts',(-7.02137249028616,4.09439579761098,6.24866004147324));
#18560=CARTESIAN_POINT('Ctrl Pts',(-7.12483804868518,3.91157624367483,6.25688182964653));
#18561=CARTESIAN_POINT('Ctrl Pts',(-7.22106741500805,3.7250332817854,6.26510361781983));
#18562=CARTESIAN_POINT('Ctrl Pts',(-7.31729651432003,3.53849083750306,6.27332538317985));
#18563=CARTESIAN_POINT('Ctrl Pts',(-7.40628932890439,3.34822526928211,6.28154714853988));
#18564=CARTESIAN_POINT('Ctrl Pts',(-7.48777728107325,3.15481837061079,6.2897689138999));
#18565=CARTESIAN_POINT('Ctrl Pts',(-7.56928222212754,2.96137114981138,6.29799239336153));
#18566=CARTESIAN_POINT('Ctrl Pts',(-7.64327906053075,2.76478156207116,6.30621587282316));
#18567=CARTESIAN_POINT('Ctrl Pts',(-7.70954736643835,2.56565137287657,6.31443935228479));
#18568=CARTESIAN_POINT('Ctrl Pts',(-7.73632221606669,2.48519540227155,6.31776194251841));
#18569=CARTESIAN_POINT('Ctrl Pts',(-7.76183597327306,2.40432488902521,6.32108453275202));
#18570=CARTESIAN_POINT('Ctrl Pts',(-7.78607639342532,2.32308027374107,6.32440712298563));
#18571=CARTESIAN_POINT('Ctrl Pts',(-7.84637220828773,2.12099176822143,6.3326717604932));
#18572=CARTESIAN_POINT('Ctrl Pts',(-7.89880495416801,1.916524583584,6.34093639800078));
#18573=CARTESIAN_POINT('Ctrl Pts',(-7.94320769728739,1.71030378595568,6.34920103550835));
#18574=CARTESIAN_POINT('Ctrl Pts',(-7.98760119827069,1.50412591181677,6.35746395278651));
#18575=CARTESIAN_POINT('Ctrl Pts',(-8.02396797252378,1.2961954355431,6.36572687006468));
#18576=CARTESIAN_POINT('Ctrl Pts',(-8.05219193447165,1.08714884580252,6.37398978734284));
#18577=CARTESIAN_POINT('Ctrl Pts',(-8.0804132772077,0.878121655793909,6.38225193781404));
#18578=CARTESIAN_POINT('Ctrl Pts',(-8.1004932758947,0.667978844956448,6.39051408828524));
#18579=CARTESIAN_POINT('Ctrl Pts',(-8.11236743935685,0.457364287371444,
6.39877623875644));
#18580=CARTESIAN_POINT('Ctrl Pts',(-8.1209551967177,0.305041412335285,6.40475167810016));
#18581=CARTESIAN_POINT('Ctrl Pts',(-8.12525186452795,0.152471955905835,
6.41072711744389));
#18582=CARTESIAN_POINT('Ctrl Pts',(-8.12524999939287,-9.93285784619588E-5,
6.41670255678762));
#18583=CARTESIAN_POINT('Origin',(0.,0.,-16.4167025567876));
#18584=CARTESIAN_POINT('',(4.94669362673306,-6.44580471440964,3.12504817176739));
#18585=CARTESIAN_POINT('',(4.94675008185372,-6.44587862049699,3.29164655258555));
#18586=CARTESIAN_POINT('',(4.94675008185374,-6.44587862049697,-16.4167025567876));
#18587=CARTESIAN_POINT('',(-8.12524999971641,6.78850738286463E-5,4.58329744324838));
#18588=CARTESIAN_POINT('Ctrl Pts',(4.94675008185374,-6.44587862049698,3.29164655258555));
#18589=CARTESIAN_POINT('Ctrl Pts',(5.08212104463498,-6.34199110404742,3.29833220814838));
#18590=CARTESIAN_POINT('Ctrl Pts',(5.21420479585878,-6.23384795954413,3.30501786371122));
#18591=CARTESIAN_POINT('Ctrl Pts',(5.3427373285523,-6.12167014797382,3.31170351927405));
#18592=CARTESIAN_POINT('Ctrl Pts',(5.50083585680398,-5.98368837370932,3.31992705834802));
#18593=CARTESIAN_POINT('Ctrl Pts',(5.65361192257898,-5.83955632578681,3.32815059742199));
#18594=CARTESIAN_POINT('Ctrl Pts',(5.8005949295409,-5.68970878216841,3.33637413649596));
#18595=CARTESIAN_POINT('Ctrl Pts',(5.94755121243908,-5.53988848343627,3.34459618038769));
#18596=CARTESIAN_POINT('Ctrl Pts',(6.0887163323222,-5.38435497353434,3.35281822427941));
#18597=CARTESIAN_POINT('Ctrl Pts',(6.22365654899584,-5.22357987616167,3.36104026817114));
#18598=CARTESIAN_POINT('Ctrl Pts',(6.35858186720471,-5.06282252962847,3.36926140428433));
#18599=CARTESIAN_POINT('Ctrl Pts',(6.48728346479563,-4.89682497682462,3.37748254039753));
#18600=CARTESIAN_POINT('Ctrl Pts',(6.60936736013709,-4.72609253625597,3.38570367651073));
#18601=CARTESIAN_POINT('Ctrl Pts',(6.73146093857325,-4.55534655402907,3.39392546468404));
#18602=CARTESIAN_POINT('Ctrl Pts',(6.8469355922835,-4.37986517203383,3.40214725285737));
#18603=CARTESIAN_POINT('Ctrl Pts',(6.95543960683962,-4.20018421478233,3.41036904103068));
#18604=CARTESIAN_POINT('Ctrl Pts',(7.06394332032602,-4.0205037560976,3.41859080639073));
#18605=CARTESIAN_POINT('Ctrl Pts',(7.16547628319758,-3.83662399933009,3.42681257175077));
#18606=CARTESIAN_POINT('Ctrl Pts',(7.25973156458414,-3.64910744877165,3.43503433711082));
#18607=CARTESIAN_POINT('Ctrl Pts',(7.35400649663197,-3.46155180412571,3.44325781657244));
#18608=CARTESIAN_POINT('Ctrl Pts',(7.4410005836328,-3.27035811456371,3.45148129603406));
#18609=CARTESIAN_POINT('Ctrl Pts',(7.52045359721303,-3.07611203545411,3.45970477549568));
#18610=CARTESIAN_POINT('Ctrl Pts',(7.55255555699539,-2.99762942619271,3.46302736572923));
#18611=CARTESIAN_POINT('Ctrl Pts',(7.58342701162677,-2.91864876395072,3.46634995596279));
#18612=CARTESIAN_POINT('Ctrl Pts',(7.61305303611869,-2.83920957869332,3.46967254619634));
#18613=CARTESIAN_POINT('Ctrl Pts',(7.68637859024654,-2.64259452897409,3.47789608527028));
#18614=CARTESIAN_POINT('Ctrl Pts',(7.75209530064891,-2.44310546289366,3.48611962434423));
#18615=CARTESIAN_POINT('Ctrl Pts',(7.80999636316043,-2.24134878363917,3.49434316341818));
#18616=CARTESIAN_POINT('Ctrl Pts',(7.86788689825338,-2.03962878725234,3.50256520730992));
#18617=CARTESIAN_POINT('Ctrl Pts',(7.9179645403325,-1.83564228392911,3.51078725120166));
#18618=CARTESIAN_POINT('Ctrl Pts',(7.96007243934189,-1.63001052847204,3.51900929509341));
#18619=CARTESIAN_POINT('Ctrl Pts',(8.00217568930684,-1.42440147638395,3.52723043120661));
#18620=CARTESIAN_POINT('Ctrl Pts',(8.03631089379098,-1.21714782364372,3.53545156731982));
#18621=CARTESIAN_POINT('Ctrl Pts',(8.0623722088047,-1.00888152386375,3.54367270343301));
#18622=CARTESIAN_POINT('Ctrl Pts',(8.08843559087381,-0.800598705424667,
3.55189449160631));
#18623=CARTESIAN_POINT('Ctrl Pts',(8.10642376468057,-0.591303371794449,
3.56011627977961));
#18624=CARTESIAN_POINT('Ctrl Pts',(8.11628257995049,-0.381634176787381,
3.56833806795291));
#18625=CARTESIAN_POINT('Ctrl Pts',(8.12614136786481,-0.171965563556886,
3.57655983331292));
#18626=CARTESIAN_POINT('Ctrl Pts',(8.12787083120482,0.0380766142421395,
3.58478159867294));
#18627=CARTESIAN_POINT('Ctrl Pts',(8.12146890433173,0.247851565403032,3.59300336403296));
#18628=CARTESIAN_POINT('Ctrl Pts',(8.11506564276316,0.457670251159153,3.60122684349457));
#18629=CARTESIAN_POINT('Ctrl Pts',(8.10052761333665,0.667221304131454,3.60945032295619));
#18630=CARTESIAN_POINT('Ctrl Pts',(8.07790484229059,0.875865812438278,3.61767380241781));
#18631=CARTESIAN_POINT('Ctrl Pts',(8.06876440502367,0.960165920297958,3.62099639265142));
#18632=CARTESIAN_POINT('Ctrl Pts',(8.05830475824943,1.04431808906881,3.62431898288502));
#18633=CARTESIAN_POINT('Ctrl Pts',(8.0465315997878,1.12828045100338,3.62764157311863));
#18634=CARTESIAN_POINT('Ctrl Pts',(8.0173925781733,1.33609053758197,3.63586511219259));
#18635=CARTESIAN_POINT('Ctrl Pts',(7.98019415312815,1.5428049557683,3.64408865126656));
#18636=CARTESIAN_POINT('Ctrl Pts',(7.93504320927252,1.74779198690176,3.65231219034052));
#18637=CARTESIAN_POINT('Ctrl Pts',(7.8899004746428,1.95274174783213,3.66053423423223));
#18638=CARTESIAN_POINT('Ctrl Pts',(7.83680817047664,2.15596446066753,3.66875627812394));
#18639=CARTESIAN_POINT('Ctrl Pts',(7.77592418080798,2.35683913257263,3.67697832201565));
#18640=CARTESIAN_POINT('Ctrl Pts',(7.71504691321255,2.55769162632774,3.68519945812879));
#18641=CARTESIAN_POINT('Ctrl Pts',(7.64637976311568,2.75619631457534,3.69342059424192));
#18642=CARTESIAN_POINT('Ctrl Pts',(7.57013056164728,2.95174708301944,3.70164173035506));
#18643=CARTESIAN_POINT('Ctrl Pts',(7.49387531246663,3.14731336159029,3.70986351852835));
#18644=CARTESIAN_POINT('Ctrl Pts',(7.41003691499807,3.33992497646865,3.71808530670165));
#18645=CARTESIAN_POINT('Ctrl Pts',(7.31887184821249,3.52899453555013,3.72630709487493));
#18646=CARTESIAN_POINT('Ctrl Pts',(7.22770703438496,3.71806357001544,3.73452886023501));
#18647=CARTESIAN_POINT('Ctrl Pts',(7.12921572243173,3.903590303853,3.74275062559509));
#18648=CARTESIAN_POINT('Ctrl Pts',(7.02370121033173,4.08501026565228,3.75097239095517));
#18649=CARTESIAN_POINT('Ctrl Pts',(6.91816470020808,4.26646805050104,3.7591958704168));
#18650=CARTESIAN_POINT('Ctrl Pts',(6.80560221315041,4.44381709788767,3.76741934987843));
#18651=CARTESIAN_POINT('Ctrl Pts',(6.68636195994309,4.61651939269468,3.77564282934006));
#18652=CARTESIAN_POINT('Ctrl Pts',(6.63818448195345,4.68629751529189,3.77896541957368));
#18653=CARTESIAN_POINT('Ctrl Pts',(6.58891738198813,4.75531740069121,3.7822880098073));
#18654=CARTESIAN_POINT('Ctrl Pts',(6.53858560593556,4.82354494499142,3.78561060004092));
#18655=CARTESIAN_POINT('Ctrl Pts',(6.4140125174933,4.9924107505897,3.79383413911488));
#18656=CARTESIAN_POINT('Ctrl Pts',(6.28287399612001,5.15647556011302,3.80205767818884));
#18657=CARTESIAN_POINT('Ctrl Pts',(6.14556482666594,5.31523475716232,3.8102812172628));
#18658=CARTESIAN_POINT('Ctrl Pts',(6.00828062240444,5.47396508903138,3.81850326115448));
#18659=CARTESIAN_POINT('Ctrl Pts',(5.86482820214791,5.62739151079798,3.82672530504616));
#18660=CARTESIAN_POINT('Ctrl Pts',(5.71564209059604,5.77504312145866,3.83494734893784));
#18661=CARTESIAN_POINT('Ctrl Pts',(5.5664724503674,5.9226784302171,3.84316848505104));
#18662=CARTESIAN_POINT('Ctrl Pts',(5.41157059223792,6.06453999339521,3.85138962116423));
#18663=CARTESIAN_POINT('Ctrl Pts',(5.25140787806196,6.20019377606287,3.85961075727743));
#18664=CARTESIAN_POINT('Ctrl Pts',(5.09123246056684,6.33585831812173,3.86783254545073));
#18665=CARTESIAN_POINT('Ctrl Pts',(4.92579557664273,6.46531390322236,3.87605433362403));
#18666=CARTESIAN_POINT('Ctrl Pts',(4.75560245261724,6.58816612382846,3.88427612179732));
#18667=CARTESIAN_POINT('Ctrl Pts',(4.58540980083205,6.71101800355257,3.89249788715736));
#18668=CARTESIAN_POINT('Ctrl Pts',(4.41046117606165,6.82726638500032,3.9007196525174));
#18669=CARTESIAN_POINT('Ctrl Pts',(4.23129206177159,6.93655930923168,3.90894141787744));
#18670=CARTESIAN_POINT('Ctrl Pts',(4.05208559369574,7.04587501922328,3.91716489733906));
#18671=CARTESIAN_POINT('Ctrl Pts',(3.86865713013893,7.14823222150355,3.92538837680069));
#18672=CARTESIAN_POINT('Ctrl Pts',(3.68156905197642,7.24332360715918,3.93361185626231));
#18673=CARTESIAN_POINT('Ctrl Pts',(3.60597854017021,7.28174404837952,3.93693444649594));
#18674=CARTESIAN_POINT('Ctrl Pts',(3.5297908921433,7.31897889775098,3.94025703672957));
#18675=CARTESIAN_POINT('Ctrl Pts',(3.45304428304078,7.35501004362736,3.9435796269632));
#18676=CARTESIAN_POINT('Ctrl Pts',(3.26309346323797,7.44418852040556,3.95180316603715));
#18677=CARTESIAN_POINT('Ctrl Pts',(3.06965525391331,7.52601903234945,3.96002670511109));
#18678=CARTESIAN_POINT('Ctrl Pts',(2.87331708854787,7.60024581649559,3.96825024418503));
#18679=CARTESIAN_POINT('Ctrl Pts',(2.67701462087164,7.67445910492293,3.97647228807672));
#18680=CARTESIAN_POINT('Ctrl Pts',(2.47781352525126,7.7410713205985,3.9846943319684));
#18681=CARTESIAN_POINT('Ctrl Pts',(2.2763201272324,7.79987527085252,3.99291637586009));
#18682=CARTESIAN_POINT('Ctrl Pts',(2.07484897567346,7.85867272868676,4.00113751197329));
#18683=CARTESIAN_POINT('Ctrl Pts',(1.87108631001129,7.90966355964353,4.0093586480865));
#18684=CARTESIAN_POINT('Ctrl Pts',(1.6656532951312,7.9526905298093,4.01757978419971));
#18685=CARTESIAN_POINT('Ctrl Pts',(1.46020398631403,7.99572091266288,4.02580157237302));
#18686=CARTESIAN_POINT('Ctrl Pts',(1.2530843517001,8.03078610956598,4.03402336054634));
#18687=CARTESIAN_POINT('Ctrl Pts',(1.04492646663933,8.05777985811332,4.04224514871966));
#18688=CARTESIAN_POINT('Ctrl Pts',(0.836769159161336,8.08477353176017,4.0504669140797));
#18689=CARTESIAN_POINT('Ctrl Pts',(0.627573899829079,8.10369576659661,4.05868867943974));
#18690=CARTESIAN_POINT('Ctrl Pts',(0.417979158978247,8.1144920349434,4.06691044479978));
#18691=CARTESIAN_POINT('Ctrl Pts',(0.208340721103928,8.12529055413288,4.07513392426139));
#18692=CARTESIAN_POINT('Ctrl Pts',(-0.0016970700738789,8.12795970727399,
4.083357403723));
#18693=CARTESIAN_POINT('Ctrl Pts',(-0.211493351870177,8.12249703752576,
4.09158088318461));
#18694=CARTESIAN_POINT('Ctrl Pts',(-0.29625881887258,8.12028991665438,4.09490347341824));
#18695=CARTESIAN_POINT('Ctrl Pts',(-0.380984862473706,8.1167559026096,4.09822606365188));
#18696=CARTESIAN_POINT('Ctrl Pts',(-0.465629288968856,8.11189724588239,
4.10154865388551));
#18697=CARTESIAN_POINT('Ctrl Pts',(-0.675127511659835,8.09987188294756,
4.10977219295946));
#18698=CARTESIAN_POINT('Ctrl Pts',(-0.88419366157695,8.0797244644846,4.11799573203341));
#18699=CARTESIAN_POINT('Ctrl Pts',(-1.09218938944958,8.05150979009985,4.12621927110737));
#18700=CARTESIAN_POINT('Ctrl Pts',(-1.30014730008499,8.02330024563312,4.13444131499905));
#18701=CARTESIAN_POINT('Ctrl Pts',(-1.50703488500452,7.98702641236962,4.14266335889072));
#18702=CARTESIAN_POINT('Ctrl Pts',(-1.71222030883513,7.94279479632406,4.15088540278239));
#18703=CARTESIAN_POINT('Ctrl Pts',(-1.91738307858027,7.89856806379698,4.15910653889572));
#18704=CARTESIAN_POINT('Ctrl Pts',(-2.12084377423616,7.84638536471089,4.16732767500905));
#18705=CARTESIAN_POINT('Ctrl Pts',(-2.32198129926246,7.7864042027354,4.17554881112237));
#18706=CARTESIAN_POINT('Ctrl Pts',(-2.52313477752521,7.72641828334996,4.18377059929566));
#18707=CARTESIAN_POINT('Ctrl Pts',(-2.7219644335846,7.65863274693165,4.19199238746896));
#18708=CARTESIAN_POINT('Ctrl Pts',(-2.91786384686345,7.58325511463693,4.20021417564225));
#18709=CARTESIAN_POINT('Ctrl Pts',(-3.11376271657489,7.50787769149458,4.20843594100233));
#18710=CARTESIAN_POINT('Ctrl Pts',(-3.30673108547964,7.42490832304518,4.21665770636239));
#18711=CARTESIAN_POINT('Ctrl Pts',(-3.49618154311534,7.33460306902014,4.22487947172247));
#18712=CARTESIAN_POINT('Ctrl Pts',(-3.6856714980252,7.24427898784936,4.23310295118408));
#18713=CARTESIAN_POINT('Ctrl Pts',(-3.87164181020962,7.14661609270801,4.2413264306457));
#18714=CARTESIAN_POINT('Ctrl Pts',(-4.05352775913069,7.04191737160107,4.24954991010731));
#18715=CARTESIAN_POINT('Ctrl Pts',(-4.12701641807567,6.99961521108211,4.25287250034081));
#18716=CARTESIAN_POINT('Ctrl Pts',(-4.19983860586707,6.9561650018275,4.2561950905743));
#18717=CARTESIAN_POINT('Ctrl Pts',(-4.27195829051431,6.91158881347885,4.2595176808078));
#18718=CARTESIAN_POINT('Ctrl Pts',(-4.45045729370785,6.80126102675432,4.26774121988178));
#18719=CARTESIAN_POINT('Ctrl Pts',(-4.6247090100639,6.68399674037906,4.27596475895575));
#18720=CARTESIAN_POINT('Ctrl Pts',(-4.79417819205573,6.56014809477021,4.28418829802973));
#18721=CARTESIAN_POINT('Ctrl Pts',(-4.96361656160669,6.43632196699632,4.29241034192147));
#18722=CARTESIAN_POINT('Ctrl Pts',(-5.12827389430558,6.30591404330055,4.30063238581321));
#18723=CARTESIAN_POINT('Ctrl Pts',(-5.28764529084683,6.16931883117458,4.30885442970495));
#18724=CARTESIAN_POINT('Ctrl Pts',(-5.44699909152857,6.03273870023768,4.31707556581817));
#18725=CARTESIAN_POINT('Ctrl Pts',(-5.6010678973565,5.88997283656444,4.3252967019314));
#18726=CARTESIAN_POINT('Ctrl Pts',(-5.74938053502141,5.74145547975572,4.33351783804462));
#18727=CARTESIAN_POINT('Ctrl Pts',(-5.89770493611548,5.59292634328051,4.34173962621794));
#18728=CARTESIAN_POINT('Ctrl Pts',(-6.04027204652823,5.4386450090076,4.34996141439125));
#18729=CARTESIAN_POINT('Ctrl Pts',(-6.17664741440262,5.27908271204889,4.35818320256457));
#18730=CARTESIAN_POINT('Ctrl Pts',(-6.31302240387277,5.11952085783178,4.36640496792468));
#18731=CARTESIAN_POINT('Ctrl Pts',(-6.4432054956,4.95467829619373,4.37462673328479));
#18732=CARTESIAN_POINT('Ctrl Pts',(-6.56680206628266,4.78505989354008,4.3828484986449));
#18733=CARTESIAN_POINT('Ctrl Pts',(-6.69042440479803,4.61540612826592,4.39107197810657));
#18734=CARTESIAN_POINT('Ctrl Pts',(-6.80745730532773,4.44097477129257,4.39929545756824));
#18735=CARTESIAN_POINT('Ctrl Pts',(-6.91754844226356,4.26230115212863,4.40751893702991));
#18736=CARTESIAN_POINT('Ctrl Pts',(-6.96202933846692,4.19011039336715,4.41084152726329));
#18737=CARTESIAN_POINT('Ctrl Pts',(-7.00537751839709,4.11722742543054,4.41416411749668));
#18738=CARTESIAN_POINT('Ctrl Pts',(-7.04757180538556,4.04368881226468,4.41748670773006));
#18739=CARTESIAN_POINT('Ctrl Pts',(-7.15200429430959,3.86167790621401,4.42571024680401));
#18740=CARTESIAN_POINT('Ctrl Pts',(-7.24939904522159,3.67558965831389,4.43393378587795));
#18741=CARTESIAN_POINT('Ctrl Pts',(-7.33945305402924,3.48598858721609,4.4421573249519));
#18742=CARTESIAN_POINT('Ctrl Pts',(-7.42949068945407,3.29642198888592,4.45037936884362));
#18743=CARTESIAN_POINT('Ctrl Pts',(-7.5121901201584,3.10334410839429,4.45860141273533));
#18744=CARTESIAN_POINT('Ctrl Pts',(-7.58729520233631,2.9073422700302,4.46682345662705));
#18745=CARTESIAN_POINT('Ctrl Pts',(-7.66239199232013,2.71136207181669,4.47504459274021));
#18746=CARTESIAN_POINT('Ctrl Pts',(-7.72989600227281,2.5124588355455,4.48326572885336));
#18747=CARTESIAN_POINT('Ctrl Pts',(-7.7895996643185,2.31123876571616,4.49148686496651));
#18748=CARTESIAN_POINT('Ctrl Pts',(-7.84930806176531,2.11000273609957,4.49970865313979));
#18749=CARTESIAN_POINT('Ctrl Pts',(-7.90121478867765,1.90644978776118,4.50793044131307));
#18750=CARTESIAN_POINT('Ctrl Pts',(-7.94516218416331,1.70120117265459,4.51615222948634));
#18751=CARTESIAN_POINT('Ctrl Pts',(-7.98910945770717,1.49595312705577,4.52437399484644));
#18752=CARTESIAN_POINT('Ctrl Pts',(-8.02509738488821,1.28900971306024,4.53259576020654));
#18753=CARTESIAN_POINT('Ctrl Pts',(-8.05301934218722,1.08100279225286,4.54081752556664));
#18754=CARTESIAN_POINT('Ctrl Pts',(-8.0809471207503,0.872952505459324,4.54904100502818));
#18755=CARTESIAN_POINT('Ctrl Pts',(-8.10080553078993,0.663838561277428,
4.55726448448973));
#18756=CARTESIAN_POINT('Ctrl Pts',(-8.11253964888555,0.454299469248954,
4.56548796395127));
#18757=CARTESIAN_POINT('Ctrl Pts',(-8.11728066713311,0.369637916434513,
4.56881055418497));
#18758=CARTESIAN_POINT('Ctrl Pts',(-8.12069601977494,0.284907006571542,
4.57213314441867));
#18759=CARTESIAN_POINT('Ctrl Pts',(-8.12278449485915,0.200148975954921,
4.57545573465237));
#18760=CARTESIAN_POINT('Ctrl Pts',(-8.12442751148105,0.133469294594977,
4.57806963750571));
#18761=CARTESIAN_POINT('Ctrl Pts',(-8.12524944242962,0.0667693416606271,
4.58068354035906));
#18762=CARTESIAN_POINT('Ctrl Pts',(-8.12524999971641,6.78859918389947E-5,
4.5832974432124));
#18763=CARTESIAN_POINT('Ctrl Pts',(-8.12524999971641,6.78850738330637E-5,
4.58329744324837));
#18764=CARTESIAN_POINT('Ctrl Pts',(-8.12525174938836,-0.209352554230827,
4.59150423091677));
#18765=CARTESIAN_POINT('Ctrl Pts',(-8.11715274258138,-0.418809030230974,
4.59971101858517));
#18766=CARTESIAN_POINT('Ctrl Pts',(-8.1009706810933,-0.627663593469262,
4.60791780625356));
#18767=CARTESIAN_POINT('Ctrl Pts',(-8.08479158305025,-0.836479908860154,
4.6161230910007));
#18768=CARTESIAN_POINT('Ctrl Pts',(-8.06053240758662,-1.04469423516969,
4.62432837574785));
#18769=CARTESIAN_POINT('Ctrl Pts',(-8.02826285212299,-1.25167213747131,
4.63253366049499));
#18770=CARTESIAN_POINT('Ctrl Pts',(-7.99519766829729,-1.46375322409101,
4.64094125225162));
#18771=CARTESIAN_POINT('Ctrl Pts',(-7.95372205275651,-1.67453581134853,
4.64934884400826));
#18772=CARTESIAN_POINT('Ctrl Pts',(-7.90396714321867,-1.88334568293228,
4.6577564357649));
#18773=CARTESIAN_POINT('Ctrl Pts',(-7.8554106962377,-2.08712588377755,4.66596151114663));
#18774=CARTESIAN_POINT('Ctrl Pts',(-7.79896928620375,-2.2890270092906,4.67416658652835));
#18775=CARTESIAN_POINT('Ctrl Pts',(-7.73481614457164,-2.4884346027521,4.68237166191008));
#18776=CARTESIAN_POINT('Ctrl Pts',(-7.66828787637243,-2.69522481631387,
4.69088051185417));
#18777=CARTESIAN_POINT('Ctrl Pts',(-7.59346606056834,-2.89933301398041,
4.69938936179826));
#18778=CARTESIAN_POINT('Ctrl Pts',(-7.5106000776987,-3.10009258496779,4.70789821174236));
#18779=CARTESIAN_POINT('Ctrl Pts',(-7.42773409482906,-3.30085215595517,
4.71640706168646));
#18780=CARTESIAN_POINT('Ctrl Pts',(-7.33682408930247,-3.49826277449,4.72491591163056));
#18781=CARTESIAN_POINT('Ctrl Pts',(-7.23817473186267,-3.69168174596954,
4.73342476157465));
#18782=CARTESIAN_POINT('Ctrl Pts',(-7.14283319324639,-3.87861517176193,
4.74164830064859));
#18783=CARTESIAN_POINT('Ctrl Pts',(-7.04023067284676,-4.06188354415428,
4.74987183972253));
#18784=CARTESIAN_POINT('Ctrl Pts',(-6.93067430172067,-4.24092457914176,
4.75809537879648));
#18785=CARTESIAN_POINT('Ctrl Pts',(-6.82113784984571,-4.41993306135935,
4.76631742268818));
#18786=CARTESIAN_POINT('Ctrl Pts',(-6.70465022456719,-4.59471548876772,
4.77453946657988));
#18787=CARTESIAN_POINT('Ctrl Pts',(-6.58156326671015,-4.7647363545942,4.78276151047158));
#18788=CARTESIAN_POINT('Ctrl Pts',(-6.45848989862347,-4.93473844877693,
4.79098264658483));
#18789=CARTESIAN_POINT('Ctrl Pts',(-6.32881882550354,-5.09997979213808,
4.79920378269808));
#18790=CARTESIAN_POINT('Ctrl Pts',(-6.19294424840373,-5.25995523732505,
4.80742491881133));
#18791=CARTESIAN_POINT('Ctrl Pts',(-6.0570588944014,-5.41994337097673,4.81564670698462));
#18792=CARTESIAN_POINT('Ctrl Pts',(-5.9149692422097,-5.57466454540419,4.82386849515791));
#18793=CARTESIAN_POINT('Ctrl Pts',(-5.767109370974,-5.72364718214915,4.8320902833312));
#18794=CARTESIAN_POINT('Ctrl Pts',(-5.61924991000991,-5.87262940550712,
4.84031204869123));
#18795=CARTESIAN_POINT('Ctrl Pts',(-5.46562047170121,-6.01587291559778,
4.84853381405125));
#18796=CARTESIAN_POINT('Ctrl Pts',(-5.30669191477893,-6.15294307499427,
4.85675557941128));
#18797=CARTESIAN_POINT('Ctrl Pts',(-5.14773022389095,-6.29004181124344,
4.86497905887289));
#18798=CARTESIAN_POINT('Ctrl Pts',(-4.98346743074074,-6.42096443300091,
4.87320253833451));
#18799=CARTESIAN_POINT('Ctrl Pts',(-4.8144082182703,-6.5453159641343,4.88142601779612));
#18800=CARTESIAN_POINT('Ctrl Pts',(-4.74610203584738,-6.59555858768641,
4.88474860802973));
#18801=CARTESIAN_POINT('Ctrl Pts',(-4.67701322007725,-6.6447289777089,4.88807119826334));
#18802=CARTESIAN_POINT('Ctrl Pts',(-4.60717647814811,-6.69280303473057,
4.89139378849695));
#18803=CARTESIAN_POINT('Ctrl Pts',(-4.43432784630585,-6.8117881814279,4.8996173275709));
#18804=CARTESIAN_POINT('Ctrl Pts',(-4.25683930315909,-6.92409308142546,
4.90784086664485));
#18805=CARTESIAN_POINT('Ctrl Pts',(-4.07524866129991,-7.02936952443626,
4.9160644057188));
#18806=CARTESIAN_POINT('Ctrl Pts',(-3.89369103577317,-7.13462682636136,
4.92428644961053));
#18807=CARTESIAN_POINT('Ctrl Pts',(-3.70803305516046,-7.23285807398075,
4.93250849350227));
#18808=CARTESIAN_POINT('Ctrl Pts',(-3.51883909810416,-7.32375989257932,
4.940730537394));
#18809=CARTESIAN_POINT('Ctrl Pts',(-3.32966602955252,-7.41465167490036,
4.94895167350725));
#18810=CARTESIAN_POINT('Ctrl Pts',(-3.13695802971415,-7.49821551611294,
4.9571728096205));
#18811=CARTESIAN_POINT('Ctrl Pts',(-2.94130227151591,-7.57419490837642,
4.96539394573375));
#18812=CARTESIAN_POINT('Ctrl Pts',(-2.74563099486588,-7.65018032695136,
4.97361573390705));
#18813=CARTESIAN_POINT('Ctrl Pts',(-2.5470117666796,-7.71857998536448,4.98183752208036));
#18814=CARTESIAN_POINT('Ctrl Pts',(-2.34605084327077,-7.77918588306569,
4.99005931025366));
#18815=CARTESIAN_POINT('Ctrl Pts',(-2.1450904774757,-7.83979161260145,4.99828107561367));
#18816=CARTESIAN_POINT('Ctrl Pts',(-1.94178871260472,-7.89260354210846,
5.00650284097367));
#18817=CARTESIAN_POINT('Ctrl Pts',(-1.73676655799566,-7.93746366829656,
5.01472460633368));
#18818=CARTESIAN_POINT('Ctrl Pts',(-1.53170165967014,-7.98233314707642,
5.0229480857953));
#18819=CARTESIAN_POINT('Ctrl Pts',(-1.32491594324953,-8.01924744763745,
5.03117156525693));
#18820=CARTESIAN_POINT('Ctrl Pts',(-1.11704127698926,-8.04809954883774,
5.03939504471856));
#18821=CARTESIAN_POINT('Ctrl Pts',(-1.03305221382633,-8.05975686617077,
5.04271763495212));
#18822=CARTESIAN_POINT('Ctrl Pts',(-0.948885478957651,-8.0700986484556,
5.04604022518568));
#18823=CARTESIAN_POINT('Ctrl Pts',(-0.864583067614918,-8.07912022943671,
5.04936281541924));
#18824=CARTESIAN_POINT('Ctrl Pts',(-0.65593134562326,-8.10144899058145,
5.05758635449319));
#18825=CARTESIAN_POINT('Ctrl Pts',(-0.446380276048424,-8.1156940862947,
5.06580989356714));
#18826=CARTESIAN_POINT('Ctrl Pts',(-0.236568592441918,-8.12180539434245,
5.0740334326411));
#18827=CARTESIAN_POINT('Ctrl Pts',(-0.0267950562442058,-8.12791559124823,
5.08225547653279));
#18828=CARTESIAN_POINT('Ctrl Pts',(0.183238704748132,-8.12589494354887,
5.09047752042449));
#18829=CARTESIAN_POINT('Ctrl Pts',(0.392891944367202,-8.11574540523243,
5.09869956431618));
#18830=CARTESIAN_POINT('Ctrl Pts',(0.602522036615081,-8.10559698750508,
5.10692070042939));
#18831=CARTESIAN_POINT('Ctrl Pts',(0.811771396891179,-8.08732148522944,
5.11514183654259));
#18832=CARTESIAN_POINT('Ctrl Pts',(1.02000155037131,-8.06097291893107,5.12336297265579));
#18833=CARTESIAN_POINT('Ctrl Pts',(1.22824821964307,-8.03462226279402,5.13158476082908));
#18834=CARTESIAN_POINT('Ctrl Pts',(1.43547522765356,-8.00019729762124,5.13980654900237));
#18835=CARTESIAN_POINT('Ctrl Pts',(1.6410504152354,-7.95780378604271,5.14802833717566));
#18836=CARTESIAN_POINT('Ctrl Pts',(1.84662503240088,-7.91541039209488,5.15625010253567));
#18837=CARTESIAN_POINT('Ctrl Pts',(2.05054754999661,-7.86504855817847,5.16447186789569));
#18838=CARTESIAN_POINT('Ctrl Pts',(2.25219664192422,-7.80687503733762,5.1726936332557));
#18839=CARTESIAN_POINT('Ctrl Pts',(2.45388777434055,-7.74868938828324,5.18091711271733));
#18840=CARTESIAN_POINT('Ctrl Pts',(2.65330425080242,-7.68268888058018,5.18914059217896));
#18841=CARTESIAN_POINT('Ctrl Pts',(2.84983947156939,-7.60908026957168,5.19736407164059));
#18842=CARTESIAN_POINT('Ctrl Pts',(2.92924697883384,-7.5793396648568,5.20068666187423));
#18843=CARTESIAN_POINT('Ctrl Pts',(3.00818432847376,-7.54835762890888,5.20400925210788));
#18844=CARTESIAN_POINT('Ctrl Pts',(3.08661236960119,-7.51615005453756,5.20733184234153));
#18845=CARTESIAN_POINT('Ctrl Pts',(3.28072594193355,-7.43643459527703,5.21555542985409));
#18846=CARTESIAN_POINT('Ctrl Pts',(3.47178127225479,-7.34918234703222,5.22377901736665));
#18847=CARTESIAN_POINT('Ctrl Pts',(3.6591928060199,-7.25465337358528,5.23200260487921));
#18848=CARTESIAN_POINT('Ctrl Pts',(3.84656772804117,-7.16014286682761,5.24022458587443));
#18849=CARTESIAN_POINT('Ctrl Pts',(4.03030001128134,-7.05835860533478,5.24844656686964));
#18850=CARTESIAN_POINT('Ctrl Pts',(4.20982715084995,-6.9496073934048,5.25666854786486));
#18851=CARTESIAN_POINT('Ctrl Pts',(4.38934121253718,-6.84086410359429,5.26488992991947));
#18852=CARTESIAN_POINT('Ctrl Pts',(4.56465048924521,-6.72515502819134,5.2731113119741));
#18853=CARTESIAN_POINT('Ctrl Pts',(4.73521920437887,-6.60283171442234,5.28133269402872));
#18854=CARTESIAN_POINT('Ctrl Pts',(4.80657126731715,-6.55166159933984,5.28477185090658));
#18855=CARTESIAN_POINT('Ctrl Pts',(4.87709411933547,-6.4993345818291,5.28821100778445));
#18856=CARTESIAN_POINT('Ctrl Pts',(4.94675008185375,-6.44587862049697,5.29165016466231));
#18857=CARTESIAN_POINT('',(-8.12526471614247,-0.000101443950621347,4.41670255650755));
#18858=CARTESIAN_POINT('Ctrl Pts',(-8.12524999936665,-0.000101450914391436,
4.41670255678762));
#18859=CARTESIAN_POINT('Ctrl Pts',(-8.12524871677588,-0.102824730074738,
4.42072797116447));
#18860=CARTESIAN_POINT('Ctrl Pts',(-8.12329924737115,-0.205542899283528,
4.42475338554132));
#18861=CARTESIAN_POINT('Ctrl Pts',(-8.11940320204833,-0.308186964466829,
4.42877879991817));
#18862=CARTESIAN_POINT('Ctrl Pts',(-8.11144395165902,-0.517879036318932,
4.43700233899213));
#18863=CARTESIAN_POINT('Ctrl Pts',(-8.09535579262662,-0.727296668458236,
4.44522587806608));
#18864=CARTESIAN_POINT('Ctrl Pts',(-8.07118113153707,-0.935800568721758,
4.45344941714004));
#18865=CARTESIAN_POINT('Ctrl Pts',(-8.04701086582079,-1.14426655935471,
4.46167146103176));
#18866=CARTESIAN_POINT('Ctrl Pts',(-8.01475706648258,-1.35181885686601,
4.46989350492348));
#18867=CARTESIAN_POINT('Ctrl Pts',(-7.97451396314443,-1.55782367876292,
4.4781155488152));
#18868=CARTESIAN_POINT('Ctrl Pts',(-7.93427530296225,-1.76380575610296,
4.48633668492844));
#18869=CARTESIAN_POINT('Ctrl Pts',(-7.88604915634932,-1.9682404095808,4.49455782104168));
#18870=CARTESIAN_POINT('Ctrl Pts',(-7.82998094929889,-2.17050360426248,
4.50277895715491));
#18871=CARTESIAN_POINT('Ctrl Pts',(-7.7739082951942,-2.37278284146538,4.51100074532821));
#18872=CARTESIAN_POINT('Ctrl Pts',(-7.7099924140863,-2.57288999080897,4.5192225335015));
#18873=CARTESIAN_POINT('Ctrl Pts',(-7.63842902472862,-2.77021472032103,
4.5274443216748));
#18874=CARTESIAN_POINT('Ctrl Pts',(-7.56686583394015,-2.9675389023099,4.53566608703483));
#18875=CARTESIAN_POINT('Ctrl Pts',(-7.48765528043779,-3.16208040356892,
4.54388785239487));
#18876=CARTESIAN_POINT('Ctrl Pts',(-7.40104198117546,-3.35324695711164,
4.5521096177549));
#18877=CARTESIAN_POINT('Ctrl Pts',(-7.31441062447808,-3.54445336570725,
4.56033309721653));
#18878=CARTESIAN_POINT('Ctrl Pts',(-7.22037356058989,-3.73228315226096,
4.56855657667816));
#18879=CARTESIAN_POINT('Ctrl Pts',(-7.11922276604786,-3.91616582512613,
4.57678005613979));
#18880=CARTESIAN_POINT('Ctrl Pts',(-7.07835409924694,-3.99046123448811,
4.58010264637334));
#18881=CARTESIAN_POINT('Ctrl Pts',(-7.03632467150822,-4.06411256796687,
4.5834252366069));
#18882=CARTESIAN_POINT('Ctrl Pts',(-6.99315584937157,-4.13708337224428,
4.58674782684045));
#18883=CARTESIAN_POINT('Ctrl Pts',(-6.88631134834553,-4.3176889293709,4.59497136591442));
#18884=CARTESIAN_POINT('Ctrl Pts',(-6.77244926389735,-4.49418255315695,
4.60319490498838));
#18885=CARTESIAN_POINT('Ctrl Pts',(-6.6519112874456,-4.66602226596207,4.61141844406236));
#18886=CARTESIAN_POINT('Ctrl Pts',(-6.53139522689179,-4.83783073532244,
4.61964048795407));
#18887=CARTESIAN_POINT('Ctrl Pts',(-6.40420586621263,-5.00498674120909,
4.62786253184579));
#18888=CARTESIAN_POINT('Ctrl Pts',(-6.27072784462478,-5.1669778266553,4.63608457573751));
#18889=CARTESIAN_POINT('Ctrl Pts',(-6.13726456006332,-5.32895102700796,
4.64430571185073));
#18890=CARTESIAN_POINT('Ctrl Pts',(-5.99751418825371,-5.48576021786953,
4.65252684796396));
#18891=CARTESIAN_POINT('Ctrl Pts',(-5.8519017472633,-5.63692589119963,4.66074798407718));
#18892=CARTESIAN_POINT('Ctrl Pts',(-5.70627775701031,-5.78810355424738,
4.66896977225048));
#18893=CARTESIAN_POINT('Ctrl Pts',(-5.55479097127226,-5.93363659112568,
4.67719156042378));
#18894=CARTESIAN_POINT('Ctrl Pts',(-5.39790410898977,-6.0730814906974,4.68541334859708));
#18895=CARTESIAN_POINT('Ctrl Pts',(-5.24101768202619,-6.21252600334697,
4.69363511395712));
#18896=CARTESIAN_POINT('Ctrl Pts',(-5.07873143072443,-6.34588221856302,
4.70185687931717));
#18897=CARTESIAN_POINT('Ctrl Pts',(-4.91154247158541,-6.47274579388938,
4.71007864467722));
#18898=CARTESIAN_POINT('Ctrl Pts',(-4.74431865632401,-6.59963581816506,
4.71830212413885));
#18899=CARTESIAN_POINT('Ctrl Pts',(-4.57219032628825,-6.72003032011855,
4.72652560360047));
#18900=CARTESIAN_POINT('Ctrl Pts',(-4.39568587584185,-6.83356665610459,
4.7347490830621));
#18901=CARTESIAN_POINT('Ctrl Pts',(-4.32437154156672,-6.87943954030895,
4.73807167329565));
#18902=CARTESIAN_POINT('Ctrl Pts',(-4.25234315591362,-6.9241933488556,4.74139426352919));
#18903=CARTESIAN_POINT('Ctrl Pts',(-4.17963686516321,-6.96780619979263,
4.74471685376274));
#18904=CARTESIAN_POINT('Ctrl Pts',(-3.99968598922559,-7.07574968923837,
4.75294039283671));
#18905=CARTESIAN_POINT('Ctrl Pts',(-3.81552202047381,-7.17673585722949,
4.76116393191067));
#18906=CARTESIAN_POINT('Ctrl Pts',(-3.62770349366205,-7.27045080614484,
4.76938747098463));
#18907=CARTESIAN_POINT('Ctrl Pts',(-3.43991911552068,-7.36414871605475,
4.77760951487635));
#18908=CARTESIAN_POINT('Ctrl Pts',(-3.24848176928581,-7.4505779139023,4.78583155876808));
#18909=CARTESIAN_POINT('Ctrl Pts',(-3.05397370005434,-7.52947091115149,
4.79405360265981));
#18910=CARTESIAN_POINT('Ctrl Pts',(-2.8594871060484,-7.60835519799129,4.80227473877301));
#18911=CARTESIAN_POINT('Ctrl Pts',(-2.66193073911324,-7.67970483459022,
4.81049587488622));
#18912=CARTESIAN_POINT('Ctrl Pts',(-2.46190666328045,-7.74330053296366,
4.81871701099942));
#18913=CARTESIAN_POINT('Ctrl Pts',(-2.26186672252148,-7.8069012754352,4.82693879917272));
#18914=CARTESIAN_POINT('Ctrl Pts',(-2.05935896206095,-7.8627467589547,4.83516058734602));
#18915=CARTESIAN_POINT('Ctrl Pts',(-1.85500145864965,-7.91066730123999,
4.84338237551932));
#18916=CARTESIAN_POINT('Ctrl Pts',(-1.65064452227567,-7.95858771055862,
4.85160414087936));
#18917=CARTESIAN_POINT('Ctrl Pts',(-1.44443814097656,-7.99858315792208,
4.8598259062394));
#18918=CARTESIAN_POINT('Ctrl Pts',(-1.23701198916193,-8.03053478301225,
4.86804767159944));
#18919=CARTESIAN_POINT('Ctrl Pts',(-1.02954259243837,-8.06249306948579,
4.87627115106106));
#18920=CARTESIAN_POINT('Ctrl Pts',(-0.820853208724146,-8.08640413860473,
4.88449463052268));
#18921=CARTESIAN_POINT('Ctrl Pts',(-0.611581162014199,-8.10220069146459,
4.89271810998429));
#18922=CARTESIAN_POINT('Ctrl Pts',(-0.527027505401506,-8.10858308379637,
4.89604070021787));
#18923=CARTESIAN_POINT('Ctrl Pts',(-0.442378789507941,-8.11364140534786,
4.89936329045145));
#18924=CARTESIAN_POINT('Ctrl Pts',(-0.35767721917171,-8.11737362509485,
4.90268588068503));
#18925=CARTESIAN_POINT('Ctrl Pts',(-0.148037563265098,-8.12661101302548,
4.91090941975899));
#18926=CARTESIAN_POINT('Ctrl Pts',(0.0619941821116159,-8.12772431708582,
4.91913295883295));
#18927=CARTESIAN_POINT('Ctrl Pts',(0.27177739917805,-8.12070345523071,4.92735649790691));
#18928=CARTESIAN_POINT('Ctrl Pts',(0.481522474011634,-8.11368386989024,
4.93557854179862));
#18929=CARTESIAN_POINT('Ctrl Pts',(0.691018816098849,-8.09853308027499,
4.94380058569034));
#18930=CARTESIAN_POINT('Ctrl Pts',(0.899627055477995,-8.07529310449794,
4.95202262958205));
#18931=CARTESIAN_POINT('Ctrl Pts',(1.10821226286226,-8.0520556945975,4.96024376569527));
#18932=CARTESIAN_POINT('Ctrl Pts',(1.31590927029149,-8.02073091423877,4.96846490180849));
#18933=CARTESIAN_POINT('Ctrl Pts',(1.5220842305929,-7.98141260413722,4.97668603792171));
#18934=CARTESIAN_POINT('Ctrl Pts',(1.72827554367802,-7.94209117550071,4.98490782609501));
#18935=CARTESIAN_POINT('Ctrl Pts',(1.93294427820473,-7.89477500296424,4.99312961426832));
#18936=CARTESIAN_POINT('Ctrl Pts',(2.13546612589927,-7.83960917314356,5.00135140244162));
#18937=CARTESIAN_POINT('Ctrl Pts',(2.33798741164973,-7.78444349639335,5.00957316780165));
#18938=CARTESIAN_POINT('Ctrl Pts',(2.53836153862907,-7.7214282860434,5.01779493316167));
#18939=CARTESIAN_POINT('Ctrl Pts',(2.73597819902793,-7.65075884190215,5.0260166985217));
#18940=CARTESIAN_POINT('Ctrl Pts',(2.93363605921998,-7.58007466435493,5.03424017798333));
#18941=CARTESIAN_POINT('Ctrl Pts',(3.12853502661477,-7.50173316443347,5.04246365744495));
#18942=CARTESIAN_POINT('Ctrl Pts',(3.32008261774654,-7.4159786254976,5.05068713690658));
#18943=CARTESIAN_POINT('Ctrl Pts',(3.39747493793533,-7.38133061611386,5.05400972714016));
#18944=CARTESIAN_POINT('Ctrl Pts',(3.47432038990769,-7.34547300561736,5.05733231737374));
#18945=CARTESIAN_POINT('Ctrl Pts',(3.55058089322787,-7.30842410394643,5.06065490760732));
#18946=CARTESIAN_POINT('Ctrl Pts',(3.73932684629326,-7.21672748575672,5.06887837103831));
#18947=CARTESIAN_POINT('Ctrl Pts',(3.92454934907012,-7.11770029217112,5.0771018344693));
#18948=CARTESIAN_POINT('Ctrl Pts',(4.10568028118637,-7.01163868087749,5.08532529790029));
#18949=CARTESIAN_POINT('Ctrl Pts',(4.28678357617951,-6.90559325256141,5.09354750658773));
#18950=CARTESIAN_POINT('Ctrl Pts',(4.46379629155707,-6.79251569672306,5.10176971527516));
#18951=CARTESIAN_POINT('Ctrl Pts',(4.63617616371462,-6.67274742077837,5.10999192396259));
#18952=CARTESIAN_POINT('Ctrl Pts',(4.74146819312724,-6.59959128789795,5.11501416367142));
#18953=CARTESIAN_POINT('Ctrl Pts',(4.8450322541169,-6.52393976658856,5.12003640338026));
#18954=CARTESIAN_POINT('Ctrl Pts',(4.94675008185377,-6.44587862049696,5.12505864308909));
#18955=CARTESIAN_POINT('Ctrl Pts',(4.94669362673306,-6.44580471440964,3.12504817176739));
#18956=CARTESIAN_POINT('Ctrl Pts',(5.21676564029461,-6.2389782961655,3.13837430935821));
#18957=CARTESIAN_POINT('Ctrl Pts',(6.4896144375474,-5.13135356726175,3.20435678925645));
#18958=CARTESIAN_POINT('Ctrl Pts',(8.10215992848685,-2.45656664941747,3.32299561146213));
#18959=CARTESIAN_POINT('Ctrl Pts',(8.29443749013271,1.69765188778186,3.48096463838442));
#18960=CARTESIAN_POINT('Ctrl Pts',(6.4854770730954,5.44226996244785,3.63893366530671));
#18961=CARTESIAN_POINT('Ctrl Pts',(3.11173507273828,7.87380594419869,3.796902692229));
#18962=CARTESIAN_POINT('Ctrl Pts',(-1.01278989687652,8.40559170044518,3.95487171915129));
#18963=CARTESIAN_POINT('Ctrl Pts',(-4.8929542804399,6.90932077843641,4.11284074607358));
#18964=CARTESIAN_POINT('Ctrl Pts',(-7.52378000230581,3.82661413385391,4.2667843549656));
#18965=CARTESIAN_POINT('Ctrl Pts',(-8.12504676703811,1.2409840046644,4.36807162155021));
#18966=CARTESIAN_POINT('Ctrl Pts',(-8.12582592545285,-0.000101178394316476,
4.41670254582737));
#18967=CARTESIAN_POINT('Origin',(0.,0.,-16.4167025567876));
#18968=CARTESIAN_POINT('',(4.94675008185375,-6.44587862049697,1.12505977544705));
#18969=CARTESIAN_POINT('',(4.94675008185373,-6.44587862049698,1.2916563605374));
#18970=CARTESIAN_POINT('',(4.94675008185374,-6.44587862049697,-16.4167025567876));
#18971=CARTESIAN_POINT('',(-8.1252499990086,0.000126927995773117,2.58329744318944));
#18972=CARTESIAN_POINT('Ctrl Pts',(4.94675008185373,-6.44587862049698,1.2916563605374));
#18973=CARTESIAN_POINT('Ctrl Pts',(5.11324136688352,-6.31810848606874,1.29987801001623));
#18974=CARTESIAN_POINT('Ctrl Pts',(5.27479522180978,-6.18387253167384,1.30809965949505));
#18975=CARTESIAN_POINT('Ctrl Pts',(5.43091670084337,-6.04357769462763,1.31632130897387));
#18976=CARTESIAN_POINT('Ctrl Pts',(5.58876949804491,-5.90172704987481,1.32463413290993));
#18977=CARTESIAN_POINT('Ctrl Pts',(5.74106847034745,-5.75368252541814,1.33294695684599));
#18978=CARTESIAN_POINT('Ctrl Pts',(5.88733799517582,-5.59990525750742,1.34125978078205));
#18979=CARTESIAN_POINT('Ctrl Pts',(6.0320043272919,-5.44781347121373,1.34948149169392));
#18980=CARTESIAN_POINT('Ctrl Pts',(6.17077252345175,-5.29011420496733,1.3577032026058));
#18981=CARTESIAN_POINT('Ctrl Pts',(6.30322044694293,-5.12728968946953,1.36592491351767));
#18982=CARTESIAN_POINT('Ctrl Pts',(6.4378700528428,-4.9617585413419,1.37428329396582));
#18983=CARTESIAN_POINT('Ctrl Pts',(6.56598720440906,-4.79093048482667,1.38264167441398));
#18984=CARTESIAN_POINT('Ctrl Pts',(6.68717150955179,-4.61534665700626,1.39100005486213));
#18985=CARTESIAN_POINT('Ctrl Pts',(6.80835581469451,-4.43976282918586,1.39935843531028));
#18986=CARTESIAN_POINT('Ctrl Pts',(6.92260709824771,-4.25942349788531,1.40771681575842));
#18987=CARTESIAN_POINT('Ctrl Pts',(7.02957126271241,-4.07490066442704,1.41607519620657));
#18988=CARTESIAN_POINT('Ctrl Pts',(7.13480983033269,-3.89335464119984,1.42429873528053));
#18989=CARTESIAN_POINT('Ctrl Pts',(7.23302880961726,-3.70770010820867,1.43252227435448));
#18990=CARTESIAN_POINT('Ctrl Pts',(7.32392269616285,-3.5185002349198,1.44074581342844));
#18991=CARTESIAN_POINT('Ctrl Pts',(7.41480005662104,-3.32933476145429,1.44896785732015));
#18992=CARTESIAN_POINT('Ctrl Pts',(7.49835485486565,-3.13662549996389,1.45718990121187));
#18993=CARTESIAN_POINT('Ctrl Pts',(7.57432834519024,-2.94095863312419,1.46541194510358));
#18994=CARTESIAN_POINT('Ctrl Pts',(7.65029344744221,-2.74531336945002,1.47363308121679));
#18995=CARTESIAN_POINT('Ctrl Pts',(7.71867880617511,-2.54671142718753,1.48185421733));
#18996=CARTESIAN_POINT('Ctrl Pts',(7.77927416741292,-2.34575808444135,1.49007535344321));
#18997=CARTESIAN_POINT('Ctrl Pts',(7.8398743347768,-2.14478880306424,1.4982971416165));
#18998=CARTESIAN_POINT('Ctrl Pts',(7.89268318240884,-1.94146803017562,1.5065189297898));
#18999=CARTESIAN_POINT('Ctrl Pts',(7.93754029609987,-1.73641631249272,1.5147407179631));
#19000=CARTESIAN_POINT('Ctrl Pts',(7.98239728532437,-1.53136516377361,1.52296248332313));
#19001=CARTESIAN_POINT('Ctrl Pts',(8.01930252434898,-1.32458336856255,1.53118424868316));
#19002=CARTESIAN_POINT('Ctrl Pts',(8.0481465887886,-1.1167023094229,1.53940601404319));
#19003=CARTESIAN_POINT('Ctrl Pts',(8.07699666673683,-0.90877791053336,1.54762949350481));
#19004=CARTESIAN_POINT('Ctrl Pts',(8.09778217215948,-0.699754082069268,
1.55585297296643));
#19005=CARTESIAN_POINT('Ctrl Pts',(8.11044535078226,-0.49026908374332,1.56407645242805));
#19006=CARTESIAN_POINT('Ctrl Pts',(8.11556174388749,-0.405629386791053,
1.56739904266166));
#19007=CARTESIAN_POINT('Ctrl Pts',(8.11935279197638,-0.320914454967553,
1.57072163289526));
#19008=CARTESIAN_POINT('Ctrl Pts',(8.12181709581718,-0.236166518778118,
1.57404422312887));
#19009=CARTESIAN_POINT('Ctrl Pts',(8.12791634294069,-0.0264121055970575,
1.58226776220283));
#19010=CARTESIAN_POINT('Ctrl Pts',(8.12588654852,0.183612782086546,1.59049130127679));
#19011=CARTESIAN_POINT('Ctrl Pts',(8.1157272180226,0.393267447352448,1.59871484035075));
#19012=CARTESIAN_POINT('Ctrl Pts',(8.10556973466795,0.602883993758469,1.60693688424246));
#19013=CARTESIAN_POINT('Ctrl Pts',(8.0872856796049,0.81213015765241,1.61515892813417));
#19014=CARTESIAN_POINT('Ctrl Pts',(8.06092663395265,1.02036726943433,1.62338097202588));
#19015=CARTESIAN_POINT('Ctrl Pts',(8.03457049854694,1.22858139019665,1.6316021081391));
#19016=CARTESIAN_POINT('Ctrl Pts',(8.00014118950747,1.43578638878158,1.63982324425231));
#19017=CARTESIAN_POINT('Ctrl Pts',(7.95774202210878,1.64134989324762,1.64804438036553));
#19018=CARTESIAN_POINT('Ctrl Pts',(7.91533949181666,1.84692970199986,1.65626616853883));
#19019=CARTESIAN_POINT('Ctrl Pts',(7.86496589709659,2.05086746709314,1.66448795671213));
#19020=CARTESIAN_POINT('Ctrl Pts',(7.80677565064256,2.25254112127492,1.67270974488543));
#19021=CARTESIAN_POINT('Ctrl Pts',(7.74858556565089,2.45421421586626,1.68093151024546));
#19022=CARTESIAN_POINT('Ctrl Pts',(7.68257895666524,2.65362292948847,1.6891532756055));
#19023=CARTESIAN_POINT('Ctrl Pts',(7.60896023444299,2.85015994518997,1.69737504096554));
#19024=CARTESIAN_POINT('Ctrl Pts',(7.53532616393932,3.04673793559647,1.70559852042716));
#19025=CARTESIAN_POINT('Ctrl Pts',(7.45407691330428,3.24044275580677,1.71382199988878));
#19026=CARTESIAN_POINT('Ctrl Pts',(7.3654656046334,3.43068564422074,1.7220454793504));
#19027=CARTESIAN_POINT('Ctrl Pts',(7.32966335448509,3.50755081619593,1.72536806958398));
#19028=CARTESIAN_POINT('Ctrl Pts',(7.29265982215346,3.58385108037853,1.72869065981756));
#19029=CARTESIAN_POINT('Ctrl Pts',(7.25447388537293,3.65954863459173,1.73201325005114));
#19030=CARTESIAN_POINT('Ctrl Pts',(7.15996221793444,3.84690300305528,1.74023678912509));
#19031=CARTESIAN_POINT('Ctrl Pts',(7.0581733878635,4.03062455210347,1.74846032819905));
#19032=CARTESIAN_POINT('Ctrl Pts',(6.94941202981653,4.21014964132408,1.75668386727301));
#19033=CARTESIAN_POINT('Ctrl Pts',(6.84067044647371,4.389642089765,1.76490591116471));
#19034=CARTESIAN_POINT('Ctrl Pts',(6.72495901813897,4.56493934908913,1.77312795505642));
#19035=CARTESIAN_POINT('Ctrl Pts',(6.60262720753773,4.73550435759302,1.78134999894813));
#19036=CARTESIAN_POINT('Ctrl Pts',(6.48030890333319,4.90605053437477,1.78957113506134));
#19037=CARTESIAN_POINT('Ctrl Pts',(6.35137184798668,5.07186526387154,1.79779227117456));
#19038=CARTESIAN_POINT('Ctrl Pts',(6.21620799866067,5.23244165566011,1.80601340728777));
#19039=CARTESIAN_POINT('Ctrl Pts',(6.08103342880286,5.39303078357836,1.81423519546107));
#19040=CARTESIAN_POINT('Ctrl Pts',(5.93963126605871,5.5483805162706,1.82245698363437));
#19041=CARTESIAN_POINT('Ctrl Pts',(5.79243349414781,5.69801735504329,1.83067877180767));
#19042=CARTESIAN_POINT('Ctrl Pts',(5.64523613067152,5.84765377861362,1.8389005371677));
#19043=CARTESIAN_POINT('Ctrl Pts',(5.49224339894691,5.99157713160955,1.84712230252773));
#19044=CARTESIAN_POINT('Ctrl Pts',(5.33392422572816,6.12935069291114,1.85534406788776));
#19045=CARTESIAN_POINT('Ctrl Pts',(5.17557204558999,6.26715297771313,1.86356754734938));
#19046=CARTESIAN_POINT('Ctrl Pts',(5.01189142807282,6.39880271584666,1.87179102681099));
#19047=CARTESIAN_POINT('Ctrl Pts',(4.84338529968251,6.52390269710696,1.88001450627261));
#19048=CARTESIAN_POINT('Ctrl Pts',(4.77530258370977,6.57444772222682,1.88333709650622));
#19049=CARTESIAN_POINT('Ctrl Pts',(4.706432487394,6.62392399485261,1.88665968673983));
#19050=CARTESIAN_POINT('Ctrl Pts',(4.63680961071596,6.67230726184519,1.88998227697344));
#19051=CARTESIAN_POINT('Ctrl Pts',(4.46449030362483,6.79205771515557,1.8982058160474));
#19052=CARTESIAN_POINT('Ctrl Pts',(4.28750150809802,6.90514856257424,1.90642935512136));
#19053=CARTESIAN_POINT('Ctrl Pts',(4.10637948734327,7.01122921237257,1.91465289419532));
#19054=CARTESIAN_POINT('Ctrl Pts',(3.92529039771805,7.1172905748661,1.92287493808703));
#19055=CARTESIAN_POINT('Ctrl Pts',(3.74006983712862,7.21634413466484,1.93109698197874));
#19056=CARTESIAN_POINT('Ctrl Pts',(3.55128083338975,7.30808401736724,1.93931902587045));
#19057=CARTESIAN_POINT('Ctrl Pts',(3.36251267344561,7.39981377126318,1.94754016198368));
#19058=CARTESIAN_POINT('Ctrl Pts',(3.17017712209659,7.48423133132588,1.95576129809691));
#19059=CARTESIAN_POINT('Ctrl Pts',(2.97486020904337,7.56107758848899,1.96398243421014));
#19060=CARTESIAN_POINT('Ctrl Pts',(2.77952780441349,7.63792994071915,1.97220422238344));
#19061=CARTESIAN_POINT('Ctrl Pts',(2.58121383909049,7.70720967970647,1.98042601055674));
#19062=CARTESIAN_POINT('Ctrl Pts',(2.380523641074,7.7687061185752,1.98864779873004));
#19063=CARTESIAN_POINT('Ctrl Pts',(2.17983399991929,7.83020238680771,1.99686956409007));
#19064=CARTESIAN_POINT('Ctrl Pts',(1.97676842204044,7.88391531429189,2.00509132945011));
#19065=CARTESIAN_POINT('Ctrl Pts',(1.77194721002299,7.92968414549985,2.01331309481014));
#19066=CARTESIAN_POINT('Ctrl Pts',(1.56708329618284,7.97546251874937,2.02153657427177));
#19067=CARTESIAN_POINT('Ctrl Pts',(1.36046330488571,8.01329342275546,2.02976005373339));
#19068=CARTESIAN_POINT('Ctrl Pts',(1.1527186236022,8.0430670354847,2.03798353319502));
#19069=CARTESIAN_POINT('Ctrl Pts',(1.06878207918339,8.05509667760076,2.04130612342859));
#19070=CARTESIAN_POINT('Ctrl Pts',(0.98466203122376,8.06581158546664,2.04462871366216));
#19071=CARTESIAN_POINT('Ctrl Pts',(0.900400453850177,8.07520690664991,2.04795130389573));
#19072=CARTESIAN_POINT('Ctrl Pts',(0.691849797508385,8.09846068922064,2.05617484296969));
#19073=CARTESIAN_POINT('Ctrl Pts',(0.482363956383825,8.11363487388641,2.06439838204366));
#19074=CARTESIAN_POINT('Ctrl Pts',(0.272581435487024,8.12067650651889,2.07262192111762));
#19075=CARTESIAN_POINT('Ctrl Pts',(0.0628370566964013,8.12771685886025,
2.08084396500934));
#19076=CARTESIAN_POINT('Ctrl Pts',(-0.147203599582602,8.1266276004737,2.08906600890105));
#19077=CARTESIAN_POINT('Ctrl Pts',(-0.356899784817117,8.11740784401631,
2.09728805279277));
#19078=CARTESIAN_POINT('Ctrl Pts',(-0.566572817939022,8.10818910549274,
2.105509188906));
#19079=CARTESIAN_POINT('Ctrl Pts',(-0.775901161411214,8.09084167401546,
2.11373032501923));
#19080=CARTESIAN_POINT('Ctrl Pts',(-0.984246107139381,8.06541673833913,
2.12195146113246));
#19081=CARTESIAN_POINT('Ctrl Pts',(-1.19260757776358,8.03998978608198,2.13017324930576));
#19082=CARTESIAN_POINT('Ctrl Pts',(-1.39998520170378,8.00648408260978,2.13839503747905));
#19083=CARTESIAN_POINT('Ctrl Pts',(-1.60574635701631,7.96500258627886,2.14661682565235));
#19084=CARTESIAN_POINT('Ctrl Pts',(-1.8115069413964,7.92352120504804,2.15483859101237));
#19085=CARTESIAN_POINT('Ctrl Pts',(-2.01565077753847,7.87406413615681,2.1630603563724));
#19086=CARTESIAN_POINT('Ctrl Pts',(-2.21755585035044,7.81678537591231,2.17128212173242));
#19087=CARTESIAN_POINT('Ctrl Pts',(-2.41950301701857,7.75949467399709,2.17950560119405));
#19088=CARTESIAN_POINT('Ctrl Pts',(-2.61921020414699,7.69437910358001,2.18772908065567));
#19089=CARTESIAN_POINT('Ctrl Pts',(-2.81606990112761,7.62164272807793,2.1959525601173));
#19090=CARTESIAN_POINT('Ctrl Pts',(-2.8956085087966,7.59225453880882,2.19927515035087));
#19091=CARTESIAN_POINT('Ctrl Pts',(-2.97468246844109,7.56162284565495,2.20259774058444));
#19092=CARTESIAN_POINT('Ctrl Pts',(-3.05325255908329,7.52976336765979,2.20592033081802));
#19093=CARTESIAN_POINT('Ctrl Pts',(-3.24771656608354,7.4509099299046,2.21414386989198));
#19094=CARTESIAN_POINT('Ctrl Pts',(-3.43915581777879,7.36450630485182,2.22236740896594));
#19095=CARTESIAN_POINT('Ctrl Pts',(-3.62698362246535,7.27080995246527,2.2305909480399));
#19096=CARTESIAN_POINT('Ctrl Pts',(-3.8147772767944,7.17713063570312,2.23881299193161));
#19097=CARTESIAN_POINT('Ctrl Pts',(-3.99896053087167,7.07616136962983,2.24703503582332));
#19098=CARTESIAN_POINT('Ctrl Pts',(-4.17896951186102,6.96820646805446,2.25525707971503));
#19099=CARTESIAN_POINT('Ctrl Pts',(-4.35895861843857,6.86026348555201,2.26347821582822));
#19100=CARTESIAN_POINT('Ctrl Pts',(-4.53477411920625,6.74533655898958,2.27169935194142));
#19101=CARTESIAN_POINT('Ctrl Pts',(-4.70587873178468,6.62377482439104,2.27992048805461));
#19102=CARTESIAN_POINT('Ctrl Pts',(-4.87699691553992,6.50220344811325,2.28814227622791));
#19103=CARTESIAN_POINT('Ctrl Pts',(-5.04340322255487,6.37399638098395,2.29636406440121));
#19104=CARTESIAN_POINT('Ctrl Pts',(-5.2045903726162,6.23954538534425,2.30458585257451));
#19105=CARTESIAN_POINT('Ctrl Pts',(-5.3657770754266,6.10509476276985,2.31280761793456));
#19106=CARTESIAN_POINT('Ctrl Pts',(-5.52174442549491,5.96440043732968,2.32102938329461));
#19107=CARTESIAN_POINT('Ctrl Pts',(-5.67201877173187,5.81789400175194,2.32925114865466));
#19108=CARTESIAN_POINT('Ctrl Pts',(-5.82232444767511,5.67135702201474,2.33747462811628));
#19109=CARTESIAN_POINT('Ctrl Pts',(-5.96693453749004,5.51900571737564,2.34569810757791));
#19110=CARTESIAN_POINT('Ctrl Pts',(-6.10541198437529,5.36130880136059,2.35392158703954));
#19111=CARTESIAN_POINT('Ctrl Pts',(-6.16136200100031,5.29759340747361,2.35724417727313));
#19112=CARTESIAN_POINT('Ctrl Pts',(-6.21631132585167,5.23300576610325,2.36056676750671));
#19113=CARTESIAN_POINT('Ctrl Pts',(-6.2702329541306,5.1675783751613,2.36388935774031));
#19114=CARTESIAN_POINT('Ctrl Pts',(-6.40369106539566,5.00564305720415,2.37211289681426));
#19115=CARTESIAN_POINT('Ctrl Pts',(-6.53089427821922,4.83850863178803,2.38033643588821));
#19116=CARTESIAN_POINT('Ctrl Pts',(-6.65144926807356,4.66668085439145,2.38855997496216));
#19117=CARTESIAN_POINT('Ctrl Pts',(-6.77198233893676,4.49488431826937,2.39678201885387));
#19118=CARTESIAN_POINT('Ctrl Pts',(-6.88586943007247,4.31839637464006,2.40500406274559));
#19119=CARTESIAN_POINT('Ctrl Pts',(-6.9927595925948,4.1377531152394,2.4132261066373));
#19120=CARTESIAN_POINT('Ctrl Pts',(-7.09963795360082,3.95712980027819,2.42144724275056));
#19121=CARTESIAN_POINT('Ctrl Pts',(-7.19952077815735,3.77235233921032,2.42966837886383));
#19122=CARTESIAN_POINT('Ctrl Pts',(-7.29210184224885,3.58398357763689,2.4378895149771));
#19123=CARTESIAN_POINT('Ctrl Pts',(-7.38469024941451,3.39559987558077,2.44611130315041));
#19124=CARTESIAN_POINT('Ctrl Pts',(-7.4699756064655,3.20362456740546,2.4543330913237));
#19125=CARTESIAN_POINT('Ctrl Pts',(-7.5476983688039,3.0086436970926,2.46255487949701));
#19126=CARTESIAN_POINT('Ctrl Pts',(-7.62542091548221,2.81366336780001,2.47077664485702));
#19127=CARTESIAN_POINT('Ctrl Pts',(-7.6955808027202,2.61567776801857,2.47899841021705));
#19128=CARTESIAN_POINT('Ctrl Pts',(-7.75796702345944,2.4152919544883,2.48722017557707));
#19129=CARTESIAN_POINT('Ctrl Pts',(-7.82036625069022,2.2148643638419,2.4954436550387));
#19130=CARTESIAN_POINT('Ctrl Pts',(-7.87498848608079,2.01203584143313,2.50366713450033));
#19131=CARTESIAN_POINT('Ctrl Pts',(-7.92167257738839,1.80742666217823,2.51189061396197));
#19132=CARTESIAN_POINT('Ctrl Pts',(-7.94053467907712,1.7247569766932,2.51521320419551));
#19133=CARTESIAN_POINT('Ctrl Pts',(-7.95810148685798,1.64179675138254,2.51853579442906));
#19134=CARTESIAN_POINT('Ctrl Pts',(-7.97436472768614,1.55858742210219,2.5218583846626));
#19135=CARTESIAN_POINT('Ctrl Pts',(-8.01566387109975,1.34728427166554,2.53029582539226));
#19136=CARTESIAN_POINT('Ctrl Pts',(-8.04856370238538,1.13432059785419,2.53873326612193));
#19137=CARTESIAN_POINT('Ctrl Pts',(-8.07295618582614,0.920361876780752,
2.54717070685159));
#19138=CARTESIAN_POINT('Ctrl Pts',(-8.09734200868676,0.706461579000405,
2.55560584366454));
#19139=CARTESIAN_POINT('Ctrl Pts',(-8.11322509376166,0.491567035436145,
2.5640409804775));
#19140=CARTESIAN_POINT('Ctrl Pts',(-8.12054913382223,0.276350009370382,
2.57247611729046));
#19141=CARTESIAN_POINT('Ctrl Pts',(-8.12368110532627,0.184316980161344,
2.57608322592345));
#19142=CARTESIAN_POINT('Ctrl Pts',(-8.12524856030468,0.092225042011402,
2.57969033455644));
#19143=CARTESIAN_POINT('Ctrl Pts',(-8.1252499990086,0.000126927995783942,
2.58329744318944));
#19144=CARTESIAN_POINT('Ctrl Pts',(-8.12524999900861,0.000126927409469058,
2.5832974432124));
#19145=CARTESIAN_POINT('Ctrl Pts',(-8.12525328844262,-0.210445980594937,
2.59154472777903));
#19146=CARTESIAN_POINT('Ctrl Pts',(-8.11706646380963,-0.421019864585635,
2.59979201234565));
#19147=CARTESIAN_POINT('Ctrl Pts',(-8.1007153570126,-0.630950288976996,
2.60803929691228));
#19148=CARTESIAN_POINT('Ctrl Pts',(-8.08436443564097,-0.840878332708048,
2.61628648795277));
#19149=CARTESIAN_POINT('Ctrl Pts',(-8.05984944240335,-1.05016264135977,
2.62453367899326));
#19150=CARTESIAN_POINT('Ctrl Pts',(-8.02724816546579,-1.2581631263577,2.63278087003375));
#19151=CARTESIAN_POINT('Ctrl Pts',(-7.99463828803845,-1.46621848362481,
2.64103023675228));
#19152=CARTESIAN_POINT('Ctrl Pts',(-7.95393790784404,-1.67298905246805,
2.6492796034708));
#19153=CARTESIAN_POINT('Ctrl Pts',(-7.90527631458381,-1.87784289880177,
2.65752897018933));
#19154=CARTESIAN_POINT('Ctrl Pts',(-7.86143142634161,-2.06241955149075,
2.66496178398785));
#19155=CARTESIAN_POINT('Ctrl Pts',(-7.81112407879475,-2.24544011732185,
2.67239459778637));
#19156=CARTESIAN_POINT('Ctrl Pts',(-7.75448398467238,-2.42645125522018,
2.67982741158489));
#19157=CARTESIAN_POINT('Ctrl Pts',(-7.69181834554913,-2.62671890697087,
2.68805095065885));
#19158=CARTESIAN_POINT('Ctrl Pts',(-7.62138020049275,-2.82459018137162,
2.69627448973282));
#19159=CARTESIAN_POINT('Ctrl Pts',(-7.54337810570844,-3.0194592755688,2.70449802880679));
#19160=CARTESIAN_POINT('Ctrl Pts',(-7.46539019305993,-3.21429293917961,
2.7127200726985));
#19161=CARTESIAN_POINT('Ctrl Pts',(-7.37984118508777,-3.40612523836004,
2.72094211659021));
#19162=CARTESIAN_POINT('Ctrl Pts',(-7.28698820295463,-3.59436927603441,
2.72916416048192));
#19163=CARTESIAN_POINT('Ctrl Pts',(-7.19414547252293,-3.78259253008256,
2.73738529659515));
#19164=CARTESIAN_POINT('Ctrl Pts',(-7.09400050833028,-3.96722804916409,
2.74560643270837));
#19165=CARTESIAN_POINT('Ctrl Pts',(-6.98685728051198,-4.14771176725876,
2.7538275688216));
#19166=CARTESIAN_POINT('Ctrl Pts',(-6.87970555461987,-4.32820980043416,
2.7620493569949));
#19167=CARTESIAN_POINT('Ctrl Pts',(-6.7655546043071,-4.50455511967747,2.77027114516821));
#19168=CARTESIAN_POINT('Ctrl Pts',(-6.64475333951376,-4.67621007008033,
2.77849293334152));
#19169=CARTESIAN_POINT('Ctrl Pts',(-6.52395240991147,-4.84786454418683,
2.78671469870157));
#19170=CARTESIAN_POINT('Ctrl Pts',(-6.3965013746841,-5.01482843584574,2.79493646406162));
#19171=CARTESIAN_POINT('Ctrl Pts',(-6.26279159401588,-5.1765943449747,2.80315822942167));
#19172=CARTESIAN_POINT('Ctrl Pts',(-6.12905393707836,-5.33839397960992,
2.8113817088833));
#19173=CARTESIAN_POINT('Ctrl Pts',(-5.98905511593022,-5.49499323943775,
2.81960518834492));
#19174=CARTESIAN_POINT('Ctrl Pts',(-5.84322648330132,-5.64591815627415,
2.82782866780654));
#19175=CARTESIAN_POINT('Ctrl Pts',(-5.78430631540832,-5.70689741171206,
2.83115125804009));
#19176=CARTESIAN_POINT('Ctrl Pts',(-5.72443489078691,-5.76695075660639,
2.83447384827363));
#19177=CARTESIAN_POINT('Ctrl Pts',(-5.66364238702835,-5.82604861585928,
2.83779643850717));
#19178=CARTESIAN_POINT('Ctrl Pts',(-5.51317859374565,-5.97231809858025,
2.84601997758114));
#19179=CARTESIAN_POINT('Ctrl Pts',(-5.35702099047824,-6.11277939735596,
2.85424351665511));
#19180=CARTESIAN_POINT('Ctrl Pts',(-5.19564142839055,-6.24699909637354,
2.86246705572907));
#19181=CARTESIAN_POINT('Ctrl Pts',(-5.03429120791019,-6.38119439191862,
2.8706890996208));
#19182=CARTESIAN_POINT('Ctrl Pts',(-4.86772115023346,-6.50915016419816,
2.87891114351254));
#19183=CARTESIAN_POINT('Ctrl Pts',(-4.69643681069821,-6.63047274676692,
2.88713318740427));
#19184=CARTESIAN_POINT('Ctrl Pts',(-4.52517138230544,-6.75178193436535,
2.89535432351748));
#19185=CARTESIAN_POINT('Ctrl Pts',(-4.34919295178381,-6.86645922396823,
2.90357545963069));
#19186=CARTESIAN_POINT('Ctrl Pts',(-4.16903740064043,-6.97415333316965,
2.91179659574391));
#19187=CARTESIAN_POINT('Ctrl Pts',(-3.98886756044491,-7.08185598413805,
2.9200183839172));
#19188=CARTESIAN_POINT('Ctrl Pts',(-3.80452018944167,-7.18257419440997,
2.92824017209049));
#19189=CARTESIAN_POINT('Ctrl Pts',(-3.61655811180281,-7.27600130473142,
2.93646196026378));
#19190=CARTESIAN_POINT('Ctrl Pts',(-3.42859655570825,-7.36942815581772,
2.94468372562382));
#19191=CARTESIAN_POINT('Ctrl Pts',(-3.23702057834738,-7.45556381856249,
2.95290549098386));
#19192=CARTESIAN_POINT('Ctrl Pts',(-3.0424159271361,-7.53414845147138,2.9611272563439));
#19193=CARTESIAN_POINT('Ctrl Pts',(-2.84777070408543,-7.61274946797175,
2.96935073580553));
#19194=CARTESIAN_POINT('Ctrl Pts',(-2.65009581929774,-7.68379619925315,
2.97757421526716));
#19195=CARTESIAN_POINT('Ctrl Pts',(-2.44999626945303,-7.74707724514002,
2.9857976947288));
#19196=CARTESIAN_POINT('Ctrl Pts',(-2.36914864124961,-7.77264513109556,
2.98912028496235));
#19197=CARTESIAN_POINT('Ctrl Pts',(-2.28790538816167,-7.79694586250298,
2.99244287519591));
#19198=CARTESIAN_POINT('Ctrl Pts',(-2.20630712949662,-7.8199678012657,2.99576546542946));
#19199=CARTESIAN_POINT('Ctrl Pts',(-2.00434828975688,-7.87694798830823,
3.00398900450342));
#19200=CARTESIAN_POINT('Ctrl Pts',(-1.80014810831906,-7.92610955269224,
3.01221254357739));
#19201=CARTESIAN_POINT('Ctrl Pts',(-1.59432788555514,-7.96729603791909,
3.02043608265135));
#19202=CARTESIAN_POINT('Ctrl Pts',(-1.388545084483,-8.00847503472748,3.02865812654305));
#19203=CARTESIAN_POINT('Ctrl Pts',(-1.18114311903416,-8.04168178858559,
3.03688017043476));
#19204=CARTESIAN_POINT('Ctrl Pts',(-0.972754001005447,-8.06681084543501,
3.04510221432647));
#19205=CARTESIAN_POINT('Ctrl Pts',(-0.764387890778811,-8.09193712783837,
3.05332335043969));
#19206=CARTESIAN_POINT('Ctrl Pts',(-0.555035138265151,-8.10898745846579,
3.06154448655291));
#19207=CARTESIAN_POINT('Ctrl Pts',(-0.345334241689457,-8.11790809408537,
3.06976562266613));
#19208=CARTESIAN_POINT('Ctrl Pts',(-0.135616712669919,-8.1268294372459,
3.07798741083943));
#19209=CARTESIAN_POINT('Ctrl Pts',(0.0744487210210313,-8.12761978183108,
3.08620919901274));
#19210=CARTESIAN_POINT('Ctrl Pts',(0.284221116216748,-8.12027745336306,
3.09443098718604));
#19211=CARTESIAN_POINT('Ctrl Pts',(0.493992929349538,-8.11293514526807,
3.10265275254606));
#19212=CARTESIAN_POINT('Ctrl Pts',(0.703471410956348,-8.09746022227151,
3.11087451790608));
#19213=CARTESIAN_POINT('Ctrl Pts',(0.91201775242604,-8.07390309464758,3.1190962832661));
#19214=CARTESIAN_POINT('Ctrl Pts',(1.12060757234675,-8.05034105575351,3.12731976272774));
#19215=CARTESIAN_POINT('Ctrl Pts',(1.32826457078167,-8.01869347918493,3.13554324218938));
#19216=CARTESIAN_POINT('Ctrl Pts',(1.53435607749764,-7.9790625382902,3.14376672165102));
#19217=CARTESIAN_POINT('Ctrl Pts',(1.61762467817113,-7.96305017055966,3.1470893118846));
#19218=CARTESIAN_POINT('Ctrl Pts',(1.700637817607,-7.9457351366193,3.15041190211817));
#19219=CARTESIAN_POINT('Ctrl Pts',(1.78335423519316,-7.92712654335218,3.15373449235175));
#19220=CARTESIAN_POINT('Ctrl Pts',(1.98807904402292,-7.88106989812531,3.16195797047423));
#19221=CARTESIAN_POINT('Ctrl Pts',(2.1910519731871,-7.82707074522186,3.1701814485967));
#19222=CARTESIAN_POINT('Ctrl Pts',(2.39165219092882,-7.76528733274728,3.17840492671917));
#19223=CARTESIAN_POINT('Ctrl Pts',(2.59221537026594,-7.70351532783274,3.18662688647585));
#19224=CARTESIAN_POINT('Ctrl Pts',(2.79040643087923,-7.63396201884482,3.19484884623252));
#19225=CARTESIAN_POINT('Ctrl Pts',(2.98561941136611,-7.55683560049932,3.2030708059892));
#19226=CARTESIAN_POINT('Ctrl Pts',(3.18082858102689,-7.47971068776767,3.2112926052419));
#19227=CARTESIAN_POINT('Ctrl Pts',(3.3730595111537,-7.39501306610892,3.2195144044946));
#19228=CARTESIAN_POINT('Ctrl Pts',(3.56172499869025,-7.30299956156407,3.22773620374729));
#19229=CARTESIAN_POINT('Ctrl Pts',(3.75037759399235,-7.21099234465395,3.235957441173));
#19230=CARTESIAN_POINT('Ctrl Pts',(3.93546496886292,-7.11167037386672,3.24417867859872));
#19231=CARTESIAN_POINT('Ctrl Pts',(4.11642281865087,-7.0053373038413,3.25239991602442));
#19232=CARTESIAN_POINT('Ctrl Pts',(4.29740606490845,-6.89898931053629,3.26062230725698));
#19233=CARTESIAN_POINT('Ctrl Pts',(4.47425837329976,-6.7856284006226,3.26884469848954));
#19234=CARTESIAN_POINT('Ctrl Pts',(4.64644188055243,-6.6656031544901,3.27706708972209));
#19235=CARTESIAN_POINT('Ctrl Pts',(4.74821045284433,-6.59466257410128,3.28192691067657));
#19236=CARTESIAN_POINT('Ctrl Pts',(4.84834856604575,-6.52139473475173,3.28678673163106));
#19237=CARTESIAN_POINT('Ctrl Pts',(4.94675008185374,-6.44587862049698,3.29164655258555));
#19238=CARTESIAN_POINT('',(-8.12524999744415,0.000203798425227694,2.41670255624515));
#19239=CARTESIAN_POINT('Ctrl Pts',(-8.125117379974,0.000203781251170848,
2.41670255678762));
#19240=CARTESIAN_POINT('Ctrl Pts',(-8.12415321314374,-0.990648431134313,
2.45551853014197));
#19241=CARTESIAN_POINT('Ctrl Pts',(-7.69622348325201,-3.32646489320684,
2.54699084580375));
#19242=CARTESIAN_POINT('Ctrl Pts',(-5.51026191012776,-6.42780902731277,
2.69111950377297));
#19243=CARTESIAN_POINT('Ctrl Pts',(-1.78490025904692,-8.27610091015463,
2.84908853069526));
#19244=CARTESIAN_POINT('Ctrl Pts',(2.02051483585045,-8.14010815660882,2.99373142002673));
#19245=CARTESIAN_POINT('Ctrl Pts',(4.14961438984119,-7.05622354844238,3.08571796705077));
#19246=CARTESIAN_POINT('Ctrl Pts',(4.94669362673306,-6.44580471440964,3.12504817176739));
#19247=CARTESIAN_POINT('Ctrl Pts',(4.94675008185375,-6.44587862049697,1.12505977544705));
#19248=CARTESIAN_POINT('Ctrl Pts',(5.11323077301675,-6.31811661610258,1.13328241581699));
#19249=CARTESIAN_POINT('Ctrl Pts',(5.27478151473168,-6.18388435476994,1.14150505618694));
#19250=CARTESIAN_POINT('Ctrl Pts',(5.43090611222471,-6.04358720982003,1.14972769655688));
#19251=CARTESIAN_POINT('Ctrl Pts',(5.58700848365971,-5.90331003771576,1.1579491663433));
#19252=CARTESIAN_POINT('Ctrl Pts',(5.73768603355537,-5.75696990251955,1.16617063612971));
#19253=CARTESIAN_POINT('Ctrl Pts',(5.88247713338117,-5.60501118087624,1.17439210591613));
#19254=CARTESIAN_POINT('Ctrl Pts',(6.02727738266826,-5.45304285684409,1.18261409522356));
#19255=CARTESIAN_POINT('Ctrl Pts',(6.16619023247752,-5.29545544791427,1.190836084531));
#19256=CARTESIAN_POINT('Ctrl Pts',(6.2987915383268,-5.13272955835418,1.19905807383843));
#19257=CARTESIAN_POINT('Ctrl Pts',(6.43138822169437,-4.97000934141884,1.20727977652731));
#19258=CARTESIAN_POINT('Ctrl Pts',(6.55767361594782,-4.8021512317033,1.21550147921619));
#19259=CARTESIAN_POINT('Ctrl Pts',(6.67726411910909,-4.6296686108358,1.22372318190506));
#19260=CARTESIAN_POINT('Ctrl Pts',(6.79688321455685,-4.45714475197381,1.23194685027911));
#19261=CARTESIAN_POINT('Ctrl Pts',(6.90980405111591,-4.27999441430689,1.24017051865315));
#19262=CARTESIAN_POINT('Ctrl Pts',(7.01568590929727,-4.09876064007009,1.24839418702719));
#19263=CARTESIAN_POINT('Ctrl Pts',(7.10583020705181,-3.94446422339785,1.25539554517558));
#19264=CARTESIAN_POINT('Ctrl Pts',(7.19087314623396,-3.78720860347607,1.26239690332397));
#19265=CARTESIAN_POINT('Ctrl Pts',(7.2706303882144,-3.6273435625087,1.26939826147236));
#19266=CARTESIAN_POINT('Ctrl Pts',(7.36431032601451,-3.43957193547693,1.27762180054632));
#19267=CARTESIAN_POINT('Ctrl Pts',(7.45072749512893,-3.24813879729511,1.28584533962027));
#19268=CARTESIAN_POINT('Ctrl Pts',(7.52961220588782,-3.05362531942691,1.29406887869423));
#19269=CARTESIAN_POINT('Ctrl Pts',(7.60848257403608,-2.85914720748768,1.30229092258595));
#19270=CARTESIAN_POINT('Ctrl Pts',(7.67982310647036,-2.66159014685487,1.31051296647766));
#19271=CARTESIAN_POINT('Ctrl Pts',(7.74341221979638,-2.4615553531879,1.31873501036937));
#19272=CARTESIAN_POINT('Ctrl Pts',(7.80699431238271,-2.26154264494003,1.32695614648258));
#19273=CARTESIAN_POINT('Ctrl Pts',(7.86282660515338,-2.05905303077812,1.33517728259579));
#19274=CARTESIAN_POINT('Ctrl Pts',(7.91073710563994,-1.85470375207241,1.343398418709));
#19275=CARTESIAN_POINT('Ctrl Pts',(7.95865140615179,-1.65033826538681,1.3516202068823));
#19276=CARTESIAN_POINT('Ctrl Pts',(7.99864258903827,-1.44411310599154,1.3598419950556));
#19277=CARTESIAN_POINT('Ctrl Pts',(8.03058935885154,-1.23665763734365,1.3680637832289));
#19278=CARTESIAN_POINT('Ctrl Pts',(8.06253604002105,-1.02920274432932,1.37628554858893));
#19279=CARTESIAN_POINT('Ctrl Pts',(8.08643831054409,-0.820517840797621,
1.38450731394896));
#19280=CARTESIAN_POINT('Ctrl Pts',(8.10222644260455,-0.611239916284599,
1.392729079309));
#19281=CARTESIAN_POINT('Ctrl Pts',(8.11801786622845,-0.401918360798402,
1.40095255877062));
#19282=CARTESIAN_POINT('Ctrl Pts',(8.12569174974096,-0.19200383149342,1.40917603823225));
#19283=CARTESIAN_POINT('Ctrl Pts',(8.12523036436275,0.0178630495050401,
1.41739951769387));
#19284=CARTESIAN_POINT('Ctrl Pts',(8.12504394758397,0.102657041198461,1.42072210792747));
#19285=CARTESIAN_POINT('Ctrl Pts',(8.12353007496566,0.187443242370045,1.42404469816106));
#19286=CARTESIAN_POINT('Ctrl Pts',(8.12068999082584,0.272179417666121,1.42736728839465));
#19287=CARTESIAN_POINT('Ctrl Pts',(8.1136606729578,0.481904722183047,1.43559082746861));
#19288=CARTESIAN_POINT('Ctrl Pts',(8.09850130939948,0.691391636352905,1.44381436654256));
#19289=CARTESIAN_POINT('Ctrl Pts',(8.07525147145568,0.900000686251279,1.45203790561652));
#19290=CARTESIAN_POINT('Ctrl Pts',(8.05200586073628,1.10857180740081,1.46025994950824));
#19291=CARTESIAN_POINT('Ctrl Pts',(8.0206727442093,1.31626508986942,1.46848199339995));
#19292=CARTESIAN_POINT('Ctrl Pts',(7.98134354013807,1.52244633954577,1.47670403729166));
#19293=CARTESIAN_POINT('Ctrl Pts',(7.94201867832116,1.72860482518594,1.48492517340488));
#19294=CARTESIAN_POINT('Ctrl Pts',(7.89469954674085,1.93325132172575,1.4931463095181));
#19295=CARTESIAN_POINT('Ctrl Pts',(7.83952880275268,2.13576115549259,1.50136744563132));
#19296=CARTESIAN_POINT('Ctrl Pts',(7.78435368289246,2.33828705134343,1.50958923380462));
#19297=CARTESIAN_POINT('Ctrl Pts',(7.72132578128062,2.53867566053733,1.51781102197792));
#19298=CARTESIAN_POINT('Ctrl Pts',(7.65063810830258,2.73631578921154,1.52603281015121));
#19299=CARTESIAN_POINT('Ctrl Pts',(7.57995063146392,2.93395536948725,1.53425457551125));
#19300=CARTESIAN_POINT('Ctrl Pts',(7.50160352763663,3.12884620770216,1.54247634087128));
#19301=CARTESIAN_POINT('Ctrl Pts',(7.41583878503286,3.32039495796847,1.55069810623131));
#19302=CARTESIAN_POINT('Ctrl Pts',(7.33005616190401,3.51198364296934,1.55892158569294));
#19303=CARTESIAN_POINT('Ctrl Pts',(7.23685293117237,3.7002285788446,1.56714506515456));
#19304=CARTESIAN_POINT('Ctrl Pts',(7.13651853672765,3.88455798482178,1.57536854461619));
#19305=CARTESIAN_POINT('Ctrl Pts',(7.09597972579851,3.95903389090508,1.57869113484977));
#19306=CARTESIAN_POINT('Ctrl Pts',(7.05427730926703,4.03287087469238,1.58201372508336));
#19307=CARTESIAN_POINT('Ctrl Pts',(7.01143249181514,4.10603238847661,1.58533631531694));
#19308=CARTESIAN_POINT('Ctrl Pts',(6.90538991489095,4.2871099589918,1.5935598543909));
#19309=CARTESIAN_POINT('Ctrl Pts',(6.79231158966716,4.46410675522406,1.60178339346486));
#19310=CARTESIAN_POINT('Ctrl Pts',(6.67253680086821,4.63647928967222,1.61000693253882));
#19311=CARTESIAN_POINT('Ctrl Pts',(6.55278378920634,4.80882048379953,1.61822897643053));
#19312=CARTESIAN_POINT('Ctrl Pts',(6.42633691224082,4.97653885214234,1.62645102032225));
#19313=CARTESIAN_POINT('Ctrl Pts',(6.29357853297781,5.13912023713601,1.63467306421396));
#19314=CARTESIAN_POINT('Ctrl Pts',(6.16083481128717,5.30168367186222,1.64289420032717));
#19315=CARTESIAN_POINT('Ctrl Pts',(6.02178116498362,5.45911102720148,1.65111533644038));
#19316=CARTESIAN_POINT('Ctrl Pts',(5.87684048163505,5.61092091513644,1.65933647255359));
#19317=CARTESIAN_POINT('Ctrl Pts',(5.73188830230415,5.76274284388524,1.66755826072689));
#19318=CARTESIAN_POINT('Ctrl Pts',(5.58104835471498,5.90894619982334,1.67578004890019));
#19319=CARTESIAN_POINT('Ctrl Pts',(5.42478138656193,6.04908542430268,1.68400183707348));
#19320=CARTESIAN_POINT('Ctrl Pts',(5.26851485200798,6.18922425993312,1.69222360243352));
#19321=CARTESIAN_POINT('Ctrl Pts',(5.10682154838389,6.32329880286109,1.70044536779355));
#19322=CARTESIAN_POINT('Ctrl Pts',(4.94019679429501,6.45090251020253,1.70866713315358));
#19323=CARTESIAN_POINT('Ctrl Pts',(4.77353730171102,6.57853282079862,1.7168906126152));
#19324=CARTESIAN_POINT('Ctrl Pts',(4.6019445389611,6.69968942141668,1.72511409207682));
#19325=CARTESIAN_POINT('Ctrl Pts',(4.42594528711422,6.81400732887567,1.73333757153845));
#19326=CARTESIAN_POINT('Ctrl Pts',(4.35483507178077,6.86019599689882,1.73666016177204));
#19327=CARTESIAN_POINT('Ctrl Pts',(4.28300584968343,6.90526876664184,1.73998275200564));
#19328=CARTESIAN_POINT('Ctrl Pts',(4.2104936697146,6.94920359608159,1.74330534223923));
#19329=CARTESIAN_POINT('Ctrl Pts',(4.03102322545611,7.05794399474789,1.75152888131319));
#19330=CARTESIAN_POINT('Ctrl Pts',(3.84730887840118,7.15974582281657,1.75975242038716));
#19331=CARTESIAN_POINT('Ctrl Pts',(3.6599077658713,7.25429270899755,1.76797595946112));
#19332=CARTESIAN_POINT('Ctrl Pts',(3.47254072611889,7.3488224049123,1.77619800335284));
#19333=CARTESIAN_POINT('Ctrl Pts',(3.28148852195944,7.43609965887759,1.78442004724455));
#19334=CARTESIAN_POINT('Ctrl Pts',(3.08733220661952,7.5158544030915,1.79264209113626));
#19335=CARTESIAN_POINT('Ctrl Pts',(2.8931973276681,7.59560034175262,1.80086322724948));
#19336=CARTESIAN_POINT('Ctrl Pts',(2.69595929446911,7.6678253167916,1.80908436336271));
#19337=CARTESIAN_POINT('Ctrl Pts',(2.4962191927285,7.73230737259932,1.81730549947593));
#19338=CARTESIAN_POINT('Ctrl Pts',(2.29646324858557,7.79679454280652,1.82552728764923));
#19339=CARTESIAN_POINT('Ctrl Pts',(2.0942051192416,7.85353747356029,1.83374907582253));
#19340=CARTESIAN_POINT('Ctrl Pts',(1.89006212293483,7.90236374345974,1.84197086399583));
#19341=CARTESIAN_POINT('Ctrl Pts',(1.68591969307024,7.95118987787937,1.85019262935586));
#19342=CARTESIAN_POINT('Ctrl Pts',(1.47989269417367,7.99209932940237,1.8584143947159));
#19343=CARTESIAN_POINT('Ctrl Pts',(1.27261026739207,8.02497044666385,1.86663616007593));
#19344=CARTESIAN_POINT('Ctrl Pts',(1.06528462566549,8.05784841700761,1.87485963953756));
#19345=CARTESIAN_POINT('Ctrl Pts',(0.856703324525786,8.0826846590018,1.88308311899918));
#19346=CARTESIAN_POINT('Ctrl Pts',(0.647503383272865,8.09940904826705,1.89130659846081));
#19347=CARTESIAN_POINT('Ctrl Pts',(0.562978859935354,8.10616632086613,1.89462918869438));
#19348=CARTESIAN_POINT('Ctrl Pts',(0.478353406818998,8.11159995723201,1.89795177892795));
#19349=CARTESIAN_POINT('Ctrl Pts',(0.393669219340714,8.11570773920819,1.90127436916152));
#19350=CARTESIAN_POINT('Ctrl Pts',(0.184072586677869,8.12587465815208,1.90949790823548));
#19351=CARTESIAN_POINT('Ctrl Pts',(-0.0259521568726862,8.12791931177454,
1.91772144730944));
#19352=CARTESIAN_POINT('Ctrl Pts',(-0.235764444536679,8.12182877738704,
1.9259449863834));
#19353=CARTESIAN_POINT('Ctrl Pts',(-0.445538584682319,8.11573935036449,
1.93416703027511));
#19354=CARTESIAN_POINT('Ctrl Pts',(-0.655100051374277,8.10151769603698,
1.94238907416682));
#19355=CARTESIAN_POINT('Ctrl Pts',(-0.86380929461282,8.07920299689521,1.95061111805854));
#19356=CARTESIAN_POINT('Ctrl Pts',(-1.07249549470422,8.05689076147227,1.95883225417173));
#19357=CARTESIAN_POINT('Ctrl Pts',(-1.28032936604469,8.02648729648953,1.96705339028493));
#19358=CARTESIAN_POINT('Ctrl Pts',(-1.486676651568,7.98808363102081,1.97527452639813));
#19359=CARTESIAN_POINT('Ctrl Pts',(-1.69304030354357,7.94967691956213,1.98349631457143));
#19360=CARTESIAN_POINT('Ctrl Pts',(-1.89791684366065,7.90326879111565,1.99171810274472));
#19361=CARTESIAN_POINT('Ctrl Pts',(-2.10068132641448,7.8490015624507,1.99993989091802));
#19362=CARTESIAN_POINT('Ctrl Pts',(-2.30344524655115,7.79473448436278,2.00816165627806));
#19363=CARTESIAN_POINT('Ctrl Pts',(-2.50409683683983,7.73260842853375,2.01638342163809));
#19364=CARTESIAN_POINT('Ctrl Pts',(-2.70202492943812,7.66281598651533,2.02460518699813));
#19365=CARTESIAN_POINT('Ctrl Pts',(-2.89999428675781,7.59300899393141,2.03282866645975));
#19366=CARTESIAN_POINT('Ctrl Pts',(-3.0952387338803,7.51553252028115,2.04105214592138));
#19367=CARTESIAN_POINT('Ctrl Pts',(-3.28716470991994,7.43062821922594,2.049275625383));
#19368=CARTESIAN_POINT('Ctrl Pts',(-3.36470991162445,7.39632373743164,2.0525982156166));
#19369=CARTESIAN_POINT('Ctrl Pts',(-3.44171361431989,7.36080724139594,2.0559208058502));
#19370=CARTESIAN_POINT('Ctrl Pts',(-3.51813765675171,7.32409687201402,2.05924339608381));
#19371=CARTESIAN_POINT('Ctrl Pts',(-3.70729011159588,7.23323729084203,2.06746693515776));
#19372=CARTESIAN_POINT('Ctrl Pts',(-3.89295159308986,7.13503144681388,2.07569047423172));
#19373=CARTESIAN_POINT('Ctrl Pts',(-4.07455265756765,7.02977298376046,2.08391401330567));
#19374=CARTESIAN_POINT('Ctrl Pts',(-4.25612070381756,6.92453365852393,2.09213605719738));
#19375=CARTESIAN_POINT('Ctrl Pts',(-4.43362955147839,6.81224442139068,2.10035810108909));
#19376=CARTESIAN_POINT('Ctrl Pts',(-4.60653546101629,6.69324425140002,2.1085801449808));
#19377=CARTESIAN_POINT('Ctrl Pts',(-4.77942228037852,6.57425721996637,2.11680128109403));
#19378=CARTESIAN_POINT('Ctrl Pts',(-4.94770693336127,6.4485609020799,2.12502241720726));
#19379=CARTESIAN_POINT('Ctrl Pts',(-5.11087502172616,6.31653734848419,2.1332435533205));
#19380=CARTESIAN_POINT('Ctrl Pts',(-5.27405605178104,6.18450332342975,2.1414653414938));
#19381=CARTESIAN_POINT('Ctrl Pts',(-5.43211947539644,6.04614124339584,2.14968712966711));
#19382=CARTESIAN_POINT('Ctrl Pts',(-5.5845835033449,5.90187382588513,2.15790891784042));
#19383=CARTESIAN_POINT('Ctrl Pts',(-5.73704710824618,5.75760680867819,2.16613068320044));
#19384=CARTESIAN_POINT('Ctrl Pts',(-5.88391113618556,5.60743469144081,2.17435244856047));
#19385=CARTESIAN_POINT('Ctrl Pts',(-6.02472985196757,5.45181784117104,2.1825742139205));
#19386=CARTESIAN_POINT('Ctrl Pts',(-6.16557792611431,5.29616854737113,2.19079769338212));
#19387=CARTESIAN_POINT('Ctrl Pts',(-6.30037797236411,5.13507247158846,2.19902117284375));
#19388=CARTESIAN_POINT('Ctrl Pts',(-6.42872309947458,4.96902474060875,2.20724465230538));
#19389=CARTESIAN_POINT('Ctrl Pts',(-6.48057928369124,4.90193530822983,2.21056724253895));
#19390=CARTESIAN_POINT('Ctrl Pts',(-6.53138219012593,4.83403791198284,2.21388983277253));
#19391=CARTESIAN_POINT('Ctrl Pts',(-6.58110689903197,4.76536667487547,2.2172124230061));
#19392=CARTESIAN_POINT('Ctrl Pts',(-6.70417747285668,4.59540271245138,2.22543596208006));
#19393=CARTESIAN_POINT('Ctrl Pts',(-6.82068027266697,4.42064095705765,2.23365950115403));
#19394=CARTESIAN_POINT('Ctrl Pts',(-6.93025437025903,4.24161077021521,2.24188304022799));
#19395=CARTESIAN_POINT('Ctrl Pts',(-7.039808545377,4.06261313417023,2.25010508411972));
#19396=CARTESIAN_POINT('Ctrl Pts',(-7.14243637872241,3.87934886706699,2.25832712801145));
#19397=CARTESIAN_POINT('Ctrl Pts',(-7.23782113182425,3.69237495742487,2.26654917190318));
#19398=CARTESIAN_POINT('Ctrl Pts',(-7.33319535369666,3.50542169117781,2.27477030801638));
#19399=CARTESIAN_POINT('Ctrl Pts',(-7.42132795790786,3.31475986271094,2.28299144412958));
#19400=CARTESIAN_POINT('Ctrl Pts',(-7.50194851633176,3.12097036525625,2.29121258024279));
#19401=CARTESIAN_POINT('Ctrl Pts',(-7.58257546918197,2.9271654973714,2.29943436841608));
#19402=CARTESIAN_POINT('Ctrl Pts',(-7.65568907000813,2.73023273612918,2.30765615658938));
#19403=CARTESIAN_POINT('Ctrl Pts',(-7.721066929415,2.53077320872379,2.31587794476268));
#19404=CARTESIAN_POINT('Ctrl Pts',(-7.78644460741566,2.33131423476562,2.3240997101227));
#19405=CARTESIAN_POINT('Ctrl Pts',(-7.84408649763372,2.12932878976982,2.33232147548272));
#19406=CARTESIAN_POINT('Ctrl Pts',(-7.8938198421495,1.925433941268,2.34054324084274));
#19407=CARTESIAN_POINT('Ctrl Pts',(-7.94356355524215,1.72149658407445,2.34876672030437));
#19408=CARTESIAN_POINT('Ctrl Pts',(-7.98539535889943,1.51564931471102,2.35699019976601));
#19409=CARTESIAN_POINT('Ctrl Pts',(-8.01919320408771,1.30852127151739,2.36521367922764));
#19410=CARTESIAN_POINT('Ctrl Pts',(-8.03284878514227,1.22483387172174,2.36853626946123));
#19411=CARTESIAN_POINT('Ctrl Pts',(-8.0451934389306,1.14093749967722,2.37185885969482));
#19412=CARTESIAN_POINT('Ctrl Pts',(-8.05622149971853,1.0568740274853,2.37518144992841));
#19413=CARTESIAN_POINT('Ctrl Pts',(-8.0848220889386,0.838860644823607,2.38379838088706));
#19414=CARTESIAN_POINT('Ctrl Pts',(-8.10457002472343,0.619675802307401,
2.39241531184572));
#19415=CARTESIAN_POINT('Ctrl Pts',(-8.11539718216024,0.400020172348403,
2.40103224280438));
#19416=CARTESIAN_POINT('Ctrl Pts',(-8.1219604218845,0.266868644385693,2.40625568061797));
#19417=CARTESIAN_POINT('Ctrl Pts',(-8.1252466529842,0.133544246018425,2.41147911843156));
#19418=CARTESIAN_POINT('Ctrl Pts',(-8.12524999744415,0.000203798425227694,
2.41670255624514));
#19419=CARTESIAN_POINT('Origin',(0.,0.,-16.4167025567876));
#19420=CARTESIAN_POINT('',(4.94675008185375,-6.44587862049697,-0.874941805641416));
#19421=CARTESIAN_POINT('',(4.94635340022636,-6.44536135767517,-0.708351351910811));
#19422=CARTESIAN_POINT('',(4.94675008185374,-6.44587862049697,-16.4167025567876));
#19423=CARTESIAN_POINT('',(-8.12524999749084,-0.000201928347416534,0.583297443881996));
#19424=CARTESIAN_POINT('Ctrl Pts',(4.94635340024336,-6.44536135766213,-0.708351351909972));
#19425=CARTESIAN_POINT('Ctrl Pts',(5.42466120603632,-6.07850642233277,-0.684741619201049));
#19426=CARTESIAN_POINT('Ctrl Pts',(6.83911309263365,-4.72344623181886,-0.608475544184695));
#19427=CARTESIAN_POINT('Ctrl Pts',(8.30188397303846,-1.66085451139327,-0.479553126860913));
#19428=CARTESIAN_POINT('Ctrl Pts',(8.09118691949813,2.49247055018721,-0.321584099938621));
#19429=CARTESIAN_POINT('Ctrl Pts',(5.92829110923838,6.0444255090069,-0.163615073016332));
#19430=CARTESIAN_POINT('Ctrl Pts',(2.33504859606946,8.13801347159135,-0.00564604609403982));
#19431=CARTESIAN_POINT('Ctrl Pts',(-1.82158208393826,8.26810461480037,0.152322980828249));
#19432=CARTESIAN_POINT('Ctrl Pts',(-5.53871107959393,6.40331123611773,0.310292007750539));
#19433=CARTESIAN_POINT('Ctrl Pts',(-7.70380757957238,3.30246000310552,0.453950161878586));
#19434=CARTESIAN_POINT('Ctrl Pts',(-8.1241451581117,0.978652145372449,0.544951973699204));
#19435=CARTESIAN_POINT('Ctrl Pts',(-8.12508170520043,-0.000201907072085276,
0.583297443212393));
#19436=CARTESIAN_POINT('Ctrl Pts',(-8.12524999749084,-0.000201928347416534,
0.583297443881996));
#19437=CARTESIAN_POINT('Ctrl Pts',(-8.12524454021968,-0.219793150063702,
0.591899496739723));
#19438=CARTESIAN_POINT('Ctrl Pts',(-8.11633280779128,-0.43934077896469,
0.600501549597456));
#19439=CARTESIAN_POINT('Ctrl Pts',(-8.09855135892644,-0.658143942713689,
0.609103602455193));
#19440=CARTESIAN_POINT('Ctrl Pts',(-8.08675056119947,-0.803354375060902,
0.614812422168505));
#19441=CARTESIAN_POINT('Ctrl Pts',(-8.07104424286953,-0.948236954424036,
0.620521241881815));
#19442=CARTESIAN_POINT('Ctrl Pts',(-8.05145571094098,-1.09258798147143,
0.626230061595127));
#19443=CARTESIAN_POINT('Ctrl Pts',(-8.02323848464808,-1.30052523836575,
0.634453600669086));
#19444=CARTESIAN_POINT('Ctrl Pts',(-7.9869570755542,-1.50740257609528,0.642677139743043));
#19445=CARTESIAN_POINT('Ctrl Pts',(-7.94271556594821,-1.71258780824344,
0.650900678817003));
#19446=CARTESIAN_POINT('Ctrl Pts',(-7.8984821002171,-1.9177357341525,0.659122722708722));
#19447=CARTESIAN_POINT('Ctrl Pts',(-7.84629148472197,-2.12119188035655,
0.667344766600445));
#19448=CARTESIAN_POINT('Ctrl Pts',(-7.78629884822644,-2.32233456000802,
0.675566810492164));
#19449=CARTESIAN_POINT('Ctrl Pts',(-7.7263128353911,-2.52345503192138,0.683787946605395));
#19450=CARTESIAN_POINT('Ctrl Pts',(-7.65852660558248,-2.7222622647074,0.692009082718634));
#19451=CARTESIAN_POINT('Ctrl Pts',(-7.58314530014621,-2.91814922842722,
0.700230218831866));
#19452=CARTESIAN_POINT('Ctrl Pts',(-7.50775801583566,-3.11405172893727,
0.708452007005168));
#19453=CARTESIAN_POINT('Ctrl Pts',(-7.42477455569331,-3.30703322136361,
0.716673795178469));
#19454=CARTESIAN_POINT('Ctrl Pts',(-7.33444879144874,-3.49650518205193,
0.724895583351771));
#19455=CARTESIAN_POINT('Ctrl Pts',(-7.24412327783427,-3.68597661700571,
0.733117348711786));
#19456=CARTESIAN_POINT('Ctrl Pts',(-7.14645563022167,-3.87193827463395,
0.741339114071796));
#19457=CARTESIAN_POINT('Ctrl Pts',(-7.04174664052734,-4.05382434413752,
0.749560879431812));
#19458=CARTESIAN_POINT('Ctrl Pts',(-6.93701582074652,-4.23574833386779,
0.757784358893447));
#19459=CARTESIAN_POINT('Ctrl Pts',(-6.82524087340846,-4.41359478238217,
0.766007838355089));
#19460=CARTESIAN_POINT('Ctrl Pts',(-6.70676762011063,-4.58682413575401,
0.774231317816724));
#19461=CARTESIAN_POINT('Ctrl Pts',(-6.65890003848872,-4.65681520952821,
0.777553908050289));
#19462=CARTESIAN_POINT('Ctrl Pts',(-6.60993948329258,-4.72605288535702,
0.780876498283847));
#19463=CARTESIAN_POINT('Ctrl Pts',(-6.55991074893576,-4.794502949055,0.784199088517411));
#19464=CARTESIAN_POINT('Ctrl Pts',(-6.43608770038518,-4.96391949875449,
0.792422627591374));
#19465=CARTESIAN_POINT('Ctrl Pts',(-6.30567799401478,-5.12856421320448,
0.800646166665331));
#19466=CARTESIAN_POINT('Ctrl Pts',(-6.1690741731326,-5.28793073034135,0.808869705739294));
#19467=CARTESIAN_POINT('Ctrl Pts',(-6.03249518919806,-5.44726827187697,
0.817091749630999));
#19468=CARTESIAN_POINT('Ctrl Pts',(-5.8897245303625,-5.60132930766949,0.825313793522708));
#19469=CARTESIAN_POINT('Ctrl Pts',(-5.74119462889958,-5.74964101449774,
0.833535837414413));
#19470=CARTESIAN_POINT('Ctrl Pts',(-5.59268112630853,-5.89793634654453,
0.841756973527664));
#19471=CARTESIAN_POINT('Ctrl Pts',(-5.43840985919502,-6.04048340860856,
0.84997810964091));
#19472=CARTESIAN_POINT('Ctrl Pts',(-5.27885026010335,-6.17684607982964,
0.858199245754161));
#19473=CARTESIAN_POINT('Ctrl Pts',(-5.11927800552985,-6.31321956666644,
0.866421033927452));
#19474=CARTESIAN_POINT('Ctrl Pts',(-4.95441680338497,-6.44340748893084,
0.874642822100743));
#19475=CARTESIAN_POINT('Ctrl Pts',(-4.78477012607616,-6.56701320259897,
0.882864610274034));
#19476=CARTESIAN_POINT('Ctrl Pts',(-4.61512391949124,-6.69061857329449,
0.891086375634074));
#19477=CARTESIAN_POINT('Ctrl Pts',(-4.4406925042627,-6.80764160042871,0.899308140994116));
#19478=CARTESIAN_POINT('Ctrl Pts',(-4.26200979787171,-6.917727953985,0.907529906354156));
#19479=CARTESIAN_POINT('Ctrl Pts',(-4.08328983910292,-7.02783725871836,
0.915753385815777));
#19480=CARTESIAN_POINT('Ctrl Pts',(-3.90031706969813,-7.13100684608687,
0.923976865277399));
#19481=CARTESIAN_POINT('Ctrl Pts',(-3.71365250227889,-7.2269269163883,0.932200344739019));
#19482=CARTESIAN_POINT('Ctrl Pts',(-3.63823310449802,-7.26568217689248,
0.935522934972579));
#19483=CARTESIAN_POINT('Ctrl Pts',(-3.56221131900306,-7.30325450513318,
0.938845525206136));
#19484=CARTESIAN_POINT('Ctrl Pts',(-3.48562524024981,-7.33962562035922,
0.942168115439696));
#19485=CARTESIAN_POINT('Ctrl Pts',(-3.29607173925316,-7.4296455344021,0.950391654513652));
#19486=CARTESIAN_POINT('Ctrl Pts',(-3.10299829935624,-7.51233302026449,
0.958615193587611));
#19487=CARTESIAN_POINT('Ctrl Pts',(-2.90699121411446,-7.58742971259447,
0.966838732661568));
#19488=CARTESIAN_POINT('Ctrl Pts',(-2.71101976636533,-7.66251275104139,
0.975060776553282));
#19489=CARTESIAN_POINT('Ctrl Pts',(-2.51211601312836,-7.73000764508645,
0.983282820444989));
#19490=CARTESIAN_POINT('Ctrl Pts',(-2.31088535521694,-7.7897045154193,0.991504864336704));
#19491=CARTESIAN_POINT('Ctrl Pts',(-2.10967691475733,-7.84939479474681,
0.999726000449923));
#19492=CARTESIAN_POINT('Ctrl Pts',(-1.9061423651767,-7.9012886853945,1.00794713656314));
#19493=CARTESIAN_POINT('Ctrl Pts',(-1.70090216801825,-7.94522620051379,
1.01616827267636));
#19494=CARTESIAN_POINT('Ctrl Pts',(-1.49564569221677,-7.98916720054069,
1.02439006084967));
#19495=CARTESIAN_POINT('Ctrl Pts',(-1.28868358638215,-8.02515049978894,
1.03261184902297));
#19496=CARTESIAN_POINT('Ctrl Pts',(-1.08064744844194,-8.05306703403591,
1.04083363719628));
#19497=CARTESIAN_POINT('Ctrl Pts',(-0.872611887746392,-8.08098349082196,
1.04905540255631));
#19498=CARTESIAN_POINT('Ctrl Pts',(-0.663502593577219,-8.10083319082789,
1.05727716791634));
#19499=CARTESIAN_POINT('Ctrl Pts',(-0.453957788196302,-8.11255877569068,
1.06549893327638));
#19500=CARTESIAN_POINT('Ctrl Pts',(-0.244369296202404,-8.12428680514325,
1.07372241273799));
#19501=CARTESIAN_POINT('Ctrl Pts',(-0.0343454061356596,-8.12788731935881,
1.08194589219961));
#19502=CARTESIAN_POINT('Ctrl Pts',(0.175473036514424,-8.12335501969207,
1.09016937166123));
#19503=CARTESIAN_POINT('Ctrl Pts',(0.260247457321311,-8.12152380278703,
1.09349196189481));
#19504=CARTESIAN_POINT('Ctrl Pts',(0.344988339062686,-8.11836553093617,
1.0968145521284));
#19505=CARTESIAN_POINT('Ctrl Pts',(0.429653478469153,-8.11388226750545,
1.10013714236199));
#19506=CARTESIAN_POINT('Ctrl Pts',(0.639202966417737,-8.10278601746875,
1.10836068143595));
#19507=CARTESIAN_POINT('Ctrl Pts',(0.848356402118719,-8.08356587578453,
1.1165842205099));
#19508=CARTESIAN_POINT('Ctrl Pts',(1.05647519957539,-8.05627381083725,1.12480775958386));
#19509=CARTESIAN_POINT('Ctrl Pts',(1.26455615741984,-8.02898670806142,1.13302980347558));
#19510=CARTESIAN_POINT('Ctrl Pts',(1.47160256019026,-7.99363064954546,1.1412518473673));
#19511=CARTESIAN_POINT('Ctrl Pts',(1.67698210643768,-7.95030933845897,1.14947389125902));
#19512=CARTESIAN_POINT('Ctrl Pts',(1.88233897716292,-7.90699281038699,1.15769502737223));
#19513=CARTESIAN_POINT('Ctrl Pts',(2.08602907031019,-7.85571284633579,1.16591616348543));
#19514=CARTESIAN_POINT('Ctrl Pts',(2.28743059701466,-7.79662419424851,1.17413729959864));
#19515=CARTESIAN_POINT('Ctrl Pts',(2.48884809789793,-7.73753085553987,1.18235908777194));
#19516=CARTESIAN_POINT('Ctrl Pts',(2.68797638588887,-7.67062767177349,1.19058087594524));
#19517=CARTESIAN_POINT('Ctrl Pts',(2.88420812614501,-7.59611947296638,1.19880266411855));
#19518=CARTESIAN_POINT('Ctrl Pts',(3.08043932191014,-7.52161148089976,1.20702442947857));
#19519=CARTESIAN_POINT('Ctrl Pts',(3.27377371124921,-7.43949862321621,1.21524619483858));
#19520=CARTESIAN_POINT('Ctrl Pts',(3.46362275400914,-7.35003435232858,1.2234679601986));
#19521=CARTESIAN_POINT('Ctrl Pts',(3.65351137714319,-7.26055142962547,1.23169143966023));
#19522=CARTESIAN_POINT('Ctrl Pts',(3.83991293524429,-7.16371415767408,1.23991491912185));
#19523=CARTESIAN_POINT('Ctrl Pts',(4.02226136976297,-7.05982301731513,1.24813839858348));
#19524=CARTESIAN_POINT('Ctrl Pts',(4.09593689001824,-7.01784714932338,1.25146098881708));
#19525=CARTESIAN_POINT('Ctrl Pts',(4.16895103655659,-6.97472028849727,1.25478357905068));
#19526=CARTESIAN_POINT('Ctrl Pts',(4.24126767987653,-6.93046434448189,1.25810616928428));
#19527=CARTESIAN_POINT('Ctrl Pts',(4.42025268512709,-6.82093007950061,1.26632964043981));
#19528=CARTESIAN_POINT('Ctrl Pts',(4.59502127405933,-6.70444066393231,1.27455311159534));
#19529=CARTESIAN_POINT('Ctrl Pts',(4.76503665606771,-6.58134585239456,1.28277658275087));
#19530=CARTESIAN_POINT('Ctrl Pts',(4.82623136667004,-6.53703955916557,1.28573650867971));
#19531=CARTESIAN_POINT('Ctrl Pts',(4.88681054383818,-6.4918779220727,1.28869643460856));
#19532=CARTESIAN_POINT('Ctrl Pts',(4.94675008185373,-6.44587862049698,1.2916563605374));
#19533=CARTESIAN_POINT('',(-8.12524999914245,-0.000118049505365691,0.416702556809683));
#19534=CARTESIAN_POINT('Ctrl Pts',(-8.12524999914245,-0.000118049505388336,
0.416702556809685));
#19535=CARTESIAN_POINT('Ctrl Pts',(-8.12524687413322,-0.215209854325447,
0.425126747983452));
#19536=CARTESIAN_POINT('Ctrl Pts',(-8.11669853744178,-0.430268792361165,
0.433550939157217));
#19537=CARTESIAN_POINT('Ctrl Pts',(-8.09963879299085,-0.644623134535036,
0.441975130330984));
#19538=CARTESIAN_POINT('Ctrl Pts',(-8.0825735898145,-0.859046065162715,
0.450402017051954));
#19539=CARTESIAN_POINT('Ctrl Pts',(-8.05699155812681,-1.07276368770188,
0.458828903772924));
#19540=CARTESIAN_POINT('Ctrl Pts',(-8.02297843455734,-1.28510878960804,
0.467255790493894));
#19541=CARTESIAN_POINT('Ctrl Pts',(-8.00643334361702,-1.38840036218568,
0.471354902616232));
#19542=CARTESIAN_POINT('Ctrl Pts',(-7.98789409470883,-1.49136727577943,
0.475454014738572));
#19543=CARTESIAN_POINT('Ctrl Pts',(-7.96737495602483,-1.59393345927877,
0.47955312686091));
#19544=CARTESIAN_POINT('Ctrl Pts',(-7.92620995889962,-1.79969924281946,
0.487776665934872));
#19545=CARTESIAN_POINT('Ctrl Pts',(-7.87706284174904,-2.00390290191428,
0.496000205008835));
#19546=CARTESIAN_POINT('Ctrl Pts',(-7.82007701584039,-2.20591999601636,
0.504223744082797));
#19547=CARTESIAN_POINT('Ctrl Pts',(-7.76310155094478,-2.40790035990155,
0.512445787974506));
#19548=CARTESIAN_POINT('Ctrl Pts',(-7.69829030188612,-2.6076946685525,0.520667831866216));
#19549=CARTESIAN_POINT('Ctrl Pts',(-7.62583696993005,-2.8046921525451,0.528889875757926));
#19550=CARTESIAN_POINT('Ctrl Pts',(-7.55339163739346,-3.00166788646123,
0.537111011871121));
#19551=CARTESIAN_POINT('Ctrl Pts',(-7.47330600823432,-3.19584713551087,
0.545332147984315));
#19552=CARTESIAN_POINT('Ctrl Pts',(-7.38582278187531,-3.38663688594329,
0.553553284097511));
#19553=CARTESIAN_POINT('Ctrl Pts',(-7.29833261677692,-3.57744176888064,
0.561775072270801));
#19554=CARTESIAN_POINT('Ctrl Pts',(-7.20344380264089,-3.76485634683022,
0.569996860444087));
#19555=CARTESIAN_POINT('Ctrl Pts',(-7.10144651664431,-3.94830912337678,
0.578218648617376));
#19556=CARTESIAN_POINT('Ctrl Pts',(-6.9994495136629,-4.13176139089098,0.586440413977404));
#19557=CARTESIAN_POINT('Ctrl Pts',(-6.89034422394947,-4.31125162253243,
0.594662179337436));
#19558=CARTESIAN_POINT('Ctrl Pts',(-6.77446623273054,-4.48623392436168,
0.602883944697464));
#19559=CARTESIAN_POINT('Ctrl Pts',(-6.65856408287404,-4.66125270709613,
0.611107424159086));
#19560=CARTESIAN_POINT('Ctrl Pts',(-6.53588657362123,-4.83176143656474,
0.619330903620711));
#19561=CARTESIAN_POINT('Ctrl Pts',(-6.40681258982334,-4.99724324016563,
0.627554383082334));
#19562=CARTESIAN_POINT('Ctrl Pts',(-6.35466192051321,-5.06410401692719,
0.630876973315957));
#19563=CARTESIAN_POINT('Ctrl Pts',(-6.30146752914131,-5.13014452302852,
0.634199563549582));
#19564=CARTESIAN_POINT('Ctrl Pts',(-6.24725630112025,-5.19533216172107,
0.637522153783205));
#19565=CARTESIAN_POINT('Ctrl Pts',(-6.11308141931654,-5.35667408360554,
0.645745692857165));
#19566=CARTESIAN_POINT('Ctrl Pts',(-5.97263116900281,-5.51284162408282,
0.653969231931124));
#19567=CARTESIAN_POINT('Ctrl Pts',(-5.82632898970532,-5.66335395911463,
0.662192771005085));
#19568=CARTESIAN_POINT('Ctrl Pts',(-5.68005341068557,-5.81383892838926,
0.670414814896784));
#19569=CARTESIAN_POINT('Ctrl Pts',(-5.52792823173882,-5.95867053303468,
0.678636858788479));
#19570=CARTESIAN_POINT('Ctrl Pts',(-5.37041460599619,-6.09740391660277,
0.686858902680179));
#19571=CARTESIAN_POINT('Ctrl Pts',(-5.21291837099923,-6.23612198291194,
0.695080038793433));
#19572=CARTESIAN_POINT('Ctrl Pts',(-5.05003509819688,-6.36874297748343,
0.703301174906686));
#19573=CARTESIAN_POINT('Ctrl Pts',(-4.88226057345853,-6.49486098814689,
0.711522311019941));
#19574=CARTESIAN_POINT('Ctrl Pts',(-4.71447274167077,-6.62098900187012,
0.719744099193243));
#19575=CARTESIAN_POINT('Ctrl Pts',(-4.54179311695569,-6.74061282175792,
0.727965887366544));
#19576=CARTESIAN_POINT('Ctrl Pts',(-4.36474898981035,-6.85336806383909,
0.736187675539846));
#19577=CARTESIAN_POINT('Ctrl Pts',(-4.1877053539147,-6.96612299305487,0.744409440899902));
#19578=CARTESIAN_POINT('Ctrl Pts',(-4.00629749002726,-7.0720092264295,0.752631206259964));
#19579=CARTESIAN_POINT('Ctrl Pts',(-3.82108042810118,-7.17070651501525,
0.760852971620022));
#19580=CARTESIAN_POINT('Ctrl Pts',(-3.63582475149297,-7.26942438034692,
0.769076451081645));
#19581=CARTESIAN_POINT('Ctrl Pts',(-3.4467585506843,-7.36095016804224,0.777299930543269));
#19582=CARTESIAN_POINT('Ctrl Pts',(-3.25446111311436,-7.44500976666428,
0.785523410004892));
#19583=CARTESIAN_POINT('Ctrl Pts',(-3.17676582719734,-7.47897295739391,
0.788846000238426));
#19584=CARTESIAN_POINT('Ctrl Pts',(-3.09854330512629,-7.51171786173033,
0.792168590471956));
#19585=CARTESIAN_POINT('Ctrl Pts',(-3.01983270995662,-7.54322861687063,
0.79549118070549));
#19586=CARTESIAN_POINT('Ctrl Pts',(-2.82502094882545,-7.62121895210089,
0.803714719779445));
#19587=CARTESIAN_POINT('Ctrl Pts',(-2.62715465840083,-7.69167109632274,
0.8119382588534));
#19588=CARTESIAN_POINT('Ctrl Pts',(-2.4268351412202,-7.75436385268571,0.820161797927355));
#19589=CARTESIAN_POINT('Ctrl Pts',(-2.22655204560707,-7.81704521041668,
0.828383841819075));
#19590=CARTESIAN_POINT('Ctrl Pts',(-2.02381689481391,-7.87196990802028,
0.836605885710796));
#19591=CARTESIAN_POINT('Ctrl Pts',(-1.81924702925051,-7.91896633463378,
0.844827929602516));
#19592=CARTESIAN_POINT('Ctrl Pts',(-1.61469974981416,-7.96595757247102,
0.853049065715726));
#19593=CARTESIAN_POINT('Ctrl Pts',(-1.40831844736009,-8.00502222089918,
0.86127020182893));
#19594=CARTESIAN_POINT('Ctrl Pts',(-1.20073237361383,-8.03603940566842,
0.86949133794214));
#19595=CARTESIAN_POINT('Ctrl Pts',(-0.993129835160831,-8.06705905056826,
0.877713126115445));
#19596=CARTESIAN_POINT('Ctrl Pts',(-0.784322625798179,-8.09002991024968,
0.885934914288751));
#19597=CARTESIAN_POINT('Ctrl Pts',(-0.574947927482478,-8.10488262982158,
0.894156702462055));
#19598=CARTESIAN_POINT('Ctrl Pts',(-0.365573810125681,-8.11973530818115,
0.902378467822092));
#19599=CARTESIAN_POINT('Ctrl Pts',(-0.155632501349239,-8.12646987331069,
0.91060023318213));
#19600=CARTESIAN_POINT('Ctrl Pts',(0.0542354388566744,-8.12506898922538,
0.918821998542168));
#19601=CARTESIAN_POINT('Ctrl Pts',(0.264147133044124,-8.123667813079,0.927045478003794));
#19602=CARTESIAN_POINT('Ctrl Pts',(0.473985133124605,-8.11412780135323,
0.935268957465419));
#19603=CARTESIAN_POINT('Ctrl Pts',(0.683109516478365,-8.09648373993283,
0.943492436927045));
#19604=CARTESIAN_POINT('Ctrl Pts',(0.767603511626854,-8.08935488572584,
0.946815027160623));
#19605=CARTESIAN_POINT('Ctrl Pts',(0.851981048272906,-8.08090367108565,
0.950137617394203));
#19606=CARTESIAN_POINT('Ctrl Pts',(0.936200134772983,-8.07113479444812,
0.953460207627781));
#19607=CARTESIAN_POINT('Ctrl Pts',(1.14464562456212,-8.04695644770961,0.961683746701744));
#19608=CARTESIAN_POINT('Ctrl Pts',(1.35218782376651,-8.01469487519154,0.969907285775705));
#19609=CARTESIAN_POINT('Ctrl Pts',(1.55819264593138,-7.97444187643658,0.978130824849668));
#19610=CARTESIAN_POINT('Ctrl Pts',(1.76416001284117,-7.93419619637601,0.986352868741379));
#19611=CARTESIAN_POINT('Ctrl Pts',(1.96859027128783,-7.88596204659278,0.994574912633096));
#19612=CARTESIAN_POINT('Ctrl Pts',(2.17085884220969,-7.82988246717025,1.00279695652481));
#19613=CARTESIAN_POINT('Ctrl Pts',(2.3731050810857,-7.77380907937566,1.01101809263801));
#19614=CARTESIAN_POINT('Ctrl Pts',(2.57318982482481,-7.70989207004109,1.01923922875122));
#19615=CARTESIAN_POINT('Ctrl Pts',(2.77050217837134,-7.63832476673646,1.02746036486442));
#19616=CARTESIAN_POINT('Ctrl Pts',(2.96783018176366,-7.56675178706521,1.03568215303772));
#19617=CARTESIAN_POINT('Ctrl Pts',(3.16238507742671,-7.48752739909126,1.04390394121103));
#19618=CARTESIAN_POINT('Ctrl Pts',(3.35357352783447,-7.40089401058466,1.05212572938433));
#19619=CARTESIAN_POINT('Ctrl Pts',(3.54476144774538,-7.31426086246256,1.06034749474437));
#19620=CARTESIAN_POINT('Ctrl Pts',(3.73258267355998,-7.22021887911594,1.0685692601044));
#19621=CARTESIAN_POINT('Ctrl Pts',(3.91646566617528,-7.11905782025755,1.07679102546444));
#19622=CARTESIAN_POINT('Ctrl Pts',(4.1003869953419,-7.01787567099776,1.08501450492607));
#19623=CARTESIAN_POINT('Ctrl Pts',(4.28036819261821,-6.90957162338873,1.0932379843877));
#19624=CARTESIAN_POINT('Ctrl Pts',(4.45586309734674,-6.79448096768278,1.10146146384933));
#19625=CARTESIAN_POINT('Ctrl Pts',(4.52676953776714,-6.74798008075171,1.10478405408291));
#19626=CARTESIAN_POINT('Ctrl Pts',(4.59694392351972,-6.70037181147411,1.10810664431649));
#19627=CARTESIAN_POINT('Ctrl Pts',(4.66635156589433,-6.65168028591088,1.11142923455007));
#19628=CARTESIAN_POINT('Ctrl Pts',(4.76126383227299,-6.58509650800792,1.1159727481824));
#19629=CARTESIAN_POINT('Ctrl Pts',(4.85475927892587,-6.51647497185647,1.12051626181472));
#19630=CARTESIAN_POINT('Ctrl Pts',(4.94675008185375,-6.44587862049697,1.12505977544705));
#19631=CARTESIAN_POINT('Ctrl Pts',(4.94675008185375,-6.44587862049697,-0.874941805641418));
#19632=CARTESIAN_POINT('Ctrl Pts',(5.11327314749972,-6.31808409672245,-0.86671990801957));
#19633=CARTESIAN_POINT('Ctrl Pts',(5.27484531963509,-6.18383017067312,-0.858498010397723));
#19634=CARTESIAN_POINT('Ctrl Pts',(5.43097363732824,-6.04352652953106,-0.850276112775875));
#19635=CARTESIAN_POINT('Ctrl Pts',(5.58709844738019,-5.90322604050668,-0.842054399870465));
#19636=CARTESIAN_POINT('Ctrl Pts',(5.73777942951179,-5.75687630682174,-0.833832686965053));
#19637=CARTESIAN_POINT('Ctrl Pts',(5.88255864950201,-5.60492562820142,-0.825610974059643));
#19638=CARTESIAN_POINT('Ctrl Pts',(6.02737062138856,-5.45294057536032,-0.817387401241679));
#19639=CARTESIAN_POINT('Ctrl Pts',(6.16627795939731,-5.29535225899986,-0.809163828423718));
#19640=CARTESIAN_POINT('Ctrl Pts',(6.2988605775536,-5.13264483351821,-0.800940255605756));
#19641=CARTESIAN_POINT('Ctrl Pts',(6.38882908689042,-5.02223409693612,-0.795359866576308));
#19642=CARTESIAN_POINT('Ctrl Pts',(6.47588600295847,-4.90946686505836,-0.789779477546862));
#19643=CARTESIAN_POINT('Ctrl Pts',(6.55991074893582,-4.79450294905492,-0.784199088517413));
#19644=CARTESIAN_POINT('Ctrl Pts',(6.68373379748634,-4.6250863993555,-0.775975549443454));
#19645=CARTESIAN_POINT('Ctrl Pts',(6.80101041183197,-4.45084297985416,-0.767752010369493));
#19646=CARTESIAN_POINT('Ctrl Pts',(6.91137731992751,-4.27230044637449,-0.759528471295534));
#19647=CARTESIAN_POINT('Ctrl Pts',(7.02172416140205,-4.09379037502874,-0.751306427403823));
#19648=CARTESIAN_POINT('Ctrl Pts',(7.12516364906538,-3.91098300054452,-0.743084383512117));
#19649=CARTESIAN_POINT('Ctrl Pts',(7.22137657766206,-3.72443390142633,-0.734862339620406));
#19650=CARTESIAN_POINT('Ctrl Pts',(7.3175788835926,-3.53790539879999,-0.726641203507188));
#19651=CARTESIAN_POINT('Ctrl Pts',(7.40655608823384,-3.34763625833373,-0.718420067393964));
#19652=CARTESIAN_POINT('Ctrl Pts',(7.48803519021739,-3.15420616836724,-0.710198931280747));
#19653=CARTESIAN_POINT('Ctrl Pts',(7.56952075472257,-2.96076073647738,-0.701977143107448));
#19654=CARTESIAN_POINT('Ctrl Pts',(7.6435069113411,-2.7641541249276,-0.69375535493415));
#19655=CARTESIAN_POINT('Ctrl Pts',(7.70976860723802,-2.56498646884289,-0.685533566760851));
#19656=CARTESIAN_POINT('Ctrl Pts',(7.7760301192764,-2.36581936539532,-0.677311801400822));
#19657=CARTESIAN_POINT('Ctrl Pts',(7.83456712292162,-2.16409151232984,-0.669090036040793));
#19658=CARTESIAN_POINT('Ctrl Pts',(7.88520412564079,-1.96041920503689,-0.660868270680764));
#19659=CARTESIAN_POINT('Ctrl Pts',(7.93585168533444,-1.75670443544888,-0.65264479121914));
#19660=CARTESIAN_POINT('Ctrl Pts',(7.97859588265768,-1.55104468805848,-0.644421311757514));
#19661=CARTESIAN_POINT('Ctrl Pts',(8.01331187993856,-1.344068553808,-0.63619783229589));
#19662=CARTESIAN_POINT('Ctrl Pts',(8.02733842843948,-1.26044253085067,-0.6328752420623));
#19663=CARTESIAN_POINT('Ctrl Pts',(8.0400549892254,-1.17660172454979,-0.629552651828708));
#19664=CARTESIAN_POINT('Ctrl Pts',(8.05145571094102,-1.09258798147116,-0.626230061595118));
#19665=CARTESIAN_POINT('Ctrl Pts',(8.07967293723391,-0.88465072457684,-0.618006522521159));
#19666=CARTESIAN_POINT('Ctrl Pts',(8.09983514702286,-0.675586000607633,
-0.609782983447201));
#19667=CARTESIAN_POINT('Ctrl Pts',(8.11187418476942,-0.466030871264436,
-0.601559444373242));
#19668=CARTESIAN_POINT('Ctrl Pts',(8.12391103360979,-0.256513842683761,
-0.593337400481531));
#19669=CARTESIAN_POINT('Ctrl Pts',(8.12782764129082,-0.046506880994045,
-0.585115356589818));
#19670=CARTESIAN_POINT('Ctrl Pts',(8.12360785080587,0.163349468395798,-0.576893312698108));
#19671=CARTESIAN_POINT('Ctrl Pts',(8.11938852621907,0.373182647989396,-0.568672176584895));
#19672=CARTESIAN_POINT('Ctrl Pts',(8.10703460286112,0.582864953721563,-0.560451040471686));
#19673=CARTESIAN_POINT('Ctrl Pts',(8.08658203365941,0.791756638997664,-0.552229904358473));
#19674=CARTESIAN_POINT('Ctrl Pts',(8.06612784226048,1.00066489253497,-0.544008116185173));
#19675=CARTESIAN_POINT('Ctrl Pts',(8.03757374765707,1.20878210652183,-0.53578632801187));
#19676=CARTESIAN_POINT('Ctrl Pts',(8.00100760271659,1.41547338504518,-0.52756453983857));
#19677=CARTESIAN_POINT('Ctrl Pts',(7.96444155923741,1.6221640900554,-0.519342774478538));
#19678=CARTESIAN_POINT('Ctrl Pts',(7.91986356392611,1.82742857756414,-0.511121009118508));
#19679=CARTESIAN_POINT('Ctrl Pts',(7.86741274588157,2.03064133919318,-0.502899243758476));
#19680=CARTESIAN_POINT('Ctrl Pts',(7.81495099271218,2.23389646730957,-0.494675764296853));
#19681=CARTESIAN_POINT('Ctrl Pts',(7.75461321157937,2.43509872939787,-0.486452284835224));
#19682=CARTESIAN_POINT('Ctrl Pts',(7.68658893013407,2.63363592427662,-0.4782288053736));
#19683=CARTESIAN_POINT('Ctrl Pts',(7.65910460136156,2.71385230321782,-0.474906215140009));
#19684=CARTESIAN_POINT('Ctrl Pts',(7.63036604866938,2.79363380049986,-0.471583624906421));
#19685=CARTESIAN_POINT('Ctrl Pts',(7.60038805194703,2.87294083167766,-0.46826103467283));
#19686=CARTESIAN_POINT('Ctrl Pts',(7.52619135296413,3.06922879494708,-0.460037495598869));
#19687=CARTESIAN_POINT('Ctrl Pts',(7.44437452692853,3.26267279327572,-0.451813956524908));
#19688=CARTESIAN_POINT('Ctrl Pts',(7.35518097901611,3.45268016596088,-0.443590417450947));
#19689=CARTESIAN_POINT('Ctrl Pts',(7.26600364803999,3.64265299200525,-0.435368373559233));
#19690=CARTESIAN_POINT('Ctrl Pts',(7.16945239736635,3.82919017266169,-0.427146329667522));
#19691=CARTESIAN_POINT('Ctrl Pts',(7.06581801651437,4.01172074302299,-0.418924285775809));
#19692=CARTESIAN_POINT('Ctrl Pts',(6.96219507771549,4.19423116056954,-0.410703149662595));
#19693=CARTESIAN_POINT('Ctrl Pts',(6.8514907156021,4.3727355946001,-0.402482013549381));
#19694=CARTESIAN_POINT('Ctrl Pts',(6.73404116286537,4.54668859493752,-0.394260877436167));
#19695=CARTESIAN_POINT('Ctrl Pts',(6.61658229460772,4.72065539237142,-0.386039089262869));
#19696=CARTESIAN_POINT('Ctrl Pts',(6.49237732960357,4.89006978888062,-0.377817301089569));
#19697=CARTESIAN_POINT('Ctrl Pts',(6.36180582974787,5.05441531208962,-0.36959551291627));
#19698=CARTESIAN_POINT('Ctrl Pts',(6.23123469219314,5.21876037928376,-0.361373747556233));
#19699=CARTESIAN_POINT('Ctrl Pts',(6.09429724070153,5.37803637206743,-0.353151982196201));
#19700=CARTESIAN_POINT('Ctrl Pts',(5.95141365767106,5.53175948842557,-0.344930216836165));
#19701=CARTESIAN_POINT('Ctrl Pts',(5.8085002857856,5.68551465350145,-0.336706737374544));
#19702=CARTESIAN_POINT('Ctrl Pts',(5.65963850668627,5.8337144133691,-0.328483257912925));
#19703=CARTESIAN_POINT('Ctrl Pts',(5.50528648511832,5.97591066526882,-0.320259778451305));
#19704=CARTESIAN_POINT('Ctrl Pts',(5.4429225524558,6.03336321683408,-0.316937188217719));
#19705=CARTESIAN_POINT('Ctrl Pts',(5.37966277217823,6.08983614768258,-0.313614597984127));
#19706=CARTESIAN_POINT('Ctrl Pts',(5.31553898940635,6.14530168621532,-0.31029200775054));
#19707=CARTESIAN_POINT('Ctrl Pts',(5.15683015198659,6.28258103495103,-0.302068468676578));
#19708=CARTESIAN_POINT('Ctrl Pts',(4.99277462089054,6.4137311635393,-0.293844929602612));
#19709=CARTESIAN_POINT('Ctrl Pts',(4.82386863449584,6.53834680631329,-0.28562139052865));
#19710=CARTESIAN_POINT('Ctrl Pts',(4.6549933581435,6.66293979179875,-0.277399346636941));
#19711=CARTESIAN_POINT('Ctrl Pts',(4.48126962387305,6.7810004877351,-0.269177302745237));
#19712=CARTESIAN_POINT('Ctrl Pts',(4.30322500757334,6.89216526910777,-0.260955258853528));
#19713=CARTESIAN_POINT('Ctrl Pts',(4.12520004880356,7.0033177770118,-0.252734122740314));
#19714=CARTESIAN_POINT('Ctrl Pts',(3.94285541051428,7.10757573424601,-0.244512986627104));
#19715=CARTESIAN_POINT('Ctrl Pts',(3.75674648071624,7.2046195903827,-0.23629185051389));
#19716=CARTESIAN_POINT('Ctrl Pts',(3.57062278967321,7.30167114356077,-0.228070062340593));
#19717=CARTESIAN_POINT('Ctrl Pts',(3.38073447086042,7.39150731364108,-0.21984827416729));
#19718=CARTESIAN_POINT('Ctrl Pts',(3.1876612165152,7.47385466350697,-0.211626485993992));
#19719=CARTESIAN_POINT('Ctrl Pts',(2.99458849789658,7.55620178488101,-0.203404720633957));
#19720=CARTESIAN_POINT('Ctrl Pts',(2.79833113376881,7.63106001438087,-0.195182955273926));
#19721=CARTESIAN_POINT('Ctrl Pts',(2.59948898044392,7.69820398554433,-0.186961189913891));
#19722=CARTESIAN_POINT('Ctrl Pts',(2.4006053718309,7.76536195511117,-0.178737710452262));
#19723=CARTESIAN_POINT('Ctrl Pts',(2.1991361769637,7.82480235905585,-0.17051423099063));
#19724=CARTESIAN_POINT('Ctrl Pts',(1.99569765411705,7.87634930890268,-0.162290751529));
#19725=CARTESIAN_POINT('Ctrl Pts',(1.91350095717157,7.89717618552239,-0.158968161295416));
#19726=CARTESIAN_POINT('Ctrl Pts',(1.83098293428684,7.91671506006955,-0.155645571061832));
#19727=CARTESIAN_POINT('Ctrl Pts',(1.74818481239271,7.9349566743757,-0.152322980828249));
#19728=CARTESIAN_POINT('Ctrl Pts',(1.54325626485029,7.98010537387601,-0.144099441754288));
#19729=CARTESIAN_POINT('Ctrl Pts',(1.33654447896043,8.01731842382004,-0.135875902680326));
#19730=CARTESIAN_POINT('Ctrl Pts',(1.12867879653315,8.046475733932,-0.127652363606366));
#19731=CARTESIAN_POINT('Ctrl Pts',(0.920850907697369,8.07562774273854,-0.119430319714644));
#19732=CARTESIAN_POINT('Ctrl Pts',(0.711869832988523,8.09672689408454,-0.11120827582293));
#19733=CARTESIAN_POINT('Ctrl Pts',(0.502372643946926,8.10970463636708,-0.102986231931208));
#19734=CARTESIAN_POINT('Ctrl Pts',(0.292898585047747,8.12268094580449,-0.0947650958179964));
#19735=CARTESIAN_POINT('Ctrl Pts',(0.0829088198363098,8.12753761811397,
-0.0865439597047853));
#19736=CARTESIAN_POINT('Ctrl Pts',(-0.12695610943686,8.12425810205317,-0.0783228235915736));
#19737=CARTESIAN_POINT('Ctrl Pts',(-0.336837684164142,8.12097832587729,
-0.0701010354182755));
#19738=CARTESIAN_POINT('Ctrl Pts',(-0.546594108220713,8.10956107387643,
-0.061879247244974));
#19739=CARTESIAN_POINT('Ctrl Pts',(-0.755585424101854,8.09004191765314,
-0.0536574590716761));
#19740=CARTESIAN_POINT('Ctrl Pts',(-0.96457616008799,8.07052281559028,-0.0454356937116414));
#19741=CARTESIAN_POINT('Ctrl Pts',(-1.17280149874207,8.04290188438544,-0.0372139283516024));
#19742=CARTESIAN_POINT('Ctrl Pts',(-1.37962663999424,8.00726656835641,-0.0289921629915675));
#19743=CARTESIAN_POINT('Ctrl Pts',(-1.58649490085494,7.97162382295555,-0.0207686835299415));
#19744=CARTESIAN_POINT('Ctrl Pts',(-1.7919620904431,7.92796340490616,-0.0125452040683227));
#19745=CARTESIAN_POINT('Ctrl Pts',(-1.99540254448947,7.87642407745704,-0.00432172460669733));
#19746=CARTESIAN_POINT('Ctrl Pts',(-2.07760002171104,7.8556002805683,-0.000999134373119851));
#19747=CARTESIAN_POINT('Ctrl Pts',(-2.15946677537406,7.83349086257444,0.00232345586046502));
#19748=CARTESIAN_POINT('Ctrl Pts',(-2.24096214375505,7.81010731249941,0.00564604609404284));
#19749=CARTESIAN_POINT('Ctrl Pts',(-2.44266632606883,7.75223212350183,0.013869585168));
#19750=CARTESIAN_POINT('Ctrl Pts',(-2.64216004109066,7.68652952706406,0.022093124241958));
#19751=CARTESIAN_POINT('Ctrl Pts',(-2.83883268783922,7.61319358304749,0.0303166633159151));
#19752=CARTESIAN_POINT('Ctrl Pts',(-3.03546957608432,7.53987097277942,0.0385387072076221));
#19753=CARTESIAN_POINT('Ctrl Pts',(-3.22928614357328,7.45891788796716,0.0467607510993229));
#19754=CARTESIAN_POINT('Ctrl Pts',(-3.41968953236387,7.37057739018735,0.0549827949910302));
#19755=CARTESIAN_POINT('Ctrl Pts',(-3.61007189911896,7.28224664589508,0.0632039311042589));
#19756=CARTESIAN_POINT('Ctrl Pts',(-3.79704157208945,7.18653024108916,0.0714250672174895));
#19757=CARTESIAN_POINT('Ctrl Pts',(-3.98002740142911,7.08371861710878,0.0796462033307179));
#19758=CARTESIAN_POINT('Ctrl Pts',(-4.16302774430435,6.98089883861626,0.0878679915040102));
#19759=CARTESIAN_POINT('Ctrl Pts',(-4.34204335375989,6.87098285867043,0.0960897796773056));
#19760=CARTESIAN_POINT('Ctrl Pts',(-4.51652841258331,6.754306675065,0.104311567850598));
#19761=CARTESIAN_POINT('Ctrl Pts',(-4.69101298725775,6.63763081520452,0.112533333210645));
#19762=CARTESIAN_POINT('Ctrl Pts',(-4.86096679277625,6.51419495539005,0.120755098570688));
#19763=CARTESIAN_POINT('Ctrl Pts',(-5.0258732465123,6.38437825261724,0.128976863930735));
#19764=CARTESIAN_POINT('Ctrl Pts',(-5.19081408050607,6.2545344852172,0.137200343392356));
#19765=CARTESIAN_POINT('Ctrl Pts',(-5.35070522876196,6.11830739976473,0.14542382285398));
#19766=CARTESIAN_POINT('Ctrl Pts',(-5.50506257797969,5.97611693117091,0.153647302315601));
#19767=CARTESIAN_POINT('Ctrl Pts',(-5.56742866320986,5.91866671627553,0.156969892549181));
#19768=CARTESIAN_POINT('Ctrl Pts',(-5.6288917706135,5.86024344909845,0.160292482782762));
#19769=CARTESIAN_POINT('Ctrl Pts',(-5.68942161431893,5.80087659384515,0.163615073016341));
#19770=CARTESIAN_POINT('Ctrl Pts',(-5.83923531383011,5.65394133564222,0.171838612090299));
#19771=CARTESIAN_POINT('Ctrl Pts',(-5.98337817025907,5.50117546755519,0.18006215116426));
#19772=CARTESIAN_POINT('Ctrl Pts',(-6.12140564602634,5.34304037784638,0.188285690238217));
#19773=CARTESIAN_POINT('Ctrl Pts',(-6.259408026001,5.18493403984367,0.196507734129929));
#19774=CARTESIAN_POINT('Ctrl Pts',(-6.39129705065561,5.02146065072623,0.204729778021638));
#19775=CARTESIAN_POINT('Ctrl Pts',(-6.51666711727254,4.85311624063949,0.21295182191335));
#19776=CARTESIAN_POINT('Ctrl Pts',(-6.64202334204516,4.68479041710358,0.221172958026559));
#19777=CARTESIAN_POINT('Ctrl Pts',(-6.76086186963076,4.51159488274793,0.229394094139772));
#19778=CARTESIAN_POINT('Ctrl Pts',(-6.87281874659945,4.3340569953441,0.237615230252981));
#19779=CARTESIAN_POINT('Ctrl Pts',(-6.98478450343718,4.15650502650792,0.245837018426287));
#19780=CARTESIAN_POINT('Ctrl Pts',(-7.08986735949618,3.97461026451954,0.254058806599588));
#19781=CARTESIAN_POINT('Ctrl Pts',(-7.18774732974459,3.78892806559447,0.262280594772893));
#19782=CARTESIAN_POINT('Ctrl Pts',(-7.285627028402,3.60324638188835,0.270502360132912));
#19783=CARTESIAN_POINT('Ctrl Pts',(-7.37630374608216,3.41377754442737,0.278724125492935));
#19784=CARTESIAN_POINT('Ctrl Pts',(-7.45950375592395,3.22110094189184,0.286945890852955));
#19785=CARTESIAN_POINT('Ctrl Pts',(-7.54272111158676,3.0283841694829,0.29516937031458));
#19786=CARTESIAN_POINT('Ctrl Pts',(-7.61845852849534,2.83245856681313,0.303392849776207));
#19787=CARTESIAN_POINT('Ctrl Pts',(-7.68649024861327,2.63392392078306,0.311616329237832));
#19788=CARTESIAN_POINT('Ctrl Pts',(-7.713977582885,2.55370857167107,0.314938919471426));
#19789=CARTESIAN_POINT('Ctrl Pts',(-7.74020755077312,2.47306751200538,0.318261509705021));
#19790=CARTESIAN_POINT('Ctrl Pts',(-7.7651675494726,2.39204107220542,0.321584099938615));
#19791=CARTESIAN_POINT('Ctrl Pts',(-7.82717535069625,2.19074813812044,0.329838367786659));
#19792=CARTESIAN_POINT('Ctrl Pts',(-7.88136145535427,1.98701200604582,0.338092635634704));
#19793=CARTESIAN_POINT('Ctrl Pts',(-7.92755364808531,1.78145466381532,0.346346903482747));
#19794=CARTESIAN_POINT('Ctrl Pts',(-7.97373622309538,1.57594012087713,0.354599452701727));
#19795=CARTESIAN_POINT('Ctrl Pts',(-8.01192814537018,1.3686054079537,0.362852001920708));
#19796=CARTESIAN_POINT('Ctrl Pts',(-8.04200794311919,1.16008439576948,0.371104551139688));
#19797=CARTESIAN_POINT('Ctrl Pts',(-8.07208563879751,0.951577955688139,
0.379356523644623));
#19798=CARTESIAN_POINT('Ctrl Pts',(-8.09405229791888,0.741885668826661,
0.387608496149557));
#19799=CARTESIAN_POINT('Ctrl Pts',(-8.10783797364475,0.531649278777049,
0.395860468654494));
#19800=CARTESIAN_POINT('Ctrl Pts',(-8.11944417924312,0.354650572605817,
0.402807831365534));
#19801=CARTESIAN_POINT('Ctrl Pts',(-8.12525257630012,0.177266432657982,
0.409755194076573));
#19802=CARTESIAN_POINT('Ctrl Pts',(-8.12524999914245,-0.000118048941944703,
0.416702556787612));
#19803=CARTESIAN_POINT('Origin',(0.,0.,-16.4167025567876));
#19804=CARTESIAN_POINT('',(4.94673849251696,-6.44586330438811,-2.8749518510811));
#19805=CARTESIAN_POINT('',(4.94675008185376,-6.44587862049696,-2.70835307946025));
#19806=CARTESIAN_POINT('',(4.94675008185374,-6.44587862049697,-16.4167025567876));
#19807=CARTESIAN_POINT('',(-8.12527573348029,9.06015700713918E-5,-1.41670255634212));
#19808=CARTESIAN_POINT('Ctrl Pts',(4.94675008185376,-6.44587862049696,-2.70835307946025));
#19809=CARTESIAN_POINT('Ctrl Pts',(5.06306175751159,-6.35661774157638,-2.70260855423116));
#19810=CARTESIAN_POINT('Ctrl Pts',(5.17694645893466,-6.2642158434986,-2.69686402900206));
#19811=CARTESIAN_POINT('Ctrl Pts',(5.28823612645863,-6.16881238435064,-2.69111950377297));
#19812=CARTESIAN_POINT('Ctrl Pts',(5.44755215222471,-6.0322381605799,-2.682895964699));
#19813=CARTESIAN_POINT('Ctrl Pts',(5.60160046959401,-5.8894667018507,-2.67467242562504));
#19814=CARTESIAN_POINT('Ctrl Pts',(5.74990664483424,-5.7409285954618,-2.66644888655107));
#19815=CARTESIAN_POINT('Ctrl Pts',(5.89818585543617,-5.59241749588032,-2.65822684265933));
#19816=CARTESIAN_POINT('Ctrl Pts',(6.04072479937175,-5.43814204988859,-2.65000479876759));
#19817=CARTESIAN_POINT('Ctrl Pts',(6.17708557082848,-5.27857001593827,-2.64178275487584));
#19818=CARTESIAN_POINT('Ctrl Pts',(6.31343128697988,-5.11901559999985,-2.63356161876263));
#19819=CARTESIAN_POINT('Ctrl Pts',(6.44360000094805,-4.95416598773666,-2.62534048264943));
#19820=CARTESIAN_POINT('Ctrl Pts',(6.56719326509157,-4.78452298368771,-2.61711934653622));
#19821=CARTESIAN_POINT('Ctrl Pts',(6.69079633204521,-4.61486652438965,-2.60889755836291));
#19822=CARTESIAN_POINT('Ctrl Pts',(6.80782273128667,-4.44041615048072,-2.6006757701896));
#19823=CARTESIAN_POINT('Ctrl Pts',(6.91791601016778,-4.2617045461604,-2.59245398201628));
#19824=CARTESIAN_POINT('Ctrl Pts',(7.02800898356961,-4.08299343771681,-2.58423221665623));
#19825=CARTESIAN_POINT('Ctrl Pts',(7.13116872269657,-3.9000213750359,-2.57601045129617));
#19826=CARTESIAN_POINT('Ctrl Pts',(7.22708332008315,-3.71334811821837,-2.56778868593612));
#19827=CARTESIAN_POINT('Ctrl Pts',(7.32301791407054,-3.52663594312667,-2.55956520647452));
#19828=CARTESIAN_POINT('Ctrl Pts',(7.41170421397583,-3.33622129476586,-2.55134172701291));
#19829=CARTESIAN_POINT('Ctrl Pts',(7.49287680767403,-3.14268749759192,-2.54311824755131));
#19830=CARTESIAN_POINT('Ctrl Pts',(7.52567354150333,-3.06449267660979,-2.53979565731777));
#19831=CARTESIAN_POINT('Ctrl Pts',(7.5572442356429,-2.98578890928741,-2.53647306708422));
#19832=CARTESIAN_POINT('Ctrl Pts',(7.58757361511294,-2.90661559167049,-2.53315047685068));
#19833=CARTESIAN_POINT('Ctrl Pts',(7.66263999996019,-2.7106585746225,-2.52492693777672));
#19834=CARTESIAN_POINT('Ctrl Pts',(7.73012332902734,-2.51176017390019,-2.51670339870277));
#19835=CARTESIAN_POINT('Ctrl Pts',(7.78981142829103,-2.31052493476405,-2.50847985962881));
#19836=CARTESIAN_POINT('Ctrl Pts',(7.84948867522159,-2.10932628368951,-2.50025781573709));
#19837=CARTESIAN_POINT('Ctrl Pts',(7.90137343730657,-1.9057919248274,-2.49203577184536));
#19838=CARTESIAN_POINT('Ctrl Pts',(7.94530336095335,-1.70054169749622,-2.48381372795363));
#19839=CARTESIAN_POINT('Ctrl Pts',(7.98922843438995,-1.49531413140961,-2.47559259184043));
#19840=CARTESIAN_POINT('Ctrl Pts',(8.0252003611327,-1.28837136336534,-2.46737145572723));
#19841=CARTESIAN_POINT('Ctrl Pts',(8.05310769676512,-1.08034438342702,-2.45915031961402));
#19842=CARTESIAN_POINT('Ctrl Pts',(8.08101724587018,-0.872300903811568,
-2.45092853144073));
#19843=CARTESIAN_POINT('Ctrl Pts',(8.10086088395555,-0.663173332449556,
-2.44270674326743));
#19844=CARTESIAN_POINT('Ctrl Pts',(8.112578798865,-0.453599817797638,-2.43448495509413));
#19845=CARTESIAN_POINT('Ctrl Pts',(8.12429668126033,-0.244026884656978,
-2.42626318973413));
#19846=CARTESIAN_POINT('Ctrl Pts',(8.12788887180866,-0.0340083053242616,
-2.41804142437413));
#19847=CARTESIAN_POINT('Ctrl Pts',(8.12334762198528,0.175815172514029,-2.40981965901413));
#19848=CARTESIAN_POINT('Ctrl Pts',(8.11880542538668,0.385682395064902,-2.40159617955251));
#19849=CARTESIAN_POINT('Ctrl Pts',(8.10612640730235,0.595354139946849,-2.39337270009089));
#19850=CARTESIAN_POINT('Ctrl Pts',(8.08535492570326,0.80419107673868,-2.38514922062928));
#19851=CARTESIAN_POINT('Ctrl Pts',(8.07696247792963,0.88856893283274,-2.38182663039565));
#19852=CARTESIAN_POINT('Ctrl Pts',(8.06724956050654,0.972810555292713,-2.37850404016202));
#19853=CARTESIAN_POINT('Ctrl Pts',(8.05622149971848,1.05687402748562,-2.37518144992839));
#19854=CARTESIAN_POINT('Ctrl Pts',(8.02892662360567,1.26493436585477,-2.36695791085444));
#19855=CARTESIAN_POINT('Ctrl Pts',(7.99356294389417,1.47197055512868,-2.35873437178049));
#19856=CARTESIAN_POINT('Ctrl Pts',(7.95023173849494,1.67734995356596,-2.35051083270654));
#19857=CARTESIAN_POINT('Ctrl Pts',(7.90690841146144,1.88269201046153,-2.34228878881483));
#19858=CARTESIAN_POINT('Ctrl Pts',(7.85562051090432,2.0863775893089,-2.33406674492311));
#19859=CARTESIAN_POINT('Ctrl Pts',(7.79652040726645,2.28778432147304,-2.32584470103139));
#19860=CARTESIAN_POINT('Ctrl Pts',(7.73742682874643,2.48916881674446,-2.31762356491821));
#19861=CARTESIAN_POINT('Ctrl Pts',(7.67052285216363,2.68827468475593,-2.30940242880502));
#19862=CARTESIAN_POINT('Ctrl Pts',(7.5960109250455,2.88449399186225,-2.30118129269183));
#19863=CARTESIAN_POINT('Ctrl Pts',(7.52149308800743,3.08072886211985,-2.29295950451853));
#19864=CARTESIAN_POINT('Ctrl Pts',(7.43936619696353,3.27407643734074,-2.28473771634522));
#19865=CARTESIAN_POINT('Ctrl Pts',(7.34988151140998,3.46394707389327,-2.27651592817192));
#19866=CARTESIAN_POINT('Ctrl Pts',(7.26039707415217,3.65381718360626,-2.26829416281184));
#19867=CARTESIAN_POINT('Ctrl Pts',(7.16355501139801,3.84021010831143,-2.26007239745177));
#19868=CARTESIAN_POINT('Ctrl Pts',(7.05965360308662,4.02255870894709,-2.2518506320917));
#19869=CARTESIAN_POINT('Ctrl Pts',(6.95573053305696,4.20494532623794,-2.24362715263008));
#19870=CARTESIAN_POINT('Ctrl Pts',(6.84474532336131,4.38328567873918,-2.23540367316846));
#19871=CARTESIAN_POINT('Ctrl Pts',(6.72704139961008,4.55703868432473,-2.22718019370684));
#19872=CARTESIAN_POINT('Ctrl Pts',(6.67948465561444,4.62724133298553,-2.22385760347326));
#19873=CARTESIAN_POINT('Ctrl Pts',(6.63083160793803,4.69669543776809,-2.22053501323968));
#19874=CARTESIAN_POINT('Ctrl Pts',(6.58110689903192,4.76536667487555,-2.2172124230061));
#19875=CARTESIAN_POINT('Ctrl Pts',(6.45803632520719,4.93533063729968,-2.20898888393214));
#19876=CARTESIAN_POINT('Ctrl Pts',(6.3283579981927,5.10055201913228,-2.20076534485817));
#19877=CARTESIAN_POINT('Ctrl Pts',(6.19246221203539,5.26052272260217,-2.19254180578421));
#19878=CARTESIAN_POINT('Ctrl Pts',(6.05659113409252,5.42046434061946,-2.18431976189249));
#19879=CARTESIAN_POINT('Ctrl Pts',(5.91450504409466,5.57515696100924,-2.17609771800078));
#19880=CARTESIAN_POINT('Ctrl Pts',(5.76663427338612,5.72412584763023,-2.16787567410906));
#19881=CARTESIAN_POINT('Ctrl Pts',(5.61877982877697,5.87307828691117,-2.15965453799584));
#19882=CARTESIAN_POINT('Ctrl Pts',(5.46514218624349,6.01630804483998,-2.15143340188261));
#19883=CARTESIAN_POINT('Ctrl Pts',(5.30618883978909,6.15337692320223,-2.14321226576939));
#19884=CARTESIAN_POINT('Ctrl Pts',(5.14722288593736,6.29045667319348,-2.13499047759611));
#19885=CARTESIAN_POINT('Ctrl Pts',(4.98294060737273,6.42137437262999,-2.12676868942282));
#19886=CARTESIAN_POINT('Ctrl Pts',(4.81384371268235,6.54573114879985,-2.11854690124953));
#19887=CARTESIAN_POINT('Ctrl Pts',(4.64474728719106,6.6700875799126,-2.11032513588953));
#19888=CARTESIAN_POINT('Ctrl Pts',(4.47083651149325,6.78788295161319,-2.10210337052952));
#19889=CARTESIAN_POINT('Ctrl Pts',(4.29264372658684,6.8987605697759,-2.09388160516952));
#19890=CARTESIAN_POINT('Ctrl Pts',(4.11441379144225,7.00966130408175,-2.0856581257079));
#19891=CARTESIAN_POINT('Ctrl Pts',(3.93190031413309,7.11364124783058,-2.07743464624627));
#19892=CARTESIAN_POINT('Ctrl Pts',(3.74566292799559,7.21038811662309,-2.06921116678465));
#19893=CARTESIAN_POINT('Ctrl Pts',(3.67041612727074,7.24947743433618,-2.06588857655103));
#19894=CARTESIAN_POINT('Ctrl Pts',(3.59456169918358,7.28738650263208,-2.06256598631742));
#19895=CARTESIAN_POINT('Ctrl Pts',(3.51813765675159,7.32409687201408,-2.05924339608381));
#19896=CARTESIAN_POINT('Ctrl Pts',(3.32898520190726,7.41495645318615,-2.05101985700985));
#19897=CARTESIAN_POINT('Ctrl Pts',(3.13628032799971,7.4984992870151,-2.0427963179359));
#19898=CARTESIAN_POINT('Ctrl Pts',(2.94060817712988,7.574464410841,-2.03457277886194));
#19899=CARTESIAN_POINT('Ctrl Pts',(2.74497160285539,7.65041572288807,-2.0263507349702));
#19900=CARTESIAN_POINT('Ctrl Pts',(2.54636910320972,7.71879196809515,-2.01812869107846));
#19901=CARTESIAN_POINT('Ctrl Pts',(2.34540514236945,7.77938058463827,-2.00990664718673));
#19902=CARTESIAN_POINT('Ctrl Pts',(2.14446336953325,7.83996251172094,-2.0016855110734));
#19903=CARTESIAN_POINT('Ctrl Pts',(1.94116093829837,7.89275844162801,-1.99346437496007));
#19904=CARTESIAN_POINT('Ctrl Pts',(1.73611759466528,7.93760563772185,-1.98524323884674));
#19905=CARTESIAN_POINT('Ctrl Pts',(1.53105798800579,7.98245639087401,-1.97702145067345));
#19906=CARTESIAN_POINT('Ctrl Pts',(1.32425748061597,8.01935708489814,-1.96879966250016));
#19907=CARTESIAN_POINT('Ctrl Pts',(1.11634718058141,8.04819585589888,-1.96057787432687));
#19908=CARTESIAN_POINT('Ctrl Pts',(0.908437457442484,8.07703454687973,-1.95235610896685));
#19909=CARTESIAN_POINT('Ctrl Pts',(0.699418240324269,8.09781132173404,-1.94413434360683));
#19910=CARTESIAN_POINT('Ctrl Pts',(0.48992749086497,8.11046599254289,-1.93591257824681));
#19911=CARTESIAN_POINT('Ctrl Pts',(0.280393066061586,8.12312330164056,-1.92768909878518));
#19912=CARTESIAN_POINT('Ctrl Pts',(0.0703872069775901,8.12765510613058,
-1.91946561932356));
#19913=CARTESIAN_POINT('Ctrl Pts',(-0.139449270694467,8.1240532656675,-1.91124213986193));
#19914=CARTESIAN_POINT('Ctrl Pts',(-0.224230978314887,8.12259798873747,
-1.90791954962846));
#19915=CARTESIAN_POINT('Ctrl Pts',(-0.308985031865068,8.11981552118424,
-1.90459695939499));
#19916=CARTESIAN_POINT('Ctrl Pts',(-0.393669219340797,8.11570773920818,
-1.90127436916152));
#19917=CARTESIAN_POINT('Ctrl Pts',(-0.603265852003794,8.10554082026428,
-1.89305083008756));
#19918=CARTESIAN_POINT('Ctrl Pts',(-0.812502460733349,8.08724833330016,
-1.88482729101359));
#19919=CARTESIAN_POINT('Ctrl Pts',(-1.02074023536371,8.06087941445656,-1.87660375193962));
#19920=CARTESIAN_POINT('Ctrl Pts',(-1.22894014874827,8.03451528994061,-1.86838170804795));
#19921=CARTESIAN_POINT('Ctrl Pts',(-1.43614129804398,8.00007770140785,-1.86015966415628));
#19922=CARTESIAN_POINT('Ctrl Pts',(-1.64171092815941,7.95766754714357,-1.85193762026462));
#19923=CARTESIAN_POINT('Ctrl Pts',(-1.84725786176637,7.91526207529481,-1.84371648415144));
#19924=CARTESIAN_POINT('Ctrl Pts',(-2.05117334708184,7.86488585463802,-1.83549534803826));
#19925=CARTESIAN_POINT('Ctrl Pts',(-2.25283491514321,7.80669087434693,-1.82727421192509));
#19926=CARTESIAN_POINT('Ctrl Pts',(-2.45451247800942,7.74849127831592,-1.81905242375178));
#19927=CARTESIAN_POINT('Ctrl Pts',(-2.65393548230901,7.68247176277367,-1.81083063557848));
#19928=CARTESIAN_POINT('Ctrl Pts',(-2.8504956908767,7.60883446257003,-1.80260884740517));
#19929=CARTESIAN_POINT('Ctrl Pts',(-3.0470553540411,7.53519736669069,-1.79438708204519));
#19930=CARTESIAN_POINT('Ctrl Pts',(-3.24075196212233,7.45394263442523,-1.7861653166852));
#19931=CARTESIAN_POINT('Ctrl Pts',(-3.43099585684955,7.36532110588406,-1.77794355132522));
#19932=CARTESIAN_POINT('Ctrl Pts',(-3.62127941427141,7.27668110122501,-1.76972007186361));
#19933=CARTESIAN_POINT('Ctrl Pts',(-3.80810855292187,7.18067135665459,-1.76149659240199));
#19934=CARTESIAN_POINT('Ctrl Pts',(-3.99091588737073,7.0775898399407,-1.75327311294038));
#19935=CARTESIAN_POINT('Ctrl Pts',(-4.06477682019452,7.03594108988189,-1.74995052270666));
#19936=CARTESIAN_POINT('Ctrl Pts',(-4.13798148974316,6.99313842552292,-1.74662793247295));
#19937=CARTESIAN_POINT('Ctrl Pts',(-4.2104936697147,6.94920359608152,-1.74330534223923));
#19938=CARTESIAN_POINT('Ctrl Pts',(-4.38996411397347,6.84046319741505,-1.73508180316526));
#19939=CARTESIAN_POINT('Ctrl Pts',(-4.56524895597131,6.72474890409797,-1.72685826409128));
#19940=CARTESIAN_POINT('Ctrl Pts',(-4.73580984621355,6.60240809576376,-1.7186347250173));
#19941=CARTESIAN_POINT('Ctrl Pts',(-4.90633972552256,6.48008953111408,-1.71041268112561));
#19942=CARTESIAN_POINT('Ctrl Pts',(-5.07214712779607,6.3511470279392,-1.70219063723391));
#19943=CARTESIAN_POINT('Ctrl Pts',(-5.23272367482728,6.21597060042935,-1.69396859334222));
#19944=CARTESIAN_POINT('Ctrl Pts',(-5.39328249294177,6.0808090974628,-1.68574745722899));
#19945=CARTESIAN_POINT('Ctrl Pts',(-5.54861138328381,5.93941523414199,-1.67752632111576));
#19946=CARTESIAN_POINT('Ctrl Pts',(-5.69823533994547,5.79221905430868,-1.66930518500253));
#19947=CARTESIAN_POINT('Ctrl Pts',(-5.84787116404307,5.64501119959874,-1.66108339682924));
#19948=CARTESIAN_POINT('Ctrl Pts',(-5.99180093823563,5.49200031378658,-1.65286160865596));
#19949=CARTESIAN_POINT('Ctrl Pts',(-6.1295860485223,5.33365376044046,-1.64463982048267));
#19950=CARTESIAN_POINT('Ctrl Pts',(-6.26737077649119,5.17530764646479,-1.6364180551227));
#19951=CARTESIAN_POINT('Ctrl Pts',(-6.39901068309201,5.01162611883369,-1.62819628976273));
#19952=CARTESIAN_POINT('Ctrl Pts',(-6.52410668304801,4.84311052431268,-1.61997452440276));
#19953=CARTESIAN_POINT('Ctrl Pts',(-6.64922876344443,4.6745597970862,-1.61175104494113));
#19954=CARTESIAN_POINT('Ctrl Pts',(-6.76780403589574,4.50117322648551,-1.6035275654795));
#19955=CARTESIAN_POINT('Ctrl Pts',(-6.87947544098783,4.32348299630579,-1.59530408601787));
#19956=CARTESIAN_POINT('Ctrl Pts',(-6.92459482405033,4.25168956310478,-1.59198149578423));
#19957=CARTESIAN_POINT('Ctrl Pts',(-6.96858767436257,4.17919390226202,-1.58865890555058));
#19958=CARTESIAN_POINT('Ctrl Pts',(-7.0114324918152,4.1060323884765,-1.58533631531694));
#19959=CARTESIAN_POINT('Ctrl Pts',(-7.11747506873956,3.92495481796101,-1.57711277624297));
#19960=CARTESIAN_POINT('Ctrl Pts',(-7.21651634503643,3.73973765055601,-1.56888923716899));
#19961=CARTESIAN_POINT('Ctrl Pts',(-7.30824832199898,3.55094269546822,-1.56066569809502));
#19962=CARTESIAN_POINT('Ctrl Pts',(-7.39996362049496,3.36218206658217,-1.55244365420328));
#19963=CARTESIAN_POINT('Ctrl Pts',(-7.48437214327375,3.16984521349217,-1.54422161031153));
#19964=CARTESIAN_POINT('Ctrl Pts',(-7.56121254781631,2.97451716573382,-1.53599956641978));
#19965=CARTESIAN_POINT('Ctrl Pts',(-7.63804446857178,2.77921068373347,-1.52777843030657));
#19966=CARTESIAN_POINT('Ctrl Pts',(-7.70730983136704,2.58091394075382,-1.51955729419336));
#19967=CARTESIAN_POINT('Ctrl Pts',(-7.76879570026032,2.38023127660249,-1.51133615808014));
#19968=CARTESIAN_POINT('Ctrl Pts',(-7.83028644591053,2.17953269528856,-1.50311436990682));
#19969=CARTESIAN_POINT('Ctrl Pts',(-7.88399637583863,1.97644809591272,-1.49489258173349));
#19970=CARTESIAN_POINT('Ctrl Pts',(-7.92976232567285,1.77159730775352,-1.48667079356017));
#19971=CARTESIAN_POINT('Ctrl Pts',(-7.97552814851867,1.56674708800103,-1.47844902820013));
#19972=CARTESIAN_POINT('Ctrl Pts',(-8.01334997368914,1.36013097769249,-1.4702272628401));
#19973=CARTESIAN_POINT('Ctrl Pts',(-8.043115578085,1.15237986795429,-1.46200549748006));
#19974=CARTESIAN_POINT('Ctrl Pts',(-8.0728873881153,0.944585445558167,-1.45378201801842));
#19975=CARTESIAN_POINT('Ctrl Pts',(-8.09459958019832,0.735655843020287,
-1.44555853855677));
#19976=CARTESIAN_POINT('Ctrl Pts',(-8.10819157034168,0.526229057673656,
-1.43733505909513));
#19977=CARTESIAN_POINT('Ctrl Pts',(-8.11368323769669,0.441612880923745,
-1.43401246886163));
#19978=CARTESIAN_POINT('Ctrl Pts',(-8.11784990668612,0.356915592959289,
-1.43068987862813));
#19979=CARTESIAN_POINT('Ctrl Pts',(-8.12068999082585,0.272179417665621,
-1.42736728839464));
#19980=CARTESIAN_POINT('Ctrl Pts',(-8.12372865774564,0.181518366758098,
-1.42381237785896));
#19981=CARTESIAN_POINT('Ctrl Pts',(-8.125248987835,0.0908062923927736,-1.42025746732329));
#19982=CARTESIAN_POINT('Ctrl Pts',(-8.12524999949474,9.06126520568907E-5,
-1.41670255678761));
#19983=CARTESIAN_POINT('Ctrl Pts',(-8.12584796001076,9.03551486182587E-5,
-1.41670254643617));
#19984=CARTESIAN_POINT('Ctrl Pts',(-8.12513209299635,-1.25299245336929,
-1.3676011181149));
#19985=CARTESIAN_POINT('Ctrl Pts',(-7.51481976840467,-3.850553756064,-1.2658433474862));
#19986=CARTESIAN_POINT('Ctrl Pts',(-4.8622676215541,-6.9309500637499,-1.11142923455007));
#19987=CARTESIAN_POINT('Ctrl Pts',(-0.975506354015658,-8.41000015238307,
-0.953460207627781));
#19988=CARTESIAN_POINT('Ctrl Pts',(2.5305352297047,-7.94214230500563,-0.819100913414416));
#19989=CARTESIAN_POINT('Ctrl Pts',(4.35790031294788,-6.89669607699888,-0.737397961508479));
#19990=CARTESIAN_POINT('Ctrl Pts',(4.94635340024336,-6.44536135766213,-0.708351351909972));
#19991=CARTESIAN_POINT('',(-8.12528566984828,-7.93977388155583E-5,-1.58329744376396));
#19992=CARTESIAN_POINT('Ctrl Pts',(-8.12524999961194,-7.94114662834033E-5,
-1.58329744321239));
#19993=CARTESIAN_POINT('Ctrl Pts',(-8.12524923036167,-0.078787827428694,
-1.58021303651788));
#19994=CARTESIAN_POINT('Ctrl Pts',(-8.12410474332392,-0.157493831703078,
-1.57712862982337));
#19995=CARTESIAN_POINT('Ctrl Pts',(-8.12181709581716,-0.236166518778639,
-1.57404422312885));
#19996=CARTESIAN_POINT('Ctrl Pts',(-8.11571784869364,-0.445920931959764,
-1.56582068405489));
#19997=CARTESIAN_POINT('Ctrl Pts',(-8.10148757870039,-0.655473008847223,
-1.55759714498093));
#19998=CARTESIAN_POINT('Ctrl Pts',(-8.07916302108297,-0.86418310632966,
-1.54937360590697));
#19999=CARTESIAN_POINT('Ctrl Pts',(-8.056842522458,-1.07285525669011,-1.54115156201529));
#20000=CARTESIAN_POINT('Ctrl Pts',(-8.02643070487113,-1.28068544007206,
-1.53292951812361));
#20001=CARTESIAN_POINT('Ctrl Pts',(-7.98801617342936,-1.48703906321621,
-1.52470747423194));
#20002=CARTESIAN_POINT('Ctrl Pts',(-7.94960588325472,-1.6933699032935,-1.51648633811873));
#20003=CARTESIAN_POINT('Ctrl Pts',(-7.90319469718185,-1.89822421876373,
-1.50826520200552));
#20004=CARTESIAN_POINT('Ctrl Pts',(-7.84892250112346,-2.10097670949914,
-1.50004406589231));
#20005=CARTESIAN_POINT('Ctrl Pts',(-7.79464600046137,-2.30374528156509,
-1.49182227771901));
#20006=CARTESIAN_POINT('Ctrl Pts',(-7.73250731771493,-2.5044114102037,-1.4836004895457));
#20007=CARTESIAN_POINT('Ctrl Pts',(-7.66269675110625,-2.70236305168009,
-1.4753787013724));
#20008=CARTESIAN_POINT('Ctrl Pts',(-7.59288637820341,-2.90031414389308,
-1.46715693601239));
#20009=CARTESIAN_POINT('Ctrl Pts',(-7.51540426465473,-3.09555048676511,
-1.45893517065238));
#20010=CARTESIAN_POINT('Ctrl Pts',(-7.43048976517222,-3.28747766717448,
-1.45071340529236));
#20011=CARTESIAN_POINT('Ctrl Pts',(-7.34555756242592,-3.47944486121545,
-1.44248992583073));
#20012=CARTESIAN_POINT('Ctrl Pts',(-7.25318999758232,-3.66810124479795,
-1.4342664463691));
#20013=CARTESIAN_POINT('Ctrl Pts',(-7.15367397619229,-3.85287375926712,
-1.42604296690747));
#20014=CARTESIAN_POINT('Ctrl Pts',(-7.1134658182826,-3.92752869759137,-1.42272037667384));
#20015=CARTESIAN_POINT('Ctrl Pts',(-7.07209123298693,-4.00154987977049,
-1.4193977864402));
#20016=CARTESIAN_POINT('Ctrl Pts',(-7.02957126271235,-4.07490066442714,
-1.41607519620657));
#20017=CARTESIAN_POINT('Ctrl Pts',(-6.92433269509206,-4.25644668765432,
-1.40785165713262));
#20018=CARTESIAN_POINT('Ctrl Pts',(-6.81204035264438,-4.43394317589982,
-1.39962811805866));
#20019=CARTESIAN_POINT('Ctrl Pts',(-6.69303110672799,-4.60684514248867,
-1.3914045789847));
#20020=CARTESIAN_POINT('Ctrl Pts',(-6.5740434987594,-4.77971567249713,-1.38318253509297));
#20021=CARTESIAN_POINT('Ctrl Pts',(-6.44834159193582,-4.94799310531268,
-1.37496049120124));
#20022=CARTESIAN_POINT('Ctrl Pts',(-6.31630546553415,-5.11116159288311,
-1.36673844730951));
#20023=CARTESIAN_POINT('Ctrl Pts',(-6.18428391696299,-5.27431206536463,
-1.35851731119632));
#20024=CARTESIAN_POINT('Ctrl Pts',(-6.04592973049139,-5.43235448955832,
-1.35029617508313));
#20025=CARTESIAN_POINT('Ctrl Pts',(-5.90166365487219,-5.58480560693572,
-1.34207503896994));
#20026=CARTESIAN_POINT('Ctrl Pts',(-5.75738613677688,-5.7372688159865,-1.33385325079664));
#20027=CARTESIAN_POINT('Ctrl Pts',(-5.60719599342608,-5.88413961606792,
-1.32563146262334));
#20028=CARTESIAN_POINT('Ctrl Pts',(-5.45155199220795,-6.0249704097824,-1.31740967445004));
#20029=CARTESIAN_POINT('Ctrl Pts',(-5.29590842286007,-6.1658008127293,-1.30918790908999));
#20030=CARTESIAN_POINT('Ctrl Pts',(-5.13481124642108,-6.30059104695188,
-1.30096614372994));
#20031=CARTESIAN_POINT('Ctrl Pts',(-4.96875397386089,-6.42893237713243,
-1.29274437836989));
#20032=CARTESIAN_POINT('Ctrl Pts',(-4.80266208111646,-6.55730046434943,
-1.28452089890827));
#20033=CARTESIAN_POINT('Ctrl Pts',(-4.63160825982146,-6.67921678123042,
-1.27629741944665));
#20034=CARTESIAN_POINT('Ctrl Pts',(-4.45611766739158,-6.79431401223557,
-1.26807393998502));
#20035=CARTESIAN_POINT('Ctrl Pts',(-4.38521296929947,-6.84081755583104,
-1.26475134975144));
#20036=CARTESIAN_POINT('Ctrl Pts',(-4.31358432319599,-6.88620840046679,
-1.26142875951786));
#20037=CARTESIAN_POINT('Ctrl Pts',(-4.24126767987644,-6.93046434448194,
-1.25810616928428));
#20038=CARTESIAN_POINT('Ctrl Pts',(-4.06228119637158,-7.03999951411719,
-1.24988263021032));
#20039=CARTESIAN_POINT('Ctrl Pts',(-3.87902008353936,-7.14261500045062,
-1.24165909113635));
#20040=CARTESIAN_POINT('Ctrl Pts',(-3.6920400703131,-7.23799196474426,-1.23343555206239));
#20041=CARTESIAN_POINT('Ctrl Pts',(-3.50509405330119,-7.33335158784903,
-1.22521350817067));
#20042=CARTESIAN_POINT('Ctrl Pts',(-3.3144307480331,-7.42147518172794,-1.21699146427896));
#20043=CARTESIAN_POINT('Ctrl Pts',(-3.12063000443933,-7.50209010462371,
-1.20876942038725));
#20044=CARTESIAN_POINT('Ctrl Pts',(-2.92685065797582,-7.58269612699632,
-1.20054828427402));
#20045=CARTESIAN_POINT('Ctrl Pts',(-2.72993483696624,-7.6557950202564,-1.19232714816078));
#20046=CARTESIAN_POINT('Ctrl Pts',(-2.5304826369713,-7.72116216553485,-1.18410601204754));
#20047=CARTESIAN_POINT('Ctrl Pts',(-2.33101461740929,-7.7865344954136,-1.17588422387424));
#20048=CARTESIAN_POINT('Ctrl Pts',(-2.12901009634928,-7.84417375761885,
-1.16766243570095));
#20049=CARTESIAN_POINT('Ctrl Pts',(-1.92508562137813,-7.89390479502148,
-1.15944064752765));
#20050=CARTESIAN_POINT('Ctrl Pts',(-1.72116171224275,-7.94363569443381,
-1.15121888216761));
#20051=CARTESIAN_POINT('Ctrl Pts',(-1.51531814702637,-7.98545834568029,
-1.14299711680757));
#20052=CARTESIAN_POINT('Ctrl Pts',(-1.30818352124196,-8.01924830874135,
-1.13477535144753));
#20053=CARTESIAN_POINT('Ctrl Pts',(-1.10100571132674,-8.05304531644875,
-1.12655187198591));
#20054=CARTESIAN_POINT('Ctrl Pts',(-0.892536594266989,-8.07880624294275,
-1.11832839252428));
#20055=CARTESIAN_POINT('Ctrl Pts',(-0.683412872141368,-8.09645813974799,
-1.11010491306265));
#20056=CARTESIAN_POINT('Ctrl Pts',(-0.598919144154128,-8.10359015974056,
-1.1067823228291));
#20057=CARTESIAN_POINT('Ctrl Pts',(-0.514318617874732,-8.10939900407478,
-1.10345973259555));
#20058=CARTESIAN_POINT('Ctrl Pts',(-0.42965347846909,-8.11388226750545,
-1.10013714236199));
#20059=CARTESIAN_POINT('Ctrl Pts',(-0.220103990520467,-8.12497851754215,
-1.09191360328803));
#20060=CARTESIAN_POINT('Ctrl Pts',(-0.0100903786848266,-8.12795448052103,
-1.08369006421408));
#20061=CARTESIAN_POINT('Ctrl Pts',(0.199746853865668,-8.12279439336432,
-1.07546652514012));
#20062=CARTESIAN_POINT('Ctrl Pts',(0.409545934362378,-8.11763524440108,
-1.0672444812484));
#20063=CARTESIAN_POINT('Ctrl Pts',(0.61916840488007,-8.10434300501338,-1.05902243735669));
#20064=CARTESIAN_POINT('Ctrl Pts',(0.827974547956963,-8.08295402129911,
-1.05080039346498));
#20065=CARTESIAN_POINT('Ctrl Pts',(1.03675763718865,-8.06156739909736,-1.04257925735176));
#20066=CARTESIAN_POINT('Ctrl Pts',(1.24472428563353,-8.03208584733869,-1.03435812123855));
#20067=CARTESIAN_POINT('Ctrl Pts',(1.45123983880385,-7.99459758166529,-1.02613698512534));
#20068=CARTESIAN_POINT('Ctrl Pts',(1.65777177177236,-7.957106342607,-1.01791519695204));
#20069=CARTESIAN_POINT('Ctrl Pts',(1.86285208882459,-7.91160717081146,-1.00969340877873));
#20070=CARTESIAN_POINT('Ctrl Pts',(2.06585521951359,-7.85823961040311,-1.00147162060542));
#20071=CARTESIAN_POINT('Ctrl Pts',(2.268857786923,-7.80487219807552,-0.99324985524539));
#20072=CARTESIAN_POINT('Ctrl Pts',(2.46978289494403,-7.74363651840299,-0.985028089885358));
#20073=CARTESIAN_POINT('Ctrl Pts',(2.66801852771913,-7.67472245089342,-0.976806324525324));
#20074=CARTESIAN_POINT('Ctrl Pts',(2.86629548933278,-7.6057940159448,-0.968582845063701));
#20075=CARTESIAN_POINT('Ctrl Pts',(3.06188157693146,-7.52918409204903,-0.960359365602076));
#20076=CARTESIAN_POINT('Ctrl Pts',(3.25418216388124,-7.44513169841724,-0.952135886140454));
#20077=CARTESIAN_POINT('Ctrl Pts',(3.33187872226552,-7.41117141876996,-0.948813295906869));
#20078=CARTESIAN_POINT('Ctrl Pts',(3.40903916149606,-7.3759967355855,-0.945490705673285));
#20079=CARTESIAN_POINT('Ctrl Pts',(3.48562524024988,-7.33962562035918,-0.942168115439701));
#20080=CARTESIAN_POINT('Ctrl Pts',(3.67517718563534,-7.24960644508391,-0.93394464385397));
#20081=CARTESIAN_POINT('Ctrl Pts',(3.8612708249081,-7.15222571977221,-0.92572117226824));
#20082=CARTESIAN_POINT('Ctrl Pts',(4.04333543182722,-7.04777455288055,-0.91749770068251));
#20083=CARTESIAN_POINT('Ctrl Pts',(4.22537413651904,-6.94333824619654,-0.90927539904537));
#20084=CARTESIAN_POINT('Ctrl Pts',(4.4033846964227,-6.83183365095716,-0.901053097408225));
#20085=CARTESIAN_POINT('Ctrl Pts',(4.57682182311896,-6.71359736370316,-0.892830795771085));
#20086=CARTESIAN_POINT('Ctrl Pts',(4.70260229937768,-6.62784976856503,-0.886867799061196));
#20087=CARTESIAN_POINT('Ctrl Pts',(4.82597790270025,-6.53856261631617,-0.880904802351308));
#20088=CARTESIAN_POINT('Ctrl Pts',(4.94675008185375,-6.44587862049697,-0.874941805641418));
#20089=CARTESIAN_POINT('Ctrl Pts',(4.94673849251696,-6.44586330438811,-2.8749518510811));
#20090=CARTESIAN_POINT('Ctrl Pts',(5.19773710945893,-6.25365150213958,-2.86256671355646));
#20091=CARTESIAN_POINT('Ctrl Pts',(6.4568287000089,-5.16760485441946,-2.79752523372439));
#20092=CARTESIAN_POINT('Ctrl Pts',(8.08005480686637,-2.52832543946459,-2.67982741158489));
#20093=CARTESIAN_POINT('Ctrl Pts',(8.30916720919218,1.62402447626065,-2.5218583846626));
#20094=CARTESIAN_POINT('Ctrl Pts',(6.5334877241783,5.38453836162577,-2.36388935774031));
#20095=CARTESIAN_POINT('Ctrl Pts',(3.18144290005129,7.84589932917326,-2.20592033081802));
#20096=CARTESIAN_POINT('Ctrl Pts',(-0.938203628973559,8.41424323159183,
-2.04795130389573));
#20097=CARTESIAN_POINT('Ctrl Pts',(-4.83148535191313,6.95244306010894,-1.88998227697344));
#20098=CARTESIAN_POINT('Ctrl Pts',(-7.50579500816724,3.87448934127983,-1.73509765993017));
#20099=CARTESIAN_POINT('Ctrl Pts',(-8.12522203952541,1.26500204491867,-1.63286938519434));
#20100=CARTESIAN_POINT('Ctrl Pts',(-8.1258678326399,-7.91736970983551E-5,
-1.58329745276593));
#20101=CARTESIAN_POINT('Origin',(0.,0.,-16.4167025567876));
#20102=CARTESIAN_POINT('',(4.94675008185375,-6.44587862049697,-4.87493975109638));
#20103=CARTESIAN_POINT('',(4.94675083769988,-6.44587978308508,-4.70834087481909));
#20104=CARTESIAN_POINT('',(4.94675008185374,-6.44587862049697,-16.4167025567876));
#20105=CARTESIAN_POINT('',(-8.12522972379081,0.000108848713032344,-3.41670255712189));
#20106=CARTESIAN_POINT('Ctrl Pts',(4.94675083769988,-6.44587978308508,-4.70834087481909));
#20107=CARTESIAN_POINT('Ctrl Pts',(5.76684755869603,-5.81516257124187,-4.66780985882621));
#20108=CARTESIAN_POINT('Ctrl Pts',(7.3768399998997,-4.00454199459098,-4.5746225005259));
#20109=CARTESIAN_POINT('Ctrl Pts',(8.46029510168218,-0.321126146958935,
-4.42877879991817));
#20110=CARTESIAN_POINT('Ctrl Pts',(7.59257255154836,3.74600550710789,-4.27080977299587));
#20111=CARTESIAN_POINT('Ctrl Pts',(4.89295428043989,6.9093207784364,-4.11284074607359));
#20112=CARTESIAN_POINT('Ctrl Pts',(1.01278989687648,8.4055917004452,-3.95487171915129));
#20113=CARTESIAN_POINT('Ctrl Pts',(-3.11173507273836,7.87380594419866,-3.79690269222901));
#20114=CARTESIAN_POINT('Ctrl Pts',(-6.48547707309547,5.44226996244777,-3.63893366530671));
#20115=CARTESIAN_POINT('Ctrl Pts',(-7.93674675436804,2.43808555436179,-3.51220029005247));
#20116=CARTESIAN_POINT('Ctrl Pts',(-8.12492425771545,0.547001067506262,
-3.43812325710566));
#20117=CARTESIAN_POINT('Ctrl Pts',(-8.12466295576038,0.000109079692641577,
-3.41670256646628));
#20118=CARTESIAN_POINT('Ctrl Pts',(-8.12524999927102,0.000108840450000125,
-3.41670255678761));
#20119=CARTESIAN_POINT('Ctrl Pts',(-8.12525282338782,-0.210719532315853,
-3.40844541790656));
#20120=CARTESIAN_POINT('Ctrl Pts',(-8.11704565989559,-0.42154584143425,
-3.4001882790255));
#20121=CARTESIAN_POINT('Ctrl Pts',(-8.10065504422437,-0.631724162101,-3.39193114014445));
#20122=CARTESIAN_POINT('Ctrl Pts',(-8.08426436384872,-0.841903312478525,
-3.3836739686671));
#20123=CARTESIAN_POINT('Ctrl Pts',(-8.05969019230419,-1.05143418077564,
-3.37541679718974));
#20124=CARTESIAN_POINT('Ctrl Pts',(-8.02701101511336,-1.25967524614433,
-3.36715962571238));
#20125=CARTESIAN_POINT('Ctrl Pts',(-7.99432344888107,-1.46796976888498,
-3.35890033454415));
#20126=CARTESIAN_POINT('Ctrl Pts',(-7.95352676351121,-1.67497354070713,
-3.35064104337591));
#20127=CARTESIAN_POINT('Ctrl Pts',(-7.90475092986181,-1.8800532703487,-3.34238175220767));
#20128=CARTESIAN_POINT('Ctrl Pts',(-7.86658885045947,-2.04050709226893,
-3.33591970529249));
#20129=CARTESIAN_POINT('Ctrl Pts',(-7.82354340356189,-2.19978325012226,
-3.32945765837732));
#20130=CARTESIAN_POINT('Ctrl Pts',(-7.77569842141607,-2.35758385252523,
-3.32299561146214));
#20131=CARTESIAN_POINT('Ctrl Pts',(-7.71481135492858,-2.55839938927245,
-3.31477207238817));
#20132=CARTESIAN_POINT('Ctrl Pts',(-7.64613083549557,-2.75688757472043,
-3.3065485333142));
#20133=CARTESIAN_POINT('Ctrl Pts',(-7.56986003845332,-2.95244078022363,
-3.29832499424023));
#20134=CARTESIAN_POINT('Ctrl Pts',(-7.49360310876675,-3.14795843075743,
-3.2901029503485));
#20135=CARTESIAN_POINT('Ctrl Pts',(-7.40975876299778,-3.34054189177276,
-3.28188090645677));
#20136=CARTESIAN_POINT('Ctrl Pts',(-7.31857890719936,-3.52960200895179,
-3.27365886256504));
#20137=CARTESIAN_POINT('Ctrl Pts',(-7.22740911837657,-3.71864125240194,
-3.26543772645184));
#20138=CARTESIAN_POINT('Ctrl Pts',(-7.12890556452571,-3.90415766309951,
-3.25721659033864));
#20139=CARTESIAN_POINT('Ctrl Pts',(-7.02336720131108,-4.08558450139607,
-3.24899545422544));
#20140=CARTESIAN_POINT('Ctrl Pts',(-6.91782046731242,-4.26702572957735,
-3.24077366605215));
#20141=CARTESIAN_POINT('Ctrl Pts',(-6.80523795509613,-4.44437648096923,
-3.23255187787885));
#20142=CARTESIAN_POINT('Ctrl Pts',(-6.68596379259542,-4.61709602744009,
-3.22433008970556));
#20143=CARTESIAN_POINT('Ctrl Pts',(-6.56668996104819,-4.78981509466101,
-3.2161083243455));
#20144=CARTESIAN_POINT('Ctrl Pts',(-6.44072468616938,-4.95790274150987,
-3.20788655898544));
#20145=CARTESIAN_POINT('Ctrl Pts',(-6.30845481278701,-5.12084811701386,
-3.19966479362538));
#20146=CARTESIAN_POINT('Ctrl Pts',(-6.17615736333197,-5.28382746392345,
-3.19144131416374));
#20147=CARTESIAN_POINT('Ctrl Pts',(-6.03755287548238,-5.44166216875608,
-3.1832178347021));
#20148=CARTESIAN_POINT('Ctrl Pts',(-5.89306848153566,-5.59387445644171,
-3.17499435524046));
#20149=CARTESIAN_POINT('Ctrl Pts',(-5.8346914358501,-5.65537385737634,-3.17167176500692));
#20150=CARTESIAN_POINT('Ctrl Pts',(-5.77535495924955,-5.71595582056519,
-3.16834917477338));
#20151=CARTESIAN_POINT('Ctrl Pts',(-5.71508896584658,-5.77559050443837,
-3.16502658453984));
#20152=CARTESIAN_POINT('Ctrl Pts',(-5.56592830601656,-5.92318864881475,
-3.1568030454659));
#20153=CARTESIAN_POINT('Ctrl Pts',(-5.41102254924536,-6.06502933420128,
-3.14857950639195));
#20154=CARTESIAN_POINT('Ctrl Pts',(-5.25083968431792,-6.20067497713693,
-3.140355967318));
#20155=CARTESIAN_POINT('Ctrl Pts',(-5.09068594341744,-6.33629595733875,
-3.13213392342629));
#20156=CARTESIAN_POINT('Ctrl Pts',(-4.92525723431693,-6.46572395268463,
-3.12391187953457));
#20157=CARTESIAN_POINT('Ctrl Pts',(-4.75505560117337,-6.58856082860663,
-3.11568983564286));
#20158=CARTESIAN_POINT('Ctrl Pts',(-4.58487275963417,-6.71138414236751,
-3.10746869952971));
#20159=CARTESIAN_POINT('Ctrl Pts',(-4.40991828518714,-6.82761761701956,
-3.09924756341657));
#20160=CARTESIAN_POINT('Ctrl Pts',(-4.23072492285598,-6.93690523141446,
-3.09102642730343));
#20161=CARTESIAN_POINT('Ctrl Pts',(-4.05151734778677,-7.04620151396657,
-3.08280463913012));
#20162=CARTESIAN_POINT('Ctrl Pts',(-3.86807046348638,-7.14855067965373,
-3.07458285095681));
#20163=CARTESIAN_POINT('Ctrl Pts',(-3.68094435233206,-7.243641089779,-3.0663610627835));
#20164=CARTESIAN_POINT('Ctrl Pts',(-3.4938187604034,-7.33873123605344,-3.05813929742349));
#20165=CARTESIAN_POINT('Ctrl Pts',(-3.30301422619502,-7.42656253584763,
-3.04991753206347));
#20166=CARTESIAN_POINT('Ctrl Pts',(-3.10911416963784,-7.50686996308429,
-3.04169576670346));
#20167=CARTESIAN_POINT('Ctrl Pts',(-2.91517368813687,-7.58719413308674,
-3.03347228724182));
#20168=CARTESIAN_POINT('Ctrl Pts',(-2.71813666756841,-7.6599911840378,-3.02524880778018));
#20169=CARTESIAN_POINT('Ctrl Pts',(-2.51860620598059,-7.72504435855847,
-3.01702532831853));
#20170=CARTESIAN_POINT('Ctrl Pts',(-2.43798851050486,-7.75132825010818,
-3.01370273808487));
#20171=CARTESIAN_POINT('Ctrl Pts',(-2.35696396772518,-7.77634854561106,
-3.01038014785121));
#20172=CARTESIAN_POINT('Ctrl Pts',(-2.27557309213706,-7.80009324718889,
-3.00705755761755));
#20173=CARTESIAN_POINT('Ctrl Pts',(-2.07412753352353,-7.85886230009434,
-2.99883401854358));
#20174=CARTESIAN_POINT('Ctrl Pts',(-1.87037138055673,-7.90983291555254,
-2.99061047946961));
#20175=CARTESIAN_POINT('Ctrl Pts',(-1.66492452161307,-7.95284313310853,
-2.98238694039564));
#20176=CARTESIAN_POINT('Ctrl Pts',(-1.45951501647798,-7.99584553065967,
-2.97416489650396));
#20177=CARTESIAN_POINT('Ctrl Pts',(-1.25241570743435,-8.03089035862664,
-2.96594285261227));
#20178=CARTESIAN_POINT('Ctrl Pts',(-1.04425764618611,-8.05786656199281,
-2.95772080872059));
#20179=CARTESIAN_POINT('Ctrl Pts',(-0.836122567227863,-8.08483978697359,
-2.94949967260733));
#20180=CARTESIAN_POINT('Ctrl Pts',(-0.626929261815653,-8.10374612799193,
-2.94127853649407));
#20181=CARTESIAN_POINT('Ctrl Pts',(-0.417315726432918,-8.11452618129806,
-2.93305740038081));
#20182=CARTESIAN_POINT('Ctrl Pts',(-0.207685565536802,-8.12530708962494,
-2.92483561220752));
#20183=CARTESIAN_POINT('Ctrl Pts',(0.00236459750956827,-8.1279604046004,
-2.91661382403423));
#20184=CARTESIAN_POINT('Ctrl Pts',(0.212193859596608,-8.12247876749761,
-2.90839203586094));
#20185=CARTESIAN_POINT('Ctrl Pts',(0.42202253946395,-8.11699714560488,-2.9001702705009));
#20186=CARTESIAN_POINT('Ctrl Pts',(0.631630024836994,-8.10338062718437,
-2.89194850514086));
#20187=CARTESIAN_POINT('Ctrl Pts',(0.840377085155128,-8.08167395514359,
-2.88372673978081));
#20188=CARTESIAN_POINT('Ctrl Pts',(1.04916766576987,-8.05996275762204,-2.87550326031919));
#20189=CARTESIAN_POINT('Ctrl Pts',(1.25709716956753,-8.03015806752157,-2.86727978085756));
#20190=CARTESIAN_POINT('Ctrl Pts',(1.46353204505432,-7.99235644322744,-2.85905630139593));
#20191=CARTESIAN_POINT('Ctrl Pts',(1.54693937942639,-7.97708318714668,-2.85573371116237));
#20192=CARTESIAN_POINT('Ctrl Pts',(1.63010281552708,-7.96050505048469,-2.85241112092882));
#20193=CARTESIAN_POINT('Ctrl Pts',(1.71298101360102,-7.94263077383951,-2.84908853069526));
#20194=CARTESIAN_POINT('Ctrl Pts',(1.91810638711379,-7.89839154376067,-2.84086504637095));
#20195=CARTESIAN_POINT('Ctrl Pts',(2.12155038681738,-7.84619456950808,-2.83264156204664));
#20196=CARTESIAN_POINT('Ctrl Pts',(2.32269080051696,-7.78619258737503,-2.82441807772233));
#20197=CARTESIAN_POINT('Ctrl Pts',(2.52379415594392,-7.72620166005573,-2.81619610849943));
#20198=CARTESIAN_POINT('Ctrl Pts',(2.72259449000077,-7.65840867929775,-2.80797413927652));
#20199=CARTESIAN_POINT('Ctrl Pts',(2.91848401662767,-7.58301645832243,-2.79975217005362));
#20200=CARTESIAN_POINT('Ctrl Pts',(3.11437128332761,-7.50762510712772,-2.79153029568546));
#20201=CARTESIAN_POINT('Ctrl Pts',(3.30734753312896,-7.42463479330348,-2.7833084213173));
#20202=CARTESIAN_POINT('Ctrl Pts',(3.49682329234003,-7.33429713228529,-2.77508654694913));
#20203=CARTESIAN_POINT('Ctrl Pts',(3.68628594035273,-7.24396572238333,-2.76686524151193));
#20204=CARTESIAN_POINT('Ctrl Pts',(3.87224831595824,-7.14628810893926,-2.75864393607473));
#20205=CARTESIAN_POINT('Ctrl Pts',(4.05414342998451,-7.04156293812769,-2.75042263063753));
#20206=CARTESIAN_POINT('Ctrl Pts',(4.23606724799523,-6.93682124114557,-2.74220002783605));
#20207=CARTESIAN_POINT('Ctrl Pts',(4.41392226563831,-6.82502991067713,-2.73397742503457));
#20208=CARTESIAN_POINT('Ctrl Pts',(4.58716750850335,-6.70653277121876,-2.72575482223309));
#20209=CARTESIAN_POINT('Ctrl Pts',(4.70938222265734,-6.62293974558946,-2.71995424130881));
#20210=CARTESIAN_POINT('Ctrl Pts',(4.82930342435198,-6.53601051667679,-2.71415366038453));
#20211=CARTESIAN_POINT('Ctrl Pts',(4.94675008185376,-6.44587862049696,-2.70835307946025));
#20212=CARTESIAN_POINT('',(-8.12524999755206,0.000199449834196055,-3.58329744397444));
#20213=CARTESIAN_POINT('Ctrl Pts',(-8.12504666895516,0.00019942538992946,
-3.58329744321239));
#20214=CARTESIAN_POINT('Ctrl Pts',(-8.12413961048046,-0.966655941748394,
-3.54542247754037));
#20215=CARTESIAN_POINT('Ctrl Pts',(-7.71133025888803,-3.27845306278411,
-3.45489116956092));
#20216=CARTESIAN_POINT('Ctrl Pts',(-5.56705133684236,-6.37868753136333,
-3.31170351927405));
#20217=CARTESIAN_POINT('Ctrl Pts',(-1.85822808956723,-8.25994573692536,
-3.15373449235176));
#20218=CARTESIAN_POINT('Ctrl Pts',(1.97300710128673,-8.15704218041728,-3.00815060295411));
#20219=CARTESIAN_POINT('Ctrl Pts',(4.13059763958269,-7.07085441446827,-2.91522305586389));
#20220=CARTESIAN_POINT('Ctrl Pts',(4.94673849251696,-6.44586330438811,-2.8749518510811));
#20221=CARTESIAN_POINT('Ctrl Pts',(4.94675008185375,-6.44587862049697,-4.87493975109638));
#20222=CARTESIAN_POINT('Ctrl Pts',(5.1132324741457,-6.31811531060797,-4.86671727446932));
#20223=CARTESIAN_POINT('Ctrl Pts',(5.27478384445414,-6.18388235747323,-4.85849479784226));
#20224=CARTESIAN_POINT('Ctrl Pts',(5.43090817343691,-6.04358535756683,-4.8502723212152));
#20225=CARTESIAN_POINT('Ctrl Pts',(5.58701155230035,-5.90330718393119,-4.84205094795152));
#20226=CARTESIAN_POINT('Ctrl Pts',(5.73768912429145,-5.75696678494614,-4.83382957468783));
#20227=CARTESIAN_POINT('Ctrl Pts',(5.88247945748213,-5.60500874172385,-4.82560820142415));
#20228=CARTESIAN_POINT('Ctrl Pts',(6.02727953633488,-5.4530404703896,-4.81738627478978));
#20229=CARTESIAN_POINT('Ctrl Pts',(6.16619137864326,-5.29545401045529,-4.80916434815541));
#20230=CARTESIAN_POINT('Ctrl Pts',(6.29879106094806,-5.13273014418456,-4.80094242152104));
#20231=CARTESIAN_POINT('Ctrl Pts',(6.43138720887069,-4.97001061524195,-4.79272071403826));
#20232=CARTESIAN_POINT('Ctrl Pts',(6.55767134834218,-4.80215418362125,-4.78449900655548));
#20233=CARTESIAN_POINT('Ctrl Pts',(6.67726011485629,-4.6296743860718,-4.7762772990727));
#20234=CARTESIAN_POINT('Ctrl Pts',(6.7968764370129,-4.45715484572897,-4.76805369714416));
#20235=CARTESIAN_POINT('Ctrl Pts',(6.90979413463771,-4.2800100527293,-4.75983009521562));
#20236=CARTESIAN_POINT('Ctrl Pts',(7.01567275688913,-4.09878315244215,-4.75160649328707));
#20237=CARTESIAN_POINT('Ctrl Pts',(7.09370250267782,-3.96522371750828,-4.7455459160496));
#20238=CARTESIAN_POINT('Ctrl Pts',(7.16791000112718,-3.82944779232662,-4.73948533881213));
#20239=CARTESIAN_POINT('Ctrl Pts',(7.23817473186266,-3.69168174596956,-4.73342476157466));
#20240=CARTESIAN_POINT('Ctrl Pts',(7.33351627047917,-3.50474832017674,-4.7252012225007));
#20241=CARTESIAN_POINT('Ctrl Pts',(7.4216277987783,-3.31408911611699,-4.71697768342674));
#20242=CARTESIAN_POINT('Ctrl Pts',(7.50223448347721,-3.12028289060871,-4.70875414435278));
#20243=CARTESIAN_POINT('Ctrl Pts',(7.5828265124807,-2.92651190243866,-4.70053210046107));
#20244=CARTESIAN_POINT('Ctrl Pts',(7.65591630808611,-2.72959530701753,-4.69231005656936));
#20245=CARTESIAN_POINT('Ctrl Pts',(7.72127696362888,-2.53013233120998,-4.68408801267765));
#20246=CARTESIAN_POINT('Ctrl Pts',(7.78663040283976,-2.33069137768815,-4.67586687656443));
#20247=CARTESIAN_POINT('Ctrl Pts',(7.84425631388144,-2.12870488522847,-4.66764574045121));
#20248=CARTESIAN_POINT('Ctrl Pts',(7.89397723693811,-1.92478854558182,-4.65942460433799));
#20249=CARTESIAN_POINT('Ctrl Pts',(7.94370210361384,-1.72085603229403,-4.65120281616469));
#20250=CARTESIAN_POINT('Ctrl Pts',(7.98552065708786,-1.51499365189972,-4.64298102799139));
#20251=CARTESIAN_POINT('Ctrl Pts',(8.01930602506436,-1.3078296673751,-4.63475923981809));
#20252=CARTESIAN_POINT('Ctrl Pts',(8.05309129929548,-1.10066625767523,-4.62653747445805));
#20253=CARTESIAN_POINT('Ctrl Pts',(8.07884338780635,-0.892201542590064,
-4.61831570909802));
#20254=CARTESIAN_POINT('Ctrl Pts',(8.09648691627167,-0.683071868211351,
-4.61009394373799));
#20255=CARTESIAN_POINT('Ctrl Pts',(8.11413412311977,-0.473898593767195,
-4.60187046427636));
#20256=CARTESIAN_POINT('Ctrl Pts',(8.12366936798904,-0.264060377022058,
-4.59364698481474));
#20257=CARTESIAN_POINT('Ctrl Pts',(8.12506924132972,-0.0541976576764842,
-4.58542350535312));
#20258=CARTESIAN_POINT('Ctrl Pts',(8.12563484199933,0.0305946525547484,
-4.58210091511954));
#20259=CARTESIAN_POINT('Ctrl Pts',(8.12487296994328,0.11539094534123,-4.57877832488595));
#20260=CARTESIAN_POINT('Ctrl Pts',(8.12278449485915,0.200148975954851,-4.57545573465237));
#20261=CARTESIAN_POINT('Ctrl Pts',(8.11761543841465,0.409928373227015,-4.56723219557842));
#20262=CARTESIAN_POINT('Ctrl Pts',(8.10431454180795,0.619541492237617,-4.55900865650445));
#20263=CARTESIAN_POINT('Ctrl Pts',(8.08291570350302,0.828348533266186,-4.55078511743049));
#20264=CARTESIAN_POINT('Ctrl Pts',(8.06152075587859,1.0371176095477,-4.54256307353878));
#20265=CARTESIAN_POINT('Ctrl Pts',(8.03203083524404,1.24508060710941,-4.53434102964707));
#20266=CARTESIAN_POINT('Ctrl Pts',(7.99453173180774,1.45160254602257,-4.52611898575536));
#20267=CARTESIAN_POINT('Ctrl Pts',(7.95703676856823,1.65810168328472,-4.51789784964215));
#20268=CARTESIAN_POINT('Ctrl Pts',(7.91153444062383,1.8631597894672,-4.50967671352893));
#20269=CARTESIAN_POINT('Ctrl Pts',(7.85816185969371,2.06615095028293,-4.50145557741572));
#20270=CARTESIAN_POINT('Ctrl Pts',(7.80478504551296,2.26915821135924,-4.49323378924242));
#20271=CARTESIAN_POINT('Ctrl Pts',(7.74353680351568,2.47009791357987,-4.48501200106911));
#20272=CARTESIAN_POINT('Ctrl Pts',(7.67460471601866,2.66835717537292,-4.47679021289581));
#20273=CARTESIAN_POINT('Ctrl Pts',(7.60567281978979,2.86661588704942,-4.46856844753578));
#20274=CARTESIAN_POINT('Ctrl Pts',(7.52905722011355,3.06219389548709,-4.46034668217575));
#20275=CARTESIAN_POINT('Ctrl Pts',(7.44499463349515,3.25449573201878,-4.45212491681572));
#20276=CARTESIAN_POINT('Ctrl Pts',(7.36091452122291,3.44683766029109,-4.4439014373541));
#20277=CARTESIAN_POINT('Ctrl Pts',(7.2693844385665,3.63590178187527,-4.43567795789247));
#20278=CARTESIAN_POINT('Ctrl Pts',(7.1706887470963,3.82111377150256,-4.42745447843085));
#20279=CARTESIAN_POINT('Ctrl Pts',(7.13081203285308,3.8959462740644,-4.42413188819726));
#20280=CARTESIAN_POINT('Ctrl Pts',(7.08976609237674,3.97015019909408,-4.42080929796367));
#20281=CARTESIAN_POINT('Ctrl Pts',(7.04757180538567,4.04368881226449,-4.41748670773008));
#20282=CARTESIAN_POINT('Ctrl Pts',(6.94313931646145,4.22569971831549,-4.40926316865612));
#20283=CARTESIAN_POINT('Ctrl Pts',(6.83163516488619,4.40369240831537,-4.40103962958216));
#20284=CARTESIAN_POINT('Ctrl Pts',(6.71339380202864,4.57712040713192,-4.3928160905082));
#20285=CARTESIAN_POINT('Ctrl Pts',(6.59517393750472,4.75051687372583,-4.38459404661648));
#20286=CARTESIAN_POINT('Ctrl Pts',(6.47021947260325,4.91935006203631,-4.37637200272477));
#20287=CARTESIAN_POINT('Ctrl Pts',(6.33890819539813,5.08310244366709,-4.36814995883306));
#20288=CARTESIAN_POINT('Ctrl Pts',(6.20761141599382,5.24683674574323,-4.35992882271985));
#20289=CARTESIAN_POINT('Ctrl Pts',(6.06995940992534,5.40549113107433,-4.35170768660663));
#20290=CARTESIAN_POINT('Ctrl Pts',(5.92637077885693,5.55858048012356,-4.34348655049342));
#20291=CARTESIAN_POINT('Ctrl Pts',(5.78277075904442,5.71168197146712,-4.33526476232012));
#20292=CARTESIAN_POINT('Ctrl Pts',(5.63323337324402,5.85921732765079,-4.32704297414682));
#20293=CARTESIAN_POINT('Ctrl Pts',(5.47821539951651,6.00073692132893,-4.31882118597352));
#20294=CARTESIAN_POINT('Ctrl Pts',(5.32319785592232,6.14225612232813,-4.31059942061348));
#20295=CARTESIAN_POINT('Ctrl Pts',(5.16269997445483,6.27775939735401,-4.30237765525344));
#20296=CARTESIAN_POINT('Ctrl Pts',(4.99721344874421,6.40683582669245,-4.2941558898934));
#20297=CARTESIAN_POINT('Ctrl Pts',(4.83169242184021,6.53593916632363,-4.28593241043177));
#20298=CARTESIAN_POINT('Ctrl Pts',(4.66118090557146,6.65861280212723,-4.27770893097014));
#20299=CARTESIAN_POINT('Ctrl Pts',(4.48620242337377,6.77448709342746,-4.26948545150851));
#20300=CARTESIAN_POINT('Ctrl Pts',(4.41550463678005,6.82130459815806,-4.26616286127494));
#20301=CARTESIAN_POINT('Ctrl Pts',(4.34407797516309,6.86701262512926,-4.26284027104136));
#20302=CARTESIAN_POINT('Ctrl Pts',(4.2719582905141,6.91158881347899,-4.25951768080778));
#20303=CARTESIAN_POINT('Ctrl Pts',(4.09345928732092,7.02191660020329,-4.25129414173382));
#20304=CARTESIAN_POINT('Ctrl Pts',(3.91065501232499,7.12534372698899,-4.24307060265986));
#20305=CARTESIAN_POINT('Ctrl Pts',(3.72409977514372,7.22154889391981,-4.2348470635859));
#20306=CARTESIAN_POINT('Ctrl Pts',(3.53757845694513,7.31773656908015,-4.22662501969419));
#20307=CARTESIAN_POINT('Ctrl Pts',(3.34730779973729,7.4067047700262,-4.21840297580247));
#20308=CARTESIAN_POINT('Ctrl Pts',(3.15386643875261,7.48817828640651,-4.21018093191076));
#20309=CARTESIAN_POINT('Ctrl Pts',(2.96044643521978,7.56964280746806,-4.20195979579754));
#20310=CARTESIAN_POINT('Ctrl Pts',(2.7638566985175,7.64361418154556,-4.19373865968432));
#20311=CARTESIAN_POINT('Ctrl Pts',(2.56469632226102,7.70986513092679,-4.18551752357109));
#20312=CARTESIAN_POINT('Ctrl Pts',(2.36552014958323,7.77612133500741,-4.1772957353978));
#20313=CARTESIAN_POINT('Ctrl Pts',(2.16377320898779,7.8346557952561,-4.1690739472245));
#20314=CARTESIAN_POINT('Ctrl Pts',(1.9600712652865,7.88529062225979,-4.16085215905121));
#20315=CARTESIAN_POINT('Ctrl Pts',(1.75636988680338,7.93592530876543,-4.15263039369117));
#20316=CARTESIAN_POINT('Ctrl Pts',(1.55071380293803,7.97866033734236,-4.14440862833113));
#20317=CARTESIAN_POINT('Ctrl Pts',(1.34373105120879,8.01336848176329,-4.13618686297108));
#20318=CARTESIAN_POINT('Ctrl Pts',(1.136705147012,8.04808386225614,-4.12796338350946));
#20319=CARTESIAN_POINT('Ctrl Pts',(0.928352313331279,8.0747689666918,-4.11973990404783));
#20320=CARTESIAN_POINT('Ctrl Pts',(0.719308922504071,8.09334802393336,-4.1115164245862));
#20321=CARTESIAN_POINT('Ctrl Pts',(0.634847651335928,8.10085465107674,-4.10819383435263));
#20322=CARTESIAN_POINT('Ctrl Pts',(0.550273715462386,8.10703858915528,-4.10487124411907));
#20323=CARTESIAN_POINT('Ctrl Pts',(0.465629288968813,8.1118972458824,-4.1015486538855));
#20324=CARTESIAN_POINT('Ctrl Pts',(0.25613106627784,8.12392260881723,-4.09332511481154));
#20325=CARTESIAN_POINT('Ctrl Pts',(0.0461327158269894,8.12782982263373,
-4.08510157573759));
#20326=CARTESIAN_POINT('Ctrl Pts',(-0.16372533540842,8.12360028417483,-4.07687803666363));
#20327=CARTESIAN_POINT('Ctrl Pts',(-0.373545230804828,8.11937151471949,
-4.06865599277192));
#20328=CARTESIAN_POINT('Ctrl Pts',(-0.583224583169709,8.10700895164779,
-4.06043394888021));
#20329=CARTESIAN_POINT('Ctrl Pts',(-0.792123520158524,8.08654610395017,
-4.0522119049885));
#20330=CARTESIAN_POINT('Ctrl Pts',(-1.00099939305715,8.06608551551232,-4.04399076887528));
#20331=CARTESIAN_POINT('Ctrl Pts',(-1.20909472918742,8.03752645669771,-4.03576963276207));
#20332=CARTESIAN_POINT('Ctrl Pts',(-1.41577448911982,8.00095432798222,-4.02754849664885));
#20333=CARTESIAN_POINT('Ctrl Pts',(-1.6224706418742,7.96437929854537,-4.01932670847555));
#20334=CARTESIAN_POINT('Ctrl Pts',(-1.82775070319881,7.91978997808841,-4.01110492030225));
#20335=CARTESIAN_POINT('Ctrl Pts',(-2.03098849000564,7.8673231353469,-4.00288313212895));
#20336=CARTESIAN_POINT('Ctrl Pts',(-2.23422571288189,7.81485643818687,-3.99466136676892));
#20337=CARTESIAN_POINT('Ctrl Pts',(-2.43542038768013,7.75451233879826,-3.98643960140889));
#20338=CARTESIAN_POINT('Ctrl Pts',(-2.63395966256229,7.68647800091139,-3.97821783604886));
#20339=CARTESIAN_POINT('Ctrl Pts',(-2.83254032958749,7.61842947899445,-3.96999435658723));
#20340=CARTESIAN_POINT('Ctrl Pts',(-3.02846421169279,7.54268761129695,-3.9617708771256));
#20341=CARTESIAN_POINT('Ctrl Pts',(-3.22113562818867,7.45948877787973,-3.95354739766397));
#20342=CARTESIAN_POINT('Ctrl Pts',(-3.29898201544212,7.42587336816808,-3.95022480743039));
#20343=CARTESIAN_POINT('Ctrl Pts',(-3.3762976739393,7.39104118950326,-3.9469022171968));
#20344=CARTESIAN_POINT('Ctrl Pts',(-3.45304428304078,7.35501004362736,-3.94357962696321));
#20345=CARTESIAN_POINT('Ctrl Pts',(-3.64299510284388,7.26583156684903,-3.93535608788926));
#20346=CARTESIAN_POINT('Ctrl Pts',(-3.82952023818505,7.16927615582599,-3.9271325488153));
#20347=CARTESIAN_POINT('Ctrl Pts',(-4.01204766356215,7.06563239263164,-3.91890900974134));
#20348=CARTESIAN_POINT('Ctrl Pts',(-4.1945419022827,6.9620074736738,-3.91068696584964));
#20349=CARTESIAN_POINT('Ctrl Pts',(-4.37303962540975,6.8512969203726,-3.90246492195793));
#20350=CARTESIAN_POINT('Ctrl Pts',(-4.54699410849938,6.73383487618845,-3.89424287806623));
#20351=CARTESIAN_POINT('Ctrl Pts',(-4.7209293856421,6.6163858007404,-3.88602174195302));
#20352=CARTESIAN_POINT('Ctrl Pts',(-4.8903221798591,6.49218688759362,-3.87780060583981));
#20353=CARTESIAN_POINT('Ctrl Pts',(-5.05465472485914,6.36161561043727,-3.8695794697266));
#20354=CARTESIAN_POINT('Ctrl Pts',(-5.2190003039085,6.23103397700934,-3.8613576815533));
#20355=CARTESIAN_POINT('Ctrl Pts',(-5.37828459922607,6.09407915109421,-3.85313589337999));
#20356=CARTESIAN_POINT('Ctrl Pts',(-5.53202209158898,5.95116956073943,-3.84491410520669));
#20357=CARTESIAN_POINT('Ctrl Pts',(-5.68575915737158,5.80826036692043,-3.83669233984665));
#20358=CARTESIAN_POINT('Ctrl Pts',(-5.83394923680583,5.65939664449093,-3.82847057448661));
#20359=CARTESIAN_POINT('Ctrl Pts',(-5.97614252938187,5.50503478926457,-3.82024880912657));
#20360=CARTESIAN_POINT('Ctrl Pts',(-6.11836546689877,5.35064075215407,-3.81202532966495));
#20361=CARTESIAN_POINT('Ctrl Pts',(-6.25458892009618,5.19074650929195,-3.80380185020333));
#20362=CARTESIAN_POINT('Ctrl Pts',(-6.38440162261658,5.0258435594068,-3.7955783707417));
#20363=CARTESIAN_POINT('Ctrl Pts',(-6.43685076164627,4.95921666098309,-3.79225578050811));
#20364=CARTESIAN_POINT('Ctrl Pts',(-6.4882538298834,4.89177248929108,-3.78893319027452));
#20365=CARTESIAN_POINT('Ctrl Pts',(-6.53858560593557,4.82354494499141,-3.78561060004092));
#20366=CARTESIAN_POINT('Ctrl Pts',(-6.66315869437788,4.65467913939306,-3.77738706096696));
#20367=CARTESIAN_POINT('Ctrl Pts',(-6.78120681715271,4.48095748207517,-3.769163521893));
#20368=CARTESIAN_POINT('Ctrl Pts',(-6.89236436551681,4.30290611278634,-3.76093998281904));
#20369=CARTESIAN_POINT('Ctrl Pts',(-7.00350170350785,4.12488711632912,-3.75271793892732));
#20370=CARTESIAN_POINT('Ctrl Pts',(-7.10775081147395,3.9425402291546,-3.7444958950356));
#20371=CARTESIAN_POINT('Ctrl Pts',(-7.20479002365202,3.75641960882758,-3.73627385114388));
#20372=CARTESIAN_POINT('Ctrl Pts',(-7.30181852193517,3.57031953768601,-3.7280527150307));
#20373=CARTESIAN_POINT('Ctrl Pts',(-7.39163857737415,3.38044682663969,-3.71983157891752));
#20374=CARTESIAN_POINT('Ctrl Pts',(-7.47397462072646,3.18737994773712,-3.71161044280434));
#20375=CARTESIAN_POINT('Ctrl Pts',(-7.55631719456911,2.99429775571852,-3.70338865463104));
#20376=CARTESIAN_POINT('Ctrl Pts',(-7.63117445212954,2.79802115989834,-3.69516686645774));
#20377=CARTESIAN_POINT('Ctrl Pts',(-7.69831868155846,2.59914929153136,-3.68694507828445));
#20378=CARTESIAN_POINT('Ctrl Pts',(-7.76546272468028,2.40027797498013,-3.6787233129244));
#20379=CARTESIAN_POINT('Ctrl Pts',(-7.82489369069168,2.19881168058482,-3.67050154756434));
#20380=CARTESIAN_POINT('Ctrl Pts',(-7.87643335589743,1.995365919476,-3.66227978220429));
#20381=CARTESIAN_POINT('Ctrl Pts',(-7.92798376626765,1.79187774330387,-3.65405630274267));
#20382=CARTESIAN_POINT('Ctrl Pts',(-7.97163951674269,1.58640956194257,-3.64583282328105));
#20383=CARTESIAN_POINT('Ctrl Pts',(-8.00727298346709,1.37958940657647,-3.63760934381942));
#20384=CARTESIAN_POINT('Ctrl Pts',(-8.02167022359886,1.29602640486445,-3.63428675358583));
#20385=CARTESIAN_POINT('Ctrl Pts',(-8.0347584413262,1.21224281293768,-3.63096416335223));
#20386=CARTESIAN_POINT('Ctrl Pts',(-8.0465315997878,1.1282804510034,-3.62764157311864));
#20387=CARTESIAN_POINT('Ctrl Pts',(-8.07696037224254,0.911272278184235,
-3.61905404390901));
#20388=CARTESIAN_POINT('Ctrl Pts',(-8.09860760385926,0.693021489309309,
-3.61046651469939));
#20389=CARTESIAN_POINT('Ctrl Pts',(-8.11139938405216,0.474223148842588,
-3.60187898548977));
#20390=CARTESIAN_POINT('Ctrl Pts',(-8.12062559215414,0.316412508644634,
-3.59568513831799));
#20391=CARTESIAN_POINT('Ctrl Pts',(-8.125246116249,0.158317193216755,-3.58949129114622));
#20392=CARTESIAN_POINT('Ctrl Pts',(-8.12524999755206,0.000199449834196055,
-3.58329744397444));
#20393=CARTESIAN_POINT('Origin',(0.,0.,-16.4167025567876));
#20394=CARTESIAN_POINT('',(4.94635656995632,-6.44536625007808,-6.87494113800006));
#20395=CARTESIAN_POINT('',(4.94675008185374,-6.44587862049698,-6.70835078220711));
#20396=CARTESIAN_POINT('',(4.94675008185374,-6.44587862049697,-16.4167025567876));
#20397=CARTESIAN_POINT('',(-8.12524999741292,-0.000205039998872057,-5.41670255678761));
#20398=CARTESIAN_POINT('Ctrl Pts',(4.94675008185374,-6.44587862049698,-6.70835078220711));
#20399=CARTESIAN_POINT('Ctrl Pts',(5.11326951467367,-6.3180868846562,-6.70012907610502));
#20400=CARTESIAN_POINT('Ctrl Pts',(5.27483045724498,-6.18384202628876,-6.69190737000293));
#20401=CARTESIAN_POINT('Ctrl Pts',(5.43094150658574,-6.04355540344789,-6.68368566390084));
#20402=CARTESIAN_POINT('Ctrl Pts',(5.587088754445,-5.90323625140468,-6.67546205137649));
#20403=CARTESIAN_POINT('Ctrl Pts',(5.73778336380036,-5.75687273201702,-6.66723843885213));
#20404=CARTESIAN_POINT('Ctrl Pts',(5.88256886172007,-5.60491491011428,-6.65901482632778));
#20405=CARTESIAN_POINT('Ctrl Pts',(5.99213524715329,-5.48992087049424,-6.65279160982859));
#20406=CARTESIAN_POINT('Ctrl Pts',(6.09831836201026,-5.37172394965353,-6.6465683933294));
#20407=CARTESIAN_POINT('Ctrl Pts',(6.20093491455416,-5.25053271087451,-6.64034517683022));
#20408=CARTESIAN_POINT('Ctrl Pts',(6.33653540822028,-5.09038708720026,-6.63212163775625));
#20409=CARTESIAN_POINT('Ctrl Pts',(6.46595071955236,-4.92495960851299,-6.62389809868228));
#20410=CARTESIAN_POINT('Ctrl Pts',(6.58878083086729,-4.75475075322521,-6.61567455960831));
#20411=CARTESIAN_POINT('Ctrl Pts',(6.71158860953403,-4.58457284486441,-6.60745251571662));
#20412=CARTESIAN_POINT('Ctrl Pts',(6.82781340535999,-4.40961553404571,-6.59923047182492));
#20413=CARTESIAN_POINT('Ctrl Pts',(6.93709716899744,-4.23041019646886,-6.59100842793323));
#20414=CARTESIAN_POINT('Ctrl Pts',(7.04636886684463,-4.05122464457604,-6.58278729182009));
#20415=CARTESIAN_POINT('Ctrl Pts',(7.14870090898439,-3.86779225400607,-6.57456615570695));
#20416=CARTESIAN_POINT('Ctrl Pts',(7.24377961108072,-3.68067174692219,-6.56634501959381));
#20417=CARTESIAN_POINT('Ctrl Pts',(7.33886585435287,-3.49353639835843,-6.55812323142052));
#20418=CARTESIAN_POINT('Ctrl Pts',(7.4266974721114,-3.30271261053811,-6.54990144324723));
#20419=CARTESIAN_POINT('Ctrl Pts',(7.50700714670423,-3.10878292291882,-6.54167965507394));
#20420=CARTESIAN_POINT('Ctrl Pts',(7.58731659845966,-2.91485377340139,-6.53345788971386));
#20421=CARTESIAN_POINT('Ctrl Pts',(7.66010403844753,-2.71781901484677,-6.52523612435379));
#20422=CARTESIAN_POINT('Ctrl Pts',(7.72515042933764,-2.51828084347326,-6.51701435899371));
#20423=CARTESIAN_POINT('Ctrl Pts',(7.79021038131989,-2.31870107170516,-6.50879087953212));
#20424=CARTESIAN_POINT('Ctrl Pts',(7.84752596870894,-2.1166171249319,-6.50056740007052));
#20425=CARTESIAN_POINT('Ctrl Pts',(7.89692780213458,-1.91264707940956,-6.49234392060892));
#20426=CARTESIAN_POINT('Ctrl Pts',(7.91688797228293,-1.83023562761756,-6.48902133037526));
#20427=CARTESIAN_POINT('Ctrl Pts',(7.93555682812912,-1.74751643068539,-6.4856987401416));
#20428=CARTESIAN_POINT('Ctrl Pts',(7.95292554614784,-1.66453081074789,-6.48237614990794));
#20429=CARTESIAN_POINT('Ctrl Pts',(7.99591379364358,-1.45913819831596,-6.47415261083398));
#20430=CARTESIAN_POINT('Ctrl Pts',(8.03094805362722,-1.25204601077799,-6.46592907176003));
#20431=CARTESIAN_POINT('Ctrl Pts',(8.05791486960765,-1.04388481963096,-6.45770553268607));
#20432=CARTESIAN_POINT('Ctrl Pts',(8.08487678255251,-0.835761475804336,
-6.44948348879436));
#20433=CARTESIAN_POINT('Ctrl Pts',(8.10377414118939,-0.626569808641515,
-6.44126144490266));
#20434=CARTESIAN_POINT('Ctrl Pts',(8.1145451062385,-0.416947576226108,-6.43303940101096));
#20435=CARTESIAN_POINT('Ctrl Pts',(8.12531488208813,-0.207348487758192,
-6.42481826489773));
#20436=CARTESIAN_POINT('Ctrl Pts',(8.12796004048379,0.00268077662337693,
-6.41659712878451));
#20437=CARTESIAN_POINT('Ctrl Pts',(8.12247077617056,0.212499535893956,-6.40837599267128));
#20438=CARTESIAN_POINT('Ctrl Pts',(8.11698107647588,0.422334936956949,-6.40015420449796));
#20439=CARTESIAN_POINT('Ctrl Pts',(8.1033556700032,0.63195950463673,-6.39193241632464));
#20440=CARTESIAN_POINT('Ctrl Pts',(8.08163686529504,0.840733691488665,-6.38371062815132));
#20441=CARTESIAN_POINT('Ctrl Pts',(8.05991812085099,1.04950729904586,-6.37548886279135));
#20442=CARTESIAN_POINT('Ctrl Pts',(8.03010605629281,1.25743023742523,-6.36726709743138));
#20443=CARTESIAN_POINT('Ctrl Pts',(7.99229479569316,1.46386866256367,-6.35904533207141));
#20444=CARTESIAN_POINT('Ctrl Pts',(7.95447565207312,1.67035012668813,-6.35082185260979));
#20445=CARTESIAN_POINT('Ctrl Pts',(7.90865403397151,1.87534616912787,-6.34259837314818));
#20446=CARTESIAN_POINT('Ctrl Pts',(7.85497528534438,2.07823262151497,-6.33437489368657));
#20447=CARTESIAN_POINT('Ctrl Pts',(7.83328708307246,2.16020626155208,-6.33105230345293));
#20448=CARTESIAN_POINT('Ctrl Pts',(7.81031681357776,2.24183565845636,-6.32772971321928));
#20449=CARTESIAN_POINT('Ctrl Pts',(7.78607639342532,2.32308027374109,-6.32440712298564));
#20450=CARTESIAN_POINT('Ctrl Pts',(7.72608041791378,2.52416383245887,-6.3161835839117));
#20451=CARTESIAN_POINT('Ctrl Pts',(7.65828074572195,2.72295462188927,-6.30796004483777));
#20452=CARTESIAN_POINT('Ctrl Pts',(7.58287785573238,2.91884411840432,-6.29973650576383));
#20453=CARTESIAN_POINT('Ctrl Pts',(7.5074886752977,3.11469799880699,-6.2915144618721));
#20454=CARTESIAN_POINT('Ctrl Pts',(7.42449914206898,3.30765136402373,-6.28329241798038));
#20455=CARTESIAN_POINT('Ctrl Pts',(7.33415854708852,3.49711394848214,-6.27507037408866));
#20456=CARTESIAN_POINT('Ctrl Pts',(7.24382792642313,3.68655561477513,-6.26684923797551));
#20457=CARTESIAN_POINT('Ctrl Pts',(7.14614799125664,3.87250700365054,-6.25862810186236));
#20458=CARTESIAN_POINT('Ctrl Pts',(7.04141518117523,4.05440005534913,-6.25040696574921));
#20459=CARTESIAN_POINT('Ctrl Pts',(6.93667406420138,4.2363075339118,-6.24218517757589));
#20460=CARTESIAN_POINT('Ctrl Pts',(6.82487909945776,4.41415577521435,-6.23396338940258));
#20461=CARTESIAN_POINT('Ctrl Pts',(6.7063720137003,4.58740253044764,-6.22574160122926));
#20462=CARTESIAN_POINT('Ctrl Pts',(6.5878652567695,4.76064880496577,-6.21751983586929));
#20463=CARTESIAN_POINT('Ctrl Pts',(6.46264658482042,4.92929337704814,-6.20929807050932));
#20464=CARTESIAN_POINT('Ctrl Pts',(6.33110057357052,5.09282368532772,-6.20107630514935));
#20465=CARTESIAN_POINT('Ctrl Pts',(6.19952713715985,5.25638808696333,-6.19285282568771));
#20466=CARTESIAN_POINT('Ctrl Pts',(6.06162391106848,5.41483586490666,-6.18462934622608));
#20467=CARTESIAN_POINT('Ctrl Pts',(5.91781590475822,5.56768735471836,-6.17640586676445));
#20468=CARTESIAN_POINT('Ctrl Pts',(5.85971214472291,5.62944501698576,-6.17308327653075));
#20469=CARTESIAN_POINT('Ctrl Pts',(5.80064489493821,5.69028950500846,-6.16976068629705));
#20470=CARTESIAN_POINT('Ctrl Pts',(5.74064393689378,5.75019084485938,-6.16643809606335));
#20471=CARTESIAN_POINT('Ctrl Pts',(5.59213924981279,5.89844897306637,-6.15821455698939));
#20472=CARTESIAN_POINT('Ctrl Pts',(5.43786399151661,6.04097517483154,-6.14999101791542));
#20473=CARTESIAN_POINT('Ctrl Pts',(5.27828420577773,6.1773297957562,-6.14176747884146));
#20474=CARTESIAN_POINT('Ctrl Pts',(5.11873343441515,6.31365962504285,-6.13354543494971));
#20475=CARTESIAN_POINT('Ctrl Pts',(4.95388028466916,6.44381992157428,-6.12532339105795));
#20476=CARTESIAN_POINT('Ctrl Pts',(4.78422503028089,6.56741032844254,-6.1171013471662));
#20477=CARTESIAN_POINT('Ctrl Pts',(4.6145885071715,6.6909870899546,-6.10888021105298));
#20478=CARTESIAN_POINT('Ctrl Pts',(4.44015117621969,6.80799523638049,-6.10065907493975));
#20479=CARTESIAN_POINT('Ctrl Pts',(4.26144419847832,6.91807638767855,-6.09243793882653));
#20480=CARTESIAN_POINT('Ctrl Pts',(4.08272304657839,7.02816627007213,-6.08421615065322));
#20481=CARTESIAN_POINT('Ctrl Pts',(3.89973182097379,7.13132790261098,-6.07599436247992));
#20482=CARTESIAN_POINT('Ctrl Pts',(3.7130292166108,7.22724716604425,-6.06777257430661));
#20483=CARTESIAN_POINT('Ctrl Pts',(3.52632713029842,7.32316616332679,-6.0595508089466));
#20484=CARTESIAN_POINT('Ctrl Pts',(3.33591394939592,7.41184269932437,-6.05132904358659));
#20485=CARTESIAN_POINT('Ctrl Pts',(3.14237191287177,7.49300916345994,-6.04310727822659));
#20486=CARTESIAN_POINT('Ctrl Pts',(2.94878952604574,7.57419254945594,-6.03488379876498));
#20487=CARTESIAN_POINT('Ctrl Pts',(2.7520772524932,7.64786262163657,-6.02666031930337));
#20488=CARTESIAN_POINT('Ctrl Pts',(2.55283722314821,7.7137999503882,-6.01843683984177));
#20489=CARTESIAN_POINT('Ctrl Pts',(2.47233687305581,7.74044107298848,-6.0151142496082));
#20490=CARTESIAN_POINT('Ctrl Pts',(2.39142407639492,7.76582041608099,-6.01179165937464));
#20491=CARTESIAN_POINT('Ctrl Pts',(2.31013929405954,7.78992580224883,-6.00846906914107));
#20492=CARTESIAN_POINT('Ctrl Pts',(2.10895632033603,7.84958756343791,-6.00024553006711));
#20493=CARTESIAN_POINT('Ctrl Pts',(1.90542819374412,7.90146120990598,-5.99202199099315));
#20494=CARTESIAN_POINT('Ctrl Pts',(1.70017407837136,7.94538203397005,-5.98379845191919));
#20495=CARTESIAN_POINT('Ctrl Pts',(1.49495728176153,7.98929487246551,-5.97557640802745));
#20496=CARTESIAN_POINT('Ctrl Pts',(1.28801541097213,8.02525771284695,-5.96735436413572));
#20497=CARTESIAN_POINT('Ctrl Pts',(1.07997901904253,8.05315670286677,-5.95913232024398));
#20498=CARTESIAN_POINT('Ctrl Pts',(0.871965595972208,8.08105261261793,-5.95091118413078));
#20499=CARTESIAN_POINT('Ctrl Pts',(0.662858185225844,8.10088641029755,-5.94269004801757));
#20500=CARTESIAN_POINT('Ctrl Pts',(0.453294513595352,8.11259586362123,-5.93446891190436));
#20501=CARTESIAN_POINT('Ctrl Pts',(0.243714220404542,8.1243062456812,-5.92624712373105));
#20502=CARTESIAN_POINT('Ctrl Pts',(0.0336778883579213,8.12789097674848,
-5.91802533555773));
#20503=CARTESIAN_POINT('Ctrl Pts',(-0.176173618367589,8.12333985616084,
-5.90980354738442));
#20504=CARTESIAN_POINT('Ctrl Pts',(-0.386024542812005,8.11878874820134,
-5.90158178202434));
#20505=CARTESIAN_POINT('Ctrl Pts',(-0.595690348156888,8.10610184283517,
-5.89336001666426));
#20506=CARTESIAN_POINT('Ctrl Pts',(-0.804531611719473,8.08532104793892,
-5.88513825130418));
#20507=CARTESIAN_POINT('Ctrl Pts',(-1.01341641521735,8.06453592059203,-5.87691477184256));
#20508=CARTESIAN_POINT('Ctrl Pts',(-1.22147603998337,8.03565356189918,-5.86869129238094));
#20509=CARTESIAN_POINT('Ctrl Pts',(-1.42807651257622,7.99876771988837,-5.86046781291932));
#20510=CARTESIAN_POINT('Ctrl Pts',(-1.51155075431057,7.9838644737634,-5.85714522268581));
#20511=CARTESIAN_POINT('Ctrl Pts',(-1.59478688650748,7.96765527834915,-5.85382263245229));
#20512=CARTESIAN_POINT('Ctrl Pts',(-1.67774353105893,7.95014869084157,-5.85050004221878));
#20513=CARTESIAN_POINT('Ctrl Pts',(-1.88306442830071,7.90681921103757,-5.84227650314483));
#20514=CARTESIAN_POINT('Ctrl Pts',(-2.08673923399196,7.8555245033341,-5.83405296407088));
#20515=CARTESIAN_POINT('Ctrl Pts',(-2.28814505236409,7.79641454656188,-5.82582942499694));
#20516=CARTESIAN_POINT('Ctrl Pts',(-2.48951425166124,7.73731533700619,-5.81760738110519));
#20517=CARTESIAN_POINT('Ctrl Pts',(-2.6886150041662,7.67040379744663,-5.80938533721345));
#20518=CARTESIAN_POINT('Ctrl Pts',(-2.88483861404142,7.59588004996364,-5.8011632933217));
#20519=CARTESIAN_POINT('Ctrl Pts',(-3.08104055927825,7.52136453049174,-5.79294215720862));
#20520=CARTESIAN_POINT('Ctrl Pts',(-3.27436572046839,7.43923858569441,-5.78472102109554));
#20521=CARTESIAN_POINT('Ctrl Pts',(-3.46422367242602,7.34975114612074,-5.77649988498246));
#20522=CARTESIAN_POINT('Ctrl Pts',(-3.65409668298617,7.26025660884182,-5.76827809680914));
#20523=CARTESIAN_POINT('Ctrl Pts',(-3.84050166691176,7.16339953349815,-5.76005630863583));
#20524=CARTESIAN_POINT('Ctrl Pts',(-4.02287021511202,7.05947609917794,-5.75183452046252));
#20525=CARTESIAN_POINT('Ctrl Pts',(-4.20523825728861,6.9555529532173,-5.74361275510245));
#20526=CARTESIAN_POINT('Ctrl Pts',(-4.38356963123258,6.84456363586739,-5.73539098974239));
#20527=CARTESIAN_POINT('Ctrl Pts',(-4.55732200706753,6.72684946214778,-5.72716922438233));
#20528=CARTESIAN_POINT('Ctrl Pts',(-4.73111060738766,6.60911074697762,-5.71894574492071));
#20529=CARTESIAN_POINT('Ctrl Pts',(-4.90031805827466,6.48464454005489,-5.71072226545909));
#20530=CARTESIAN_POINT('Ctrl Pts',(-5.06443150553653,6.35383514802115,-5.70249878599748));
#20531=CARTESIAN_POINT('Ctrl Pts',(-5.13073941566506,6.30098330951763,-5.69917619576382));
#20532=CARTESIAN_POINT('Ctrl Pts',(-5.19621610995916,6.24709644447586,-5.69585360553015));
#20533=CARTESIAN_POINT('Ctrl Pts',(-5.26082927658764,6.1922017800697,-5.69253101529649));
#20534=CARTESIAN_POINT('Ctrl Pts',(-5.42074935793885,6.05633536683449,-5.6843074762225));
#20535=CARTESIAN_POINT('Ctrl Pts',(-5.57542926357776,5.91424842055227,-5.67608393714851));
#20536=CARTESIAN_POINT('Ctrl Pts',(-5.72439265504912,5.76636942046897,-5.66786039807451));
#20537=CARTESIAN_POINT('Ctrl Pts',(-5.87332896238828,5.61851730735668,-5.65963835418277));
#20538=CARTESIAN_POINT('Ctrl Pts',(-6.0165506207996,5.46487544998669,-5.65141631029103));
#20539=CARTESIAN_POINT('Ctrl Pts',(-6.15361765455743,5.30590966037108,-5.64319426639929));
#20540=CARTESIAN_POINT('Ctrl Pts',(-6.29066955503286,5.14696142183336,-5.63497313028609));
#20541=CARTESIAN_POINT('Ctrl Pts',(-6.42156799496789,4.98269064785968,-5.62675199417289));
#20542=CARTESIAN_POINT('Ctrl Pts',(-6.54591230544676,4.81359737118724,-5.61853085805969));
#20543=CARTESIAN_POINT('Ctrl Pts',(-6.67026647830487,4.6444906828676,-5.6103090698864));
#20544=CARTESIAN_POINT('Ctrl Pts',(-6.78806530614967,4.47056096362867,-5.60208728171312));
#20545=CARTESIAN_POINT('Ctrl Pts',(-6.8989499777136,4.29233931178623,-5.59386549353983));
#20546=CARTESIAN_POINT('Ctrl Pts',(-7.00983434160183,4.11411815446185,-5.58564372817984));
#20547=CARTESIAN_POINT('Ctrl Pts',(-7.11380443407122,3.9316053402002,-5.57742196281984));
#20548=CARTESIAN_POINT('Ctrl Pts',(-7.21054586853405,3.74535924048235,-5.56920019745984));
#20549=CARTESIAN_POINT('Ctrl Pts',(-7.30730747198066,3.55907431154324,-5.5609767179982));
#20550=CARTESIAN_POINT('Ctrl Pts',(-7.39683727078198,3.36905480404923,-5.55275323853656));
#20551=CARTESIAN_POINT('Ctrl Pts',(-7.47886726874041,3.17588285978297,-5.54452975907492));
#20552=CARTESIAN_POINT('Ctrl Pts',(-7.5120104256423,3.09783424077528,-5.54120716884134));
#20553=CARTESIAN_POINT('Ctrl Pts',(-7.54392981177007,3.01927124370574,-5.53788457860777));
#20554=CARTESIAN_POINT('Ctrl Pts',(-7.57460997759708,2.94023319649765,-5.5345619883742));
#20555=CARTESIAN_POINT('Ctrl Pts',(-7.65032303275941,2.74518170746946,-5.52636244150556));
#20556=CARTESIAN_POINT('Ctrl Pts',(-7.71851174710653,2.54716866060428,-5.51816289463691));
#20557=CARTESIAN_POINT('Ctrl Pts',(-7.77896172904498,2.34679397914549,-5.50996334776827));
#20558=CARTESIAN_POINT('Ctrl Pts',(-7.83940391141622,2.14644515105746,-5.50176485884729));
#20559=CARTESIAN_POINT('Ctrl Pts',(-7.8921092654707,1.94373558132762,-5.4935663699263));
#20560=CARTESIAN_POINT('Ctrl Pts',(-7.9369131001647,1.73928088672702,-5.48536788100532));
#20561=CARTESIAN_POINT('Ctrl Pts',(-7.98171097779131,1.53485337619231,-5.47717048214618));
#20562=CARTESIAN_POINT('Ctrl Pts',(-8.01860937032492,1.32868149561549,-5.46897308328705));
#20563=CARTESIAN_POINT('Ctrl Pts',(-8.04749445669988,1.12139222927782,-5.46077568442792));
#20564=CARTESIAN_POINT('Ctrl Pts',(-8.07638215447811,0.914084222616474,
-5.45257754446959));
#20565=CARTESIAN_POINT('Ctrl Pts',(-8.09725505496413,0.705658923625393,
-5.44437940451127));
#20566=CARTESIAN_POINT('Ctrl Pts',(-8.11005094317767,0.496750703636092,
-5.43618126455294));
#20567=CARTESIAN_POINT('Ctrl Pts',(-8.12018524877937,0.33129601157046,-5.4296883619645));
#20568=CARTESIAN_POINT('Ctrl Pts',(-8.12525417993961,0.165538596538109,
-5.42319545937606));
#20569=CARTESIAN_POINT('Ctrl Pts',(-8.12524999741292,-0.000205039998872057,
-5.41670255678761));
#20570=CARTESIAN_POINT('Ctrl Pts',(-8.12515360481363,-0.000205119571382809,
-5.41670255357508));
#20571=CARTESIAN_POINT('Ctrl Pts',(-8.12549042833445,-0.341492182439963,
-5.40333268953402));
#20572=CARTESIAN_POINT('Ctrl Pts',(-8.02126726985289,-2.02671189518092,
-5.33730648318554));
#20573=CARTESIAN_POINT('Ctrl Pts',(-6.87936488829688,-4.93498266901478,
-5.21862393452961));
#20574=CARTESIAN_POINT('Ctrl Pts',(-3.69965148811969,-7.61526717037964,
-5.06065490760733));
#20575=CARTESIAN_POINT('Ctrl Pts',(0.372694242426441,-8.45818031325121,
-4.90268588068503));
#20576=CARTESIAN_POINT('Ctrl Pts',(3.3333249850863,-7.56768303558379,-4.78524786975563));
#20577=CARTESIAN_POINT('Ctrl Pts',(4.70140933544592,-6.63456619566222,-4.72046620113364));
#20578=CARTESIAN_POINT('Ctrl Pts',(4.94675083769988,-6.44587978308508,-4.70834087481909));
#20579=CARTESIAN_POINT('',(-8.12524999887038,-0.000135487633930348,-5.58329744173371));
#20580=CARTESIAN_POINT('Ctrl Pts',(-8.12524999887038,-0.000135487633930348,
-5.58329744173372));
#20581=CARTESIAN_POINT('Ctrl Pts',(-8.12524640323817,-0.215767052978142,
-5.57485194371586));
#20582=CARTESIAN_POINT('Ctrl Pts',(-8.11665467706683,-0.431363576694395,
-5.56640644569801));
#20583=CARTESIAN_POINT('Ctrl Pts',(-8.09950915629719,-0.646249943565126,
-5.55796094768016));
#20584=CARTESIAN_POINT('Ctrl Pts',(-8.08235819985755,-0.861204436181145,
-5.54951277217348));
#20585=CARTESIAN_POINT('Ctrl Pts',(-8.0566480513228,-1.07544806406917,-5.5410645966668));
#20586=CARTESIAN_POINT('Ctrl Pts',(-8.0224649720171,-1.28831026358508,-5.53261642116012));
#20587=CARTESIAN_POINT('Ctrl Pts',(-8.00985897584013,-1.36680933762468,
-5.52950091283546));
#20588=CARTESIAN_POINT('Ctrl Pts',(-7.99610118526879,-1.44512061066931,
-5.52638540451079));
#20589=CARTESIAN_POINT('Ctrl Pts',(-7.98119769287493,-1.52321073714307,
-5.52326989618613));
#20590=CARTESIAN_POINT('Ctrl Pts',(-7.94185918394878,-1.72933350730643,
-5.51504635711217));
#20591=CARTESIAN_POINT('Ctrl Pts',(-7.89452501494402,-1.93396500526429,
-5.50682281803822));
#20592=CARTESIAN_POINT('Ctrl Pts',(-7.83933305352944,-2.13647954315989,
-5.49859927896427));
#20593=CARTESIAN_POINT('Ctrl Pts',(-7.78415112697202,-2.33895726039526,
-5.49037723507254));
#20594=CARTESIAN_POINT('Ctrl Pts',(-7.7211143370056,-2.53931850136954,-5.48215519118081));
#20595=CARTESIAN_POINT('Ctrl Pts',(-7.65041096056426,-2.73695080280561,
-5.47393314728908));
#20596=CARTESIAN_POINT('Ctrl Pts',(-7.57971539033323,-2.93456128407708,
-5.46571201117584));
#20597=CARTESIAN_POINT('Ctrl Pts',(-7.50135502284532,-3.12944314974693,
-5.45749087506261));
#20598=CARTESIAN_POINT('Ctrl Pts',(-7.4155672887339,-3.32100125696448,-5.44926973894936));
#20599=CARTESIAN_POINT('Ctrl Pts',(-7.32977275036152,-3.51257455762857,
-5.44104795077606));
#20600=CARTESIAN_POINT('Ctrl Pts',(-7.23654978641785,-3.70082330282996,
-5.43282616260275));
#20601=CARTESIAN_POINT('Ctrl Pts',(-7.13618349425367,-3.88517344514264,
-5.42460437442944));
#20602=CARTESIAN_POINT('Ctrl Pts',(-7.03581748057934,-4.06952307593254,
-5.41638260906941));
#20603=CARTESIAN_POINT('Ctrl Pts',(-6.92830832172635,-4.2499738677314,-5.40816084370939));
#20604=CARTESIAN_POINT('Ctrl Pts',(-6.81398674836912,-4.425976971873,-5.39993907834937));
#20605=CARTESIAN_POINT('Ctrl Pts',(-6.69964134086152,-4.60201676974024,
-5.39171559888774));
#20606=CARTESIAN_POINT('Ctrl Pts',(-6.57848084223118,-4.77360678015207,
-5.38349211942612));
#20607=CARTESIAN_POINT('Ctrl Pts',(-6.45087953845506,-4.94022679062833,
-5.3752686399645));
#20608=CARTESIAN_POINT('Ctrl Pts',(-6.39932388641089,-5.00754744511616,
-5.37194604973094));
#20609=CARTESIAN_POINT('Ctrl Pts',(-6.34671727864032,-5.0740571176318,-5.36862345949738));
#20610=CARTESIAN_POINT('Ctrl Pts',(-6.29308631040874,-5.13972297427071,
-5.36530086926382));
#20611=CARTESIAN_POINT('Ctrl Pts',(-6.16034759397832,-5.30224850403392,
-5.35707733018986));
#20612=CARTESIAN_POINT('Ctrl Pts',(-6.02128786593954,-5.45965551007142,
-5.3488537911159));
#20613=CARTESIAN_POINT('Ctrl Pts',(-5.8763262848951,-5.61145943190815,-5.34063025204194));
#20614=CARTESIAN_POINT('Ctrl Pts',(-5.73139106038399,-5.76323575315515,
-5.33240820815022));
#20615=CARTESIAN_POINT('Ctrl Pts',(-5.58055632815796,-5.90941081028956,
-5.3241861642585));
#20616=CARTESIAN_POINT('Ctrl Pts',(-5.42427927792612,-6.04953567454241,
-5.31596412036679));
#20617=CARTESIAN_POINT('Ctrl Pts',(-5.2680194819138,-6.18964506790452,-5.30774298425359));
#20618=CARTESIAN_POINT('Ctrl Pts',(-5.10631878702397,-6.32370540518375,
-5.29952184814041));
#20619=CARTESIAN_POINT('Ctrl Pts',(-4.93966935972606,-6.45130639321088,
-5.29130071202721));
#20620=CARTESIAN_POINT('Ctrl Pts',(-4.77300671461452,-6.57891750192132,
-5.28307892385391));
#20621=CARTESIAN_POINT('Ctrl Pts',(-4.60139478539431,-6.7000680562976,-5.2748571356806));
#20622=CARTESIAN_POINT('Ctrl Pts',(-4.4253576102235,-6.81438901033225,-5.26663534750729));
#20623=CARTESIAN_POINT('Ctrl Pts',(-4.24932092350857,-6.92870964715696,
-5.25841358214723));
#20624=CARTESIAN_POINT('Ctrl Pts',(-4.06885926422392,-7.03620056317625,
-5.25019181678718));
#20625=CARTESIAN_POINT('Ctrl Pts',(-3.88452480031184,-7.13653659965829,
-5.24197005142712));
#20626=CARTESIAN_POINT('Ctrl Pts',(-3.70015190572471,-7.23689355453795,
-5.23374657196551));
#20627=CARTESIAN_POINT('Ctrl Pts',(-3.51190485261628,-7.33009250891737,
-5.22552309250389));
#20628=CARTESIAN_POINT('Ctrl Pts',(-3.32036047463938,-7.41585422462932,
-5.21729961304227));
#20629=CARTESIAN_POINT('Ctrl Pts',(-3.2429694526841,-7.45050513369639,-5.21397702280869));
#20630=CARTESIAN_POINT('Ctrl Pts',(-3.16504041072694,-7.48394248016693,
-5.21065443257512));
#20631=CARTESIAN_POINT('Ctrl Pts',(-3.08661236960116,-7.51615005453757,
-5.20733184234154));
#20632=CARTESIAN_POINT('Ctrl Pts',(-2.89249994063715,-7.59586504425786,
-5.19910830326758));
#20633=CARTESIAN_POINT('Ctrl Pts',(-2.69526624876149,-7.66806922904659,
-5.19088476419362));
#20634=CARTESIAN_POINT('Ctrl Pts',(-2.49551061114153,-7.73253608799727,
-5.18266122511966));
#20635=CARTESIAN_POINT('Ctrl Pts',(-2.29579129256633,-7.79699122575317,
-5.17443918122795));
#20636=CARTESIAN_POINT('Ctrl Pts',(-2.09355122396812,-7.85371175490497,
-5.16621713733624));
#20637=CARTESIAN_POINT('Ctrl Pts',(-1.88940619951778,-7.90252059634923,
-5.15799509344453));
#20638=CARTESIAN_POINT('Ctrl Pts',(-1.68528371428788,-7.95132404891252,
-5.14977395733129));
#20639=CARTESIAN_POINT('Ctrl Pts',(-1.47925697984454,-7.99221748914817,
-5.14155282121806));
#20640=CARTESIAN_POINT('Ctrl Pts',(-1.27195415117231,-8.02507446693272,
-5.13333168510483));
#20641=CARTESIAN_POINT('Ctrl Pts',(-1.06463488025978,-8.05793405077108,
-5.12510989693153));
#20642=CARTESIAN_POINT('Ctrl Pts',(-0.856039603776485,-8.08275584976062,
-5.11688810875824));
#20643=CARTESIAN_POINT('Ctrl Pts',(-0.646804863534513,-8.09946486077988,
-5.10866632058494));
#20644=CARTESIAN_POINT('Ctrl Pts',(-0.437570703863254,-8.11617382543609,
-5.10044455522492));
#20645=CARTESIAN_POINT('Ctrl Pts',(-0.227697378193396,-8.12477002636174,
-5.0922227898649));
#20646=CARTESIAN_POINT('Ctrl Pts',(-0.0178252675763609,-8.12523044733722,
-5.08400102450488));
#20647=CARTESIAN_POINT('Ctrl Pts',(0.192090597892018,-8.12569096430283,
-5.07577754504326));
#20648=CARTESIAN_POINT('Ctrl Pts',(0.402004952816498,-8.1180123121998,-5.06755406558164));
#20649=CARTESIAN_POINT('Ctrl Pts',(0.611277591239238,-8.1022236002809,-5.05933058612001));
#20650=CARTESIAN_POINT('Ctrl Pts',(0.695831486926034,-8.09584437597962,
-5.05600799588642));
#20651=CARTESIAN_POINT('Ctrl Pts',(0.780280656271626,-8.08814181041789,
-5.05268540565284));
#20652=CARTESIAN_POINT('Ctrl Pts',(0.864583067615009,-8.07912022943671,
-5.04936281541925));
#20653=CARTESIAN_POINT('Ctrl Pts',(1.07323478960695,-8.05679146829194,-5.04113927634528));
#20654=CARTESIAN_POINT('Ctrl Pts',(1.28105494401805,-8.02637178827214,-5.03291573727132));
#20655=CARTESIAN_POINT('Ctrl Pts',(1.48740865519046,-7.98794736180481,-5.02469219819735));
#20656=CARTESIAN_POINT('Ctrl Pts',(1.69372484767351,-7.94952992156571,-5.01647015430565));
#20657=CARTESIAN_POINT('Ctrl Pts',(1.89857483926335,-7.90311069365899,-5.00824811041394));
#20658=CARTESIAN_POINT('Ctrl Pts',(2.1013328068858,-7.84882717335561,-5.00002606652223));
#20659=CARTESIAN_POINT('Ctrl Pts',(2.30406838842982,-7.79454964638092,-4.99180493040901));
#20660=CARTESIAN_POINT('Ctrl Pts',(2.50471212235133,-7.73240963674396,-4.98358379429578));
#20661=CARTESIAN_POINT('Ctrl Pts',(2.70265142306076,-7.66259504658361,-4.97536265818255));
#20662=CARTESIAN_POINT('Ctrl Pts',(2.9006064233417,-7.59277491907344,-4.96714087000925));
#20663=CARTESIAN_POINT('Ctrl Pts',(3.09585628278475,-7.5152790903875,-4.95891908183595));
#20664=CARTESIAN_POINT('Ctrl Pts',(3.28780553736328,-7.43034469664654,-4.95069729366265));
#20665=CARTESIAN_POINT('Ctrl Pts',(3.47975425933399,-7.34541053857579,-4.94247552830262));
#20666=CARTESIAN_POINT('Ctrl Pts',(3.66840212614289,-7.25303797854477,-4.93425376294258));
#20667=CARTESIAN_POINT('Ctrl Pts',(3.85317505138024,-7.15351169607773,-4.92603199758255));
#20668=CARTESIAN_POINT('Ctrl Pts',(4.03798649870529,-7.05396466403292,-4.91780851812091));
#20669=CARTESIAN_POINT('Ctrl Pts',(4.21892113087728,-6.94726106998677,-4.90958503865928));
#20670=CARTESIAN_POINT('Ctrl Pts',(4.39542983513849,-6.83373134728564,-4.90136155919765));
#20671=CARTESIAN_POINT('Ctrl Pts',(4.46674588811264,-6.78786113509309,-4.89803896896409));
#20672=CARTESIAN_POINT('Ctrl Pts',(4.53733973621985,-6.74087709175163,-4.89471637873052));
#20673=CARTESIAN_POINT('Ctrl Pts',(4.60717647814807,-6.6928030347306,-4.89139378849695));
#20674=CARTESIAN_POINT('Ctrl Pts',(4.7224576576741,-6.61344603947325,-4.88590910936343));
#20675=CARTESIAN_POINT('Ctrl Pts',(4.8357005107187,-6.53110121115441,-4.8804244302299));
#20676=CARTESIAN_POINT('Ctrl Pts',(4.94675008185375,-6.44587862049697,-4.87493975109638));
#20677=CARTESIAN_POINT('Ctrl Pts',(4.94635656996294,-6.445366250073,-6.87494113799973));
#20678=CARTESIAN_POINT('Ctrl Pts',(5.53980426391237,-5.98964994661794,-6.84563479585463));
#20679=CARTESIAN_POINT('Ctrl Pts',(7.02552761858039,-4.48811509720809,-6.76367211140211));
#20680=CARTESIAN_POINT('Ctrl Pts',(8.37906827853382,-1.21281902750414,-6.62905308464214));
#20681=CARTESIAN_POINT('Ctrl Pts',(7.94572663628765,2.92320772973764,-6.47108405771986));
#20682=CARTESIAN_POINT('Ctrl Pts',(5.59528212459546,6.35393839724545,-6.31311503079756));
#20683=CARTESIAN_POINT('Ctrl Pts',(1.89483755533364,8.25162443696425,-6.15514600387528));
#20684=CARTESIAN_POINT('Ctrl Pts',(-2.26278339070844,8.15840220487702,-5.99717697695297));
#20685=CARTESIAN_POINT('Ctrl Pts',(-5.87445193619213,6.09676386775613,-5.8392079500307));
#20686=CARTESIAN_POINT('Ctrl Pts',(-7.79082080228488,3.01159239845082,-5.70124810545049));
#20687=CARTESIAN_POINT('Ctrl Pts',(-8.12422248499541,0.833362078616152,
-5.61594460317773));
#20688=CARTESIAN_POINT('Ctrl Pts',(-8.12472295983679,-0.000135441094342992,
-5.58329744321239));
#20689=CARTESIAN_POINT('Origin',(0.,0.,-16.4167025567876));
#20690=CARTESIAN_POINT('',(4.94675008185375,-6.44587862049697,-8.87494907190769));
#20691=CARTESIAN_POINT('',(4.94707560568286,-6.44630337360393,-8.7083535696852));
#20692=CARTESIAN_POINT('',(4.94675008185374,-6.44587862049697,-16.4167025567876));
#20693=CARTESIAN_POINT('',(-8.12525269526789,0.000111890383953636,-7.41670255678762));
#20694=CARTESIAN_POINT('Ctrl Pts',(4.94707560569883,-6.44630337359169,-8.70835356968441));
#20695=CARTESIAN_POINT('Ctrl Pts',(5.04438551388885,-6.37173728721331,-8.70354988872961));
#20696=CARTESIAN_POINT('Ctrl Pts',(6.18791126886723,-5.45321389914109,-8.64608986546737));
#20697=CARTESIAN_POINT('Ctrl Pts',(7.8789657040664,-3.09864722800698,-8.5359734998977));
#20698=CARTESIAN_POINT('Ctrl Pts',(8.40389718874569,1.02675569189956,-8.37800447297542));
#20699=CARTESIAN_POINT('Ctrl Pts',(6.90118083796468,4.90442843270839,-8.22003544605311));
#20700=CARTESIAN_POINT('Ctrl Pts',(3.73338409962977,7.59878663829889,-8.06206641913084));
#20701=CARTESIAN_POINT('Ctrl Pts',(-0.335183795052036,8.45974982096853,
-7.90409739220853));
#20702=CARTESIAN_POINT('Ctrl Pts',(-4.32288031764655,7.27958934069048,-7.74612836528627));
#20703=CARTESIAN_POINT('Ctrl Pts',(-7.26757515637083,4.34304807207066,-7.58815933836395));
#20704=CARTESIAN_POINT('Ctrl Pts',(-8.09561982062734,1.57337616034462,-7.47835073553109));
#20705=CARTESIAN_POINT('Ctrl Pts',(-8.1258799154099,0.114850934707135,-7.42119847500564));
#20706=CARTESIAN_POINT('Ctrl Pts',(-8.12580188385528,0.000111897946662807,
-7.41670255678762));
#20707=CARTESIAN_POINT('Ctrl Pts',(-8.1252499992296,0.000111890346827312,
-7.41670255678762));
#20708=CARTESIAN_POINT('Ctrl Pts',(-8.12525288020884,-0.209098977576592,
-7.40850431079129));
#20709=CARTESIAN_POINT('Ctrl Pts',(-8.1171712012911,-0.418345744962354,
-7.40030606479496));
#20710=CARTESIAN_POINT('Ctrl Pts',(-8.101022710918,-0.626991706237579,-7.39210781879863));
#20711=CARTESIAN_POINT('Ctrl Pts',(-8.0848770728534,-0.835600814368282,
-7.38391102085881));
#20712=CARTESIAN_POINT('Ctrl Pts',(-8.06066749005515,-1.04360903066591,
-7.375714222919));
#20713=CARTESIAN_POINT('Ctrl Pts',(-8.02846370555508,-1.25038317770383,
-7.36751742497919));
#20714=CARTESIAN_POINT('Ctrl Pts',(-7.99625877375556,-1.45716469132523,
-7.35932033501836));
#20715=CARTESIAN_POINT('Ctrl Pts',(-7.95605911297337,-1.66271175218541,
-7.35112324505753));
#20716=CARTESIAN_POINT('Ctrl Pts',(-7.90798604134617,-1.86639876027982,
-7.34292615509671));
#20717=CARTESIAN_POINT('Ctrl Pts',(-7.85991515707825,-2.07007650046912,
-7.33472943810936));
#20718=CARTESIAN_POINT('Ctrl Pts',(-7.80397164799632,-2.27189406677244,
-7.32653272112201));
#20719=CARTESIAN_POINT('Ctrl Pts',(-7.74032753703739,-2.47123798568261,
-7.31833600413466));
#20720=CARTESIAN_POINT('Ctrl Pts',(-7.67666767317294,-2.67063124530748,
-7.3101372583326));
#20721=CARTESIAN_POINT('Ctrl Pts',(-7.60530348806353,-2.86754934899659,
-7.30193851253055));
#20722=CARTESIAN_POINT('Ctrl Pts',(-7.52645666268727,-3.06139472580561,
-7.29373976672849));
#20723=CARTESIAN_POINT('Ctrl Pts',(-7.4574760303618,-3.23098400986169,-7.28656693932545));
#20724=CARTESIAN_POINT('Ctrl Pts',(-7.38276901200279,-3.39822157489473,
-7.27939411192241));
#20725=CARTESIAN_POINT('Ctrl Pts',(-7.30251417390863,-3.56272007072735,
-7.27222128451937));
#20726=CARTESIAN_POINT('Ctrl Pts',(-7.21050320531049,-3.75131512984065,
-7.26399774544542));
#20727=CARTESIAN_POINT('Ctrl Pts',(-7.11116739137222,-3.93637449756095,
-7.25577420637147));
#20728=CARTESIAN_POINT('Ctrl Pts',(-7.00480384180409,-4.11733053085936,
-7.24755066729751));
#20729=CARTESIAN_POINT('Ctrl Pts',(-6.89845963097652,-4.2982536632082,-7.23932862340579));
#20730=CARTESIAN_POINT('Ctrl Pts',(-6.78509038416978,-4.47507469604229,
-7.23110657951406));
#20731=CARTESIAN_POINT('Ctrl Pts',(-6.66503838876746,-4.6472519663513,-7.22288453562233));
#20732=CARTESIAN_POINT('Ctrl Pts',(-6.54499964805273,-4.81941022693107,
-7.21466339950913));
#20733=CARTESIAN_POINT('Ctrl Pts',(-6.41827980041197,-4.98692550675144,
-7.20644226339592));
#20734=CARTESIAN_POINT('Ctrl Pts',(-6.28526402526786,-5.14928574611796,
-7.19822112728272));
#20735=CARTESIAN_POINT('Ctrl Pts',(-6.15223769996644,-5.31165886310043,
-7.18999933910942));
#20736=CARTESIAN_POINT('Ctrl Pts',(-6.01291463425759,-5.46887589283249,
-7.18177755093612));
#20737=CARTESIAN_POINT('Ctrl Pts',(-5.86772047478252,-5.6204576319298,-7.17355576276282));
#20738=CARTESIAN_POINT('Ctrl Pts',(-5.72252671818263,-5.77203895042811,
-7.16533399740279));
#20739=CARTESIAN_POINT('Ctrl Pts',(-5.57146210636364,-5.91798479844755,
-7.15711223204277));
#20740=CARTESIAN_POINT('Ctrl Pts',(-5.4149897149768,-6.05785225547764,-7.14889046668274));
#20741=CARTESIAN_POINT('Ctrl Pts',(-5.25848470169381,-6.19774887255069,
-7.14066698722112));
#20742=CARTESIAN_POINT('Ctrl Pts',(-5.09656987648587,-6.33156437045485,
-7.1324435077595));
#20743=CARTESIAN_POINT('Ctrl Pts',(-4.92974283735278,-6.45889488380706,
-7.12422002829788));
#20744=CARTESIAN_POINT('Ctrl Pts',(-4.86233853562022,-6.51034112649261,
-7.12089743806429));
#20745=CARTESIAN_POINT('Ctrl Pts',(-4.79413270582646,-6.56072918560938,
-7.1175748478307));
#20746=CARTESIAN_POINT('Ctrl Pts',(-4.72515962225625,-6.61003434988799,
-7.11425225759711));
#20747=CARTESIAN_POINT('Ctrl Pts',(-4.55444857818667,-6.73206653456559,
-7.10602871852314));
#20748=CARTESIAN_POINT('Ctrl Pts',(-4.37897986752514,-6.84750181985908,
-7.09780517944917));
#20749=CARTESIAN_POINT('Ctrl Pts',(-4.19928504217936,-6.9559825112653,-7.0895816403752));
#20750=CARTESIAN_POINT('Ctrl Pts',(-4.01962288847436,-7.06444347899736,
-7.08135959648349));
#20751=CARTESIAN_POINT('Ctrl Pts',(-3.83573640605279,-7.16595222421921,
-7.07313755259177));
#20752=CARTESIAN_POINT('Ctrl Pts',(-3.64818450392634,-7.26019540975391,
-7.06491550870006));
#20753=CARTESIAN_POINT('Ctrl Pts',(-3.46065330900949,-7.35442819009744,
-7.05669437258686));
#20754=CARTESIAN_POINT('Ctrl Pts',(-3.26945776577081,-7.44139687989461,
-7.04847323647366));
#20755=CARTESIAN_POINT('Ctrl Pts',(-3.07518040518192,-7.52083459717638,
-7.04025210036045));
#20756=CARTESIAN_POINT('Ctrl Pts',(-2.88088763546822,-7.60027861506721,
-7.03203031218717));
#20757=CARTESIAN_POINT('Ctrl Pts',(-2.68351283200177,-7.67219035286242,
-7.02380852401388));
#20758=CARTESIAN_POINT('Ctrl Pts',(-2.48365846649581,-7.73635108977764,
-7.01558673584059));
#20759=CARTESIAN_POINT('Ctrl Pts',(-2.28380465553227,-7.80051164866398,
-7.00736497048057));
#20760=CARTESIAN_POINT('Ctrl Pts',(-2.08147157793189,-7.85692116210695,
-6.99914320512054));
#20761=CARTESIAN_POINT('Ctrl Pts',(-1.87727734289502,-7.90541063704808,
-6.99092143976052));
#20762=CARTESIAN_POINT('Ctrl Pts',(-1.67304053675,-7.95391022123976,-6.9826979602989));
#20763=CARTESIAN_POINT('Ctrl Pts',(-1.46694208501947,-7.99448640015824,
-6.97447448083729));
#20764=CARTESIAN_POINT('Ctrl Pts',(-1.25961185836555,-8.02702096227267,
-6.96625100137568));
#20765=CARTESIAN_POINT('Ctrl Pts',(-1.17584276896352,-8.04016613018381,
-6.96292841114206));
#20766=CARTESIAN_POINT('Ctrl Pts',(-1.09187270262411,-8.05199912128946,
-6.95960582090843));
#20767=CARTESIAN_POINT('Ctrl Pts',(-1.00774356520918,-8.06251452521355,
-6.95628323067481));
#20768=CARTESIAN_POINT('Ctrl Pts',(-0.799520702880655,-8.08854055580051,
-6.94805969160085));
#20769=CARTESIAN_POINT('Ctrl Pts',(-0.590255257323399,-8.10650014398112,
-6.93983615252689));
#20770=CARTESIAN_POINT('Ctrl Pts',(-0.380584972611504,-8.11633184641451,
-6.93161261345293));
#20771=CARTESIAN_POINT('Ctrl Pts',(-0.170952809599473,-8.1261617612736,
-6.92339056956122));
#20772=CARTESIAN_POINT('Ctrl Pts',(0.0390837511913653,-8.1278667260791,
-6.91516852566952));
#20773=CARTESIAN_POINT('Ctrl Pts',(0.248884029729575,-8.12143732982319,
-6.90694648177781));
#20774=CARTESIAN_POINT('Ctrl Pts',(0.458661144662935,-8.11500864342331,
-6.89872534566457));
#20775=CARTESIAN_POINT('Ctrl Pts',(0.668201734744688,-8.10044739801135,
-6.89050420955133));
#20776=CARTESIAN_POINT('Ctrl Pts',(0.876866467443997,-8.07779628121261,
-6.8822830734381));
#20777=CARTESIAN_POINT('Ctrl Pts',(1.08554775040333,-8.05514336783872,-6.87406128526479));
#20778=CARTESIAN_POINT('Ctrl Pts',(1.29335274366877,-8.02439933020023,-6.86583949709148));
#20779=CARTESIAN_POINT('Ctrl Pts',(1.49964751164141,-7.98565870190604,-6.85761770891817));
#20780=CARTESIAN_POINT('Ctrl Pts',(1.70594170720096,-7.94691818110679,-6.84939594355814));
#20781=CARTESIAN_POINT('Ctrl Pts',(1.91072539648266,-7.90018117112124,-6.8411741781981));
#20782=CARTESIAN_POINT('Ctrl Pts',(2.11337457085352,-7.84559338009367,-6.83295241283807));
#20783=CARTESIAN_POINT('Ctrl Pts',(2.31606599421294,-7.79099420841792,-6.82472893337645));
#20784=CARTESIAN_POINT('Ctrl Pts',(2.51662172882447,-7.72854106265373,-6.81650545391484));
#20785=CARTESIAN_POINT('Ctrl Pts',(2.71443160322337,-7.65842990657499,-6.80828197445322));
#20786=CARTESIAN_POINT('Ctrl Pts',(2.79435411775613,-7.63010240316981,-6.80495938421965));
#20787=CARTESIAN_POINT('Ctrl Pts',(2.87382856745068,-7.60052532479736,-6.80163679398608));
#20788=CARTESIAN_POINT('Ctrl Pts',(2.95281552569261,-7.56971386736174,-6.79831420375251));
#20789=CARTESIAN_POINT('Ctrl Pts',(3.14831395442207,-7.49345328397432,-6.79009055285581));
#20790=CARTESIAN_POINT('Ctrl Pts',(3.34088825448533,-7.40960273717027,-6.78186690195911));
#20791=CARTESIAN_POINT('Ctrl Pts',(3.52994833722337,-7.31841187000527,-6.7736432510624));
#20792=CARTESIAN_POINT('Ctrl Pts',(3.71897116032074,-7.2272389745818,-6.76542122086888));
#20793=CARTESIAN_POINT('Ctrl Pts',(3.90448088313136,-7.12872877469039,-6.75719919067535));
#20794=CARTESIAN_POINT('Ctrl Pts',(4.08590963763387,-7.023178055239,-6.74897716048182));
#20795=CARTESIAN_POINT('Ctrl Pts',(4.26732931736639,-6.9176326152622,-6.74075554154082));
#20796=CARTESIAN_POINT('Ctrl Pts',(4.44466818034,-6.80504750518394,-6.73253392259982));
#20797=CARTESIAN_POINT('Ctrl Pts',(4.61738425291033,-6.68576474484974,-6.72431230365881));
#20798=CARTESIAN_POINT('Ctrl Pts',(4.72915507392777,-6.60857255388933,-6.71899179650824));
#20799=CARTESIAN_POINT('Ctrl Pts',(4.83899047307838,-6.52857640072433,-6.71367128935767));
#20800=CARTESIAN_POINT('Ctrl Pts',(4.94675008185374,-6.44587862049698,-6.70835078220711));
#20801=CARTESIAN_POINT('',(-8.12530198328732,-5.60780087209094E-5,-7.58329744321239));
#20802=CARTESIAN_POINT('Ctrl Pts',(-8.125900459786,-5.60821392014618E-5,
-7.58329744321239));
#20803=CARTESIAN_POINT('Ctrl Pts',(-8.12592100724276,-0.0547552239322313,
-7.58115404420023));
#20804=CARTESIAN_POINT('Ctrl Pts',(-8.11209200002685,-1.4532239507054,-7.52635430288063));
#20805=CARTESIAN_POINT('Ctrl Pts',(-7.36207492018725,-4.18085733783256,
-7.41889821925358));
#20806=CARTESIAN_POINT('Ctrl Pts',(-4.48320742627557,-7.18196117942933,
-7.2609291923313));
#20807=CARTESIAN_POINT('Ctrl Pts',(-0.522655372263062,-8.45023943871622,
-7.10296016540901));
#20808=CARTESIAN_POINT('Ctrl Pts',(2.80584571694962,-7.82264088224354,-6.97429748063182));
#20809=CARTESIAN_POINT('Ctrl Pts',(4.47352363566336,-6.80846089037195,-6.89829113816206));
#20810=CARTESIAN_POINT('Ctrl Pts',(4.94635656996294,-6.445366250073,-6.87494113799973));
#20811=CARTESIAN_POINT('Ctrl Pts',(4.94675008185375,-6.44587862049697,-8.87494907190769));
#20812=CARTESIAN_POINT('Ctrl Pts',(5.11327935064553,-6.31807933625242,-8.86672559489486));
#20813=CARTESIAN_POINT('Ctrl Pts',(5.27483796520581,-6.18383505470868,-8.85850211788203));
#20814=CARTESIAN_POINT('Ctrl Pts',(5.43093669428508,-6.04355972793914,-8.8502786408692));
#20815=CARTESIAN_POINT('Ctrl Pts',(5.49205381107422,-5.98863792569657,-8.84705891443087));
#20816=CARTESIAN_POINT('Ctrl Pts',(5.55233432452382,-5.93279202427241,-8.84383918799255));
#20817=CARTESIAN_POINT('Ctrl Pts',(5.61175033476285,-5.87604848029601,-8.84061946155422));
#20818=CARTESIAN_POINT('Ctrl Pts',(5.76350542534024,-5.73111916543326,-8.83239592255661));
#20819=CARTESIAN_POINT('Ctrl Pts',(5.90966773813315,-5.58028431867139,-8.82417238355901));
#20820=CARTESIAN_POINT('Ctrl Pts',(6.04978663715039,-5.42399937384368,-8.8159488445614));
#20821=CARTESIAN_POINT('Ctrl Pts',(6.18988006009988,-5.26774284435372,-8.80772680074709));
#20822=CARTESIAN_POINT('Ctrl Pts',(6.32393206556385,-5.10603841405696,-8.79950475693277));
#20823=CARTESIAN_POINT('Ctrl Pts',(6.45153048813366,-4.93937667354716,-8.79128271311846));
#20824=CARTESIAN_POINT('Ctrl Pts',(6.57911482282054,-4.77273333382196,-8.78306157708332));
#20825=CARTESIAN_POINT('Ctrl Pts',(6.70024681792474,-4.60113401069098,-8.77484044104818));
#20826=CARTESIAN_POINT('Ctrl Pts',(6.81455553689492,-4.42510117365409,-8.76661930501304));
#20827=CARTESIAN_POINT('Ctrl Pts',(6.92887332226324,-4.24905437456951,-8.75839751691835));
#20828=CARTESIAN_POINT('Ctrl Pts',(7.03636658730184,-4.06857360488389,-8.75017572882365));
#20829=CARTESIAN_POINT('Ctrl Pts',(7.13670798750923,-3.88420991496622,-8.74195394072896));
#20830=CARTESIAN_POINT('Ctrl Pts',(7.23704910929327,-3.69984673661364,-8.73373217544775));
#20831=CARTESIAN_POINT('Ctrl Pts',(7.33023826732112,-3.51160091992,-8.72551041016656));
#20832=CARTESIAN_POINT('Ctrl Pts',(7.41599405146985,-3.32004816095548,-8.71728864488535));
#20833=CARTESIAN_POINT('Ctrl Pts',(7.50176771427936,-3.12845546641303,-8.70906516550225));
#20834=CARTESIAN_POINT('Ctrl Pts',(7.58010478674925,-2.93355472152726,-8.70084168611915));
#20835=CARTESIAN_POINT('Ctrl Pts',(7.65077155198343,-2.73594265690293,-8.69261820673605));
#20836=CARTESIAN_POINT('Ctrl Pts',(7.67932354635531,-2.65610005284044,-8.68929561603467));
#20837=CARTESIAN_POINT('Ctrl Pts',(7.70662394838959,-2.57581504928362,-8.68597302533329));
#20838=CARTESIAN_POINT('Ctrl Pts',(7.73265961988366,-2.49512780544818,-8.68265043463192));
#20839=CARTESIAN_POINT('Ctrl Pts',(7.79709890303887,-2.2954237896056,-8.67442689551314));
#20840=CARTESIAN_POINT('Ctrl Pts',(7.85380817147139,-2.09318968547407,-8.66620335639438));
#20841=CARTESIAN_POINT('Ctrl Pts',(7.90260800874881,-1.88904055609168,-8.65797981727561));
#20842=CARTESIAN_POINT('Ctrl Pts',(7.95139897337147,-1.68492854455323,-8.64975777333853));
#20843=CARTESIAN_POINT('Ctrl Pts',(7.99228330852968,-1.47890248941189,-8.64153572940146));
#20844=CARTESIAN_POINT('Ctrl Pts',(8.02513216736883,-1.2715900513774,-8.63331368546439));
#20845=CARTESIAN_POINT('Ctrl Pts',(8.05797739943628,-1.06430050226239,-8.62509254930547));
#20846=CARTESIAN_POINT('Ctrl Pts',(8.08278888026715,-0.855725144992614,
-8.61687141314655));
#20847=CARTESIAN_POINT('Ctrl Pts',(8.09948919734929,-0.646500042167216,
-8.60865027698762));
#20848=CARTESIAN_POINT('Ctrl Pts',(8.11619083901902,-0.437258344628318,
-8.60042848876833));
#20849=CARTESIAN_POINT('Ctrl Pts',(8.12478000538259,-0.227367092360067,
-8.59220670054903));
#20850=CARTESIAN_POINT('Ctrl Pts',(8.12523122600442,-0.0174667244402944,
-8.58398491232973));
#20851=CARTESIAN_POINT('Ctrl Pts',(8.12568244537425,0.192433061064505,-8.5757631469236));
#20852=CARTESIAN_POINT('Ctrl Pts',(8.11799576623392,0.402341667233051,-8.56754138151748));
#20853=CARTESIAN_POINT('Ctrl Pts',(8.10219784624027,0.611618854254461,-8.55931961611135));
#20854=CARTESIAN_POINT('Ctrl Pts',(8.08639663264302,0.820939672089145,-8.55109613660386));
#20855=CARTESIAN_POINT('Ctrl Pts',(8.0624808221466,1.02962851364811,-8.54287265709637));
#20856=CARTESIAN_POINT('Ctrl Pts',(8.03052902769919,1.23704935139254,-8.53464917758888));
#20857=CARTESIAN_POINT('Ctrl Pts',(8.01761932064266,1.32085504365521,-8.53132658762913));
#20858=CARTESIAN_POINT('Ctrl Pts',(8.00339836093629,1.40445381659858,-8.52800399766938));
#20859=CARTESIAN_POINT('Ctrl Pts',(7.98787371724669,1.48780409994712,-8.52468140770963));
#20860=CARTESIAN_POINT('Ctrl Pts',(7.94944962182064,1.69409928489361,-8.51645786865599));
#20861=CARTESIAN_POINT('Ctrl Pts',(7.90302333210066,1.89893866810336,-8.50823432960235));
#20862=CARTESIAN_POINT('Ctrl Pts',(7.84872993986047,2.10169595651651,-8.50001079054871));
#20863=CARTESIAN_POINT('Ctrl Pts',(7.79444641910373,2.30441638012652,-8.49178874667757));
#20864=CARTESIAN_POINT('Ctrl Pts',(7.73229872694468,2.50505517974816,-8.48356670280642));
#20865=CARTESIAN_POINT('Ctrl Pts',(7.66247242256954,2.70299906323721,-8.47534465893528));
#20866=CARTESIAN_POINT('Ctrl Pts',(7.59265382757021,2.90092109215727,-8.46712352284276));
#20867=CARTESIAN_POINT('Ctrl Pts',(7.51515841099195,3.09614852094415,-8.45890238675023));
#20868=CARTESIAN_POINT('Ctrl Pts',(7.43022096204239,3.28808515974356,-8.45068125065771));
#20869=CARTESIAN_POINT('Ctrl Pts',(7.34527677627344,3.48003702201021,-8.44245946250523));
#20870=CARTESIAN_POINT('Ctrl Pts',(7.25288949566177,3.66869730198269,-8.43423767435275));
#20871=CARTESIAN_POINT('Ctrl Pts',(7.15334166920894,3.85349069365154,-8.42601588620027));
#20872=CARTESIAN_POINT('Ctrl Pts',(7.05379411897472,4.03828357256813,-8.41779412086105));
#20873=CARTESIAN_POINT('Ctrl Pts',(6.94708620489238,4.21920932626937,-8.40957235552184));
#20874=CARTESIAN_POINT('Ctrl Pts',(6.83354622057933,4.39571764490235,-8.40135059018262));
#20875=CARTESIAN_POINT('Ctrl Pts',(6.71998256506317,4.57226276259153,-8.39312711074173));
#20876=CARTESIAN_POINT('Ctrl Pts',(6.59958415341269,4.74438835730398,-8.38490363130084));
#20877=CARTESIAN_POINT('Ctrl Pts',(6.47272296110334,4.91157256195056,-8.37668015185995));
#20878=CARTESIAN_POINT('Ctrl Pts',(6.42146633945766,4.97912117446721,-8.37335756150241));
#20879=CARTESIAN_POINT('Ctrl Pts',(6.36915517613709,5.04586347326246,-8.37003497114487));
#20880=CARTESIAN_POINT('Ctrl Pts',(6.31581592055058,5.11176650681736,-8.36671238078733));
#20881=CARTESIAN_POINT('Ctrl Pts',(6.18379920899772,5.27487905264517,-8.35848884170685));
#20882=CARTESIAN_POINT('Ctrl Pts',(6.04543885049741,5.4329011548279,-8.35026530262637));
#20883=CARTESIAN_POINT('Ctrl Pts',(5.90115185080704,5.58534639894578,-8.34204176354589));
#20884=CARTESIAN_POINT('Ctrl Pts',(5.75689108499793,5.73776392587195,-8.33381971964757));
#20885=CARTESIAN_POINT('Ctrl Pts',(5.60670603133728,5.88460640440353,-8.32559767574925));
#20886=CARTESIAN_POINT('Ctrl Pts',(5.45105188431948,6.02542288283213,-8.31737563185093));
#20887=CARTESIAN_POINT('Ctrl Pts',(5.29541492274622,6.16622381401174,-8.30915449573105));
#20888=CARTESIAN_POINT('Ctrl Pts',(5.13431029197106,6.3009998755828,-8.30093335961117));
#20889=CARTESIAN_POINT('Ctrl Pts',(4.96822833422969,6.42933859595661,-8.2927122234913));
#20890=CARTESIAN_POINT('Ctrl Pts',(4.80213320368471,6.55768749552617,-8.28449043531136));
#20891=CARTESIAN_POINT('Ctrl Pts',(4.63106018913466,6.67959785127481,-8.27626864713142));
#20892=CARTESIAN_POINT('Ctrl Pts',(4.45553168709605,6.79469829703888,-8.26804685895148));
#20893=CARTESIAN_POINT('Ctrl Pts',(4.28000367210317,6.90979842342928,-8.25982509358486));
#20894=CARTESIAN_POINT('Ctrl Pts',(4.10002044246582,7.01808851816036,-8.25160332821823));
#20895=CARTESIAN_POINT('Ctrl Pts',(3.91613271882103,7.11924097717442,-8.2433815628516));
#20896=CARTESIAN_POINT('Ctrl Pts',(3.73220665763841,7.22041452479705,-8.23515808338338));
#20897=CARTESIAN_POINT('Ctrl Pts',(3.54437473472822,7.31444732177401,-8.22693460391516));
#20898=CARTESIAN_POINT('Ctrl Pts',(3.35321253982474,7.40105757478363,-8.21871112444694));
#20899=CARTESIAN_POINT('Ctrl Pts',(3.27597593496695,7.4360513238966,-8.21538853425297));
#20900=CARTESIAN_POINT('Ctrl Pts',(3.19819593401293,7.46983390815843,-8.21206594405901));
#20901=CARTESIAN_POINT('Ctrl Pts',(3.11991148553179,7.50238894519251,-8.20874335386504));
#20902=CARTESIAN_POINT('Ctrl Pts',(2.92615445160806,7.58296391937171,-8.20051981479161));
#20903=CARTESIAN_POINT('Ctrl Pts',(2.72924287970012,7.65604200333074,-8.19229627571818));
#20904=CARTESIAN_POINT('Ctrl Pts',(2.5297750766031,7.7213940207904,-8.18407273664475));
#20905=CARTESIAN_POINT('Ctrl Pts',(2.3303435402179,7.78673415611797,-8.17585069275358));
#20906=CARTESIAN_POINT('Ctrl Pts',(2.12835698040241,7.84435093685115,-8.16762864886241));
#20907=CARTESIAN_POINT('Ctrl Pts',(1.92443040003701,7.89406455496238,-8.15940660497124));
#20908=CARTESIAN_POINT('Ctrl Pts',(1.7205263347752,7.94377268429789,-8.15118546885859));
#20909=CARTESIAN_POINT('Ctrl Pts',(1.51468296302451,7.98557932324147,-8.14296433274595));
#20910=CARTESIAN_POINT('Ctrl Pts',(1.3075278728656,8.01935523743521,-8.13474319663331));
#20911=CARTESIAN_POINT('Ctrl Pts',(1.10035635218153,8.05313383056872,-8.12652140846049));
#20912=CARTESIAN_POINT('Ctrl Pts',(0.891873195882433,8.07888037617433,-8.11829962028767));
#20913=CARTESIAN_POINT('Ctrl Pts',(0.682714606929592,8.09651704919992,-8.11007783211486));
#20914=CARTESIAN_POINT('Ctrl Pts',(0.473556598334639,8.11415367328857,-8.10185606675525));
#20915=CARTESIAN_POINT('Ctrl Pts',(0.263723454950581,8.1236804477162,-8.09363430139565));
#20916=CARTESIAN_POINT('Ctrl Pts',(0.0538554494699272,8.12507151679678,
-8.08541253603605));
#20917=CARTESIAN_POINT('Ctrl Pts',(-0.156056310004045,8.12646287589216,
-8.07718905657493));
#20918=CARTESIAN_POINT('Ctrl Pts',(-0.366002651115076,8.11971513924518,
-8.06896557711381));
#20919=CARTESIAN_POINT('Ctrl Pts',(-0.575343245118352,8.10485457690616,
-8.06074209765269));
#20920=CARTESIAN_POINT('Ctrl Pts',(-0.659924597459199,8.0988503594004,-8.05741950741604));
#20921=CARTESIAN_POINT('Ctrl Pts',(-0.74440709268594,8.09152234924638,-8.0540969171794));
#20922=CARTESIAN_POINT('Ctrl Pts',(-0.828748680368289,8.08287468585823,
-8.05077432694275));
#20923=CARTESIAN_POINT('Ctrl Pts',(-1.03749736508767,8.06147138521168,-8.04255078787003));
#20924=CARTESIAN_POINT('Ctrl Pts',(-1.24545036860925,8.03197355775538,-8.03432724879731));
#20925=CARTESIAN_POINT('Ctrl Pts',(-1.45197243939619,7.99446455978972,-8.02610370972459));
#20926=CARTESIAN_POINT('Ctrl Pts',(-1.65845696088148,7.95696238161177,-8.01788166583419));
#20927=CARTESIAN_POINT('Ctrl Pts',(-1.86351077885487,7.91145199275005,-8.0096596219438));
#20928=CARTESIAN_POINT('Ctrl Pts',(-2.06650746668915,7.85806811198643,-8.0014375780534));
#20929=CARTESIAN_POINT('Ctrl Pts',(-2.26948174208708,7.80469012522454,-7.99321644194153));
#20930=CARTESIAN_POINT('Ctrl Pts',(-2.47039905566403,7.74344045705942,-7.98499530582966));
#20931=CARTESIAN_POINT('Ctrl Pts',(-2.66864599462405,7.67450429134527,-7.9767741697178));
#20932=CARTESIAN_POINT('Ctrl Pts',(-2.86690865755784,7.60556265795295,-7.96855238154578));
#20933=CARTESIAN_POINT('Ctrl Pts',(-3.06250024322519,7.52893340323221,-7.96033059337377));
#20934=CARTESIAN_POINT('Ctrl Pts',(-3.25482424190259,7.44485102045858,-7.95210880520175));
#20935=CARTESIAN_POINT('Ctrl Pts',(-3.44714770693051,7.36076887099187,-7.94388703984308));
#20936=CARTESIAN_POINT('Ctrl Pts',(-3.63620333395049,7.26923375545565,-7.9356652744844));
#20937=CARTESIAN_POINT('Ctrl Pts',(-3.82141577982019,7.17052780485797,-7.92744350912573));
#20938=CARTESIAN_POINT('Ctrl Pts',(-4.0066668394108,7.07180127570786,-7.91922002966543));
#20939=CARTESIAN_POINT('Ctrl Pts',(-4.18807285687975,6.96590106365069,-7.91099655020514));
#20940=CARTESIAN_POINT('Ctrl Pts',(-4.36508325960138,6.85315516380942,-7.90277307074485));
#20941=CARTESIAN_POINT('Ctrl Pts',(-4.43660201751401,6.80760164496302,-7.89945048050339));
#20942=CARTESIAN_POINT('Ctrl Pts',(-4.50740351680724,6.76093110338285,-7.89612789026193));
#20943=CARTESIAN_POINT('Ctrl Pts',(-4.57745275089621,6.71316720153854,-7.89280530002047));
#20944=CARTESIAN_POINT('Ctrl Pts',(-4.75082730865321,6.59494970113748,-7.88458176094523));
#20945=CARTESIAN_POINT('Ctrl Pts',(-4.91964794377508,6.46999304191955,-7.87635822186999));
#20946=CARTESIAN_POINT('Ctrl Pts',(-5.08339573011157,6.33867300099819,-7.86813468279475));
#20947=CARTESIAN_POINT('Ctrl Pts',(-5.24711374425553,6.20737683634186,-7.8599126389018));
#20948=CARTESIAN_POINT('Ctrl Pts',(-5.40576052051277,6.06971978359707,-7.85169059500884));
#20949=CARTESIAN_POINT('Ctrl Pts',(-5.55884934941008,5.9261185841209,-7.84346855111588));
#20950=CARTESIAN_POINT('Ctrl Pts',(-5.71192127609631,5.78253323934689,-7.83524741500125));
#20951=CARTESIAN_POINT('Ctrl Pts',(-5.85943626550875,5.63300525978098,-7.82702627888662));
#20952=CARTESIAN_POINT('Ctrl Pts',(-6.00094308112869,5.47798956730968,-7.818805142772));
#20953=CARTESIAN_POINT('Ctrl Pts',(-6.14246112037178,5.3229615797577,-7.81058335459737));
#20954=CARTESIAN_POINT('Ctrl Pts',(-6.27796983284836,5.16244522565936,-7.80236156642275));
#20955=CARTESIAN_POINT('Ctrl Pts',(-6.40705632478139,4.99693073932177,-7.79413977824813));
#20956=CARTESIAN_POINT('Ctrl Pts',(-6.53614245853388,4.83141671224267,-7.78591801288677));
#20957=CARTESIAN_POINT('Ctrl Pts',(-6.65880622813568,4.66090481488924,-7.77769624752541));
#20958=CARTESIAN_POINT('Ctrl Pts',(-6.7746760357427,4.48591709388767,-7.76947448216406));
#20959=CARTESIAN_POINT('Ctrl Pts',(-6.8905700002809,4.31089289085146,-7.76125100270112));
#20960=CARTESIAN_POINT('Ctrl Pts',(-6.99966701034645,4.13139124598455,-7.75302752323819));
#20961=CARTESIAN_POINT('Ctrl Pts',(-7.10163908868174,3.94796274255566,-7.74480404377525));
#20962=CARTESIAN_POINT('Ctrl Pts',(-7.14283958444483,3.87385083465178,-7.74148145354956));
#20963=CARTESIAN_POINT('Ctrl Pts',(-7.18287747645796,3.79909818327198,-7.73815886332387));
#20964=CARTESIAN_POINT('Ctrl Pts',(-7.2217332481857,3.72374226478542,-7.73483627309817));
#20965=CARTESIAN_POINT('Ctrl Pts',(-7.31773817055224,3.53755270317142,-7.72662681019241));
#20966=CARTESIAN_POINT('Ctrl Pts',(-7.40655543191432,3.34761605895886,-7.71841734728665));
#20967=CARTESIAN_POINT('Ctrl Pts',(-7.48790814557763,3.15450775334158,-7.71020788438089));
#20968=CARTESIAN_POINT('Ctrl Pts',(-7.56924560136053,2.96143566561184,-7.70199996117796));
#20969=CARTESIAN_POINT('Ctrl Pts',(-7.64312118829713,2.765193377224,-7.69379203797503));
#20970=CARTESIAN_POINT('Ctrl Pts',(-7.70930583954445,2.56637702508145,-7.6855841147721));
#20971=CARTESIAN_POINT('Ctrl Pts',(-7.77803828579436,2.35990718683786,-7.67706022547546));
#20972=CARTESIAN_POINT('Ctrl Pts',(-7.83847581120739,2.15066149345176,-7.66853633617881));
#20973=CARTESIAN_POINT('Ctrl Pts',(-7.89041817182838,1.93932685130188,-7.66001244688217));
#20974=CARTESIAN_POINT('Ctrl Pts',(-7.94043323609318,1.73583367959891,-7.65180483240604));
#20975=CARTESIAN_POINT('Ctrl Pts',(-7.98257211352486,1.53040408927546,-7.6435972179299));
#20976=CARTESIAN_POINT('Ctrl Pts',(-8.01670761297762,1.32366408522956,-7.63538960345376));
#20977=CARTESIAN_POINT('Ctrl Pts',(-8.05084356618041,1.11692133306856,-7.62718187987697));
#20978=CARTESIAN_POINT('Ctrl Pts',(-8.07697588355815,0.908868425877369,
-7.61897415630018));
#20979=CARTESIAN_POINT('Ctrl Pts',(-8.09502886037525,0.700139494809234,
-7.61076643272339));
#20980=CARTESIAN_POINT('Ctrl Pts',(-8.11308536121284,0.491369818935635,
-7.60255710696286));
#20981=CARTESIAN_POINT('Ctrl Pts',(-8.12305934678764,0.281924151546433,
-7.59434778120232));
#20982=CARTESIAN_POINT('Ctrl Pts',(-8.12492707114278,0.0724406730452409,
-7.58613845544179));
#20983=CARTESIAN_POINT('Ctrl Pts',(-8.1251425264225,0.0482752648400622,
-7.58519145136532));
#20984=CARTESIAN_POINT('Ctrl Pts',(-8.12525016658789,0.0241093546043511,
-7.58424444728886));
#20985=CARTESIAN_POINT('Ctrl Pts',(-8.12524999980648,-5.6077649948665E-5,
-7.58329744321239));
#20986=CARTESIAN_POINT('Origin',(0.,0.,-16.4167025567876));
#20987=CARTESIAN_POINT('',(4.94701442880054,-6.44622255101802,-10.8749380057189));
#20988=CARTESIAN_POINT('',(4.94675008185374,-6.44587862049698,-10.708343763603));
#20989=CARTESIAN_POINT('',(4.94675008185374,-6.44587862049697,-16.4167025567876));
#20990=CARTESIAN_POINT('',(-8.12477737866023,-0.000175769160715919,-11.5832974432124));
#20991=CARTESIAN_POINT('Ctrl Pts',(-8.12477737866023,-0.000175769160715919,
-11.5832974432124));
#20992=CARTESIAN_POINT('Ctrl Pts',(-8.12510001228012,-0.486965488702826,
-11.5642292685526));
#20993=CARTESIAN_POINT('Ctrl Pts',(-7.96312717430326,-2.31779341310246,
-11.4925047515855));
#20994=CARTESIAN_POINT('Ctrl Pts',(-6.60455795380853,-5.2972113717909,-11.3681238923108));
#20995=CARTESIAN_POINT('Ctrl Pts',(-3.28552397693065,-7.80285054932884,
-11.2101548653885));
#20996=CARTESIAN_POINT('Ctrl Pts',(0.826182671114322,-8.42599612481988,
-11.0521858384663));
#20997=CARTESIAN_POINT('Ctrl Pts',(3.59360149709808,-7.42870399706383,-10.9404468852431));
#20998=CARTESIAN_POINT('Ctrl Pts',(4.81699001004096,-6.54618702099177,-10.8813642743273));
#20999=CARTESIAN_POINT('Ctrl Pts',(4.94701442880054,-6.44622255101802,-10.8749380057189));
#21000=CARTESIAN_POINT('',(-2.10208451021623,7.84862588447232,-12.));
#21001=CARTESIAN_POINT('Ctrl Pts',(-2.10208451021617,7.84862588447234,-12.));
#21002=CARTESIAN_POINT('Ctrl Pts',(-3.40044170599961,7.5008890207006,-11.9473436576926));
#21003=CARTESIAN_POINT('Ctrl Pts',(-5.82000697965988,6.14913288471193,-11.8420309730777));
#21004=CARTESIAN_POINT('Ctrl Pts',(-7.77710899046075,3.05948964104654,-11.7031301208152));
#21005=CARTESIAN_POINT('Ctrl Pts',(-8.1242090666793,0.85729354821751,-11.6168856108601));
#21006=CARTESIAN_POINT('Ctrl Pts',(-8.12477737866023,-0.000175769160715919,
-11.5832974432124));
#21007=CARTESIAN_POINT('',(2.10216660754842,7.84860389601923,-12.));
#21008=CARTESIAN_POINT('Origin',(0.,0.,-12.));
#21009=CARTESIAN_POINT('',(-8.12524999739639,-0.00020569387470909,-11.4167025567622));
#21010=CARTESIAN_POINT('Ctrl Pts',(2.10216660754842,7.84860389601924,-12.));
#21011=CARTESIAN_POINT('Ctrl Pts',(1.89996534114966,7.90276139407352,-11.9917970169686));
#21012=CARTESIAN_POINT('Ctrl Pts',(1.69563573139414,7.94911002038602,-11.9835940339371));
#21013=CARTESIAN_POINT('Ctrl Pts',(1.48979808132141,7.98750206506333,-11.9753910509057));
#21014=CARTESIAN_POINT('Ctrl Pts',(1.28399710640837,8.0258872692313,-11.9671895294422));
#21015=CARTESIAN_POINT('Ctrl Pts',(1.07668892013284,8.0563186665635,-11.9589880079787));
#21016=CARTESIAN_POINT('Ctrl Pts',(0.868503869052085,8.07869968447531,-11.9507864865152));
#21017=CARTESIAN_POINT('Ctrl Pts',(0.660311461804441,8.10108149321482,-11.942584675253));
#21018=CARTESIAN_POINT('Ctrl Pts',(0.451242423565235,8.11541231797868,-11.9343828639908));
#21019=CARTESIAN_POINT('Ctrl Pts',(0.241933137304118,8.12164736488689,-11.9261810527286));
#21020=CARTESIAN_POINT('Ctrl Pts',(0.0326345503735735,8.12788209307619,
-11.917979660721));
#21021=CARTESIAN_POINT('Ctrl Pts',(-0.176903962194337,8.12602186296263,
-11.9097782687135));
#21022=CARTESIAN_POINT('Ctrl Pts',(-0.386044600651898,8.11607399724815,
-11.9015768767059));
#21023=CARTESIAN_POINT('Ctrl Pts',(-0.59523794315302,8.10612362464284,-11.8933734179239));
#21024=CARTESIAN_POINT('Ctrl Pts',(-0.804032913327771,8.08808155585036,
-11.8851699591419));
#21025=CARTESIAN_POINT('Ctrl Pts',(-1.0117941832255,8.06200720002724,-11.87696650036));
#21026=CARTESIAN_POINT('Ctrl Pts',(-1.21139251650028,8.03695730518365,-11.8690853553286));
#21027=CARTESIAN_POINT('Ctrl Pts',(-1.41003656919329,8.00449424540528,-11.8612042102972));
#21028=CARTESIAN_POINT('Ctrl Pts',(-1.60716938183343,7.96471557185799,-11.8533230652658));
#21029=CARTESIAN_POINT('Ctrl Pts',(-1.81286241034718,7.92320956520887,-11.8450996925662));
#21030=CARTESIAN_POINT('Ctrl Pts',(-2.01698012426594,7.87372435936419,-11.8368763198665));
#21031=CARTESIAN_POINT('Ctrl Pts',(-2.21889834609129,7.8164043966656,-11.8286529471669));
#21032=CARTESIAN_POINT('Ctrl Pts',(-2.42077987259646,7.75909485092871,-11.8204310689302));
#21033=CARTESIAN_POINT('Ctrl Pts',(-2.62046242119952,7.69395347066466,-11.8122091906935));
#21034=CARTESIAN_POINT('Ctrl Pts',(-2.81733556906005,7.62117496543736,-11.8039873124568));
#21035=CARTESIAN_POINT('Ctrl Pts',(-3.01418701026522,7.54840448455439,-11.7957663407403));
#21036=CARTESIAN_POINT('Ctrl Pts',(-3.20822939259246,7.46799866205816,-11.7875453690237));
#21037=CARTESIAN_POINT('Ctrl Pts',(-3.39887013048231,7.38020117602597,-11.7793243973072));
#21038=CARTESIAN_POINT('Ctrl Pts',(-3.58952606142905,7.29239669299925,-11.7711027704227));
#21039=CARTESIAN_POINT('Ctrl Pts',(-3.77677953724081,7.19719949038884,-11.7628811435383));
#21040=CARTESIAN_POINT('Ctrl Pts',(-3.96005956871056,7.0949006881537,-11.7546595166538));
#21041=CARTESIAN_POINT('Ctrl Pts',(-4.14333913846275,6.99260214362888,-11.7464379104812));
#21042=CARTESIAN_POINT('Ctrl Pts',(-4.32264502766298,6.88320218138654,-11.7382163043087));
#21043=CARTESIAN_POINT('Ctrl Pts',(-4.49743192566566,6.76703728647207,-11.7299946981361));
#21044=CARTESIAN_POINT('Ctrl Pts',(-4.67225535284077,6.65084811395141,-11.7217713737084));
#21045=CARTESIAN_POINT('Ctrl Pts',(-4.84255765641126,6.52789134764352,-11.7135480492808));
#21046=CARTESIAN_POINT('Ctrl Pts',(-5.00782261952502,6.39854672358291,-11.7053247248532));
#21047=CARTESIAN_POINT('Ctrl Pts',(-5.07461657667055,6.34627043274828,-11.7020011626833));
#21048=CARTESIAN_POINT('Ctrl Pts',(-5.14058805180424,6.29295117663334,-11.6986776005134));
#21049=CARTESIAN_POINT('Ctrl Pts',(-5.20570446436953,6.2386159195885,-11.6953540383435));
#21050=CARTESIAN_POINT('Ctrl Pts',(-5.36681564989789,6.10417949513553,-11.6871308727809));
#21051=CARTESIAN_POINT('Ctrl Pts',(-5.52274263827381,5.96347680179788,-11.6789077072183));
#21052=CARTESIAN_POINT('Ctrl Pts',(-5.67300533197767,5.81693201489006,-11.6706845416556));
#21053=CARTESIAN_POINT('Ctrl Pts',(-5.82324059656644,5.67041397842659,-11.6624628771586));
#21054=CARTESIAN_POINT('Ctrl Pts',(-5.96781341907526,5.51805618270177,-11.6542412126615));
#21055=CARTESIAN_POINT('Ctrl Pts',(-6.10627973000892,5.36032045883287,-11.6460195481645));
#21056=CARTESIAN_POINT('Ctrl Pts',(-6.24473067440802,5.20260223995442,-11.6377987960806));
#21057=CARTESIAN_POINT('Ctrl Pts',(-6.3770762656581,5.03950750607002,-11.6295780439968));
#21058=CARTESIAN_POINT('Ctrl Pts',(-6.50291143441447,4.87153265807195,-11.6213572919129));
#21059=CARTESIAN_POINT('Ctrl Pts',(-6.62875652253558,4.70354456891244,-11.6131358918017));
#21060=CARTESIAN_POINT('Ctrl Pts',(-6.74808998373867,4.5306758314968,-11.6049144916904));
#21061=CARTESIAN_POINT('Ctrl Pts',(-6.86054832813189,4.35345428365415,-11.5966930915792));
#21062=CARTESIAN_POINT('Ctrl Pts',(-6.97300633836633,4.1762332624077,-11.588471715897));
#21063=CARTESIAN_POINT('Ctrl Pts',(-7.07858911687302,3.99465970711972,-11.5802503402148));
#21064=CARTESIAN_POINT('Ctrl Pts',(-7.17697735404496,3.80928912292382,-11.5720289645327));
#21065=CARTESIAN_POINT('Ctrl Pts',(-7.27538610556852,3.62387988819965,-11.5638058746599));
#21066=CARTESIAN_POINT('Ctrl Pts',(-7.36659718068259,3.4346723035936,-11.5555827847871));
#21067=CARTESIAN_POINT('Ctrl Pts',(-7.450337447084,3.24224605591215,-11.5473596949143));
#21068=CARTESIAN_POINT('Ctrl Pts',(-7.48419668434161,3.16444112102446,-11.5440348004166));
#21069=CARTESIAN_POINT('Ctrl Pts',(-7.51683507421775,3.08611022310206,-11.5407099059189));
#21070=CARTESIAN_POINT('Ctrl Pts',(-7.54823678541172,3.00729263522149,-11.5373850114212));
#21071=CARTESIAN_POINT('Ctrl Pts',(-7.62564901103827,2.8129896923448,-11.5291884045086));
#21072=CARTESIAN_POINT('Ctrl Pts',(-7.69556892011692,2.61566045847154,-11.520991797596));
#21073=CARTESIAN_POINT('Ctrl Pts',(-7.75777691501068,2.4159025020533,-11.5127951906835));
#21074=CARTESIAN_POINT('Ctrl Pts',(-7.81997745567985,2.21616848211898,-11.5045995659493));
#21075=CARTESIAN_POINT('Ctrl Pts',(-7.87446783475686,2.01400660477959,-11.4964039412151));
#21076=CARTESIAN_POINT('Ctrl Pts',(-7.92107800867631,1.81003059172064,-11.4882083164809));
#21077=CARTESIAN_POINT('Ctrl Pts',(-7.9676820176964,1.60608155756963,-11.4800137757418));
#21078=CARTESIAN_POINT('Ctrl Pts',(-8.00640783658789,1.40031915819125,-11.4718192350027));
#21079=CARTESIAN_POINT('Ctrl Pts',(-8.037136191185,1.19336893157322,-11.4636246942637));
#21080=CARTESIAN_POINT('Ctrl Pts',(-8.06786804751145,0.986395121405414,
-11.4554292196945));
#21081=CARTESIAN_POINT('Ctrl Pts',(-8.09060057175316,0.778233508789898,
-11.4472337451252));
#21082=CARTESIAN_POINT('Ctrl Pts',(-8.10526602692919,0.569517510887509,
-11.439038270556));
#21083=CARTESIAN_POINT('Ctrl Pts',(-8.11858896535206,0.379907958743068,
-11.4315930326332));
#21084=CARTESIAN_POINT('Ctrl Pts',(-8.1252548084907,0.189841129461651,-11.4241477947104));
#21085=CARTESIAN_POINT('Ctrl Pts',(-8.12524999739641,-0.000205693225322712,
-11.4167025567876));
#21086=CARTESIAN_POINT('Ctrl Pts',(-8.12524999739639,-0.000205693874714312,
-11.4167025567622));
#21087=CARTESIAN_POINT('Ctrl Pts',(-8.12524439842859,-0.221374229701558,
-11.4080381005666));
#21088=CARTESIAN_POINT('Ctrl Pts',(-8.11620418154541,-0.442498629493132,
-11.3993736443711));
#21089=CARTESIAN_POINT('Ctrl Pts',(-8.09816610723247,-0.662867454451679,
-11.3907091881756));
#21090=CARTESIAN_POINT('Ctrl Pts',(-8.090329198889,-0.758609951849022,-11.38694478695));
#21091=CARTESIAN_POINT('Ctrl Pts',(-8.08079452229166,-0.854209868966177,
-11.3831803857244));
#21092=CARTESIAN_POINT('Ctrl Pts',(-8.0695681467729,-0.949609123317658,
-11.3794159844989));
#21093=CARTESIAN_POINT('Ctrl Pts',(-8.04504425623296,-1.15800771709347,
-11.3711926925335));
#21094=CARTESIAN_POINT('Ctrl Pts',(-8.0124391408174,-1.36548973226526,-11.362969400568));
#21095=CARTESIAN_POINT('Ctrl Pts',(-7.97184563020018,-1.57142127093859,
-11.3547461086026));
#21096=CARTESIAN_POINT('Ctrl Pts',(-7.93125951566936,-1.77731528914547,
-11.3465243149106));
#21097=CARTESIAN_POINT('Ctrl Pts',(-7.8826879679138,-1.98165910542167,-11.3383025212187));
#21098=CARTESIAN_POINT('Ctrl Pts',(-7.826275041556,-2.1838284127691,-11.3300807275267));
#21099=CARTESIAN_POINT('Ctrl Pts',(-7.76986835938902,-2.38597534255496,
-11.3218598438823));
#21100=CARTESIAN_POINT('Ctrl Pts',(-7.70562211067602,-2.58594795993353,
-11.3136389602379));
#21101=CARTESIAN_POINT('Ctrl Pts',(-7.63373061504855,-2.78313572420937,
-11.3054180765935));
#21102=CARTESIAN_POINT('Ctrl Pts',(-7.56183343020747,-2.98033909315865,
-11.2971965423803));
#21103=CARTESIAN_POINT('Ctrl Pts',(-7.48228988812273,-3.17475689061642,
-11.2889750081672));
#21104=CARTESIAN_POINT('Ctrl Pts',(-7.39534335969,-3.36579621409095,-11.280753473954));
#21105=CARTESIAN_POINT('Ctrl Pts',(-7.30839707666393,-3.55683499835681,
-11.2725319629461));
#21106=CARTESIAN_POINT('Ctrl Pts',(-7.21404797372757,-3.74449506035948,
-11.2643104519382));
#21107=CARTESIAN_POINT('Ctrl Pts',(-7.11258673769472,-3.9282053741205,-11.2560889409303));
#21108=CARTESIAN_POINT('Ctrl Pts',(-7.01110433511271,-4.11195401299502,
-11.2478657147746));
#21109=CARTESIAN_POINT('Ctrl Pts',(-6.90250697803266,-4.2917509992888,-11.2396424886189));
#21110=CARTESIAN_POINT('Ctrl Pts',(-6.78713084177567,-4.46705076075004,
-11.2314192624633));
#21111=CARTESIAN_POINT('Ctrl Pts',(-6.74049196851533,-4.53791275719571,
-11.2280951608344));
#21112=CARTESIAN_POINT('Ctrl Pts',(-6.69274591559649,-4.60804020206745,
-11.2247710592055));
#21113=CARTESIAN_POINT('Ctrl Pts',(-6.64391690075673,-4.67739839850521,
-11.2214469575766));
#21114=CARTESIAN_POINT('Ctrl Pts',(-6.52311635522553,-4.84898711464533,
-11.2132232960612));
#21115=CARTESIAN_POINT('Ctrl Pts',(-6.39564537172317,-5.01592139574531,
-11.2049996345459));
#21116=CARTESIAN_POINT('Ctrl Pts',(-6.26188746879502,-5.17768798699264,
-11.1967759730305));
#21117=CARTESIAN_POINT('Ctrl Pts',(-6.12815386162119,-5.33942519499404,
-11.1885538052591));
#21118=CARTESIAN_POINT('Ctrl Pts',(-5.98813580207213,-5.49599635942735,
-11.1803316374877));
#21119=CARTESIAN_POINT('Ctrl Pts',(-5.84225728576869,-5.64692105216486,
-11.1721094697163));
#21120=CARTESIAN_POINT('Ctrl Pts',(-5.69639485706507,-5.79782910080615,
-11.1638882086922));
#21121=CARTESIAN_POINT('Ctrl Pts',(-5.54467346679687,-5.94309170897547,
-11.155666947668));
#21122=CARTESIAN_POINT('Ctrl Pts',(-5.38755475559963,-6.08226448930953,
-11.1474456866439));
#21123=CARTESIAN_POINT('Ctrl Pts',(-5.23042357122042,-6.22144831815209,
-11.1392237729586));
#21124=CARTESIAN_POINT('Ctrl Pts',(-5.06789442878962,-6.35454115563913,
-11.1310018592732));
#21125=CARTESIAN_POINT('Ctrl Pts',(-4.90046370332159,-6.48113748156353,
-11.1227799455879));
#21126=CARTESIAN_POINT('Ctrl Pts',(-4.73303344008498,-6.60773345798936,
-11.1145580546011));
#21127=CARTESIAN_POINT('Ctrl Pts',(-4.56070185774561,-6.72783278301322,
-11.1063361636142));
#21128=CARTESIAN_POINT('Ctrl Pts',(-4.38399652189535,-6.84107170394446,
-11.0981142726274));
#21129=CARTESIAN_POINT('Ctrl Pts',(-4.2072543601162,-6.95433422421087,-11.0898906681735));
#21130=CARTESIAN_POINT('Ctrl Pts',(-4.026136872252,-7.06073332504557,-11.0816670637196));
#21131=CARTESIAN_POINT('Ctrl Pts',(-3.84119950444942,-7.15994929657449,
-11.0734434592657));
#21132=CARTESIAN_POINT('Ctrl Pts',(-3.76649590213428,-7.20002659716805,
-11.0701216163953));
#21133=CARTESIAN_POINT('Ctrl Pts',(-3.69116931179321,-7.23893236081685,
-11.0667997735248));
#21134=CARTESIAN_POINT('Ctrl Pts',(-3.61525747148042,-7.27664764691853,
-11.0634779306543));
#21135=CARTESIAN_POINT('Ctrl Pts',(-3.42733150203513,-7.37001492235752,
-11.0552544369383));
#21136=CARTESIAN_POINT('Ctrl Pts',(-3.2357561229959,-7.45611344327543,-11.0470309432224));
#21137=CARTESIAN_POINT('Ctrl Pts',(-3.04111294558001,-7.53467448631497,
-11.0388074495064));
#21138=CARTESIAN_POINT('Ctrl Pts',(-2.8465051692872,-7.61322124090529,-11.030585451455));
#21139=CARTESIAN_POINT('Ctrl Pts',(-2.64883098161428,-7.68423314342852,
-11.0223634534037));
#21140=CARTESIAN_POINT('Ctrl Pts',(-2.44869195825795,-7.74748960993578,
-11.0141414553523));
#21141=CARTESIAN_POINT('Ctrl Pts',(-2.24857504002964,-7.81073908983809,
-11.0059203654113));
#21142=CARTESIAN_POINT('Ctrl Pts',(-2.04599411075093,-7.86623475500108,
-10.9976992754703));
#21143=CARTESIAN_POINT('Ctrl Pts',(-1.84156668959712,-7.91380563889879,
-10.9894781855293));
#21144=CARTESIAN_POINT('Ctrl Pts',(-1.63712305787383,-7.96138029504542,
-10.981256443677));
#21145=CARTESIAN_POINT('Ctrl Pts',(-1.43083292838439,-8.00102884486518,
-10.9730347018247));
#21146=CARTESIAN_POINT('Ctrl Pts',(-1.22332585827275,-8.03263103889263,
-10.9648129599724));
#21147=CARTESIAN_POINT('Ctrl Pts',(-1.01581936394145,-8.06423314523187,
-10.9565912409333));
#21148=CARTESIAN_POINT('Ctrl Pts',(-0.807096227725382,-8.08778889870032,
-10.9483695218943));
#21149=CARTESIAN_POINT('Ctrl Pts',(-0.597793547226755,-8.10322963005455,
-10.9401478028553));
#21150=CARTESIAN_POINT('Ctrl Pts',(-0.388447222788129,-8.11867358112079,
-10.9319243694177));
#21151=CARTESIAN_POINT('Ctrl Pts',(-0.178521406842369,-8.12599910793916,
-10.9237009359801));
#21152=CARTESIAN_POINT('Ctrl Pts',(0.0313432567839139,-8.12518954626624,
-10.9154775025425));
#21153=CARTESIAN_POINT('Ctrl Pts',(0.116143871679868,-8.12486242436551,
-10.9121546362724));
#21154=CARTESIAN_POINT('Ctrl Pts',(0.200934490792732,-8.12320764064176,
-10.9088317700022));
#21155=CARTESIAN_POINT('Ctrl Pts',(0.285672870119704,-8.12022651000436,
-10.905508903732));
#21156=CARTESIAN_POINT('Ctrl Pts',(0.495386426716496,-8.11284870181857,
-10.8972853560415));
#21157=CARTESIAN_POINT('Ctrl Pts',(0.704848081338482,-8.09734123816306,
-10.889061808351));
#21158=CARTESIAN_POINT('Ctrl Pts',(0.913418425414848,-8.07374475337267,
-10.8808382606605));
#21159=CARTESIAN_POINT('Ctrl Pts',(1.12195084923025,-8.05015255866898,-10.8726162080966));
#21160=CARTESIAN_POINT('Ctrl Pts',(1.32959199301364,-8.01847431125548,-10.8643941555327));
#21161=CARTESIAN_POINT('Ctrl Pts',(1.53570781418867,-7.97880248357733,-10.8561721029688));
#21162=CARTESIAN_POINT('Ctrl Pts',(1.74180087925786,-7.93913503584589,-10.8479509581562));
#21163=CARTESIAN_POINT('Ctrl Pts',(1.94636866842304,-7.8914758255043,-10.8397298133436));
#21164=CARTESIAN_POINT('Ctrl Pts',(2.14878674469931,-7.83596854819521,-10.831508668531));
#21165=CARTESIAN_POINT('Ctrl Pts',(2.35122087515886,-7.78045686849272,-10.8232868716829));
#21166=CARTESIAN_POINT('Ctrl Pts',(2.55150466691681,-7.7170959535628,-10.8150650748348));
#21167=CARTESIAN_POINT('Ctrl Pts',(2.74902724646548,-7.64607982960487,-10.8068432779868));
#21168=CARTESIAN_POINT('Ctrl Pts',(2.94654927721182,-7.57506390296015,-10.7986215039823));
#21169=CARTESIAN_POINT('Ctrl Pts',(3.14130983446964,-7.49639291215554,-10.7903997299779));
#21170=CARTESIAN_POINT('Ctrl Pts',(3.33271597406544,-7.41030983149214,-10.7821779559735));
#21171=CARTESIAN_POINT('Ctrl Pts',(3.52416201627601,-7.32420880500938,-10.7739544679683));
#21172=CARTESIAN_POINT('Ctrl Pts',(3.71225197479779,-7.23069272278405,-10.7657309799631));
#21173=CARTESIAN_POINT('Ctrl Pts',(3.89641454939461,-7.13005197889651,-10.7575074919578));
#21174=CARTESIAN_POINT('Ctrl Pts',(3.97082181093149,-7.08939006825532,-10.7541849535751));
#21175=CARTESIAN_POINT('Ctrl Pts',(4.04458823726234,-7.04756565169544,-10.7508624151925));
#21176=CARTESIAN_POINT('Ctrl Pts',(4.11767731770119,-7.0045999935606,-10.7475398768098));
#21177=CARTESIAN_POINT('Ctrl Pts',(4.29857842557853,-6.89825667783403,-10.7393163382075));
#21178=CARTESIAN_POINT('Ctrl Pts',(4.47538707246437,-6.78488440581811,-10.7310927996053));
#21179=CARTESIAN_POINT('Ctrl Pts',(4.64756033596046,-6.66482336495927,-10.722869261003));
#21180=CARTESIAN_POINT('Ctrl Pts',(4.74893203705017,-6.5941341551521,-10.7180274285364));
#21181=CARTESIAN_POINT('Ctrl Pts',(4.84869734040954,-6.52112707541245,-10.7131855960697));
#21182=CARTESIAN_POINT('Ctrl Pts',(4.94675008185374,-6.44587862049698,-10.7083437636031));
#21183=CARTESIAN_POINT('Origin',(0.,0.,0.));
#21184=CARTESIAN_POINT('',(-6.5722715952584,-2.44189939200198,11.3396960824468));
#21185=CARTESIAN_POINT('',(-6.5722717076903,-2.44189908939612,11.8869527148536));
#21186=CARTESIAN_POINT('',(-6.57227159525839,-2.441899392002,0.));
#21187=CARTESIAN_POINT('',(-5.31037376991248,-4.57794244025911,12.));
#21188=CARTESIAN_POINT('Ctrl Pts',(-6.57227170769031,-2.44189908939611,
11.8869527148536));
#21189=CARTESIAN_POINT('Ctrl Pts',(-6.48361520701476,-2.68051444153043,
11.8986804082385));
#21190=CARTESIAN_POINT('Ctrl Pts',(-6.38199333019113,-2.91422192491829,
11.9103615063067));
#21191=CARTESIAN_POINT('Ctrl Pts',(-6.18969751160504,-3.29782778585046,
11.9298963196887));
#21192=CARTESIAN_POINT('Ctrl Pts',(-6.10577998828279,-3.45072098239082,
11.9377875875726));
#21193=CARTESIAN_POINT('Ctrl Pts',(-5.80946526690376,-3.94587121303711,
11.9638060428799));
#21194=CARTESIAN_POINT('Ctrl Pts',(-5.57329951969572,-4.27295083686872,
11.9817184539604));
#21195=CARTESIAN_POINT('Ctrl Pts',(-5.31037376991251,-4.57794244025908,
12.));
#21196=CARTESIAN_POINT('',(5.31042129803496,-4.57788730746801,11.9999999751457));
#21197=CARTESIAN_POINT('Origin',(0.,0.,12.));
#21198=CARTESIAN_POINT('Ctrl Pts',(5.31042129803496,-4.57788730746801,11.9999999751457));
#21199=CARTESIAN_POINT('Ctrl Pts',(5.18805357552032,-4.71983579072877,11.9914889449188));
#21200=CARTESIAN_POINT('Ctrl Pts',(5.0599695362356,-4.85690008843993,11.9829779146919));
#21201=CARTESIAN_POINT('Ctrl Pts',(4.92658399091152,-4.9886267391933,11.974466884465));
#21202=CARTESIAN_POINT('Ctrl Pts',(4.79322289753619,-5.12032924210287,11.9659574144617));
#21203=CARTESIAN_POINT('Ctrl Pts',(4.65456245732618,-5.24669583361785,11.9574479444583));
#21204=CARTESIAN_POINT('Ctrl Pts',(4.51105444164968,-5.36730979047909,11.948938474455));
#21205=CARTESIAN_POINT('Ctrl Pts',(4.3675415572123,-5.48792783938017,11.940428715753));
#21206=CARTESIAN_POINT('Ctrl Pts',(4.21918100264951,-5.60279266164602,11.931918957051));
#21207=CARTESIAN_POINT('Ctrl Pts',(4.06645841569416,-5.71152716144554,11.9234091983491));
#21208=CARTESIAN_POINT('Ctrl Pts',(3.91374276690221,-5.82025672145363,11.9148998262441));
#21209=CARTESIAN_POINT('Ctrl Pts',(3.75666573453365,-5.92285633767202,11.9063904541391));
#21210=CARTESIAN_POINT('Ctrl Pts',(3.59574305338647,-6.01899148167889,11.8978810820341));
#21211=CARTESIAN_POINT('Ctrl Pts',(3.43478164633629,-6.11514976052439,11.8893696621562));
#21212=CARTESIAN_POINT('Ctrl Pts',(3.26997300630207,-6.204840299288,11.8808582422782));
#21213=CARTESIAN_POINT('Ctrl Pts',(3.10185952256609,-6.28777337892883,11.8723468224002));
#21214=CARTESIAN_POINT('Ctrl Pts',(2.97661014657212,-6.34956090627902,11.8660055700221));
#21215=CARTESIAN_POINT('Ctrl Pts',(2.84952692432497,-6.4075985053793,11.859664317644));
#21216=CARTESIAN_POINT('Ctrl Pts',(2.72084227075256,-6.46178333745307,11.8533230652658));
#21217=CARTESIAN_POINT('Ctrl Pts',(2.54769645008476,-6.53468928976913,11.8447908796742));
#21218=CARTESIAN_POINT('Ctrl Pts',(2.37158945434072,-6.60064426719468,11.8362586940826));
#21219=CARTESIAN_POINT('Ctrl Pts',(2.19309726907259,-6.65942572080254,11.827726508491));
#21220=CARTESIAN_POINT('Ctrl Pts',(2.01463849137951,-6.71819617255157,11.8191959198299));
#21221=CARTESIAN_POINT('Ctrl Pts',(1.83379570559365,-6.76979568421087,11.8106653311689));
#21222=CARTESIAN_POINT('Ctrl Pts',(1.65116165701798,-6.81405105241322,11.8021347425078));
#21223=CARTESIAN_POINT('Ctrl Pts',(1.46065319109038,-6.86021452724741,11.7932363504941));
#21224=CARTESIAN_POINT('Ctrl Pts',(1.26819591201722,-6.89838641697431,11.7843379584804));
#21225=CARTESIAN_POINT('Ctrl Pts',(1.07447724055565,-6.9284287700768,11.7754395664667));
#21226=CARTESIAN_POINT('Ctrl Pts',(0.888771302404243,-6.95722848940732,
11.7669092362488));
#21227=CARTESIAN_POINT('Ctrl Pts',(0.701906544640717,-6.97855761093532,
11.7583789060309));
#21228=CARTESIAN_POINT('Ctrl Pts',(0.514496804174811,-6.99234721685029,
11.749848575813));
#21229=CARTESIAN_POINT('Ctrl Pts',(0.327085093881319,-7.00613696770513,
11.7413181559344));
#21230=CARTESIAN_POINT('Ctrl Pts',(0.139128694855618,-7.01238702537379,
11.7327877360559));
#21231=CARTESIAN_POINT('Ctrl Pts',(-0.0487550931711929,-7.01108048045306,
11.7242573161773));
#21232=CARTESIAN_POINT('Ctrl Pts',(-0.236676153219624,-7.00977367634248,
11.7157252040506));
#21233=CARTESIAN_POINT('Ctrl Pts',(-0.424524267500988,-7.00090727872107,
11.7071930919239));
#21234=CARTESIAN_POINT('Ctrl Pts',(-0.611682912612513,-6.98451648841335,
11.6986609797971));
#21235=CARTESIAN_POINT('Ctrl Pts',(-0.635863040297116,-6.9823988656754,
11.6975586659792));
#21236=CARTESIAN_POINT('Ctrl Pts',(-0.660031664932469,-6.98015572005915,
11.6964563521614));
#21237=CARTESIAN_POINT('Ctrl Pts',(-0.6841874625102,-6.97778719069619,11.6953540383435));
#21238=CARTESIAN_POINT('Ctrl Pts',(-0.871154688398204,-6.95945464079793,
11.6868220676675));
#21239=CARTESIAN_POINT('Ctrl Pts',(-1.05741630635565,-6.93360008947338,
11.6782900969915));
#21240=CARTESIAN_POINT('Ctrl Pts',(-1.24235987700682,-6.90030205849741,
11.6697581263155));
#21241=CARTESIAN_POINT('Ctrl Pts',(-1.42726867797124,-6.86701028760446,
11.6612277596636));
#21242=CARTESIAN_POINT('Ctrl Pts',(-1.610859625064,-6.82627788391762,11.6526973930118));
#21243=CARTESIAN_POINT('Ctrl Pts',(-1.79252903411854,-6.77823474249322,
11.6441670263599));
#21244=CARTESIAN_POINT('Ctrl Pts',(-1.98203852750899,-6.7281182620158,11.635268525115));
#21245=CARTESIAN_POINT('Ctrl Pts',(-2.16945660525274,-6.67004611011735,
11.6263700238701));
#21246=CARTESIAN_POINT('Ctrl Pts',(-2.3541130366864,-6.60422428245764,11.6174715226253));
#21247=CARTESIAN_POINT('Ctrl Pts',(-2.53112450467776,-6.54112754518476,
11.6089414283521));
#21248=CARTESIAN_POINT('Ctrl Pts',(-2.7055980832415,-6.47091000800959,11.6004113340789));
#21249=CARTESIAN_POINT('Ctrl Pts',(-2.87696119327688,-6.39380331687478,
11.5918812398057));
#21250=CARTESIAN_POINT('Ctrl Pts',(-3.04832602678408,-6.31669585024511,
11.5833510597417));
#21251=CARTESIAN_POINT('Ctrl Pts',(-3.21658005149229,-6.23269921972729,
11.5748208796777));
#21252=CARTESIAN_POINT('Ctrl Pts',(-3.38117240538391,-6.14209245514673,
11.5662906996137));
#21253=CARTESIAN_POINT('Ctrl Pts',(-3.54579733378653,-6.05146775856034,
11.5577588313398));
#21254=CARTESIAN_POINT('Ctrl Pts',(-3.70675887635521,-5.95423046350902,
11.5492269630659));
#21255=CARTESIAN_POINT('Ctrl Pts',(-3.86353166493297,-5.85070505465455,
11.540695094792));
#21256=CARTESIAN_POINT('Ctrl Pts',(-3.88380588795173,-5.8373169070923,11.5395917336684));
#21257=CARTESIAN_POINT('Ctrl Pts',(-3.90401009570616,-5.82382365557448,
11.5384883725449));
#21258=CARTESIAN_POINT('Ctrl Pts',(-3.9241431869757,-5.8102260550354,11.5373850114213));
#21259=CARTESIAN_POINT('Ctrl Pts',(-4.07984083597495,-5.70507010021346,
11.5288522565334));
#21260=CARTESIAN_POINT('Ctrl Pts',(-4.23133535648263,-5.59363451442266,
11.5203195016455));
#21261=CARTESIAN_POINT('Ctrl Pts',(-4.37812552338029,-5.47628007538202,
11.5117867467576));
#21262=CARTESIAN_POINT('Ctrl Pts',(-4.5248882993246,-5.35894753460632,11.5032555840765));
#21263=CARTESIAN_POINT('Ctrl Pts',(-4.66694823463972,-5.23569853562443,
11.4947244213953));
#21264=CARTESIAN_POINT('Ctrl Pts',(-4.80383626920622,-5.10693485969411,
11.4861932587141));
#21265=CARTESIAN_POINT('Ctrl Pts',(-4.94661215011428,-4.97263278341599,
11.4772951525295));
#21266=CARTESIAN_POINT('Ctrl Pts',(-5.0837611095287,-4.83233136739081,11.4683970463449));
#21267=CARTESIAN_POINT('Ctrl Pts',(-5.21479200244674,-4.68653079939923,
11.4594989401603));
#21268=CARTESIAN_POINT('Ctrl Pts',(-5.34041562011959,-4.54674700947027,
11.4509680337118));
#21269=CARTESIAN_POINT('Ctrl Pts',(-5.46041576835826,-4.40190906956675,
11.4424371272633));
#21270=CARTESIAN_POINT('Ctrl Pts',(-5.57439918826281,-4.25249341591436,
11.4339062208148));
#21271=CARTESIAN_POINT('Ctrl Pts',(-5.68838378442128,-4.10307622036448,
11.4253752263315));
#21272=CARTESIAN_POINT('Ctrl Pts',(-5.79635134520065,-3.94908146185761,
11.4168442318482));
#21273=CARTESIAN_POINT('Ctrl Pts',(-5.89795027185349,-3.79101690226295,
11.4083132373648));
#21274=CARTESIAN_POINT('Ctrl Pts',(-5.99956928600698,-3.6329210911379,11.3997805561869));
#21275=CARTESIAN_POINT('Ctrl Pts',(-6.0948169865471,-3.47075412969225,11.391247875009));
#21276=CARTESIAN_POINT('Ctrl Pts',(-6.18338583687873,-3.30505161151647,
11.3827151938311));
#21277=CARTESIAN_POINT('Ctrl Pts',(-6.19480105215372,-3.28369500691449,
11.3816154573871));
#21278=CARTESIAN_POINT('Ctrl Pts',(-6.206105384523,-3.26227970605504,11.380515720943));
#21279=CARTESIAN_POINT('Ctrl Pts',(-6.21729823109895,-3.24080688534105,
11.379415984499));
#21280=CARTESIAN_POINT('Ctrl Pts',(-6.30401649225029,-3.07444297945732,
11.3708956111063));
#21281=CARTESIAN_POINT('Ctrl Pts',(-6.38406895189986,-2.90456677305934,
11.3623752377136));
#21282=CARTESIAN_POINT('Ctrl Pts',(-6.4571870356737,-2.73173244459035,11.3538548643209));
#21283=CARTESIAN_POINT('Ctrl Pts',(-6.49768850790942,-2.63599628200822,
11.3491352703629));
#21284=CARTESIAN_POINT('Ctrl Pts',(-6.53606315568444,-2.53935291514877,
11.3444156764049));
#21285=CARTESIAN_POINT('Ctrl Pts',(-6.5722715952584,-2.44189939200198,11.3396960824468));
#21286=CARTESIAN_POINT('Origin',(0.,0.,0.));
#21287=CARTESIAN_POINT('',(-6.57271212262447,-2.44206338026677,9.33970533813071));
#21288=CARTESIAN_POINT('',(-6.57227161595961,-2.44189933628552,9.88702363219766));
#21289=CARTESIAN_POINT('',(-6.57227159525839,-2.441899392002,0.));
#21290=CARTESIAN_POINT('Ctrl Pts',(-6.57227161595961,-2.44189933628553,
9.88702363219766));
#21291=CARTESIAN_POINT('Ctrl Pts',(-6.51762240584789,-2.58898543730319,
9.89408880535383));
#21292=CARTESIAN_POINT('Ctrl Pts',(-6.45804127549252,-2.73422160451104,
9.90112533428217));
#21293=CARTESIAN_POINT('Ctrl Pts',(-6.32050475483063,-3.03983391538899,
9.9161417230889));
#21294=CARTESIAN_POINT('Ctrl Pts',(-6.24121965749755,-3.19946044381868,
9.92411325297914));
#21295=CARTESIAN_POINT('Ctrl Pts',(-6.11223957183643,-3.43605736682013,
9.9362397569631));
#21296=CARTESIAN_POINT('Ctrl Pts',(-6.06697651764124,-3.51536036210359,
9.94035982170694));
#21297=CARTESIAN_POINT('Ctrl Pts',(-5.98324838294239,-3.65561982138901,
9.94776882569942));
#21298=CARTESIAN_POINT('Ctrl Pts',(-5.9453677641879,-3.71690992711833,9.95105047946258));
#21299=CARTESIAN_POINT('Ctrl Pts',(-5.75005793117126,-4.02229054076895,
9.96761214156557));
#21300=CARTESIAN_POINT('Ctrl Pts',(-5.57851329092103,-4.25701494818049,
9.98101286913493));
#21301=CARTESIAN_POINT('Ctrl Pts',(-5.25091078917215,-4.65133717236473,
10.0045529312005));
#21302=CARTESIAN_POINT('Ctrl Pts',(-5.10086799233868,-4.81540753602125,
10.0147087041653));
#21303=CARTESIAN_POINT('Ctrl Pts',(-4.79578592306985,-5.11872300716941,
10.0342419513189));
#21304=CARTESIAN_POINT('Ctrl Pts',(-4.6418321302037,-5.2587340838535,10.0436185698762));
#21305=CARTESIAN_POINT('Ctrl Pts',(-4.2556159616202,-5.57977871216393,10.0661751552068));
#21306=CARTESIAN_POINT('Ctrl Pts',(-4.01773809173377,-5.75343168441,10.079291564606));
#21307=CARTESIAN_POINT('Ctrl Pts',(-3.67642124952051,-5.97107872646848,
10.0975306483328));
#21308=CARTESIAN_POINT('Ctrl Pts',(-3.58179319708035,-6.0283174766224,10.1025332653719));
#21309=CARTESIAN_POINT('Ctrl Pts',(-3.31669639046982,-6.18022328041213,
10.1164484658459));
#21310=CARTESIAN_POINT('Ctrl Pts',(-3.14357478625064,-6.27005350110009,
10.1254083506845));
#21311=CARTESIAN_POINT('Ctrl Pts',(-2.7699440223517,-6.44455645268922,10.1443775580678));
#21312=CARTESIAN_POINT('Ctrl Pts',(-2.56877648051099,-6.52734911140884,
10.1543776019011));
#21313=CARTESIAN_POINT('Ctrl Pts',(-2.18760876375722,-6.66386780209054,
10.172901260487));
#21314=CARTESIAN_POINT('Ctrl Pts',(-2.00866512548279,-6.71997263185898,
10.1814318230404));
#21315=CARTESIAN_POINT('Ctrl Pts',(-1.57069367109145,-6.83823139087503,
10.2019655360749));
#21316=CARTESIAN_POINT('Ctrl Pts',(-1.30995575265783,-6.89293156931636,
10.213900741442));
#21317=CARTESIAN_POINT('Ctrl Pts',(-0.878476050524959,-6.95807903350122,
10.2334512641542));
#21318=CARTESIAN_POINT('Ctrl Pts',(-0.709346064056967,-6.97734989399436,
10.2410676747381));
#21319=CARTESIAN_POINT('Ctrl Pts',(-0.424049143539064,-6.99937568506481,
10.2539486733267));
#21320=CARTESIAN_POINT('Ctrl Pts',(-0.308212743978904,-7.00543234021471,
10.2591890117709));
#21321=CARTESIAN_POINT('Ctrl Pts',(-0.0264193122047767,-7.01316324078707,
10.2720173889338));
#21322=CARTESIAN_POINT('Ctrl Pts',(0.139547824788628,-7.01182443707065,
10.2796303008101));
#21323=CARTESIAN_POINT('Ctrl Pts',(0.541243966839384,-6.99431573436788,
10.2981157264964));
#21324=CARTESIAN_POINT('Ctrl Pts',(0.776510315685194,-6.97211808650129,
10.3089888385472));
#21325=CARTESIAN_POINT('Ctrl Pts',(1.2004806249356,-6.91038668517117,10.32860773548));
#21326=CARTESIAN_POINT('Ctrl Pts',(1.38953526965262,-6.87486663744936,10.337366492301));
#21327=CARTESIAN_POINT('Ctrl Pts',(1.95067873795822,-6.74534202977916,10.3634537381735));
#21328=CARTESIAN_POINT('Ctrl Pts',(2.31675378507399,-6.6285323656769,10.3805621416503));
#21329=CARTESIAN_POINT('Ctrl Pts',(2.7433928068384,-6.45271105158333,10.4012659490627));
#21330=CARTESIAN_POINT('Ctrl Pts',(2.81485236618666,-6.42186032725736,10.4047623547499));
#21331=CARTESIAN_POINT('Ctrl Pts',(2.98710269862579,-6.34406837018094,10.4132771180454));
#21332=CARTESIAN_POINT('Ctrl Pts',(3.08731764523307,-6.29590783916845,10.4183057844006));
#21333=CARTESIAN_POINT('Ctrl Pts',(3.36251317937058,-6.15550524957702,10.4323746978447));
#21334=CARTESIAN_POINT('Ctrl Pts',(3.53479713651178,-6.05821322771792,10.4414645134852));
#21335=CARTESIAN_POINT('Ctrl Pts',(3.88664415092642,-5.83939447952108,10.4605244610784));
#21336=CARTESIAN_POINT('Ctrl Pts',(4.06515577942432,-5.7165584402882,10.470485048554));
#21337=CARTESIAN_POINT('Ctrl Pts',(4.38687543276301,-5.47247791034489,10.4889598807142));
#21338=CARTESIAN_POINT('Ctrl Pts',(4.53146252602292,-5.35336711657016,10.4974807945599));
#21339=CARTESIAN_POINT('Ctrl Pts',(4.86244014367859,-5.05768000030014,10.517568447996));
#21340=CARTESIAN_POINT('Ctrl Pts',(5.04424571542985,-4.87637556642389,10.5290762249333));
#21341=CARTESIAN_POINT('Ctrl Pts',(5.33309355258108,-4.55484295693266,10.5484421446617));
#21342=CARTESIAN_POINT('Ctrl Pts',(5.44552842118192,-4.41980777611782,10.5563020944382));
#21343=CARTESIAN_POINT('Ctrl Pts',(5.62455298352339,-4.18758311307204,10.5694986651677));
#21344=CARTESIAN_POINT('Ctrl Pts',(5.69397864543999,-4.09268316264512,10.574809189654));
#21345=CARTESIAN_POINT('Ctrl Pts',(5.8870366916296,-3.81435938653101,10.5902206386414));
#21346=CARTESIAN_POINT('Ctrl Pts',(6.0044176776675,-3.62677611370168,10.6003915984051));
#21347=CARTESIAN_POINT('Ctrl Pts',(6.18450929334813,-3.30619818116145,10.6173072410649));
#21348=CARTESIAN_POINT('Ctrl Pts',(6.25226028079838,-3.17621524770333,10.6240471438371));
#21349=CARTESIAN_POINT('Ctrl Pts',(6.40518254887975,-2.85894354132475,10.640200270286));
#21350=CARTESIAN_POINT('Ctrl Pts',(6.48628323939134,-2.66984145280694,10.6495855553476));
#21351=CARTESIAN_POINT('Ctrl Pts',(6.70458493281666,-2.09189512656837,10.677608857111));
#21352=CARTESIAN_POINT('Ctrl Pts',(6.81593652484964,-1.69425410793386,10.6959802067608));
#21353=CARTESIAN_POINT('Ctrl Pts',(6.91991948936726,-1.13836269427626,10.7213591962988));
#21354=CARTESIAN_POINT('Ctrl Pts',(6.94316715844705,-0.986703622890623,
10.7282597266194));
#21355=CARTESIAN_POINT('Ctrl Pts',(6.97706241459874,-0.703916761765895,
10.7411871259644));
#21356=CARTESIAN_POINT('Ctrl Pts',(6.98903082294839,-0.573014812917868,
10.7471972471737));
#21357=CARTESIAN_POINT('Ctrl Pts',(7.0142992367176,-0.172859458991969,10.7655938370517));
#21358=CARTESIAN_POINT('Ctrl Pts',(7.01575989333482,0.0968931036385455,
10.7780201520149));
#21359=CARTESIAN_POINT('Ctrl Pts',(6.99120461956265,0.566566323511386,10.7995799439267));
#21360=CARTESIAN_POINT('Ctrl Pts',(6.97211369562239,0.766532399307416,10.8087374299901));
#21361=CARTESIAN_POINT('Ctrl Pts',(6.89084093122266,1.35115325549083,10.835499824254));
#21362=CARTESIAN_POINT('Ctrl Pts',(6.80516743311891,1.73176318492726,10.8528774873014));
#21363=CARTESIAN_POINT('Ctrl Pts',(6.65253299002974,2.21713180387593,10.8756986023177));
#21364=CARTESIAN_POINT('Ctrl Pts',(6.61383188627202,2.33004205718452,10.881059826954));
#21365=CARTESIAN_POINT('Ctrl Pts',(6.53593583032247,2.53969519001638,10.8911609701844));
#21366=CARTESIAN_POINT('Ctrl Pts',(6.49742638804987,2.63665673149079,10.8958964342839));
#21367=CARTESIAN_POINT('Ctrl Pts',(6.43397333021965,2.78658106661638,10.903327387717));
#21368=CARTESIAN_POINT('Ctrl Pts',(6.41050585578187,2.84015166289279,10.9060035418419));
#21369=CARTESIAN_POINT('Ctrl Pts',(6.30886895009647,3.06448498182338,10.9172924716424));
#21370=CARTESIAN_POINT('Ctrl Pts',(6.2245253379365,3.23236440123658,10.9259407930786));
#21371=CARTESIAN_POINT('Ctrl Pts',(6.01710439291466,3.60691695122986,10.9456273632757));
#21372=CARTESIAN_POINT('Ctrl Pts',(5.88992825716127,3.81105536776905,10.9566414549474));
#21373=CARTESIAN_POINT('Ctrl Pts',(5.64487538177079,4.16274687558152,10.9761461698522));
#21374=CARTESIAN_POINT('Ctrl Pts',(5.53105151068204,4.31283553272978,10.9846603269234));
#21375=CARTESIAN_POINT('Ctrl Pts',(5.27110849168164,4.62835474488067,11.003064908825));
#21376=CARTESIAN_POINT('Ctrl Pts',(5.12294230223431,4.79183839937538,11.0129301723434));
#21377=CARTESIAN_POINT('Ctrl Pts',(4.83664867131311,5.07924584703895,11.0311089472987));
#21378=CARTESIAN_POINT('Ctrl Pts',(4.70083553667646,5.20519475819294,11.0394115609546));
#21379=CARTESIAN_POINT('Ctrl Pts',(4.47787191605606,5.39611312201303,11.0527001027281));
#21380=CARTESIAN_POINT('Ctrl Pts',(4.39392325949565,5.46468767089453,11.0576373113752));
#21381=CARTESIAN_POINT('Ctrl Pts',(4.08061042854539,5.70873269425712,11.0758079697497));
#21382=CARTESIAN_POINT('Ctrl Pts',(3.84205659407507,5.87193422859419,11.089131372587));
#21383=CARTESIAN_POINT('Ctrl Pts',(3.41072574415941,6.12945339580312,11.112187510178));
#21384=CARTESIAN_POINT('Ctrl Pts',(3.2224210313739,6.23050992419217,11.1219433703731));
#21385=CARTESIAN_POINT('Ctrl Pts',(2.83684123565165,6.41527384596874,11.1413490694916));
#21386=CARTESIAN_POINT('Ctrl Pts',(2.63975436000385,6.49885417451629,11.1509885745107));
#21387=CARTESIAN_POINT('Ctrl Pts',(2.18345875332125,6.66817185658736,11.172837904468));
#21388=CARTESIAN_POINT('Ctrl Pts',(1.9224485876417,6.7480514094493,11.1850045331482));
#21389=CARTESIAN_POINT('Ctrl Pts',(1.54662906275811,6.83948637163849,11.2024213306914));
#21390=CARTESIAN_POINT('Ctrl Pts',(1.43516671663417,6.86374034430369,11.2075771295441));
#21391=CARTESIAN_POINT('Ctrl Pts',(1.11587999504838,6.92509861165761,11.2223769349407));
#21392=CARTESIAN_POINT('Ctrl Pts',(0.9069072500884,6.95555148905481,11.2320809534955));
#21393=CARTESIAN_POINT('Ctrl Pts',(0.391244118470795,7.00706081258822,11.2559179448643));
#21394=CARTESIAN_POINT('Ctrl Pts',(0.0839256937663981,7.01747353883307,
11.2700204760206));
#21395=CARTESIAN_POINT('Ctrl Pts',(-0.413636373146145,7.00163392910981,
11.292665735672));
#21396=CARTESIAN_POINT('Ctrl Pts',(-0.603861598999197,6.98779832665097,
11.3012831167896));
#21397=CARTESIAN_POINT('Ctrl Pts',(-1.01987667185492,6.94042407261498,11.3201271543642));
#21398=CARTESIAN_POINT('Ctrl Pts',(-1.24507170085294,6.90358108477314,11.3303252104165));
#21399=CARTESIAN_POINT('Ctrl Pts',(-1.64721206087191,6.81746889605279,11.3487590302395));
#21400=CARTESIAN_POINT('Ctrl Pts',(-1.82477901356867,6.77210230553286,11.3569804818862));
#21401=CARTESIAN_POINT('Ctrl Pts',(-2.11069775697616,6.68698991719773,11.3705028475107));
#21402=CARTESIAN_POINT('Ctrl Pts',(-2.22020526724276,6.65143344332621,11.3757565415309));
#21403=CARTESIAN_POINT('Ctrl Pts',(-2.48733894101406,6.55736440888498,11.3887319458267));
#21404=CARTESIAN_POINT('Ctrl Pts',(-2.64383223071761,6.49584742068739,11.3964699746497));
#21405=CARTESIAN_POINT('Ctrl Pts',(-3.04502846612994,6.32123662186997,11.4166011836916));
#21406=CARTESIAN_POINT('Ctrl Pts',(-3.28569351286677,6.19955261298194,11.4289646091));
#21407=CARTESIAN_POINT('Ctrl Pts',(-3.67912501766784,5.97126797665015,11.4496685080679));
#21408=CARTESIAN_POINT('Ctrl Pts',(-3.83573818057884,5.87189204844748,11.4580554812727));
#21409=CARTESIAN_POINT('Ctrl Pts',(-4.16331957965394,5.64532706820208,11.475992771616));
#21410=CARTESIAN_POINT('Ctrl Pts',(-4.33280375077929,5.51631761760486,11.4855211136814));
#21411=CARTESIAN_POINT('Ctrl Pts',(-4.65538494494174,5.24672094438443,11.5043566661358));
#21412=CARTESIAN_POINT('Ctrl Pts',(-4.80862572420868,5.10664333334677,11.513654565168));
#21413=CARTESIAN_POINT('Ctrl Pts',(-5.03673802868101,4.87874039587905,11.5282644410476));
#21414=CARTESIAN_POINT('Ctrl Pts',(-5.11603891018911,4.7955169476786,11.5335072557764));
#21415=CARTESIAN_POINT('Ctrl Pts',(-5.30451285525896,4.58772204805573,11.5463541632336));
#21416=CARTESIAN_POINT('Ctrl Pts',(-5.41138774546143,4.46115819730193,11.5539736695724));
#21417=CARTESIAN_POINT('Ctrl Pts',(-5.68441422288503,4.11356984621427,11.5743030093896));
#21418=CARTESIAN_POINT('Ctrl Pts',(-5.84214761820814,3.88630120225712,11.5869823553165));
#21419=CARTESIAN_POINT('Ctrl Pts',(-6.08535813166758,3.48746661279745,11.6082379413393));
#21420=CARTESIAN_POINT('Ctrl Pts',(-6.1779768905738,3.32063398571776,11.6168620472632));
#21421=CARTESIAN_POINT('Ctrl Pts',(-6.36500977153988,2.94875209548686,11.6356014570337));
#21422=CARTESIAN_POINT('Ctrl Pts',(-6.45656080620148,2.74250096205975,11.6456896942329));
#21423=CARTESIAN_POINT('Ctrl Pts',(-6.60388423113676,2.36211877169742,11.6639736233574));
#21424=CARTESIAN_POINT('Ctrl Pts',(-6.66309359073516,2.18953746448094,11.6721564786899));
#21425=CARTESIAN_POINT('Ctrl Pts',(-6.74793885066732,1.9067472804535,11.6855299257916));
#21426=CARTESIAN_POINT('Ctrl Pts',(-6.77775634056871,1.79788265699346,11.6906754748465));
#21427=CARTESIAN_POINT('Ctrl Pts',(-6.82430473967137,1.61026801188825,11.6995247280581));
#21428=CARTESIAN_POINT('Ctrl Pts',(-6.84233144297624,1.53186114772224,11.703216886361));
#21429=CARTESIAN_POINT('Ctrl Pts',(-6.93580265587684,1.09067180451096,11.7239392513773));
#21430=CARTESIAN_POINT('Ctrl Pts',(-6.98374533615733,0.722656878633498,
11.740987542979));
#21431=CARTESIAN_POINT('Ctrl Pts',(-7.01103032324011,0.180763667780065,
11.7656614780392));
#21432=CARTESIAN_POINT('Ctrl Pts',(-7.01335493138627,0.00868728982689054,
11.7734403708871));
#21433=CARTESIAN_POINT('Ctrl Pts',(-7.00437694985596,-0.376671595304211,
11.7907988943065));
#21434=CARTESIAN_POINT('Ctrl Pts',(-6.98966581540148,-0.589703733476513,
11.8003510528075));
#21435=CARTESIAN_POINT('Ctrl Pts',(-6.94176054474013,-1.00589288757262,
11.8191213762882));
#21436=CARTESIAN_POINT('Ctrl Pts',(-6.90929625709629,-1.20891814052628,
11.828330230728));
#21437=CARTESIAN_POINT('Ctrl Pts',(-6.84831033691245,-1.50592764867967,
11.8420686108816));
#21438=CARTESIAN_POINT('Ctrl Pts',(-6.82666055077586,-1.60121131827594,
11.8465213691738));
#21439=CARTESIAN_POINT('Ctrl Pts',(-6.77259581639827,-1.81807547267181,
11.856753370197));
#21440=CARTESIAN_POINT('Ctrl Pts',(-6.73888511412836,-1.93929871884705,
11.8625411399511));
#21441=CARTESIAN_POINT('Ctrl Pts',(-6.66237564907765,-2.18826650712128,
11.8745430404549));
#21442=CARTESIAN_POINT('Ctrl Pts',(-6.61913498672279,-2.31576848709062,
11.8807535285185));
#21443=CARTESIAN_POINT('Ctrl Pts',(-6.5722717076903,-2.44189908939613,11.8869527148536));
#21444=CARTESIAN_POINT('',(-7.0113586937745,3.84368575559509E-5,11.2264656437582));
#21445=CARTESIAN_POINT('Ctrl Pts',(-6.5722715952584,-2.44189939200198,11.3396960824468));
#21446=CARTESIAN_POINT('Ctrl Pts',(-6.63762197368278,-2.26601154123109,
11.3311779785242));
#21447=CARTESIAN_POINT('Ctrl Pts',(-6.695913184144,-2.0874837403581,11.3226598746016));
#21448=CARTESIAN_POINT('Ctrl Pts',(-6.74695164053556,-1.90690065886363,
11.314141770679));
#21449=CARTESIAN_POINT('Ctrl Pts',(-6.79799297831796,-1.72630738249899,
11.3056231858644));
#21450=CARTESIAN_POINT('Ctrl Pts',(-6.84178065721233,-1.54365888898769,
11.2971046010498));
#21451=CARTESIAN_POINT('Ctrl Pts',(-6.87817116927801,-1.35955431249099,
11.2885860162351));
#21452=CARTESIAN_POINT('Ctrl Pts',(-6.91456102987243,-1.17545303187645,
11.2800675839221));
#21453=CARTESIAN_POINT('Ctrl Pts',(-6.94355393105551,-0.989896022773728,
11.2715491516092));
#21454=CARTESIAN_POINT('Ctrl Pts',(-6.9650575549051,-0.80349226465435,11.2630307192962));
#21455=CARTESIAN_POINT('Ctrl Pts',(-6.98656581623424,-0.617048306630923,
11.2545104498949));
#21456=CARTESIAN_POINT('Ctrl Pts',(-7.00058153847027,-0.429757540599929,
11.2459901804936));
#21457=CARTESIAN_POINT('Ctrl Pts',(-7.00706421654034,-0.242234654374432,
11.2374699110923));
#21458=CARTESIAN_POINT('Ctrl Pts',(-7.00985509548824,-0.161503563032406,
11.2338018220332));
#21459=CARTESIAN_POINT('Ctrl Pts',(-7.01125044263142,-0.0807294898144902,
11.2301337329741));
#21460=CARTESIAN_POINT('Ctrl Pts',(-7.01124999989467,3.84328085378804E-5,
11.226465643915));
#21461=CARTESIAN_POINT('Ctrl Pts',(-7.01182214408909,3.84541218094794E-5,
11.2264656430896));
#21462=CARTESIAN_POINT('Ctrl Pts',(-7.01183325597241,0.036877061846341,
11.2247927479186));
#21463=CARTESIAN_POINT('Ctrl Pts',(-7.01154895025294,0.0737154962315686,
11.2231198527476));
#21464=CARTESIAN_POINT('Ctrl Pts',(-6.99268714592644,1.26993509149134,11.1687906152692));
#21465=CARTESIAN_POINT('Ctrl Pts',(-6.36864378850638,3.57944046714196,11.0634779306544));
#21466=CARTESIAN_POINT('Ctrl Pts',(-3.89598737047602,6.18007435040298,10.9055089037321));
#21467=CARTESIAN_POINT('Ctrl Pts',(-0.483327077985568,7.28961040383802,
10.7475398768098));
#21468=CARTESIAN_POINT('Ctrl Pts',(3.04594747324975,6.64034897205148,10.5895708498875));
#21469=CARTESIAN_POINT('Ctrl Pts',(5.84031211439899,4.3889387019149,10.4316018229652));
#21470=CARTESIAN_POINT('Ctrl Pts',(7.22555706859702,1.07858883068963,10.2736327960429));
#21471=CARTESIAN_POINT('Ctrl Pts',(6.86745790157161,-2.49199739961005,10.1156637691206));
#21472=CARTESIAN_POINT('Ctrl Pts',(4.85241481466244,-5.46132760686174,9.95769474219825));
#21473=CARTESIAN_POINT('Ctrl Pts',(1.66660677536437,-7.11297763457679,9.79972571527604));
#21474=CARTESIAN_POINT('Ctrl Pts',(-1.92131133239526,-7.04844604350416,
9.64175668835372));
#21475=CARTESIAN_POINT('Ctrl Pts',(-4.95411394330101,-5.3350259731329,9.48841656263841));
#21476=CARTESIAN_POINT('Ctrl Pts',(-6.2036482880654,-3.43323261796278,9.3877327792305));
#21477=CARTESIAN_POINT('Ctrl Pts',(-6.57271212262969,-2.44206338025277,
9.33970533813003));
#21478=CARTESIAN_POINT('Origin',(0.,0.,0.));
#21479=CARTESIAN_POINT('',(-6.5722715952584,-2.44189939200199,7.33970278241542));
#21480=CARTESIAN_POINT('',(-6.57280081548431,-2.44209581534386,7.88676746742487));
#21481=CARTESIAN_POINT('',(-6.57227159525839,-2.441899392002,0.));
#21482=CARTESIAN_POINT('',(-7.01170386511408,-0.000104878804555574,9.77353434367529));
#21483=CARTESIAN_POINT('Ctrl Pts',(-6.57280081548428,-2.44209581534395,
7.88676746742488));
#21484=CARTESIAN_POINT('Ctrl Pts',(-6.55738010449231,-2.48364608990916,
7.88878007829007));
#21485=CARTESIAN_POINT('Ctrl Pts',(-6.12762765860759,-3.60823497536755,
7.9434490314627));
#21486=CARTESIAN_POINT('Ctrl Pts',(-4.70540847483628,-5.58848458735646,
8.05077432694275));
#21487=CARTESIAN_POINT('Ctrl Pts',(-1.47678875996353,-7.15479726159574,
8.20874335386504));
#21488=CARTESIAN_POINT('Ctrl Pts',(2.10814273077403,-6.99483832025251,8.36671238078733));
#21489=CARTESIAN_POINT('Ctrl Pts',(5.18443270117429,-5.14720180894841,8.52468140770962));
#21490=CARTESIAN_POINT('Ctrl Pts',(7.00985018797118,-2.05767568861079,8.68265043463191));
#21491=CARTESIAN_POINT('Ctrl Pts',(7.14396812247892,1.5283155343373,8.8406194615542));
#21492=CARTESIAN_POINT('Ctrl Pts',(5.55442723662981,4.74556286831861,8.99858848847649));
#21493=CARTESIAN_POINT('Ctrl Pts',(2.62474354776114,6.81782592049456,9.15655751539878));
#21494=CARTESIAN_POINT('Ctrl Pts',(-0.938224379280222,7.24511999742922,
9.31452654232109));
#21495=CARTESIAN_POINT('Ctrl Pts',(-4.27482248085003,5.9243499075208,9.47249556924335));
#21496=CARTESIAN_POINT('Ctrl Pts',(-6.50754058792984,3.26064708099906,9.62549816969478));
#21497=CARTESIAN_POINT('Ctrl Pts',(-7.01093898172325,1.05011949196855,9.72584442783875));
#21498=CARTESIAN_POINT('Ctrl Pts',(-7.01170386511407,-0.000104878804555574,
9.77353434367529));
#21499=CARTESIAN_POINT('Ctrl Pts',(-7.01124999902501,-0.000116926258460787,
9.77327286327579));
#21500=CARTESIAN_POINT('Ctrl Pts',(-7.01124832255164,-0.100643310223616,
9.77779485366763));
#21501=CARTESIAN_POINT('Ctrl Pts',(-7.00908464412642,-0.201157219552033,
9.78232974651185));
#21502=CARTESIAN_POINT('Ctrl Pts',(-7.00040283391986,-0.402802601350129,
9.79148686211807));
#21503=CARTESIAN_POINT('Ctrl Pts',(-6.99385196405524,-0.503908655088689,
9.79611034983023));
#21504=CARTESIAN_POINT('Ctrl Pts',(-6.95413787236706,-0.962557765689151,
9.81719252923423));
#21505=CARTESIAN_POINT('Ctrl Pts',(-6.89572929599919,-1.31737321865183,
9.83376990625039));
#21506=CARTESIAN_POINT('Ctrl Pts',(-6.76873539423717,-1.83646088146557,
9.85820301925403));
#21507=CARTESIAN_POINT('Ctrl Pts',(-6.72069575740167,-2.00514768445086,
9.86617845663394));
#21508=CARTESIAN_POINT('Ctrl Pts',(-6.6368466352524,-2.26251737183206,9.87842964187306));
#21509=CARTESIAN_POINT('Ctrl Pts',(-6.60546909578075,-2.35254968492693,
9.8827317871224));
#21510=CARTESIAN_POINT('Ctrl Pts',(-6.57227161595961,-2.44189933628552,
9.88702363219766));
#21511=CARTESIAN_POINT('',(-7.01124999890517,0.000123904338948809,9.22646564308964));
#21512=CARTESIAN_POINT('Ctrl Pts',(-6.57271212262969,-2.44206338025277,
9.33970533813003));
#21513=CARTESIAN_POINT('Ctrl Pts',(-6.60828262128868,-2.3465341499709,9.33507643692307));
#21514=CARTESIAN_POINT('Ctrl Pts',(-6.88115023186467,-1.56117498902781,
9.29732987190961));
#21515=CARTESIAN_POINT('Ctrl Pts',(-7.01034884492464,-0.729457585781793,
9.25958330689615));
#21516=CARTESIAN_POINT('Ctrl Pts',(-7.01081502653957,0.000123896652022004,
9.22646564308964));
#21517=CARTESIAN_POINT('Ctrl Pts',(-7.01124999890517,0.000123904338948809,
9.22646564308964));
#21518=CARTESIAN_POINT('Ctrl Pts',(-7.01124658275476,0.193430165674024,
9.21769149676437));
#21519=CARTESIAN_POINT('Ctrl Pts',(-7.00324439628698,0.386702906863349,
9.20891735043909));
#21520=CARTESIAN_POINT('Ctrl Pts',(-6.98727771593147,0.579289809117614,
9.20014320411381));
#21521=CARTESIAN_POINT('Ctrl Pts',(-6.97130597709455,0.771937725762138,
9.1913662780087));
#21522=CARTESIAN_POINT('Ctrl Pts',(-6.94736472578101,0.963899103762233,
9.18258935190358));
#21523=CARTESIAN_POINT('Ctrl Pts',(-6.91554014229809,1.15452635429589,9.17381242579847));
#21524=CARTESIAN_POINT('Ctrl Pts',(-6.90833320736833,1.19769544058329,9.17182481972793));
#21525=CARTESIAN_POINT('Ctrl Pts',(-6.90072219846778,1.24079613936,9.1698372136574));
#21526=CARTESIAN_POINT('Ctrl Pts',(-6.89270848282156,1.28382098960083,9.16784960758686));
#21527=CARTESIAN_POINT('Ctrl Pts',(-6.85830735406572,1.46851726261298,9.15931724939412));
#21528=CARTESIAN_POINT('Ctrl Pts',(-6.81647250719612,1.65186114390348,9.15078489120138));
#21529=CARTESIAN_POINT('Ctrl Pts',(-6.76733506680133,1.83324920732045,9.14225253300863));
#21530=CARTESIAN_POINT('Ctrl Pts',(-6.7182068275768,2.0146033051413,9.13372177253201));
#21531=CARTESIAN_POINT('Ctrl Pts',(-6.6617788037032,2.1940020207426,9.12519101205538));
#21532=CARTESIAN_POINT('Ctrl Pts',(-6.59823254511356,2.3708550869052,9.11666025157876));
#21533=CARTESIAN_POINT('Ctrl Pts',(-6.5319484137181,2.55532781803658,9.10776194566924));
#21534=CARTESIAN_POINT('Ctrl Pts',(-6.45791918342226,2.73703034380715,9.09886363975973));
#21535=CARTESIAN_POINT('Ctrl Pts',(-6.37640791234427,2.91531279589232,9.08996533385021));
#21536=CARTESIAN_POINT('Ctrl Pts',(-6.2982658840008,3.08622599893454,9.08143483661474));
#21537=CARTESIAN_POINT('Ctrl Pts',(-6.21324805037836,3.25399588188927,9.07290433937927));
#21538=CARTESIAN_POINT('Ctrl Pts',(-6.121634643497,3.41807194980407,9.06437384214381));
#21539=CARTESIAN_POINT('Ctrl Pts',(-6.03002029908661,3.58214969679708,9.0558432576112));
#21540=CARTESIAN_POINT('Ctrl Pts',(-5.93181039853669,3.74253328763762,9.04731267307858));
#21541=CARTESIAN_POINT('Ctrl Pts',(-5.82733050628654,3.89869795354838,9.03878208854597));
#21542=CARTESIAN_POINT('Ctrl Pts',(-5.72282993987773,4.0548935208413,9.03024981600762));
#21543=CARTESIAN_POINT('Ctrl Pts',(-5.61205707474818,4.20686824205592,9.02171754346927));
#21544=CARTESIAN_POINT('Ctrl Pts',(-5.49538056018055,4.35412667033123,9.01318527093092));
#21545=CARTESIAN_POINT('Ctrl Pts',(-5.48031697892598,4.37313854523996,9.0120837075088));
#21546=CARTESIAN_POINT('Ctrl Pts',(-5.46515505065842,4.39207185135154,9.01098214408669));
#21547=CARTESIAN_POINT('Ctrl Pts',(-5.4498956183453,4.41092556178867,9.00988058066457));
#21548=CARTESIAN_POINT('Ctrl Pts',(-5.33170093238843,4.55696037740384,9.00134822244397));
#21549=CARTESIAN_POINT('Ctrl Pts',(-5.2076132572532,4.69826636571517,8.99281586422336));
#21550=CARTESIAN_POINT('Ctrl Pts',(-5.07803522196381,4.83437533162196,8.98428350600275));
#21551=CARTESIAN_POINT('Ctrl Pts',(-4.94848145064301,4.97045881061915,8.97575274549793));
#21552=CARTESIAN_POINT('Ctrl Pts',(-4.81343958175058,5.10134698776302,8.96722198499311));
#21553=CARTESIAN_POINT('Ctrl Pts',(-4.67335032081439,5.22660724958783,8.95869122448828));
#21554=CARTESIAN_POINT('Ctrl Pts',(-4.52722535390439,5.35726431417628,8.94979291859278));
#21555=CARTESIAN_POINT('Ctrl Pts',(-4.37560867694897,5.48179751437576,8.94089461269728));
#21556=CARTESIAN_POINT('Ctrl Pts',(-4.21904104994549,5.59976063607855,8.93199630680178));
#21557=CARTESIAN_POINT('Ctrl Pts',(-4.06894509578705,5.7128477898303,8.92346580953782));
#21558=CARTESIAN_POINT('Ctrl Pts',(-3.91429951543427,5.81989689243582,8.91493531227385));
#21559=CARTESIAN_POINT('Ctrl Pts',(-3.75561285408614,5.92055729241116,8.90640481500988));
#21560=CARTESIAN_POINT('Ctrl Pts',(-3.5969245688119,6.02121872249862,8.89787423044874));
#21561=CARTESIAN_POINT('Ctrl Pts',(-3.43419538001805,6.11549115814567,8.8893436458876));
#21562=CARTESIAN_POINT('Ctrl Pts',(-3.26796144695351,6.20306815565697,8.88081306132646));
#21563=CARTESIAN_POINT('Ctrl Pts',(-3.10169462003571,6.29066248263194,8.8722807887598));
#21564=CARTESIAN_POINT('Ctrl Pts',(-2.93192193489967,6.37155858359133,8.86374851619314));
#21565=CARTESIAN_POINT('Ctrl Pts',(-2.75920347628835,6.44549631439956,8.85521624362648));
#21566=CARTESIAN_POINT('Ctrl Pts',(-2.73690457375769,6.45504208192138,8.85411468033174));
#21567=CARTESIAN_POINT('Ctrl Pts',(-2.71455659928903,6.46447193081478,8.85301311703701));
#21568=CARTESIAN_POINT('Ctrl Pts',(-2.69216078310632,6.47378535946353,8.85191155374228));
#21569=CARTESIAN_POINT('Ctrl Pts',(-2.51868992849126,6.54592420959144,8.84337919552899));
#21570=CARTESIAN_POINT('Ctrl Pts',(-2.34228864292468,6.61109874328733,8.8348468373157));
#21571=CARTESIAN_POINT('Ctrl Pts',(-2.16353391566274,6.66908896014119,8.82631447910241));
#21572=CARTESIAN_POINT('Ctrl Pts',(-1.98481266088958,6.72706831811085,8.81778371860499));
#21573=CARTESIAN_POINT('Ctrl Pts',(-1.80373913480668,6.77786594956174,8.80925295810757));
#21574=CARTESIAN_POINT('Ctrl Pts',(-1.62090686743586,6.82131127347223,8.80072219761014));
#21575=CARTESIAN_POINT('Ctrl Pts',(-1.43019732356839,6.86662842686801,8.79182389171097));
#21576=CARTESIAN_POINT('Ctrl Pts',(-1.23757446921328,6.90394559042813,8.78292558581179));
#21577=CARTESIAN_POINT('Ctrl Pts',(-1.04372629453956,6.93312786443368,8.77402727991261));
#21578=CARTESIAN_POINT('Ctrl Pts',(-0.857890772477837,6.96110389842987,
8.76549678265607));
#21579=CARTESIAN_POINT('Ctrl Pts',(-0.670929513079274,6.9816039792824,8.75696628539953));
#21580=CARTESIAN_POINT('Ctrl Pts',(-0.483456675624474,6.99456190231341,
8.748435788143));
#21581=CARTESIAN_POINT('Ctrl Pts',(-0.295981919659145,7.00751995794982,
8.73990520358929));
#21582=CARTESIAN_POINT('Ctrl Pts',(-0.107995880649334,7.01293568366323,
8.73137461903558));
#21583=CARTESIAN_POINT('Ctrl Pts',(0.0798840490155643,7.0107948979565,8.72284403448187));
#21584=CARTESIAN_POINT('Ctrl Pts',(0.267801155778221,7.00865368863773,8.71431176192254));
#21585=CARTESIAN_POINT('Ctrl Pts',(0.455611805303478,6.9989529859322,8.70577948936322));
#21586=CARTESIAN_POINT('Ctrl Pts',(0.642699611673814,6.98173071463332,8.6972472168039));
#21587=CARTESIAN_POINT('Ctrl Pts',(0.666853676745562,6.97950722465978,8.69614565347593));
#21588=CARTESIAN_POINT('Ctrl Pts',(0.690995698884943,6.97715843443401,8.69504409014796));
#21589=CARTESIAN_POINT('Ctrl Pts',(0.715124357432948,6.97468448862786,8.69394252681999));
#21590=CARTESIAN_POINT('Ctrl Pts',(0.902017251097917,6.95552209343868,8.68541016860746));
#21591=CARTESIAN_POINT('Ctrl Pts',(1.08817097862681,6.92884020609057,8.67687781039493));
#21592=CARTESIAN_POINT('Ctrl Pts',(1.27297340344457,6.89472010139808,8.6683454521824));
#21593=CARTESIAN_POINT('Ctrl Pts',(1.45774122331942,6.86060638582239,8.65981469168575));
#21594=CARTESIAN_POINT('Ctrl Pts',(1.64115794467901,6.81905728801807,8.65128393118911));
#21595=CARTESIAN_POINT('Ctrl Pts',(1.82262041678906,6.77020541629305,8.64275317069246));
#21596=CARTESIAN_POINT('Ctrl Pts',(2.01190114817992,6.71924877549342,8.63385486479289));
#21597=CARTESIAN_POINT('Ctrl Pts',(2.19905515706665,6.66034621462148,8.62495655889333));
#21598=CARTESIAN_POINT('Ctrl Pts',(2.38341321773614,6.59370669623852,8.61605825299377));
#21599=CARTESIAN_POINT('Ctrl Pts',(2.56015089661138,6.52982170115017,8.60752775573805));
#21600=CARTESIAN_POINT('Ctrl Pts',(2.73431881202718,6.4588266093185,8.59899725848233));
#21601=CARTESIAN_POINT('Ctrl Pts',(2.90534537172126,6.38095563638534,8.59046676122661));
#21602=CARTESIAN_POINT('Ctrl Pts',(3.07637368162198,6.3030838665567,8.58193617667373));
#21603=CARTESIAN_POINT('Ctrl Pts',(3.2442602944321,6.21833620475762,8.57340559212086));
#21604=CARTESIAN_POINT('Ctrl Pts',(3.40845554578905,6.12699415332509,8.56487500756798));
#21605=CARTESIAN_POINT('Ctrl Pts',(3.57268328759253,6.03563402741104,8.55634273500952));
#21606=CARTESIAN_POINT('Ctrl Pts',(3.73321794214793,5.93767705528345,8.54781046245106));
#21607=CARTESIAN_POINT('Ctrl Pts',(3.88953554069426,5.83345008037064,8.5392781898926));
#21608=CARTESIAN_POINT('Ctrl Pts',(3.90971700272182,5.81999380445538,8.53817662656096));
#21609=CARTESIAN_POINT('Ctrl Pts',(3.92982821259818,5.80643307845208,8.53707506322933));
#21610=CARTESIAN_POINT('Ctrl Pts',(3.94986807787101,5.79276865841504,8.5359734998977));
#21611=CARTESIAN_POINT('Ctrl Pts',(4.1050904824131,5.6869284191746,8.52744114168254));
#21612=CARTESIAN_POINT('Ctrl Pts',(4.25608246582144,5.57482777531395,8.51890878346739));
#21613=CARTESIAN_POINT('Ctrl Pts',(4.40234443727481,5.45682966731558,8.51037642525224));
#21614=CARTESIAN_POINT('Ctrl Pts',(4.54857902062949,5.33885365490225,8.50184566475292));
#21615=CARTESIAN_POINT('Ctrl Pts',(4.69008512153923,5.21498257421762,8.49331490425361));
#21616=CARTESIAN_POINT('Ctrl Pts',(4.82639549357391,5.08562022786892,8.4847841437543));
#21617=CARTESIAN_POINT('Ctrl Pts',(4.96857875936425,4.95068434148251,8.47588583785606));
#21618=CARTESIAN_POINT('Ctrl Pts',(5.10510839400903,4.80977375433093,8.46698753195782));
#21619=CARTESIAN_POINT('Ctrl Pts',(5.23549540348985,4.66339087387458,8.45808922605958));
#21620=CARTESIAN_POINT('Ctrl Pts',(5.36049290746771,4.52305868315257,8.44955872880114));
#21621=CARTESIAN_POINT('Ctrl Pts',(5.47984516611268,4.37769773859499,8.44102823154271));
#21622=CARTESIAN_POINT('Ctrl Pts',(5.59316106493631,4.22778616585329,8.43249773428427));
#21623=CARTESIAN_POINT('Ctrl Pts',(5.70647812338238,4.07787305898599,8.42396714972868));
#21624=CARTESIAN_POINT('Ctrl Pts',(5.81375851664481,3.92340947692052,8.41543656517308));
#21625=CARTESIAN_POINT('Ctrl Pts',(5.91465292849583,3.76490468643441,8.40690598061749));
#21626=CARTESIAN_POINT('Ctrl Pts',(6.01556730501989,3.60636853151234,8.3983737080563));
#21627=CARTESIAN_POINT('Ctrl Pts',(6.11009301282587,3.44378982968665,8.38984143549512));
#21628=CARTESIAN_POINT('Ctrl Pts',(6.1979249207185,3.27770548396841,8.38130916293393));
#21629=CARTESIAN_POINT('Ctrl Pts',(6.20926450314781,3.25626308138743,8.38020759961442));
#21630=CARTESIAN_POINT('Ctrl Pts',(6.22049257427684,3.23476228004916,8.37910603629492));
#21631=CARTESIAN_POINT('Ctrl Pts',(6.2316085334411,3.21320426497352,8.37800447297541));
#21632=CARTESIAN_POINT('Ctrl Pts',(6.31770920853686,3.04622275448865,8.36947211476243));
#21633=CARTESIAN_POINT('Ctrl Pts',(6.39710890112773,2.8757504042213,8.36093975654946));
#21634=CARTESIAN_POINT('Ctrl Pts',(6.4695411047759,2.70234425196255,8.35240739833648));
#21635=CARTESIAN_POINT('Ctrl Pts',(6.54195974522404,2.52897057065198,8.34387663783937));
#21636=CARTESIAN_POINT('Ctrl Pts',(6.60741338252163,2.35266446590524,8.33534587734227));
#21637=CARTESIAN_POINT('Ctrl Pts',(6.66568340928876,2.17400350727236,8.32681511684516));
#21638=CARTESIAN_POINT('Ctrl Pts',(6.7264639836716,1.98764499178909,8.31791681094582));
#21639=CARTESIAN_POINT('Ctrl Pts',(6.77942809646649,1.79872453902279,8.30901850504649));
#21640=CARTESIAN_POINT('Ctrl Pts',(6.82438496723768,1.60791678312045,8.30012019914715));
#21641=CARTESIAN_POINT('Ctrl Pts',(6.86748356005959,1.42499600509848,8.29158970189097));
#21642=CARTESIAN_POINT('Ctrl Pts',(6.90322348059718,1.24034112726373,8.28305920463477));
#21643=CARTESIAN_POINT('Ctrl Pts',(6.93148845816996,1.05455882565013,8.27452870737859));
#21644=CARTESIAN_POINT('Ctrl Pts',(6.95975372499345,0.868774622826431,8.26599812282524));
#21645=CARTESIAN_POINT('Ctrl Pts',(6.98054385317258,0.681863276153072,8.25746753827189));
#21646=CARTESIAN_POINT('Ctrl Pts',(6.99379415578536,0.494438943654839,8.24893695371854));
#21647=CARTESIAN_POINT('Ctrl Pts',(7.0070470803269,0.306977524211316,8.2404046811596));
#21648=CARTESIAN_POINT('Ctrl Pts',(7.01275717886277,0.119003221499164,8.23187240860065));
#21649=CARTESIAN_POINT('Ctrl Pts',(7.01091177820364,-0.0688665430052387,
8.2233401360417));
#21650=CARTESIAN_POINT('Ctrl Pts',(7.01067352682567,-0.0931215632094089,
8.22223857271217));
#21651=CARTESIAN_POINT('Ctrl Pts',(7.01030940985087,-0.117374840699323,
8.22113700938265));
#21652=CARTESIAN_POINT('Ctrl Pts',(7.00981946332768,-0.1416250474047,8.22003544605312));
#21653=CARTESIAN_POINT('Ctrl Pts',(7.00602449382425,-0.329459414103322,
8.21150308783887));
#21654=CARTESIAN_POINT('Ctrl Pts',(6.99467475803301,-0.51717280440197,8.20297072962462));
#21655=CARTESIAN_POINT('Ctrl Pts',(6.9758011351623,-0.704148482330555,8.19443837141036));
#21656=CARTESIAN_POINT('Ctrl Pts',(6.95693104644776,-0.891089148367108,
8.18590761091196));
#21657=CARTESIAN_POINT('Ctrl Pts',(6.93053991296919,-1.07729207340012,8.17737685041356));
#21658=CARTESIAN_POINT('Ctrl Pts',(6.89671051082845,-1.26214527386048,8.16884608991516));
#21659=CARTESIAN_POINT('Ctrl Pts',(6.86142357847646,-1.45496282211506,8.15994778401646));
#21660=CARTESIAN_POINT('Ctrl Pts',(6.81804326857906,-1.64631141349988,8.15104947811777));
#21661=CARTESIAN_POINT('Ctrl Pts',(6.76672304477732,-1.83550695933837,8.14215117221907));
#21662=CARTESIAN_POINT('Ctrl Pts',(6.71752412608659,-2.01688216752755,8.13362067496157));
#21663=CARTESIAN_POINT('Ctrl Pts',(6.66102856965722,-2.19627842708316,8.12509017770407));
#21664=CARTESIAN_POINT('Ctrl Pts',(6.59742300179105,-2.373106887171,8.11655968044657));
#21665=CARTESIAN_POINT('Ctrl Pts',(6.53381678301494,-2.54993715683943,8.10802909589191));
#21666=CARTESIAN_POINT('Ctrl Pts',(6.46310051401775,-2.72419928770746,8.09949851133725));
#21667=CARTESIAN_POINT('Ctrl Pts',(6.38550974450136,-2.89532241130036,8.09096792678259));
#21668=CARTESIAN_POINT('Ctrl Pts',(6.30790362156429,-3.06647939620591,8.08243565422233));
#21669=CARTESIAN_POINT('Ctrl Pts',(6.22342040846619,-3.2344958549851,8.07390338166207));
#21670=CARTESIAN_POINT('Ctrl Pts',(6.13234294774363,-3.39882281588185,8.06537110910181));
#21671=CARTESIAN_POINT('Ctrl Pts',(6.12058434654617,-3.42003833049816,8.06426954577815));
#21672=CARTESIAN_POINT('Ctrl Pts',(6.10871589364357,-3.44119238140111,8.06316798245449));
#21673=CARTESIAN_POINT('Ctrl Pts',(6.09673825309964,-3.46228381789991,8.06206641913083));
#21674=CARTESIAN_POINT('Ctrl Pts',(6.00396326914703,-3.62565135890573,8.05353406091716));
#21675=CARTESIAN_POINT('Ctrl Pts',(5.90460250915252,-3.78531529587458,8.04500170270348));
#21676=CARTESIAN_POINT('Ctrl Pts',(5.79897678759855,-3.94074799744835,8.03646934448981));
#21677=CARTESIAN_POINT('Ctrl Pts',(5.6933708448544,-4.09615159366976,8.02793858399199));
#21678=CARTESIAN_POINT('Ctrl Pts',(5.58150245361073,-4.24732528269289,8.01940782349418));
#21679=CARTESIAN_POINT('Ctrl Pts',(5.46373580167137,-4.39377032308637,8.01087706299636));
#21680=CARTESIAN_POINT('Ctrl Pts',(5.34089520687048,-4.54652490658968,8.00197875709737));
#21681=CARTESIAN_POINT('Ctrl Pts',(5.21163704586447,-4.69413406121,7.99308045119839));
#21682=CARTESIAN_POINT('Ctrl Pts',(5.07642199947609,-4.8360692970361,7.9841821452994));
#21683=CARTESIAN_POINT('Ctrl Pts',(4.94679602399237,-4.9721376850661,7.9756516480425));
#21684=CARTESIAN_POINT('Ctrl Pts',(4.81169593945423,-5.10299154626926,7.96712115078559));
#21685=CARTESIAN_POINT('Ctrl Pts',(4.67156624093936,-5.22820192982404,7.95859065352869));
#21686=CARTESIAN_POINT('Ctrl Pts',(4.53143510840219,-5.35341359472376,7.95006006897463));
#21687=CARTESIAN_POINT('Ctrl Pts',(4.38627448935698,-5.47298146511146,7.94152948442058));
#21688=CARTESIAN_POINT('Ctrl Pts',(4.23656333794403,-5.58651569818689,7.93299889986653));
#21689=CARTESIAN_POINT('Ctrl Pts',(4.08682256215286,-5.70007239706416,7.92446662730686));
#21690=CARTESIAN_POINT('Ctrl Pts',(3.93252969996467,-5.80759288994331,7.9159343547472));
#21691=CARTESIAN_POINT('Ctrl Pts',(3.7741948668916,-5.90872910778867,7.90740208218754));
#21692=CARTESIAN_POINT('Ctrl Pts',(3.75375296888909,-5.92178634989661,7.90630051886121));
#21693=CARTESIAN_POINT('Ctrl Pts',(3.73324373750947,-5.93473723693103,7.90519895553487));
#21694=CARTESIAN_POINT('Ctrl Pts',(3.71266830461015,-5.94758107321315,7.90409739220854));
#21695=CARTESIAN_POINT('Ctrl Pts',(3.55329756331394,-6.0470653328826,7.89556503399468));
#21696=CARTESIAN_POINT('Ctrl Pts',(3.38989901740822,-6.14015694685801,7.88703267578082));
#21697=CARTESIAN_POINT('Ctrl Pts',(3.22300601222923,-6.22654469249473,7.87850031756695));
#21698=CARTESIAN_POINT('Ctrl Pts',(3.05614425838705,-6.31291626170432,7.86996955706895));
#21699=CARTESIAN_POINT('Ctrl Pts',(2.88578962273823,-6.392586327142,7.86143879657094));
#21700=CARTESIAN_POINT('Ctrl Pts',(2.71249983548278,-6.46528972320699,7.85290803607293));
#21701=CARTESIAN_POINT('Ctrl Pts',(2.53174390680414,-6.54112552450812,7.84400973017404));
#21702=CARTESIAN_POINT('Ctrl Pts',(2.3477946196699,-6.60938088676141,7.83511142427515));
#21703=CARTESIAN_POINT('Ctrl Pts',(2.1613087214537,-6.66981043006982,7.82621311837626));
#21704=CARTESIAN_POINT('Ctrl Pts',(1.98253115847744,-6.72774213744172,7.81768262111916));
#21705=CARTESIAN_POINT('Ctrl Pts',(1.80142277919043,-6.77848187322731,7.80915212386206));
#21706=CARTESIAN_POINT('Ctrl Pts',(1.61857870202646,-6.82186408160162,7.80062162660496));
#21707=CARTESIAN_POINT('Ctrl Pts',(1.43573275372108,-6.86524673392932,7.79209104205071));
#21708=CARTESIAN_POINT('Ctrl Pts',(1.25115137050542,-6.90127164090224,7.78356045749647));
#21709=CARTESIAN_POINT('Ctrl Pts',(1.06544135143817,-6.92982404460212,7.77502987294222));
#21710=CARTESIAN_POINT('Ctrl Pts',(0.87969458464844,-6.95838209816307,7.76649760038236));
#21711=CARTESIAN_POINT('Ctrl Pts',(0.692819038538371,-6.97946464968945,
7.75796532782251));
#21712=CARTESIAN_POINT('Ctrl Pts',(0.505429023624814,-6.99300851312064,
7.74943305526265));
#21713=CARTESIAN_POINT('Ctrl Pts',(0.48123594182401,-6.9947571003975,7.74833149193718));
#21714=CARTESIAN_POINT('Ctrl Pts',(0.457034290815553,-6.99638010203042,
7.74722992861172));
#21715=CARTESIAN_POINT('Ctrl Pts',(0.432825397161842,-6.99787744520235,
7.74612836528625));
#21716=CARTESIAN_POINT('Ctrl Pts',(0.245311027502743,-7.00947538788665,
7.7375960070724));
#21717=CARTESIAN_POINT('Ctrl Pts',(0.0572986320455093,-7.01353402693959,
7.72906364885856));
#21718=CARTESIAN_POINT('Ctrl Pts',(-0.1305945957598,-7.01003363858251,7.72053129064471));
#21719=CARTESIAN_POINT('Ctrl Pts',(-0.318452639858229,-7.00653390568619,
7.71200053014672));
#21720=CARTESIAN_POINT('Ctrl Pts',(-0.506191255034217,-6.99547797580645,
7.70346976964874));
#21721=CARTESIAN_POINT('Ctrl Pts',(-0.693193734882397,-6.97689823692591,
7.69493900915075));
#21722=CARTESIAN_POINT('Ctrl Pts',(-0.888253163632606,-6.9575179952558,
7.68604070325185));
#21723=CARTESIAN_POINT('Ctrl Pts',(-1.08251126646201,-6.92995127258633,
7.67714239735295));
#21724=CARTESIAN_POINT('Ctrl Pts',(-1.27527368597644,-6.89429500299748,
7.66824409145405));
#21725=CARTESIAN_POINT('Ctrl Pts',(-1.46006833224076,-6.86011257396192,
7.65971359419696));
#21726=CARTESIAN_POINT('Ctrl Pts',(-1.64348813504849,-6.81849596942113,
7.65118309693986));
#21727=CARTESIAN_POINT('Ctrl Pts',(-1.82493093963575,-6.76958297297996,
7.64265259968277));
#21728=CARTESIAN_POINT('Ctrl Pts',(-2.00637560102454,-6.72066947598587,
7.63412201512852));
#21729=CARTESIAN_POINT('Ctrl Pts',(-2.18584292917541,-6.66445952065229,
7.62559143057427));
#21730=CARTESIAN_POINT('Ctrl Pts',(-2.36274468537664,-6.60114112212612,
7.61706084602002));
#21731=CARTESIAN_POINT('Ctrl Pts',(-2.53968144634822,-6.53781019435182,
7.60852857346018));
#21732=CARTESIAN_POINT('Ctrl Pts',(-2.71405133366301,-6.46736811807306,
7.59999630090035));
#21733=CARTESIAN_POINT('Ctrl Pts',(-2.88528405938972,-6.39005183540256,
7.59146402834051));
#21734=CARTESIAN_POINT('Ctrl Pts',(-2.90739114627262,-6.3800698779747,7.59036246501499));
#21735=CARTESIAN_POINT('Ctrl Pts',(-2.92944597066077,-6.3699734049718,7.58926090168947));
#21736=CARTESIAN_POINT('Ctrl Pts',(-2.9514473313527,-6.35976298400743,7.58815933836396));
#21737=CARTESIAN_POINT('Ctrl Pts',(-3.12186285469646,-6.28067631947939,
7.57962698015016));
#21738=CARTESIAN_POINT('Ctrl Pts',(-3.28912646399832,-6.19472273666056,
7.57109462193637));
#21739=CARTESIAN_POINT('Ctrl Pts',(-3.45268603086347,-6.1021787694872,7.56256226372258));
#21740=CARTESIAN_POINT('Ctrl Pts',(-3.61621497059052,-6.00965213151639,
7.55403150322464));
#21741=CARTESIAN_POINT('Ctrl Pts',(-3.77604098584443,-5.91053772256712,
7.5455007427267));
#21742=CARTESIAN_POINT('Ctrl Pts',(-3.93163718967202,-5.80515766980432,
7.53696998222876));
#21743=CARTESIAN_POINT('Ctrl Pts',(-4.09393721189208,-5.69523734730144,
7.52807167632984));
#21744=CARTESIAN_POINT('Ctrl Pts',(-4.25163456349199,-5.5784996926556,7.51917337043091));
#21745=CARTESIAN_POINT('Ctrl Pts',(-4.4041648079342,-5.45536056618203,7.51027506453199));
#21746=CARTESIAN_POINT('Ctrl Pts',(-4.55039026327477,-5.33731135630445,
7.50174456727495));
#21747=CARTESIAN_POINT('Ctrl Pts',(-4.69186693034422,-5.21337944552277,
7.49321407001791));
#21748=CARTESIAN_POINT('Ctrl Pts',(-4.82813090276307,-5.08397271317267,
7.48468357276087));
#21749=CARTESIAN_POINT('Ctrl Pts',(-4.96439626964382,-4.95456465653447,
7.4761529882067));
#21750=CARTESIAN_POINT('Ctrl Pts',(-5.09544861563702,-4.81968187942328,
7.46762240365254));
#21751=CARTESIAN_POINT('Ctrl Pts',(-5.220860189501,-4.67976980675156,7.45909181909837));
#21752=CARTESIAN_POINT('Ctrl Pts',(-5.34629657941822,-4.53983004871288,
7.45055954653859));
#21753=CARTESIAN_POINT('Ctrl Pts',(-5.46608976439216,-4.39485923597475,
7.44202727397881));
#21754=CARTESIAN_POINT('Ctrl Pts',(-5.57985107513084,-4.2453372706843,7.43349500141903));
#21755=CARTESIAN_POINT('Ctrl Pts',(-5.59453828617866,-4.2260331624049,7.43239343809325));
#21756=CARTESIAN_POINT('Ctrl Pts',(-5.60912501264739,-4.20665323833119,
7.43129187476746));
#21757=CARTESIAN_POINT('Ctrl Pts',(-5.62361046851604,-4.1871985695566,7.43019031144167));
#21758=CARTESIAN_POINT('Ctrl Pts',(-5.73581180460668,-4.03650674118037,
7.42165783044403));
#21759=CARTESIAN_POINT('Ctrl Pts',(-5.84197158997454,-3.88127706288372,
7.41312534944638));
#21760=CARTESIAN_POINT('Ctrl Pts',(-5.9417359609281,-3.72201562773638,7.40459286844873));
#21761=CARTESIAN_POINT('Ctrl Pts',(-6.04148005497682,-3.56278656215078,
7.39606212166043));
#21762=CARTESIAN_POINT('Ctrl Pts',(-6.13483116679695,-3.39952763456354,
7.38753137487214));
#21763=CARTESIAN_POINT('Ctrl Pts',(-6.22147935548776,-3.23277298796862,
7.37900062808384));
#21764=CARTESIAN_POINT('Ctrl Pts',(-6.30812283662519,-3.06602740107147,
7.37047034476682));
#21765=CARTESIAN_POINT('Ctrl Pts',(-6.38806397881865,-2.8957867448778,7.36194006144979));
#21766=CARTESIAN_POINT('Ctrl Pts',(-6.46103893650285,-2.72260948787999,
7.35340977813276));
#21767=CARTESIAN_POINT('Ctrl Pts',(-6.50012585367688,-2.62985211856445,
7.34884077956032));
#21768=CARTESIAN_POINT('Ctrl Pts',(-6.53721504204028,-2.5362526604854,7.34427178098787));
#21769=CARTESIAN_POINT('Ctrl Pts',(-6.57227159525839,-2.441899392002,7.33970278241542));
#21770=CARTESIAN_POINT('Origin',(0.,0.,0.));
#21771=CARTESIAN_POINT('',(-6.57226144972351,-2.44189579807461,5.33969278385492));
#21772=CARTESIAN_POINT('',(-6.57227159525839,-2.44189939200201,5.88677413144118));
#21773=CARTESIAN_POINT('',(-6.57227159525839,-2.441899392002,0.));
#21774=CARTESIAN_POINT('',(-7.0112499977539,0.000177470811686547,7.77353435691036));
#21775=CARTESIAN_POINT('Ctrl Pts',(-6.57227159525839,-2.44189939200201,
5.88677413144118));
#21776=CARTESIAN_POINT('Ctrl Pts',(-6.50682880781099,-2.61803595785062,
5.8953040437753));
#21777=CARTESIAN_POINT('Ctrl Pts',(-6.43429692169323,-2.79155192492353,
5.90383395610941));
#21778=CARTESIAN_POINT('Ctrl Pts',(-6.35491245195174,-2.96187681893234,
5.91236386844353));
#21779=CARTESIAN_POINT('Ctrl Pts',(-6.2755220179471,-3.13221450968202,5.92089442164155));
#21780=CARTESIAN_POINT('Ctrl Pts',(-6.18927809852885,-3.29936036986028,
5.92942497483958));
#21781=CARTESIAN_POINT('Ctrl Pts',(-6.09646455045238,-3.46276573674535,
5.93795552803761));
#21782=CARTESIAN_POINT('Ctrl Pts',(-6.00365137626517,-3.6261704453697,5.94648604687123));
#21783=CARTESIAN_POINT('Ctrl Pts',(-5.90426877993716,-3.78583442615979,
5.95501656570485));
#21784=CARTESIAN_POINT('Ctrl Pts',(-5.79864578738953,-3.94123503421068,
5.96354708453847));
#21785=CARTESIAN_POINT('Ctrl Pts',(-5.69300088556608,-4.09666787686032,
5.97207937284942));
#21786=CARTESIAN_POINT('Ctrl Pts',(-5.58111317421822,-4.24783532738211,
5.98061166116036));
#21787=CARTESIAN_POINT('Ctrl Pts',(-5.4633546053563,-4.3942443057518,5.9891439494713));
#21788=CARTESIAN_POINT('Ctrl Pts',(-5.42639860225383,-4.44019162585896,
5.99182162529853));
#21789=CARTESIAN_POINT('Ctrl Pts',(-5.38886469319287,-4.4856705278481,5.99449930112576));
#21790=CARTESIAN_POINT('Ctrl Pts',(-5.35076519733763,-4.53066643723199,
5.99717697695298));
#21791=CARTESIAN_POINT('Ctrl Pts',(-5.22936194788609,-4.67404496465363,
6.00570933516681));
#21792=CARTESIAN_POINT('Ctrl Pts',(-5.1021719965233,-4.81256517858897,6.01424169338064));
#21793=CARTESIAN_POINT('Ctrl Pts',(-4.96960825326884,-4.94576792536227,
6.02277405159447));
#21794=CARTESIAN_POINT('Ctrl Pts',(-4.83706933306923,-5.07894572942494,
6.03130481209243));
#21795=CARTESIAN_POINT('Ctrl Pts',(-4.69915884485961,-5.2068078366158,6.03983557259039));
#21796=CARTESIAN_POINT('Ctrl Pts',(-4.55632697695416,-5.32893151031046,
6.04836633308835));
#21797=CARTESIAN_POINT('Ctrl Pts',(-4.40734123845651,-5.45631684791237,
6.05726463898726));
#21798=CARTESIAN_POINT('Ctrl Pts',(-4.25300090672483,-5.57745807423381,
6.06616294488617));
#21799=CARTESIAN_POINT('Ctrl Pts',(-4.09385650148087,-5.69192107357286,
6.07506125078508));
#21800=CARTESIAN_POINT('Ctrl Pts',(-3.94129027956909,-5.8016527812699,6.08359174804215));
#21801=CARTESIAN_POINT('Ctrl Pts',(-3.78430941424043,-5.90524705599592,
6.09212224529923));
#21802=CARTESIAN_POINT('Ctrl Pts',(-3.62343009969628,-6.00236460697907,
6.1006527425563));
#21803=CARTESIAN_POINT('Ctrl Pts',(-3.46254913878823,-6.09948315181797,
6.1091833271105));
#21804=CARTESIAN_POINT('Ctrl Pts',(-3.29776991256634,-6.19012468511022,
6.1177139116647));
#21805=CARTESIAN_POINT('Ctrl Pts',(-3.12963524240122,-6.27399472521457,
6.12624449621891));
#21806=CARTESIAN_POINT('Ctrl Pts',(-2.96146730226921,-6.35788136126226,
6.13477676877872));
#21807=CARTESIAN_POINT('Ctrl Pts',(-2.78994286632788,-6.43499369223092,
6.14330904133853));
#21808=CARTESIAN_POINT('Ctrl Pts',(-2.61562764909289,-6.50508405509113,
6.15184131389834));
#21809=CARTESIAN_POINT('Ctrl Pts',(-2.59312259559609,-6.51413310652106,
6.15294287722398));
#21810=CARTESIAN_POINT('Ctrl Pts',(-2.57057105215388,-6.52306517987497,
6.15404444054963));
#21811=CARTESIAN_POINT('Ctrl Pts',(-2.54797425980885,-6.53187980093415,
6.15514600387527));
#21812=CARTESIAN_POINT('Ctrl Pts',(-2.37294671279207,-6.60015504453133,
6.16367836208909));
#21813=CARTESIAN_POINT('Ctrl Pts',(-2.19514385506042,-6.66140271533437,
6.17221072030292));
#21814=CARTESIAN_POINT('Ctrl Pts',(-2.01514741149616,-6.71541565894773,
6.18074307851674));
#21815=CARTESIAN_POINT('Ctrl Pts',(-1.83518467293613,-6.76941848843629,
6.18927383901472));
#21816=CARTESIAN_POINT('Ctrl Pts',(-1.65302946121357,-6.81618920636936,
6.1978045995127));
#21817=CARTESIAN_POINT('Ctrl Pts',(-1.46927894227537,-6.85557043230439,
6.20633536001069));
#21818=CARTESIAN_POINT('Ctrl Pts',(-1.27761158425004,-6.89664838720967,
6.21523366590959));
#21819=CARTESIAN_POINT('Ctrl Pts',(-1.08420874701755,-6.92968590019265,
6.2241319718085));
#21820=CARTESIAN_POINT('Ctrl Pts',(-0.88976124239467,-6.95456335753959,
6.2330302777074));
#21821=CARTESIAN_POINT('Ctrl Pts',(-0.70335116347931,-6.97841251310603,
6.24156077496447));
#21822=CARTESIAN_POINT('Ctrl Pts',(-0.515981366956735,-6.99476259525729,
6.25009127222153));
#21823=CARTESIAN_POINT('Ctrl Pts',(-0.328267328922525,-7.00356103159401,
6.2586217694786));
#21824=CARTESIAN_POINT('Ctrl Pts',(-0.14055136991003,-7.01235955796983,
6.26715235403281));
#21825=CARTESIAN_POINT('Ctrl Pts',(0.0475085318593298,-7.01360627301243,
6.27568293858702));
#21826=CARTESIAN_POINT('Ctrl Pts',(0.235294821337802,-7.00730068639499,
6.28421352314123));
#21827=CARTESIAN_POINT('Ctrl Pts',(0.423118269384501,-7.00099385204763,
6.29274579570104));
#21828=CARTESIAN_POINT('Ctrl Pts',(0.610667691222674,-6.98713174251941,
6.30127806826084));
#21829=CARTESIAN_POINT('Ctrl Pts',(0.797327693233565,-6.96576593865333,
6.30981034082065));
#21830=CARTESIAN_POINT('Ctrl Pts',(0.82142652635651,-6.96300749583559,6.31091190414629));
#21831=CARTESIAN_POINT('Ctrl Pts',(0.845510541581198,-6.96012405055713,
6.31201346747193));
#21832=CARTESIAN_POINT('Ctrl Pts',(0.869578421780628,-6.95711577673345,
6.31311503079756));
#21833=CARTESIAN_POINT('Ctrl Pts',(1.05600054616517,-6.93381464708294,6.3216473890114));
#21834=CARTESIAN_POINT('Ctrl Pts',(1.24151697778743,-6.90301226090025,6.33017974722523));
#21835=CARTESIAN_POINT('Ctrl Pts',(1.42551753240329,-6.86480344418621,6.33871210543906));
#21836=CARTESIAN_POINT('Ctrl Pts',(1.60948363222983,-6.82660178221544,6.34724286593703));
#21837=CARTESIAN_POINT('Ctrl Pts',(1.79193412205059,-6.78099651960513,6.355773626435));
#21838=CARTESIAN_POINT('Ctrl Pts',(1.97226893932507,-6.72813360401483,6.36430438693298));
#21839=CARTESIAN_POINT('Ctrl Pts',(2.16037343114771,-6.6729931046722,6.37320269283188));
#21840=CARTESIAN_POINT('Ctrl Pts',(2.3461755609127,-6.60995578803778,6.38210099873079));
#21841=CARTESIAN_POINT('Ctrl Pts',(2.52901090012722,-6.53924540214983,6.39099930462969));
#21842=CARTESIAN_POINT('Ctrl Pts',(2.70428879879527,-6.47145780755411,6.39952980188677));
#21843=CARTESIAN_POINT('Ctrl Pts',(2.87683993367598,-6.39661883584323,6.40806029914384));
#21844=CARTESIAN_POINT('Ctrl Pts',(3.04609804559447,-6.31497531738055,6.41659079640092));
#21845=CARTESIAN_POINT('Ctrl Pts',(3.21535788962182,-6.23333096341604,6.42512138095514));
#21846=CARTESIAN_POINT('Ctrl Pts',(3.38132436916103,-6.14488205940167,6.43365196550936));
#21847=CARTESIAN_POINT('Ctrl Pts',(3.54345419590065,-6.04992222462852,6.44218255006357));
#21848=CARTESIAN_POINT('Ctrl Pts',(3.70561610438746,-5.95494359949782,6.4507148226234));
#21849=CARTESIAN_POINT('Ctrl Pts',(3.86393958024118,-5.85345162589316,6.45924709518324));
#21850=CARTESIAN_POINT('Ctrl Pts',(4.01790802965527,-5.74578468337717,6.46777936774306));
#21851=CARTESIAN_POINT('Ctrl Pts',(4.03778620349278,-5.73188428879614,6.46888093106866));
#21852=CARTESIAN_POINT('Ctrl Pts',(4.05759182677243,-5.71788102730183,6.46998249439426));
#21853=CARTESIAN_POINT('Ctrl Pts',(4.07732382407226,-5.70377567898255,6.47108405771985));
#21854=CARTESIAN_POINT('Ctrl Pts',(4.23016158230585,-5.5945201493235,6.47961641593367));
#21855=CARTESIAN_POINT('Ctrl Pts',(4.37863116505627,-5.47909954286938,6.4881487741475));
#21856=CARTESIAN_POINT('Ctrl Pts',(4.52224115074249,-5.35788778690178,6.49668113236132));
#21857=CARTESIAN_POINT('Ctrl Pts',(4.66582424492394,-5.23669872828699,6.50521189285928));
#21858=CARTESIAN_POINT('Ctrl Pts',(4.80454932429202,-5.10972088152682,6.51374265335725));
#21859=CARTESIAN_POINT('Ctrl Pts',(4.93795820962652,-4.97736830890402,6.52227341385521));
#21860=CARTESIAN_POINT('Ctrl Pts',(5.07711497901682,-4.83931336315956,6.53117171975412));
#21861=CARTESIAN_POINT('Ctrl Pts',(5.21048704681651,-4.69541052703548,6.54007002565303));
#21862=CARTESIAN_POINT('Ctrl Pts',(5.33759667764691,-4.54617292557957,6.54896833155194));
#21863=CARTESIAN_POINT('Ctrl Pts',(5.45945227234803,-4.40310401287505,6.557498828809));
#21864=CARTESIAN_POINT('Ctrl Pts',(5.57555252100228,-4.25513273830584,6.56602932606606));
#21865=CARTESIAN_POINT('Ctrl Pts',(5.68551700537223,-4.10274578107432,6.57455982332311));
#21866=CARTESIAN_POINT('Ctrl Pts',(5.79548261506783,-3.95035726438521,6.58309040787733));
#21867=CARTESIAN_POINT('Ctrl Pts',(5.89931215858357,-3.79355322475207,6.59162099243155));
#21868=CARTESIAN_POINT('Ctrl Pts',(5.99666769607275,-3.63285054817529,6.60015157698577));
#21869=CARTESIAN_POINT('Ctrl Pts',(6.09404249797358,-3.47211607225157,6.60868384954558));
#21870=CARTESIAN_POINT('Ctrl Pts',(6.18494057752728,-3.30748168080824,6.6172161221054));
#21871=CARTESIAN_POINT('Ctrl Pts',(6.26906878175907,-3.13949090969761,6.62574839466522));
#21872=CARTESIAN_POINT('Ctrl Pts',(6.27993019573572,-3.11780237698791,6.62684995799086));
#21873=CARTESIAN_POINT('Ctrl Pts',(6.29067883110952,-3.09605793209677,6.6279515213165));
#21874=CARTESIAN_POINT('Ctrl Pts',(6.30131411363566,-3.07425877306971,6.62905308464214));
#21875=CARTESIAN_POINT('Ctrl Pts',(6.38369162031749,-2.9054094393547,6.63758544285598));
#21876=CARTESIAN_POINT('Ctrl Pts',(6.45929239905691,-2.73321868568166,6.64611780106983));
#21877=CARTESIAN_POINT('Ctrl Pts',(6.52786235853414,-2.5582493214175,6.65465015928367));
#21878=CARTESIAN_POINT('Ctrl Pts',(6.59641947803105,-2.38331272081854,6.66318091978166));
#21879=CARTESIAN_POINT('Ctrl Pts',(6.65794829400971,-2.20559883273443,6.67171168027964));
#21880=CARTESIAN_POINT('Ctrl Pts',(6.71224305762752,-2.02568993131505,6.68024244077763));
#21881=CARTESIAN_POINT('Ctrl Pts',(6.76887709576443,-1.83802970581198,6.68914074667653));
#21882=CARTESIAN_POINT('Ctrl Pts',(6.81763979496159,-1.64798146488188,6.69803905257543));
#21883=CARTESIAN_POINT('Ctrl Pts',(6.8583553784182,-1.45622390648628,6.70693735847433));
#21884=CARTESIAN_POINT('Ctrl Pts',(6.89738799619325,-1.27239258572658,6.71546785573141));
#21885=CARTESIAN_POINT('Ctrl Pts',(6.92902530509543,-1.0869907342772,6.7239983529885));
#21886=CARTESIAN_POINT('Ctrl Pts',(6.9531645131237,-0.900627456797393,6.73252885024558));
#21887=CARTESIAN_POINT('Ctrl Pts',(6.97730396818145,-0.714262272162066,
6.74105943479982));
#21888=CARTESIAN_POINT('Ctrl Pts',(6.99394513293989,-0.526935945694958,
6.74959001935406));
#21889=CARTESIAN_POINT('Ctrl Pts',(7.00303695235466,-0.339263918587315,
6.75812060390831));
#21890=CARTESIAN_POINT('Ctrl Pts',(7.01213057083044,-0.151554755521377,
6.76665287646815));
#21891=CARTESIAN_POINT('Ctrl Pts',(7.01367184653439,0.0364999391338565,
6.77518514902799));
#21892=CARTESIAN_POINT('Ctrl Pts',(7.00766179772167,0.224282614690158,6.78371742158783));
#21893=CARTESIAN_POINT('Ctrl Pts',(7.00688586735725,0.248526391141561,6.78481898491336));
#21894=CARTESIAN_POINT('Ctrl Pts',(7.00598414096941,0.272765634847337,6.7859205482389));
#21895=CARTESIAN_POINT('Ctrl Pts',(7.00495668404128,0.29699901886284,6.78702211156443));
#21896=CARTESIAN_POINT('Ctrl Pts',(6.99699833034799,0.484703083042002,6.79555446977824));
#21897=CARTESIAN_POINT('Ctrl Pts',(6.9814897493047,0.672118710219353,6.80408682799206));
#21898=CARTESIAN_POINT('Ctrl Pts',(6.95847548566177,0.858630000608037,6.81261918620587));
#21899=CARTESIAN_POINT('Ctrl Pts',(6.93546553152544,1.04510636606285,6.82114994670383));
#21900=CARTESIAN_POINT('Ctrl Pts',(6.90495273704113,1.23067842911714,6.82968070720178));
#21901=CARTESIAN_POINT('Ctrl Pts',(6.86703342573563,1.41473619177908,6.83821146769974));
#21902=CARTESIAN_POINT('Ctrl Pts',(6.82748037163766,1.60672403103774,6.84710977359866));
#21903=CARTESIAN_POINT('Ctrl Pts',(6.77986849625049,1.7970638430474,6.85600807949757));
#21904=CARTESIAN_POINT('Ctrl Pts',(6.72436639184739,1.98507510958485,6.86490638539648));
#21905=CARTESIAN_POINT('Ctrl Pts',(6.67115844926261,2.16531499026689,6.87343688265354));
#21906=CARTESIAN_POINT('Ctrl Pts',(6.61069953596366,2.34341464113093,6.88196737991059));
#21907=CARTESIAN_POINT('Ctrl Pts',(6.54318928729587,2.5187894936093,6.89049787716764));
#21908=CARTESIAN_POINT('Ctrl Pts',(6.47567834775942,2.69416614079279,6.89902846172186));
#21909=CARTESIAN_POINT('Ctrl Pts',(6.40111604160243,2.86681764948153,6.90755904627607));
#21910=CARTESIAN_POINT('Ctrl Pts',(6.31975051687379,3.03617851368682,6.91608963083029));
#21911=CARTESIAN_POINT('Ctrl Pts',(6.23836889178763,3.2055728904943,6.9246219033901));
#21912=CARTESIAN_POINT('Ctrl Pts',(6.15018149279767,3.37167504692766,6.93315417594991));
#21913=CARTESIAN_POINT('Ctrl Pts',(6.05548326370981,3.53394241682436,6.94168644850973));
#21914=CARTESIAN_POINT('Ctrl Pts',(6.04325720137559,3.55489202695198,6.94278801183539));
#21915=CARTESIAN_POINT('Ctrl Pts',(6.03092267699611,3.57577775304378,6.94388957516106));
#21916=CARTESIAN_POINT('Ctrl Pts',(6.01848037998295,3.59659845941416,6.94499113848673));
#21917=CARTESIAN_POINT('Ctrl Pts',(5.92210631537353,3.75786901089114,6.95352349670056));
#21918=CARTESIAN_POINT('Ctrl Pts',(5.81923020290133,3.91529086095971,6.96205585491439));
#21919=CARTESIAN_POINT('Ctrl Pts',(5.71018447586521,4.06834362045391,6.97058821312823));
#21920=CARTESIAN_POINT('Ctrl Pts',(5.6011591680477,4.22136772024872,6.9791189736262));
#21921=CARTESIAN_POINT('Ctrl Pts',(5.48596672866222,4.37002411305445,6.98764973412417));
#21922=CARTESIAN_POINT('Ctrl Pts',(5.36498231317421,4.51382225412432,6.99618049462214));
#21923=CARTESIAN_POINT('Ctrl Pts',(5.2387853183965,4.66381589739185,7.00507880052105));
#21924=CARTESIAN_POINT('Ctrl Pts',(5.10628640972892,4.80852309802665,7.01397710641995));
#21925=CARTESIAN_POINT('Ctrl Pts',(4.96795787146739,4.94742570937909,7.02287541231886));
#21926=CARTESIAN_POINT('Ctrl Pts',(4.83534709930238,5.08058682550653,7.03140590957593));
#21927=CARTESIAN_POINT('Ctrl Pts',(4.69737917041945,5.20841333463145,7.039936406833));
#21928=CARTESIAN_POINT('Ctrl Pts',(4.55450798055072,5.33048624588787,7.04846690409006));
#21929=CARTESIAN_POINT('Ctrl Pts',(4.41163532860432,5.45256040638202,7.0569974886443));
#21930=CARTESIAN_POINT('Ctrl Pts',(4.2638595501344,5.56888065504789,7.06552807319853));
#21931=CARTESIAN_POINT('Ctrl Pts',(4.1116681244352,5.67906786339128,7.07405865775276));
#21932=CARTESIAN_POINT('Ctrl Pts',(3.95944658356889,5.78927687523757,7.0825909303126));
#21933=CARTESIAN_POINT('Ctrl Pts',(3.80280789877415,5.89335024425383,7.09112320287243));
#21934=CARTESIAN_POINT('Ctrl Pts',(3.64226977692717,5.99095129629535,7.09965547543227));
#21935=CARTESIAN_POINT('Ctrl Pts',(3.6215434222375,6.00355212904102,7.10075703875785));
#21936=CARTESIAN_POINT('Ctrl Pts',(3.60075210862899,6.01604514006274,7.10185860208343));
#21937=CARTESIAN_POINT('Ctrl Pts',(3.57989698310413,6.02842965894618,7.10296016540901));
#21938=CARTESIAN_POINT('Ctrl Pts',(3.41835983181994,6.12435619259717,7.11149252362287));
#21939=CARTESIAN_POINT('Ctrl Pts',(3.25293759185595,6.21380235473935,7.12002488183674));
#21940=CARTESIAN_POINT('Ctrl Pts',(3.0841703773126,6.29646882357147,7.1285572400506));
#21941=CARTESIAN_POINT('Ctrl Pts',(2.91543476505874,6.37911981279941,7.13708800054861));
#21942=CARTESIAN_POINT('Ctrl Pts',(2.74335570288163,6.45499350767554,7.14561876104662));
#21943=CARTESIAN_POINT('Ctrl Pts',(2.5684966626602,6.52383717273841,7.15414952154463));
#21944=CARTESIAN_POINT('Ctrl Pts',(2.38610387019588,6.5956469476199,7.16304782744352));
#21945=CARTESIAN_POINT('Ctrl Pts',(2.20068656367103,6.6598073493845,7.17194613334241));
#21946=CARTESIAN_POINT('Ctrl Pts',(2.01290676914888,6.7160876186374,7.1808444392413));
#21947=CARTESIAN_POINT('Ctrl Pts',(1.83288879265856,6.77004156087608,7.1893749364984));
#21948=CARTESIAN_POINT('Ctrl Pts',(1.65070001986629,6.81675362467141,7.1979054337555));
#21949=CARTESIAN_POINT('Ctrl Pts',(1.4669390933311,6.85607148875775,7.2064359310126));
#21950=CARTESIAN_POINT('Ctrl Pts',(1.28317628627127,6.895389755205,7.21496651556688));
#21951=CARTESIAN_POINT('Ctrl Pts',(1.09784159320238,6.92731360988328,7.22349710012115));
#21952=CARTESIAN_POINT('Ctrl Pts',(0.911544208239945,6.95174177590942,7.23202768467543));
#21953=CARTESIAN_POINT('Ctrl Pts',(0.725209959329432,6.9761747757052,7.24055995723529));
#21954=CARTESIAN_POINT('Ctrl Pts',(0.537912941574896,6.99310908564368,7.24909222979515));
#21955=CARTESIAN_POINT('Ctrl Pts',(0.350268715347714,7.00249515455375,7.25762450235502));
#21956=CARTESIAN_POINT('Ctrl Pts',(0.326042813468689,7.00370694768491,7.25872606568044));
#21957=CARTESIAN_POINT('Ctrl Pts',(0.301811128741358,7.00479299605894,7.25982762900587));
#21958=CARTESIAN_POINT('Ctrl Pts',(0.277574989016439,7.00575325628676,7.2609291923313));
#21959=CARTESIAN_POINT('Ctrl Pts',(0.0898495799762925,7.01319112577005,
7.26946155054498));
#21960=CARTESIAN_POINT('Ctrl Pts',(-0.0982065849261312,7.01308050338434,
7.27799390875865));
#21961=CARTESIAN_POINT('Ctrl Pts',(-0.285976026660372,7.00541535347302,
7.28652626697233));
#21962=CARTESIAN_POINT('Ctrl Pts',(-0.473710307867084,6.99775163888959,
7.29505702747014));
#21963=CARTESIAN_POINT('Ctrl Pts',(-0.661157667450308,6.98253623230388,
7.30358778796795));
#21964=CARTESIAN_POINT('Ctrl Pts',(-0.847702268630366,6.95981518621428,
7.31211854846576));
#21965=CARTESIAN_POINT('Ctrl Pts',(-1.0422840911455,6.93611521028575,7.32101685436475));
#21966=CARTESIAN_POINT('Ctrl Pts',(-1.23588328914684,6.90424853101671,7.32991516026374));
#21967=CARTESIAN_POINT('Ctrl Pts',(-1.42780782494848,6.86432745267269,7.33881346616272));
#21968=CARTESIAN_POINT('Ctrl Pts',(-1.61179922115094,6.82605649939542,7.34734396341964));
#21969=CARTESIAN_POINT('Ctrl Pts',(-1.79425129499676,6.78038367833697,7.35587446067656));
#21970=CARTESIAN_POINT('Ctrl Pts',(-1.97456509440836,6.7274600891008,7.36440495793347));
#21971=CARTESIAN_POINT('Ctrl Pts',(-2.15488073906802,6.67453595826908,7.37293554248755));
#21972=CARTESIAN_POINT('Ctrl Pts',(-2.33305777288539,6.61436100026425,7.38146612704163));
#21973=CARTESIAN_POINT('Ctrl Pts',(-2.50851227005572,6.54713622536448,7.38999671159571));
#21974=CARTESIAN_POINT('Ctrl Pts',(-2.68400148561738,6.47989814823491,7.39852898415539));
#21975=CARTESIAN_POINT('Ctrl Pts',(-2.85676680316761,6.40560757842252,7.40706125671506));
#21976=CARTESIAN_POINT('Ctrl Pts',(-3.02624332798837,6.32451404317406,7.41559352927474));
#21977=CARTESIAN_POINT('Ctrl Pts',(-3.04812367968867,6.31404442165135,7.41669509260102));
#21978=CARTESIAN_POINT('Ctrl Pts',(-3.06994924291164,6.30346147136759,7.41779665592731));
#21979=CARTESIAN_POINT('Ctrl Pts',(-3.09171882933512,6.29276578642767,7.41889821925359));
#21980=CARTESIAN_POINT('Ctrl Pts',(-3.26033910300386,6.20992042195635,7.42743057746785));
#21981=CARTESIAN_POINT('Ctrl Pts',(-3.42565599669303,6.12027970542182,7.4359629356821));
#21982=CARTESIAN_POINT('Ctrl Pts',(-3.58712364851452,6.0241323435635,7.44449529389636));
#21983=CARTESIAN_POINT('Ctrl Pts',(-3.74856106491702,5.92800298565668,7.45302605439477));
#21984=CARTESIAN_POINT('Ctrl Pts',(-3.90615041507955,5.82536957037436,7.46155681489318));
#21985=CARTESIAN_POINT('Ctrl Pts',(-4.05937208316045,5.71656582687172,7.47008757539159));
#21986=CARTESIAN_POINT('Ctrl Pts',(-4.21919526342033,5.60307430489202,7.47898588129028));
#21987=CARTESIAN_POINT('Ctrl Pts',(-4.37426576303427,5.48286916830799,7.48788418718898));
#21988=CARTESIAN_POINT('Ctrl Pts',(-4.52402850388408,5.35637868886661,7.49678249308767));
#21989=CARTESIAN_POINT('Ctrl Pts',(-4.66760084952371,5.23511665311973,7.50531299034516));
#21990=CARTESIAN_POINT('Ctrl Pts',(-4.80629515369875,5.10807864373607,7.51384348760265));
#21991=CARTESIAN_POINT('Ctrl Pts',(-4.93965666680029,4.97568272467563,7.52237398486015));
#21992=CARTESIAN_POINT('Ctrl Pts',(-5.0730195446616,4.84328545073686,7.53090456941479));
#21993=CARTESIAN_POINT('Ctrl Pts',(-5.2010493075339,4.70553037542458,7.53943515396942));
#21994=CARTESIAN_POINT('Ctrl Pts',(-5.32332818445081,4.56287229748233,7.54796573852406));
#21995=CARTESIAN_POINT('Ctrl Pts',(-5.44563125753255,4.42018599080216,7.55649801108431));
#21996=CARTESIAN_POINT('Ctrl Pts',(-5.56218097344242,4.27259497672134,7.56503028364456));
#21997=CARTESIAN_POINT('Ctrl Pts',(-5.67259939792344,4.1205876562911,7.57356255620481));
#21998=CARTESIAN_POINT('Ctrl Pts',(-5.6868550239374,4.10096267502895,7.5746641195285));
#21999=CARTESIAN_POINT('Ctrl Pts',(-5.70100850922268,4.08126412436603,7.57576568285219));
#22000=CARTESIAN_POINT('Ctrl Pts',(-5.71505909169781,4.06149309255872,7.57686724617588));
#22001=CARTESIAN_POINT('Ctrl Pts',(-5.82389042277067,3.90835298522994,7.58539960438882));
#22002=CARTESIAN_POINT('Ctrl Pts',(-5.92658126006227,3.75081021222684,7.59393196260177));
#22003=CARTESIAN_POINT('Ctrl Pts',(-6.0227890614943,3.58937856505058,7.60246432081471));
#22004=CARTESIAN_POINT('Ctrl Pts',(-6.11897884765724,3.42797714655143,7.6109950813118));
#22005=CARTESIAN_POINT('Ctrl Pts',(-6.20868786402214,3.26268856984593,7.61952584180889));
#22006=CARTESIAN_POINT('Ctrl Pts',(-6.29161808584567,3.0940537203416,7.62805660230599));
#22007=CARTESIAN_POINT('Ctrl Pts',(-6.37812133281153,2.91815328606126,7.63695490820534));
#22008=CARTESIAN_POINT('Ctrl Pts',(-6.45724854463065,2.73861215131085,7.64585321410469));
#22009=CARTESIAN_POINT('Ctrl Pts',(-6.52871552906283,2.5560712241786,7.65475152000403));
#22010=CARTESIAN_POINT('Ctrl Pts',(-6.59722844843226,2.38107556819003,7.66328201726022));
#22011=CARTESIAN_POINT('Ctrl Pts',(-6.6587015552587,2.20332342906014,7.67181251451641));
#22012=CARTESIAN_POINT('Ctrl Pts',(-6.71293402198084,2.02339896684566,7.68034301177259));
#22013=CARTESIAN_POINT('Ctrl Pts',(-6.767167043693,1.84347266336737,7.68887359632595));
#22014=CARTESIAN_POINT('Ctrl Pts',(-6.81415919203053,1.66137428627552,7.6974041808793));
#22015=CARTESIAN_POINT('Ctrl Pts',(-6.85375964843323,1.47770269134507,7.70593476543265));
#22016=CARTESIAN_POINT('Ctrl Pts',(-6.89336794085143,1.29399475204902,7.71446703799162));
#22017=CARTESIAN_POINT('Ctrl Pts',(-6.92558155650827,1.10871327247893,7.7229993105506));
#22018=CARTESIAN_POINT('Ctrl Pts',(-6.95030070758529,0.922467688669611,
7.73153158310957));
#22019=CARTESIAN_POINT('Ctrl Pts',(-6.95349208598717,0.898422359128844,
7.7326331464391));
#22020=CARTESIAN_POINT('Ctrl Pts',(-6.95655861538189,0.874360969982549,
7.73373470976863));
#22021=CARTESIAN_POINT('Ctrl Pts',(-6.95950014379961,0.850284841069851,
7.73483627309817));
#22022=CARTESIAN_POINT('Ctrl Pts',(-6.98345968606632,0.654178277955419,
7.74380880349918));
#22023=CARTESIAN_POINT('Ctrl Pts',(-6.9991270096246,0.45705027964632,7.75278133390019));
#22024=CARTESIAN_POINT('Ctrl Pts',(-7.00644302121596,0.259581881020636,
7.7617538643012));
#22025=CARTESIAN_POINT('Ctrl Pts',(-7.0096448760859,0.173159771664506,7.76568069517092));
#22026=CARTESIAN_POINT('Ctrl Pts',(-7.01124780836569,0.0866725284477343,
7.76960752604064));
#22027=CARTESIAN_POINT('Ctrl Pts',(-7.0112499977539,0.000177470811686547,
7.77353435691036));
#22028=CARTESIAN_POINT('Ctrl Pts',(-7.01119847445136,0.000177469507514665,
7.77353435691036));
#22029=CARTESIAN_POINT('Ctrl Pts',(-7.01036852730354,-0.831199708459484,
7.81127872708187));
#22030=CARTESIAN_POINT('Ctrl Pts',(-6.86199980275722,-1.66286473245636,
7.84902309725337));
#22031=CARTESIAN_POINT('Ctrl Pts',(-6.57280081548428,-2.44209581534395,
7.88676746742488));
#22032=CARTESIAN_POINT('',(-7.01124999795275,-0.00016943300568554,7.22646564308963));
#22033=CARTESIAN_POINT('Ctrl Pts',(-6.57227159525839,-2.441899392002,7.33970278241542));
#22034=CARTESIAN_POINT('Ctrl Pts',(-6.63772323604687,-2.26573899775066,
7.33117232445892));
#22035=CARTESIAN_POINT('Ctrl Pts',(-6.69608654756327,-2.08695006746432,
7.32264186650241));
#22036=CARTESIAN_POINT('Ctrl Pts',(-6.74717209576847,-1.90612047693302,
7.31411140854591));
#22037=CARTESIAN_POINT('Ctrl Pts',(-6.79826929134116,-1.72524965774176,
7.30557900566795));
#22038=CARTESIAN_POINT('Ctrl Pts',(-6.84208532452037,-1.54233754315333,
7.29704660278999));
#22039=CARTESIAN_POINT('Ctrl Pts',(-6.8784809730595,-1.35798603297619,7.28851419991204));
#22040=CARTESIAN_POINT('Ctrl Pts',(-6.901647218676,-1.24064419305973,7.28308322811449));
#22041=CARTESIAN_POINT('Ctrl Pts',(-6.92180813642338,-1.12271944697059,
7.27765225631694));
#22042=CARTESIAN_POINT('Ctrl Pts',(-6.93893863521853,-1.00436904530736,
7.27222128451938));
#22043=CARTESIAN_POINT('Ctrl Pts',(-6.96699642709752,-0.810524664103404,
7.263325975736));
#22044=CARTESIAN_POINT('Ctrl Pts',(-6.98692870444038,-0.615493148353179,
7.25443066695261));
#22045=CARTESIAN_POINT('Ctrl Pts',(-6.99866239872024,-0.419941890312867,
7.24553535816922));
#22046=CARTESIAN_POINT('Ctrl Pts',(-7.00704727559547,-0.280201312251252,
7.23917878647602));
#22047=CARTESIAN_POINT('Ctrl Pts',(-7.01124661409999,-0.140195501486346,
7.23282221478283));
#22048=CARTESIAN_POINT('Ctrl Pts',(-7.01124999795275,-0.00016943300568554,
7.22646564308963));
#22049=CARTESIAN_POINT('Ctrl Pts',(-7.0110449382642,-0.000169428050237619,
7.22646564308963));
#22050=CARTESIAN_POINT('Ctrl Pts',(-7.01028915262695,0.823772614993853,
7.18906118125878));
#22051=CARTESIAN_POINT('Ctrl Pts',(-6.66051850280413,2.80824854701764,7.09900037712055));
#22052=CARTESIAN_POINT('Ctrl Pts',(-4.82814950876211,5.48279137105804,6.95628323067478));
#22053=CARTESIAN_POINT('Ctrl Pts',(-1.63504874432568,7.12029806266455,6.7983142037525));
#22054=CARTESIAN_POINT('Ctrl Pts',(1.95254792752263,7.0398569224263,6.64034517683023));
#22055=CARTESIAN_POINT('Ctrl Pts',(5.06904416942584,5.26087636291873,6.48237614990793));
#22056=CARTESIAN_POINT('Ctrl Pts',(6.96250826242842,2.21257939815105,6.32440712298563));
#22057=CARTESIAN_POINT('Ctrl Pts',(7.17609521147244,-1.36955701355905,6.16643809606336));
#22058=CARTESIAN_POINT('Ctrl Pts',(5.65827188791764,-4.62125395752143,6.00846906914106));
#22059=CARTESIAN_POINT('Ctrl Pts',(2.77525067007686,-6.75795920494823,5.85050004221877));
#22060=CARTESIAN_POINT('Ctrl Pts',(-0.777368341216584,-7.26413982241399,
5.69253101529648));
#22061=CARTESIAN_POINT('Ctrl Pts',(-4.14242803342189,-6.01766722953563,
5.53456198837419));
#22062=CARTESIAN_POINT('Ctrl Pts',(-5.90368661682782,-4.00863867080895,
5.41694924456034));
#22063=CARTESIAN_POINT('Ctrl Pts',(-6.47816622693472,-2.69595371960147,
5.35199284305391));
#22064=CARTESIAN_POINT('Ctrl Pts',(-6.57226144972351,-2.44189579807461,
5.33969278385492));
#22065=CARTESIAN_POINT('Origin',(0.,0.,0.));
#22066=CARTESIAN_POINT('',(-6.5722715952584,-2.44189939200197,3.33970491700474));
#22067=CARTESIAN_POINT('',(-6.57188903190969,-2.44175767753665,3.88676355207028));
#22068=CARTESIAN_POINT('',(-6.57227159525839,-2.441899392002,0.));
#22069=CARTESIAN_POINT('',(-7.01105936472711,-8.57079543653067E-5,5.77353435691036));
#22070=CARTESIAN_POINT('Ctrl Pts',(-6.57188903190969,-2.44175767753665,
3.88676355207028));
#22071=CARTESIAN_POINT('Ctrl Pts',(-6.42685604719305,-2.83295247522456,
3.90570224370127));
#22072=CARTESIAN_POINT('Ctrl Pts',(-5.74776975712297,-4.26300939817711,
3.97729727763977));
#22073=CARTESIAN_POINT('Ctrl Pts',(-3.75801643412087,-6.26492947912218,
4.10154865388543));
#22074=CARTESIAN_POINT('Ctrl Pts',(-0.321596567147127,-7.29853441079176,
4.25951768080783));
#22075=CARTESIAN_POINT('Ctrl Pts',(3.19241641747391,-6.57118758786775,4.41748670773006));
#22076=CARTESIAN_POINT('Ctrl Pts',(5.93618006499142,-4.25837940224982,4.57545573465238));
#22077=CARTESIAN_POINT('Ctrl Pts',(7.2476936041087,-0.918131972250711,4.73342476157467));
#22078=CARTESIAN_POINT('Ctrl Pts',(6.81052198939154,2.64363748072991,4.89139378849694));
#22079=CARTESIAN_POINT('Ctrl Pts',(4.7301436742755,5.56756407401104,5.04936281541924));
#22080=CARTESIAN_POINT('Ctrl Pts',(1.50850132807235,7.14817827426755,5.20733184234154));
#22081=CARTESIAN_POINT('Ctrl Pts',(-2.07710423471086,7.00411785278149,5.36530086926381));
#22082=CARTESIAN_POINT('Ctrl Pts',(-5.16155708097404,5.17014094559845,5.52326989618611));
#22083=CARTESIAN_POINT('Ctrl Pts',(-6.7457960670029,2.51575743913742,5.65934772540162));
#22084=CARTESIAN_POINT('Ctrl Pts',(-7.01043408368973,0.677693690487587,
5.7427692123097));
#22085=CARTESIAN_POINT('Ctrl Pts',(-7.01072884945883,-8.57039139217561E-5,
5.77353435691036));
#22086=CARTESIAN_POINT('Ctrl Pts',(-7.01124999947611,-8.57102848142028E-5,
5.77353435691036));
#22087=CARTESIAN_POINT('Ctrl Pts',(-7.01124765095286,-0.192198986928101,
5.78225393955636));
#22088=CARTESIAN_POINT('Ctrl Pts',(-7.00334490103907,-0.384283885227448,
5.79097352220236));
#22089=CARTESIAN_POINT('Ctrl Pts',(-6.9875747245799,-0.575696127233885,
5.79969310484836));
#22090=CARTESIAN_POINT('Ctrl Pts',(-6.97179945475511,-0.767170190522794,
5.80841550369763));
#22091=CARTESIAN_POINT('Ctrl Pts',(-6.94815170444357,-0.95797088838034,
5.81713790254689));
#22092=CARTESIAN_POINT('Ctrl Pts',(-6.91671637063173,-1.14745858780829,
5.82586030139616));
#22093=CARTESIAN_POINT('Ctrl Pts',(-6.90068149315975,-1.24411453747826,
5.83030951760767));
#22094=CARTESIAN_POINT('Ctrl Pts',(-6.88262117299095,-1.34042896470014,
5.83475873381918));
#22095=CARTESIAN_POINT('Ctrl Pts',(-6.86255182738119,-1.43631785444836,
5.83920795003069));
#22096=CARTESIAN_POINT('Ctrl Pts',(-6.82406356285709,-1.62021009614443,
5.84774049582481));
#22097=CARTESIAN_POINT('Ctrl Pts',(-6.7781730643909,-1.80258540508638,5.85627304161894));
#22098=CARTESIAN_POINT('Ctrl Pts',(-6.7250248124813,-1.98284337102325,5.86480558741307));
#22099=CARTESIAN_POINT('Ctrl Pts',(-6.67941162972341,-2.13754534612922,
5.87212843542244));
#22100=CARTESIAN_POINT('Ctrl Pts',(-6.62845360124105,-2.29068783787579,
5.87945128343181));
#22101=CARTESIAN_POINT('Ctrl Pts',(-6.57227159525839,-2.44189939200201,
5.88677413144118));
#22102=CARTESIAN_POINT('',(-7.01128832852494,5.85639662721804E-5,5.22646564376811));
#22103=CARTESIAN_POINT('Ctrl Pts',(-6.57226144972351,-2.44189579807461,
5.33969278385492));
#22104=CARTESIAN_POINT('Ctrl Pts',(-6.86098992792226,-1.66232639080036,
5.30195040683487));
#22105=CARTESIAN_POINT('Ctrl Pts',(-7.01142817074718,-0.831069413347963,
5.26420802981482));
#22106=CARTESIAN_POINT('Ctrl Pts',(-7.01179827228896,5.836945010246E-5,
5.22646565279477));
#22107=CARTESIAN_POINT('Ctrl Pts',(-7.01124999975529,5.85785866401273E-5,
5.22646564308964));
#22108=CARTESIAN_POINT('Ctrl Pts',(-7.01124951887446,0.0576150329797373,
5.2238517402363));
#22109=CARTESIAN_POINT('Ctrl Pts',(-7.01054027751411,0.115170190668486,
5.22123783738296));
#22110=CARTESIAN_POINT('Ctrl Pts',(-7.00912252417848,0.172707856086104,
5.21862393452962));
#22111=CARTESIAN_POINT('Ctrl Pts',(-7.00449466308461,0.36052354766447,5.210091576316));
#22112=CARTESIAN_POINT('Ctrl Pts',(-6.99231264643713,0.548184763330246,
5.20155921810237));
#22113=CARTESIAN_POINT('Ctrl Pts',(-6.97261008798218,0.735074910107246,
5.19302685988874));
#22114=CARTESIAN_POINT('Ctrl Pts',(-6.95291121890469,0.921930061008123,
5.18449609939096));
#22115=CARTESIAN_POINT('Ctrl Pts',(-6.92569465043421,1.10801412699093,5.17596533889318));
#22116=CARTESIAN_POINT('Ctrl Pts',(-6.89104587162625,1.29271549756429,5.1674345783954));
#22117=CARTESIAN_POINT('Ctrl Pts',(-6.85490425999147,1.48537467440484,5.1585362724964));
#22118=CARTESIAN_POINT('Ctrl Pts',(-6.81067586429655,1.6765290197093,5.14963796659739));
#22119=CARTESIAN_POINT('Ctrl Pts',(-6.75851718018267,1.8654951320429,5.14073966069838));
#22120=CARTESIAN_POINT('Ctrl Pts',(-6.7085144586752,2.04665039026863,5.13220916344149));
#22121=CARTESIAN_POINT('Ctrl Pts',(-6.65122394657964,2.22579436325577,5.1236786661846));
#22122=CARTESIAN_POINT('Ctrl Pts',(-6.58683487955106,2.40233903353161,5.11514816892771));
#22123=CARTESIAN_POINT('Ctrl Pts',(-6.52244515359446,2.57888551048419,5.10661758437365));
#22124=CARTESIAN_POINT('Ctrl Pts',(-6.45095683542565,2.75283234522419,5.09808699981958));
#22125=CARTESIAN_POINT('Ctrl Pts',(-6.37260800387816,2.92360971940647,5.08955641526551));
#22126=CARTESIAN_POINT('Ctrl Pts',(-6.29424366890735,3.09442088648488,5.08102414270588));
#22127=CARTESIAN_POINT('Ctrl Pts',(-6.2090162376767,3.26206106268585,5.07249187014626));
#22128=CARTESIAN_POINT('Ctrl Pts',(-6.11721098429106,3.42598253588204,5.06395959758663));
#22129=CARTESIAN_POINT('Ctrl Pts',(-6.10535842102635,3.4471456998607,5.06285803426018));
#22130=CARTESIAN_POINT('Ctrl Pts',(-6.09339627968944,3.46824691360584,5.06175647093374));
#22131=CARTESIAN_POINT('Ctrl Pts',(-6.08132522944022,3.48928502938265,5.06065490760729));
#22132=CARTESIAN_POINT('Ctrl Pts',(-5.98782672393285,3.65223956467251,5.05212254939338));
#22133=CARTESIAN_POINT('Ctrl Pts',(-5.88775893032056,3.81146132850706,5.04359019117947));
#22134=CARTESIAN_POINT('Ctrl Pts',(-5.78144499964938,3.96642411732901,5.03505783296557));
#22135=CARTESIAN_POINT('Ctrl Pts',(-5.67515097665782,4.1213578887914,5.02652707246753));
#22136=CARTESIAN_POINT('Ctrl Pts',(-5.5626133237529,4.27203402456879,5.01799631196949));
#22137=CARTESIAN_POINT('Ctrl Pts',(-5.44419843676668,4.4179554030804,5.00946555147145));
#22138=CARTESIAN_POINT('Ctrl Pts',(-5.32068167790026,4.57016376287194,5.00056724557258));
#22139=CARTESIAN_POINT('Ctrl Pts',(-5.19077023271126,4.71719828644467,4.99166893967371));
#22140=CARTESIAN_POINT('Ctrl Pts',(-5.05492712101795,4.85853253191714,4.98277063377484));
#22141=CARTESIAN_POINT('Ctrl Pts',(-4.92469904110363,4.99402477134385,4.97424013651771));
#22142=CARTESIAN_POINT('Ctrl Pts',(-4.78902002914748,5.12427826093411,4.96570963926059));
#22143=CARTESIAN_POINT('Ctrl Pts',(-4.64833647798779,5.24886602514373,4.95717914200346));
#22144=CARTESIAN_POINT('Ctrl Pts',(-4.50765148713798,5.37345506432665,4.94864855744918));
#22145=CARTESIAN_POINT('Ctrl Pts',(-4.36196208595718,5.49237806183363,4.94011797289491));
#22146=CARTESIAN_POINT('Ctrl Pts',(-4.21174895258767,5.60524730256183,4.93158738834063));
#22147=CARTESIAN_POINT('Ctrl Pts',(-4.06150609550943,5.71813887750516,4.92305511578076));
#22148=CARTESIAN_POINT('Ctrl Pts',(-3.906737963619,5.82497412011798,4.91452284322088));
#22149=CARTESIAN_POINT('Ctrl Pts',(-3.74795621088343,5.92540722683263,4.905990570661));
#22150=CARTESIAN_POINT('Ctrl Pts',(-3.72745661311323,5.93837369341327,4.90488900733568));
#22151=CARTESIAN_POINT('Ctrl Pts',(-3.70689015424685,5.95123350738451,4.90378744401036));
#22152=CARTESIAN_POINT('Ctrl Pts',(-3.68625796921544,5.96398597809348,4.90268588068505));
#22153=CARTESIAN_POINT('Ctrl Pts',(-3.52644764385761,6.06276254926201,4.89415352247125));
#22154=CARTESIAN_POINT('Ctrl Pts',(-3.36263790090961,6.15512867677351,4.88562116425744));
#22155=CARTESIAN_POINT('Ctrl Pts',(-3.19536346054325,6.24077550609899,4.87708880604364));
#22156=CARTESIAN_POINT('Ctrl Pts',(-3.02812034293867,6.32640629773678,4.86855804554568));
#22157=CARTESIAN_POINT('Ctrl Pts',(-2.85741409488146,6.40532016272714,4.86002728504772));
#22158=CARTESIAN_POINT('Ctrl Pts',(-2.68380361693303,6.47725441126387,4.85149652454976));
#22159=CARTESIAN_POINT('Ctrl Pts',(-2.50271318069211,6.55228792653388,4.84259821865084));
#22160=CARTESIAN_POINT('Ctrl Pts',(-2.3184630319374,6.61972691672231,4.83369991275192));
#22161=CARTESIAN_POINT('Ctrl Pts',(-2.1317109996931,6.67932891661187,4.82480160685301));
#22162=CARTESIAN_POINT('Ctrl Pts',(-1.95267830325577,6.73646728680816,4.81627110959596));
#22163=CARTESIAN_POINT('Ctrl Pts',(-1.7713467053569,6.78640342040452,4.80774061233891));
#22164=CARTESIAN_POINT('Ctrl Pts',(-1.58831205271651,6.82897440218482,4.79921011508187));
#22165=CARTESIAN_POINT('Ctrl Pts',(-1.40527552698445,6.87154581961678,4.79067953052767));
#22166=CARTESIAN_POINT('Ctrl Pts',(-1.22053621044141,6.90675186845741,4.78214894597348));
#22167=CARTESIAN_POINT('Ctrl Pts',(-1.03470140506026,6.93448048269417,4.77361836141928));
#22168=CARTESIAN_POINT('Ctrl Pts',(-0.848829827264217,6.96221458378311,
4.76508608885947));
#22169=CARTESIAN_POINT('Ctrl Pts',(-0.661862630460365,6.98246825089994,
4.75655381629967));
#22170=CARTESIAN_POINT('Ctrl Pts',(-0.474414399316689,6.99518102269134,
4.74802154373986));
#22171=CARTESIAN_POINT('Ctrl Pts',(-0.45021380147482,6.99682231146585,4.74691998041415));
#22172=CARTESIAN_POINT('Ctrl Pts',(-0.426005191403975,6.998337977832,4.74581841708844));
#22173=CARTESIAN_POINT('Ctrl Pts',(-0.401789895976411,6.99972795485591,
4.74471685376273));
#22174=CARTESIAN_POINT('Ctrl Pts',(-0.214225940260526,7.01049427359601,
4.7361844955489));
#22175=CARTESIAN_POINT('Ctrl Pts',(-0.026197395778026,7.01371915439505,
4.72765213733507));
#22176=CARTESIAN_POINT('Ctrl Pts',(0.161678462626507,7.0093856105384,4.71911977912124));
#22177=CARTESIAN_POINT('Ctrl Pts',(0.349519140576629,7.00505287815397,4.71058901862328));
#22178=CARTESIAN_POINT('Ctrl Pts',(0.537206883732021,6.9931645526712,4.70205825812531));
#22179=CARTESIAN_POINT('Ctrl Pts',(0.724125135371328,6.97375575646462,4.69352749762734));
#22180=CARTESIAN_POINT('Ctrl Pts',(0.91909670696476,6.95351073776824,4.68462919172844));
#22181=CARTESIAN_POINT('Ctrl Pts',(1.11323065855079,6.92508287194462,4.67573088582953));
#22182=CARTESIAN_POINT('Ctrl Pts',(1.30583306940464,6.88857217116503,4.66683257993062));
#22183=CARTESIAN_POINT('Ctrl Pts',(1.49047432091466,6.85357062858015,4.65830208267355));
#22184=CARTESIAN_POINT('Ctrl Pts',(1.67370777652848,6.81114108016015,4.64977158541649));
#22185=CARTESIAN_POINT('Ctrl Pts',(1.8549318983874,6.76142397833806,4.64124108815942));
#22186=CARTESIAN_POINT('Ctrl Pts',(2.03615787481013,6.71170636773416,4.63271050360519));
#22187=CARTESIAN_POINT('Ctrl Pts',(2.21537418216918,6.65470113877529,4.62417991905096));
#22188=CARTESIAN_POINT('Ctrl Pts',(2.39199342126689,6.5905989132336,4.61564933449673));
#22189=CARTESIAN_POINT('Ctrl Pts',(2.56864760923149,6.52648400334247,4.60711706193691));
#22190=CARTESIAN_POINT('Ctrl Pts',(2.74270341524402,6.45526939735551,4.59858478937708));
#22191=CARTESIAN_POINT('Ctrl Pts',(2.91359160767148,6.37719456392906,4.59005251681726));
#22192=CARTESIAN_POINT('Ctrl Pts',(2.93565421341179,6.36711467342487,4.58895095349166));
#22193=CARTESIAN_POINT('Ctrl Pts',(2.95766404936562,6.35692050022327,4.58784939016606));
#22194=CARTESIAN_POINT('Ctrl Pts',(2.97961991686035,6.34661261725884,4.58674782684045));
#22195=CARTESIAN_POINT('Ctrl Pts',(3.14968306439527,6.26677104316607,4.57821546862661));
#22196=CARTESIAN_POINT('Ctrl Pts',(3.3165638783545,6.18007659508099,4.56968311041277));
#22197=CARTESIAN_POINT('Ctrl Pts',(3.4797114620282,6.08680825256798,4.56115075219893));
#22198=CARTESIAN_POINT('Ctrl Pts',(3.64282849570919,5.99355737489948,4.55261999170095));
#22199=CARTESIAN_POINT('Ctrl Pts',(3.80221342864592,5.89373521119594,4.54408923120296));
#22200=CARTESIAN_POINT('Ctrl Pts',(3.95734080749966,5.78766622187198,4.53555847070498));
#22201=CARTESIAN_POINT('Ctrl Pts',(4.11915180555327,5.67702728017215,4.52666016480608));
#22202=CARTESIAN_POINT('Ctrl Pts',(4.27632994760052,5.55959148334597,4.51776185890717));
#22203=CARTESIAN_POINT('Ctrl Pts',(4.42831264673592,5.43577719054587,4.50886355300827));
#22204=CARTESIAN_POINT('Ctrl Pts',(4.57401318938176,5.31708072212603,4.50033305575119));
#22205=CARTESIAN_POINT('Ctrl Pts',(4.71493890431663,5.19252266857053,4.4918025584941));
#22206=CARTESIAN_POINT('Ctrl Pts',(4.85062769841396,5.06251296234185,4.48327206123702));
#22207=CARTESIAN_POINT('Ctrl Pts',(4.98631788108777,4.93250192565387,4.47474147668276));
#22208=CARTESIAN_POINT('Ctrl Pts',(5.11677081713854,4.79703933883374,4.46621089212851));
#22209=CARTESIAN_POINT('Ctrl Pts',(5.2415607347134,4.656572519226,4.45768030757425));
#22210=CARTESIAN_POINT('Ctrl Pts',(5.36637534532973,4.51607790448007,4.44914803501441));
#22211=CARTESIAN_POINT('Ctrl Pts',(5.48552449687935,4.37057730861295,4.44061576245457));
#22212=CARTESIAN_POINT('Ctrl Pts',(5.59862165195997,4.22055235256063,4.43208348989472));
#22213=CARTESIAN_POINT('Ctrl Pts',(5.61322311685505,4.20118330541155,4.4309819265692));
#22214=CARTESIAN_POINT('Ctrl Pts',(5.62772376196302,4.18173888880038,4.42988036324368));
#22215=CARTESIAN_POINT('Ctrl Pts',(5.64212280602026,4.16222017729554,4.42877879991815));
#22216=CARTESIAN_POINT('Ctrl Pts',(5.75365320920836,4.01103446279999,4.42024644170434));
#22217=CARTESIAN_POINT('Ctrl Pts',(5.8591221730809,3.85533786342847,4.41171408349054));
#22218=CARTESIAN_POINT('Ctrl Pts',(5.95817809650529,3.69563801431155,4.40318172527673));
#22219=CARTESIAN_POINT('Ctrl Pts',(6.05721547133908,3.53596806958618,4.39465096477877));
#22220=CARTESIAN_POINT('Ctrl Pts',(6.14984204099429,3.37229663100463,4.38612020428082));
#22221=CARTESIAN_POINT('Ctrl Pts',(6.23575023411537,3.20515921293001,4.37758944378287));
#22222=CARTESIAN_POINT('Ctrl Pts',(6.32535975741612,3.03082072651491,4.36869113788395));
#22223=CARTESIAN_POINT('Ctrl Pts',(6.40765897968901,2.85271128620633,4.35979283198503));
#22224=CARTESIAN_POINT('Ctrl Pts',(6.48235238583884,2.67146665865579,4.35089452608612));
#22225=CARTESIAN_POINT('Ctrl Pts',(6.55395836382148,2.49771372009221,4.34236402882907));
#22226=CARTESIAN_POINT('Ctrl Pts',(6.61857452743737,2.32107986933111,4.33383353157203));
#22227=CARTESIAN_POINT('Ctrl Pts',(6.67598971967607,2.14214561252951,4.32530303431498));
#22228=CARTESIAN_POINT('Ctrl Pts',(6.7334054994753,1.96320952459746,4.31677244976077));
#22229=CARTESIAN_POINT('Ctrl Pts',(6.78362007023891,1.7819732759193,4.30824186520656));
#22230=CARTESIAN_POINT('Ctrl Pts',(6.82647201543804,1.59903295305049,4.29971128065235));
#22231=CARTESIAN_POINT('Ctrl Pts',(6.86933244004708,1.41605643051839,4.29117900809254));
#22232=CARTESIAN_POINT('Ctrl Pts',(6.90482726045359,1.23137545847014,4.28264673553274));
#22233=CARTESIAN_POINT('Ctrl Pts',(6.93284589518463,1.04559760717099,4.27411446297293));
#22234=CARTESIAN_POINT('Ctrl Pts',(6.93646325506608,1.02161266455678,4.27301289964725));
#22235=CARTESIAN_POINT('Ctrl Pts',(6.93995607042438,0.997609450460709,4.27191133632156));
#22236=CARTESIAN_POINT('Ctrl Pts',(6.94332416590407,0.973589281818827,4.27080977299588));
#22237=CARTESIAN_POINT('Ctrl Pts',(6.96941235934794,0.787536715951268,4.26227741478204));
#22238=CARTESIAN_POINT('Ctrl Pts',(6.98802247973373,0.60040361675269,4.2537450565682));
#22239=CARTESIAN_POINT('Ctrl Pts',(6.9990870539665,0.412803795402279,4.24521269835437));
#22240=CARTESIAN_POINT('Ctrl Pts',(7.01014955631654,0.225239102817181,4.23668193785639));
#22241=CARTESIAN_POINT('Ctrl Pts',(7.01366931419739,0.0372081678141407,
4.22815117735841));
#22242=CARTESIAN_POINT('Ctrl Pts',(7.00963084742555,-0.150671647366538,
4.21962041686043));
#22243=CARTESIAN_POINT('Ctrl Pts',(7.00541838445617,-0.346646211193886,
4.21072211096152));
#22244=CARTESIAN_POINT('Ctrl Pts',(6.99298196617915,-0.542455991884459,
4.20182380506262));
#22245=CARTESIAN_POINT('Ctrl Pts',(6.97236444962771,-0.73740120970049,4.19292549916372));
#22246=CARTESIAN_POINT('Ctrl Pts',(6.95259915155997,-0.924288428992888,
4.18439500190664));
#22247=CARTESIAN_POINT('Ctrl Pts',(6.92531551788594,-1.11038079629712,4.17586450464957));
#22248=CARTESIAN_POINT('Ctrl Pts',(6.89060427455715,-1.29506729321484,4.16733400739249));
#22249=CARTESIAN_POINT('Ctrl Pts',(6.85589267600955,-1.4797556801287,4.15880342283826));
#22250=CARTESIAN_POINT('Ctrl Pts',(6.81375337561684,-1.66303786779166,4.15027283828402));
#22251=CARTESIAN_POINT('Ctrl Pts',(6.76432825789992,-1.84431282104653,4.14174225372979));
#22252=CARTESIAN_POINT('Ctrl Pts',(6.71489336009411,-2.02562364442655,4.13320998116996));
#22253=CARTESIAN_POINT('Ctrl Pts',(6.65816984694882,-2.20492614515935,4.12467770861013));
#22254=CARTESIAN_POINT('Ctrl Pts',(6.594349773433,-2.38163339498844,4.1161454360503));
#22255=CARTESIAN_POINT('Ctrl Pts',(6.58611025085242,-2.40444727305077,4.11504387272472));
#22256=CARTESIAN_POINT('Ctrl Pts',(6.57775250845608,-2.42721791616829,4.11394230939915));
#22257=CARTESIAN_POINT('Ctrl Pts',(6.56927701910553,-2.44994408278067,4.11284074607358));
#22258=CARTESIAN_POINT('Ctrl Pts',(6.50362858156439,-2.62597372162438,4.10430838785975));
#22259=CARTESIAN_POINT('Ctrl Pts',(6.43088970711191,-2.79939283689084,4.09577602964591));
#22260=CARTESIAN_POINT('Ctrl Pts',(6.35129333024201,-2.96962953846491,4.08724367143208));
#22261=CARTESIAN_POINT('Ctrl Pts',(6.27171185809015,-3.13983436258256,4.0787129109341));
#22262=CARTESIAN_POINT('Ctrl Pts',(6.18527557564355,-3.30685768517691,4.07018215043612));
#22263=CARTESIAN_POINT('Ctrl Pts',(6.09226482886744,-3.47014925002438,4.06165138993814));
#22264=CARTESIAN_POINT('Ctrl Pts',(5.99524674039861,-3.64047618571409,4.05275308403924));
#22265=CARTESIAN_POINT('Ctrl Pts',(5.89107527475306,-3.80674235923989,4.04385477814033));
#22266=CARTESIAN_POINT('Ctrl Pts',(5.78012132077429,-3.96835281692927,4.03495647224143));
#22267=CARTESIAN_POINT('Ctrl Pts',(5.67375361316453,-4.12328315779367,4.02642597498436));
#22268=CARTESIAN_POINT('Ctrl Pts',(5.56115303293269,-4.27393466016512,4.01789547772729));
#22269=CARTESIAN_POINT('Ctrl Pts',(5.4426902991149,-4.41981321668921,4.00936498047022));
#22270=CARTESIAN_POINT('Ctrl Pts',(5.32422635300424,-4.56569326606702,4.00083439591599));
#22271=CARTESIAN_POINT('Ctrl Pts',(5.19990032882851,-4.70680003650974,3.99230381136175));
#22272=CARTESIAN_POINT('Ctrl Pts',(5.07012317901214,-4.84267255884019,3.98377322680751));
#22273=CARTESIAN_POINT('Ctrl Pts',(4.94032034929621,-4.97857196720361,3.97524095424769));
#22274=CARTESIAN_POINT('Ctrl Pts',(4.80506445163746,-5.10923483821557,3.96670868168786));
#22275=CARTESIAN_POINT('Ctrl Pts',(4.66480383944029,-5.23423649657169,3.95817640912803));
#22276=CARTESIAN_POINT('Ctrl Pts',(4.6466954227979,-5.25037489832999,3.95707484580245));
#22277=CARTESIAN_POINT('Ctrl Pts',(4.62850363449858,-5.26641899021547,3.95597328247687));
#22278=CARTESIAN_POINT('Ctrl Pts',(4.61022948153133,-5.28236790560061,3.95487171915129));
#22279=CARTESIAN_POINT('Ctrl Pts',(4.46868372056602,-5.4059031178103,3.94633936093747));
#22280=CARTESIAN_POINT('Ctrl Pts',(4.3221459019274,-5.5237666028468,3.93780700272365));
#22281=CARTESIAN_POINT('Ctrl Pts',(4.17109316649641,-5.63556637427925,3.92927464450982));
#22282=CARTESIAN_POINT('Ctrl Pts',(4.0200687162526,-5.74734521078819,3.92074388401185));
#22283=CARTESIAN_POINT('Ctrl Pts',(3.86453128223682,-5.85306241768181,3.91221312351388));
#22284=CARTESIAN_POINT('Ctrl Pts',(3.7049893961723,-5.95236760766259,3.90368236301591));
#22285=CARTESIAN_POINT('Ctrl Pts',(3.53857369311416,-6.05595133363967,3.894784057117));
#22286=CARTESIAN_POINT('Ctrl Pts',(3.36780111999562,-6.15255807762872,3.88588575121809));
#22287=CARTESIAN_POINT('Ctrl Pts',(3.19328111137326,-6.24184125929575,3.87698744531918));
#22288=CARTESIAN_POINT('Ctrl Pts',(3.02597483175454,-6.32743394906898,3.86845694806211));
#22289=CARTESIAN_POINT('Ctrl Pts',(2.85522497701625,-6.40629618934995,3.85992645080505));
#22290=CARTESIAN_POINT('Ctrl Pts',(2.68159281415216,-6.47816999943561,3.85139595354799));
#22291=CARTESIAN_POINT('Ctrl Pts',(2.50795887441703,-6.55004454504451,3.84286536899377));
#22292=CARTESIAN_POINT('Ctrl Pts',(2.33144285156694,-6.61493040351266,3.83433478443955));
#22293=CARTESIAN_POINT('Ctrl Pts',(2.15262561350387,-6.67261789184628,3.82580419988533));
#22294=CARTESIAN_POINT('Ctrl Pts',(1.97377299164063,-6.73031679520108,3.81727192732552));
#22295=CARTESIAN_POINT('Ctrl Pts',(1.79261853660373,-6.78081439051758,3.8087396547657));
#22296=CARTESIAN_POINT('Ctrl Pts',(1.6097587238965,-6.82395071885335,3.80020738220588));
#22297=CARTESIAN_POINT('Ctrl Pts',(1.58615051611865,-6.82951985614517,3.79910581888026));
#22298=CARTESIAN_POINT('Ctrl Pts',(1.56251390031482,-6.83496636322313,3.79800425555463));
#22299=CARTESIAN_POINT('Ctrl Pts',(1.53885017464052,-6.84028995748783,3.796902692229));
#22300=CARTESIAN_POINT('Ctrl Pts',(1.35555850231485,-6.88152482088127,3.78837033401517));
#22301=CARTESIAN_POINT('Ctrl Pts',(1.17057760880845,-6.91539519781985,3.77983797580134));
#22302=CARTESIAN_POINT('Ctrl Pts',(0.984513719362816,-6.94178358196843,
3.77130561758751));
#22303=CARTESIAN_POINT('Ctrl Pts',(0.798484671073654,-6.96816702479376,
3.76277485708954));
#22304=CARTESIAN_POINT('Ctrl Pts',(0.611373334374456,-6.98707122782371,
3.75424409659157));
#22305=CARTESIAN_POINT('Ctrl Pts',(0.423793730903746,-6.99843021227952,
3.7457133360936));
#22306=CARTESIAN_POINT('Ctrl Pts',(0.228132313322538,-7.01027859536479,
3.7368150301947));
#22307=CARTESIAN_POINT('Ctrl Pts',(0.0319617353463715,-7.01391714592579,
3.72791672429579));
#22308=CARTESIAN_POINT('Ctrl Pts',(-0.164017063899415,-7.00933127803572,
3.71901841839688));
#22309=CARTESIAN_POINT('Ctrl Pts',(-0.351895141861999,-7.00493496553512,
3.71048792113981));
#22310=CARTESIAN_POINT('Ctrl Pts',(-0.539596649862154,-6.99298047977504,
3.70195742388274));
#22311=CARTESIAN_POINT('Ctrl Pts',(-0.726505192478232,-6.9735082109224,
3.69342692662567));
#22312=CARTESIAN_POINT('Ctrl Pts',(-0.913415647829727,-6.9540357427996,
3.68489634207145));
#22313=CARTESIAN_POINT('Ctrl Pts',(-1.09953281758575,-6.92704537277552,
3.67636575751722));
#22314=CARTESIAN_POINT('Ctrl Pts',(-1.28424606709989,-6.89262929524274,
3.667835172963));
#22315=CARTESIAN_POINT('Ctrl Pts',(-1.46899586709867,-6.85820640756334,
3.65930290040317));
#22316=CARTESIAN_POINT('Ctrl Pts',(-1.65234089137648,-6.81635493464879,
3.65077062784334));
#22317=CARTESIAN_POINT('Ctrl Pts',(-1.83368045678355,-6.76721822796562,
3.64223835528352));
#22318=CARTESIAN_POINT('Ctrl Pts',(-1.85709239227112,-6.76087440881972,
3.64113679195791));
#22319=CARTESIAN_POINT('Ctrl Pts',(-1.88047091801555,-6.75440922668789,
3.64003522863231));
#22320=CARTESIAN_POINT('Ctrl Pts',(-1.90381475790692,-6.74782305118294,
3.63893366530671));
#22321=CARTESIAN_POINT('Ctrl Pts',(-2.08462869697902,-6.69680863615906,
3.63040130709288));
#22322=CARTESIAN_POINT('Ctrl Pts',(-2.26342145439311,-6.63851383971342,
3.62186894887905));
#22323=CARTESIAN_POINT('Ctrl Pts',(-2.43960398736489,-6.57312398691317,
3.61333659066523));
#22324=CARTESIAN_POINT('Ctrl Pts',(-2.61575352950101,-6.50774637860647,
3.60480583016726));
#22325=CARTESIAN_POINT('Ctrl Pts',(-2.78929353586576,-6.43527647171771,
3.59627506966929));
#22326=CARTESIAN_POINT('Ctrl Pts',(-2.95965264279651,-6.35594861499742,
3.58774430917133));
#22327=CARTESIAN_POINT('Ctrl Pts',(-3.13735162361963,-6.27320294002855,
3.57884600327242));
#22328=CARTESIAN_POINT('Ctrl Pts',(-3.31158920764694,-6.18299540693946,
3.56994769737351));
#22329=CARTESIAN_POINT('Ctrl Pts',(-3.48174207006675,-6.08564694342576,
3.5610493914746));
#22330=CARTESIAN_POINT('Ctrl Pts',(-3.64486171808113,-5.99232234766365,
3.55251889421753));
#22331=CARTESIAN_POINT('Ctrl Pts',(-3.80422725291711,-5.8924354509167,3.54398839696047));
#22332=CARTESIAN_POINT('Ctrl Pts',(-3.95931587135017,-5.7863152690961,3.5354578997034));
#22333=CARTESIAN_POINT('Ctrl Pts',(-4.11440607688823,-5.68019400129077,
3.52692731514918));
#22334=CARTESIAN_POINT('Ctrl Pts',(-4.26521902787035,-5.56783949640536,
3.51839673059496));
#22335=CARTESIAN_POINT('Ctrl Pts',(-4.41126165360132,-5.44962358204368,
3.50986614604074));
#22336=CARTESIAN_POINT('Ctrl Pts',(-4.55733317779396,-5.33138427548364,
3.50133387348092));
#22337=CARTESIAN_POINT('Ctrl Pts',(-4.69863225422205,-5.20728143622081,
3.49280160092109));
#22338=CARTESIAN_POINT('Ctrl Pts',(-4.83469892174064,-5.07772713904754,
3.48426932836127));
#22339=CARTESIAN_POINT('Ctrl Pts',(-4.85226587705371,-5.06100096657222,
3.48316776503565));
#22340=CARTESIAN_POINT('Ctrl Pts',(-4.86974566578051,-5.04418398015781,
3.48206620171004));
#22341=CARTESIAN_POINT('Ctrl Pts',(-4.88713734174978,-5.02727711245113,
3.48096463838442));
#22342=CARTESIAN_POINT('Ctrl Pts',(-5.0218468407324,-4.89632275922165,3.4724323356924));
#22343=CARTESIAN_POINT('Ctrl Pts',(-5.15131248351839,-4.75992877233467,
3.46390003300037));
#22344=CARTESIAN_POINT('Ctrl Pts',(-5.27510453917352,-4.61853858523353,
3.45536773030835));
#22345=CARTESIAN_POINT('Ctrl Pts',(-5.39887311251369,-4.47717521866533,
3.44683704612261));
#22346=CARTESIAN_POINT('Ctrl Pts',(-5.51697004508846,-4.33081777338997,
3.43830636193686));
#22347=CARTESIAN_POINT('Ctrl Pts',(-5.62900449685822,-4.17994437006642,
3.42977567775112));
#22348=CARTESIAN_POINT('Ctrl Pts',(-5.74103758216335,-4.02907280691941,
3.42124509761264));
#22349=CARTESIAN_POINT('Ctrl Pts',(-5.84700814907071,-3.87368563925147,
3.41271451747416));
#22350=CARTESIAN_POINT('Ctrl Pts',(-5.94656695937722,-3.71429239023305,
3.40418393733567));
#22351=CARTESIAN_POINT('Ctrl Pts',(-6.04611930050683,-3.55490949834046,
3.39565391150105));
#22352=CARTESIAN_POINT('Ctrl Pts',(-6.13926055637389,-3.39152130535483,
3.38712388566642));
#22353=CARTESIAN_POINT('Ctrl Pts',(-6.22568574525753,-3.22466487619989,
3.37859385983179));
#22354=CARTESIAN_POINT('Ctrl Pts',(-6.31212407181111,-3.05778308285747,
3.37006253733046));
#22355=CARTESIAN_POINT('Ctrl Pts',(-6.39184415037769,-2.88743227152021,
3.36153121482914));
#22356=CARTESIAN_POINT('Ctrl Pts',(-6.46458732400406,-2.71417340876113,
3.35299989232781));
#22357=CARTESIAN_POINT('Ctrl Pts',(-6.50237430244478,-2.62417281371743,
3.34856823388679));
#22358=CARTESIAN_POINT('Ctrl Pts',(-6.53827943706638,-2.53338788513101,
3.34413657544576));
#22359=CARTESIAN_POINT('Ctrl Pts',(-6.5722715952584,-2.44189939200197,3.33970491700474));
#22360=CARTESIAN_POINT('Origin',(0.,0.,0.));
#22361=CARTESIAN_POINT('',(-6.57174751820833,-2.4417044432219,1.33970341751611));
#22362=CARTESIAN_POINT('',(-6.57227159525839,-2.441899392002,1.88676850238605));
#22363=CARTESIAN_POINT('',(-6.57227159525839,-2.441899392002,0.));
#22364=CARTESIAN_POINT('',(-7.01126267432566,-8.75058266332513E-5,3.77353435527672));
#22365=CARTESIAN_POINT('Ctrl Pts',(-6.5722715952584,-2.44189939200199,1.88676850238605));
#22366=CARTESIAN_POINT('Ctrl Pts',(-6.56405595980073,-2.46401143631154,
1.88783976058185));
#22367=CARTESIAN_POINT('Ctrl Pts',(-6.55572891713045,-2.48608151822896,
1.88891101877765));
#22368=CARTESIAN_POINT('Ctrl Pts',(-6.54729091522851,-2.50810849722778,
1.88998227697344));
#22369=CARTESIAN_POINT('Ctrl Pts',(-6.48008391030787,-2.68354899880218,
1.89851463518728));
#22370=CARTESIAN_POINT('Ctrl Pts',(-6.40580989920254,-2.8563161967038,1.90704699340112));
#22371=CARTESIAN_POINT('Ctrl Pts',(-6.3247068791517,-3.02584028912816,1.91557935161496));
#22372=CARTESIAN_POINT('Ctrl Pts',(-6.24361904594361,-3.19533263753446,
1.92411011211292));
#22373=CARTESIAN_POINT('Ctrl Pts',(-6.15570488771711,-3.36158281647229,
1.93264087261089));
#22374=CARTESIAN_POINT('Ctrl Pts',(-6.06124961945423,-3.5240430776547,1.94117163310885));
#22375=CARTESIAN_POINT('Ctrl Pts',(-5.96272477269912,-3.69350289319662,
1.95006993900776));
#22376=CARTESIAN_POINT('Ctrl Pts',(-5.85708284365987,-3.85883866531672,
1.95896824490667));
#22377=CARTESIAN_POINT('Ctrl Pts',(-5.74469998304298,-4.01945875303206,
1.96786655080557));
#22378=CARTESIAN_POINT('Ctrl Pts',(-5.63696243219612,-4.17343966055005,
1.97639704806265));
#22379=CARTESIAN_POINT('Ctrl Pts',(-5.52303020146616,-4.3230866205467,1.98492754531972));
#22380=CARTESIAN_POINT('Ctrl Pts',(-5.40327837738593,-4.46790883288521,
1.99345804257679));
#22381=CARTESIAN_POINT('Ctrl Pts',(-5.28352532782082,-4.61273252726739,
2.00198862713103));
#22382=CARTESIAN_POINT('Ctrl Pts',(-5.15795276337739,-4.75273114158654,
2.01051921168528));
#22383=CARTESIAN_POINT('Ctrl Pts',(-5.02697570850291,-4.8874473693966,2.01904979623952));
#22384=CARTESIAN_POINT('Ctrl Pts',(-4.89597273629508,-5.02219025443594,
2.02758206879937));
#22385=CARTESIAN_POINT('Ctrl Pts',(-4.7595633517329,-5.15164844659135,2.03611434135923));
#22386=CARTESIAN_POINT('Ctrl Pts',(-4.61819965689422,-5.27540126355921,
2.04464661391908));
#22387=CARTESIAN_POINT('Ctrl Pts',(-4.59994882621505,-5.29137843302361,
2.04574817724463));
#22388=CARTESIAN_POINT('Ctrl Pts',(-4.5816154635611,-5.30726055692826,2.04684974057018));
#22389=CARTESIAN_POINT('Ctrl Pts',(-4.5632005835676,-5.32304677761039,2.04795130389573));
#22390=CARTESIAN_POINT('Ctrl Pts',(-4.42056479593313,-5.44532180853984,
2.05648366210955));
#22391=CARTESIAN_POINT('Ctrl Pts',(-4.27298744763936,-5.56188106242753,
2.06501602032336));
#22392=CARTESIAN_POINT('Ctrl Pts',(-4.12094913720164,-5.6723367998645,2.07354837853718));
#22393=CARTESIAN_POINT('Ctrl Pts',(-3.96893929650412,-5.78277185405303,
2.08207913903513));
#22394=CARTESIAN_POINT('Ctrl Pts',(-3.81247040812485,-5.88710549284097,
2.09060989953307));
#22395=CARTESIAN_POINT('Ctrl Pts',(-3.6520540912579,-5.98499185271179,2.09914066003102));
#22396=CARTESIAN_POINT('Ctrl Pts',(-3.48472628279308,-6.08709561868571,
2.10803896592994));
#22397=CARTESIAN_POINT('Ctrl Pts',(-3.31310365217863,-6.1821840374061,2.11693727182885));
#22398=CARTESIAN_POINT('Ctrl Pts',(-3.13779868371105,-6.26991594704437,
2.12583557772777));
#22399=CARTESIAN_POINT('Ctrl Pts',(-2.96973989031241,-6.35402148612434,
2.13436607498484));
#22400=CARTESIAN_POINT('Ctrl Pts',(-2.79829734737156,-6.4313663004645,2.14289657224191));
#22401=CARTESIAN_POINT('Ctrl Pts',(-2.62403458775532,-6.5016973972005,2.15142706949898));
#22402=CARTESIAN_POINT('Ctrl Pts',(-2.44977004481376,-6.57202921367275,
2.15995765405326));
#22403=CARTESIAN_POINT('Ctrl Pts',(-2.27268551247757,-6.63534705760097,
2.16848823860754));
#22404=CARTESIAN_POINT('Ctrl Pts',(-2.09336369541439,-6.69144640576468,
2.17701882316181));
#22405=CARTESIAN_POINT('Ctrl Pts',(-1.91400639470832,-6.74755685469275,
2.1855510957216));
#22406=CARTESIAN_POINT('Ctrl Pts',(-1.73241121739424,-6.79644586458776,
2.19408336828139));
#22407=CARTESIAN_POINT('Ctrl Pts',(-1.54917603414106,-6.83795877274374,
2.20261564084119));
#22408=CARTESIAN_POINT('Ctrl Pts',(-1.52551936396098,-6.84331831755945,
2.2037172041668));
#22409=CARTESIAN_POINT('Ctrl Pts',(-1.5018353744393,-6.84855498504257,2.20481876749241));
#22410=CARTESIAN_POINT('Ctrl Pts',(-1.47812536618678,-6.85366850411772,
2.20592033081802));
#22411=CARTESIAN_POINT('Ctrl Pts',(-1.29447520376752,-6.89327619208995,
2.21445268903187));
#22412=CARTESIAN_POINT('Ctrl Pts',(-1.1092011998166,-6.92550470208483,2.22298504724571));
#22413=CARTESIAN_POINT('Ctrl Pts',(-0.922910597859375,-6.95024190880137,
2.23151740545955));
#22414=CARTESIAN_POINT('Ctrl Pts',(-0.736654879511946,-6.97497448338371,
2.24004816595751));
#22415=CARTESIAN_POINT('Ctrl Pts',(-0.549383246244183,-6.99221851384896,
2.24857892645547));
#22416=CARTESIAN_POINT('Ctrl Pts',(-0.361710280690892,-7.00191346956977,
2.25710968695342));
#22417=CARTESIAN_POINT('Ctrl Pts',(-0.165951478547931,-7.01202612971311,
2.26600799285233));
#22418=CARTESIAN_POINT('Ctrl Pts',(0.030243653652506,-7.01392476462728,
2.27490629875124));
#22419=CARTESIAN_POINT('Ctrl Pts',(0.226174074993435,-7.00760100535846,
2.28380460465015));
#22420=CARTESIAN_POINT('Ctrl Pts',(0.414005774736144,-7.00153863666605,
2.2923351019072));
#22421=CARTESIAN_POINT('Ctrl Pts',(0.601593880499382,-6.98791995789897,
2.30086559916426));
#22422=CARTESIAN_POINT('Ctrl Pts',(0.788322379309909,-6.96679082424463,
2.30939609642131));
#22423=CARTESIAN_POINT('Ctrl Pts',(0.975052789013054,-6.94566147436457,
2.31792668097551));
#22424=CARTESIAN_POINT('Ctrl Pts',(1.16092327051103,-6.91702155363308,2.3264572655297));
#22425=CARTESIAN_POINT('Ctrl Pts',(1.34532403081394,-6.88096866833548,2.3349878500839));
#22426=CARTESIAN_POINT('Ctrl Pts',(1.52976127976858,-6.84490864900452,2.34352012264377));
#22427=CARTESIAN_POINT('Ctrl Pts',(1.71272792656109,-6.80143279508103,2.35205239520363));
#22428=CARTESIAN_POINT('Ctrl Pts',(1.89362458300221,-6.75068977965583,2.3605846677635));
#22429=CARTESIAN_POINT('Ctrl Pts',(1.91697933650567,-6.74413857721466,2.3616862310891));
#22430=CARTESIAN_POINT('Ctrl Pts',(1.94029960525135,-6.73746631286051,2.36278779441471));
#22431=CARTESIAN_POINT('Ctrl Pts',(1.96358411645753,-6.73067336750906,2.36388935774031));
#22432=CARTESIAN_POINT('Ctrl Pts',(2.14393851445478,-6.67805737919648,2.37242171595415));
#22433=CARTESIAN_POINT('Ctrl Pts',(2.32220724296558,-6.61817922097852,2.38095407416798));
#22434=CARTESIAN_POINT('Ctrl Pts',(2.49780292595847,-6.55122943466136,2.38948643238182));
#22435=CARTESIAN_POINT('Ctrl Pts',(2.67336572800529,-6.48429218494119,2.39801719287978));
#22436=CARTESIAN_POINT('Ctrl Pts',(2.84625619763583,-6.41028605867833,2.40654795337774));
#22437=CARTESIAN_POINT('Ctrl Pts',(3.01590507201999,-6.32945046264398,2.4150787138757));
#22438=CARTESIAN_POINT('Ctrl Pts',(3.1928632201284,-6.24513208783953,2.42397701977461));
#22439=CARTESIAN_POINT('Ctrl Pts',(3.36629393079521,-6.15338284636422,2.43287532567352));
#22440=CARTESIAN_POINT('Ctrl Pts',(3.53557674992503,-6.05452918135585,2.44177363157243));
#22441=CARTESIAN_POINT('Ctrl Pts',(3.69786231761193,-5.95976160112368,2.4503041288295));
#22442=CARTESIAN_POINT('Ctrl Pts',(3.85633572086378,-5.85846527198439,2.45883462608657));
#22443=CARTESIAN_POINT('Ctrl Pts',(4.01047709495085,-5.75097383348026,2.46736512334363));
#22444=CARTESIAN_POINT('Ctrl Pts',(4.16462004644966,-5.64348129495831,2.47589570789788));
#22445=CARTESIAN_POINT('Ctrl Pts',(4.31443063106958,-5.52979369806212,2.48442629245213));
#22446=CARTESIAN_POINT('Ctrl Pts',(4.45941909512374,-5.41028722865485,2.49295687700637));
#22447=CARTESIAN_POINT('Ctrl Pts',(4.60443624904525,-5.29075711167826,2.50148914956621));
#22448=CARTESIAN_POINT('Ctrl Pts',(4.74462914114087,-5.16540601787146,2.51002142212606));
#22449=CARTESIAN_POINT('Ctrl Pts',(4.87954148291101,-5.03465008506556,2.5185536946859));
#22450=CARTESIAN_POINT('Ctrl Pts',(4.89695940841886,-5.0177687748204,2.51965525801147));
#22451=CARTESIAN_POINT('Ctrl Pts',(4.91428936536944,-5.00079742725952,2.52075682133704));
#22452=CARTESIAN_POINT('Ctrl Pts',(4.93153041590004,-4.98373698338434,2.5218583846626));
#22453=CARTESIAN_POINT('Ctrl Pts',(5.06507409486585,-4.85159222597303,2.53039074287643));
#22454=CARTESIAN_POINT('Ctrl Pts',(5.19332581262223,-4.71405448464751,2.53892310109026));
#22455=CARTESIAN_POINT('Ctrl Pts',(5.31585977961177,-4.57157099540256,2.54745545930409));
#22456=CARTESIAN_POINT('Ctrl Pts',(5.43837080165949,-4.42911418672179,2.55598621980206));
#22457=CARTESIAN_POINT('Ctrl Pts',(5.55516601017619,-4.28171371019237,2.56451698030003));
#22458=CARTESIAN_POINT('Ctrl Pts',(5.66585881085924,-4.12985114718542,2.573047740798));
#22459=CARTESIAN_POINT('Ctrl Pts',(5.78132077952185,-3.97144562864463,2.5819460466969));
#22460=CARTESIAN_POINT('Ctrl Pts',(5.89014262468045,-3.80818528217321,2.59084435259581));
#22461=CARTESIAN_POINT('Ctrl Pts',(5.9919341789416,-3.64065260052803,2.59974265849472));
#22462=CARTESIAN_POINT('Ctrl Pts',(6.08951821170951,-3.48004482894987,2.60827315575179));
#22463=CARTESIAN_POINT('Ctrl Pts',(6.18064128844554,-3.3155110916146,2.61680365300887));
#22464=CARTESIAN_POINT('Ctrl Pts',(6.26500512287398,-3.14759231363638,2.62533415026594));
#22465=CARTESIAN_POINT('Ctrl Pts',(6.34936982064302,-2.97967181725478,2.63386473482019));
#22466=CARTESIAN_POINT('Ctrl Pts',(6.42697500341061,-2.80836648587293,2.64239531937444));
#22467=CARTESIAN_POINT('Ctrl Pts',(6.49756912197041,-2.63424032079776,2.65092590392869));
#22468=CARTESIAN_POINT('Ctrl Pts',(6.56817720947545,-2.46007970017709,2.65945817648856));
#22469=CARTESIAN_POINT('Ctrl Pts',(6.6317713478514,-2.28309741497011,2.66799044904842));
#22470=CARTESIAN_POINT('Ctrl Pts',(6.68814843916256,-2.10387666421478,2.67652272160829));
#22471=CARTESIAN_POINT('Ctrl Pts',(6.69542703179458,-2.08073827935638,2.67762428493382));
#22472=CARTESIAN_POINT('Ctrl Pts',(6.70258539665775,-2.05756260550653,2.67872584825936));
#22473=CARTESIAN_POINT('Ctrl Pts',(6.70962315709093,-2.03435091671253,2.67982741158489));
#22474=CARTESIAN_POINT('Ctrl Pts',(6.76413540495461,-1.85456057788433,2.68835976979873));
#22475=CARTESIAN_POINT('Ctrl Pts',(6.81142621627836,-1.6725476317491,2.69689212801257));
#22476=CARTESIAN_POINT('Ctrl Pts',(6.85133412022972,-1.48890810175647,2.70542448622642));
#22477=CARTESIAN_POINT('Ctrl Pts',(6.89123455127736,-1.30530295895008,2.71395524672439));
#22478=CARTESIAN_POINT('Ctrl Pts',(6.92375476891662,-1.12007213900288,2.72248600722237));
#22479=CARTESIAN_POINT('Ctrl Pts',(6.94878412279961,-0.933823204481489,
2.73101676772034));
#22480=CARTESIAN_POINT('Ctrl Pts',(6.97489185930863,-0.739549787344818,
2.73991507361924));
#22481=CARTESIAN_POINT('Ctrl Pts',(6.99284888010694,-0.544168928206322,
2.74881337951815));
#22482=CARTESIAN_POINT('Ctrl Pts',(7.00258944202674,-0.348378628672426,
2.75771168541705));
#22483=CARTESIAN_POINT('Ctrl Pts',(7.01192738092019,-0.160681258845915,
2.76624218267413));
#22484=CARTESIAN_POINT('Ctrl Pts',(7.01371443746118,0.0273920573483055,
2.7747726799312));
#22485=CARTESIAN_POINT('Ctrl Pts',(7.00794587276197,0.215223620772818,2.78330317718828));
#22486=CARTESIAN_POINT('Ctrl Pts',(7.0021772490299,0.40305710637946,2.79183376174255));
#22487=CARTESIAN_POINT('Ctrl Pts',(6.98885286217811,0.590648528537988,2.80036434629683));
#22488=CARTESIAN_POINT('Ctrl Pts',(6.96802005994193,0.777382149748008,2.8088949308511));
#22489=CARTESIAN_POINT('Ctrl Pts',(6.94718313537557,0.964152721226848,2.81742720341094));
#22490=CARTESIAN_POINT('Ctrl Pts',(6.91883486290099,1.15006484875056,2.82595947597079));
#22491=CARTESIAN_POINT('Ctrl Pts',(6.88307433754139,1.3345089832516,2.83449174853063));
#22492=CARTESIAN_POINT('Ctrl Pts',(6.87845745699039,1.35832173568631,2.83559331185615));
#22493=CARTESIAN_POINT('Ctrl Pts',(6.8737170973787,1.3821100318977,2.83669487518166));
#22494=CARTESIAN_POINT('Ctrl Pts',(6.86885353412558,1.405872572188,2.83779643850718));
#22495=CARTESIAN_POINT('Ctrl Pts',(6.83118192423267,1.58992963103396,2.846328796721));
#22496=CARTESIAN_POINT('Ctrl Pts',(6.78610175245774,1.77250266165203,2.85486115493483));
#22497=CARTESIAN_POINT('Ctrl Pts',(6.73375482552113,1.95299065852117,2.86339351314865));
#22498=CARTESIAN_POINT('Ctrl Pts',(6.68141770074137,2.13344485834129,2.87192427364665));
#22499=CARTESIAN_POINT('Ctrl Pts',(6.62181662150668,2.31181450981782,2.88045503414464));
#22500=CARTESIAN_POINT('Ctrl Pts',(6.55514357855421,2.48751265866919,2.88898579464264));
#22501=CARTESIAN_POINT('Ctrl Pts',(6.48559794642201,2.67078071252176,2.89788410054154));
#22502=CARTESIAN_POINT('Ctrl Pts',(6.40835756792077,2.8511416247024,2.90678240644045));
#22503=CARTESIAN_POINT('Ctrl Pts',(6.32369698627195,3.02795029488846,2.91568071233935));
#22504=CARTESIAN_POINT('Ctrl Pts',(6.24253582281654,3.19745063497386,2.92421120959642));
#22505=CARTESIAN_POINT('Ctrl Pts',(6.15455568761851,3.36368619568767,2.93274170685348));
#22506=CARTESIAN_POINT('Ctrl Pts',(6.06004653255181,3.52611153904792,2.94127220411055));
#22507=CARTESIAN_POINT('Ctrl Pts',(5.96553641032296,3.68853854459256,2.94980278866471));
#22508=CARTESIAN_POINT('Ctrl Pts',(5.86449729139241,3.84715499202844,2.95833337321886));
#22509=CARTESIAN_POINT('Ctrl Pts',(5.75726399662617,4.00144196954698,2.96686395777301));
#22510=CARTESIAN_POINT('Ctrl Pts',(5.65000948286777,4.15575947689467,2.97539623033281));
#22511=CARTESIAN_POINT('Ctrl Pts',(5.53655852069095,4.30574555255997,2.98392850289261));
#22512=CARTESIAN_POINT('Ctrl Pts',(5.41728848895509,4.45091136621869,2.99246077545241));
#22513=CARTESIAN_POINT('Ctrl Pts',(5.40189007172301,4.46965307135633,2.9935623387781));
#22514=CARTESIAN_POINT('Ctrl Pts',(5.38639471651263,4.488314475724,2.99466390210378));
#22515=CARTESIAN_POINT('Ctrl Pts',(5.37080328437187,4.50689456755762,2.99576546542947));
#22516=CARTESIAN_POINT('Ctrl Pts',(5.25003702337753,4.65081003339936,3.0042978236433));
#22517=CARTESIAN_POINT('Ctrl Pts',(5.12346257375957,4.78989289395479,3.01283018185713));
#22518=CARTESIAN_POINT('Ctrl Pts',(4.99149080541615,4.92368216906271,3.02136254007096));
#22519=CARTESIAN_POINT('Ctrl Pts',(4.85954374927805,5.05744639163039,3.02989330056892));
#22520=CARTESIAN_POINT('Ctrl Pts',(4.72220160612443,5.18591878916185,3.03842406106688));
#22521=CARTESIAN_POINT('Ctrl Pts',(4.57991268526853,5.3086746328831,3.04695482156484));
#22522=CARTESIAN_POINT('Ctrl Pts',(4.43149328654036,5.43671937737818,3.05585312746375));
#22523=CARTESIAN_POINT('Ctrl Pts',(4.27769165846373,5.5585438162839,3.06475143336266));
#22524=CARTESIAN_POINT('Ctrl Pts',(4.11905639031389,5.67371139695299,3.07364973926157));
#22525=CARTESIAN_POINT('Ctrl Pts',(3.96697826047658,5.78411856233504,3.08218023651864));
#22526=CARTESIAN_POINT('Ctrl Pts',(3.8104583149186,5.8884079312939,3.09071073377571));
#22527=CARTESIAN_POINT('Ctrl Pts',(3.65001123822204,5.98623792739253,3.09924123103278));
#22528=CARTESIAN_POINT('Ctrl Pts',(3.48956251958513,6.0840689246376,3.10777181558697));
#22529=CARTESIAN_POINT('Ctrl Pts',(3.32518685243327,6.17544026040601,3.11630240014116));
#22530=CARTESIAN_POINT('Ctrl Pts',(3.15742574695669,6.26005504887577,3.12483298469535));
#22531=CARTESIAN_POINT('Ctrl Pts',(2.98963144543196,6.3446865806579,3.13336525725519));
#22532=CARTESIAN_POINT('Ctrl Pts',(2.81845064125773,6.42255875794218,3.14189752981504));
#22533=CARTESIAN_POINT('Ctrl Pts',(2.6444479451557,6.49342141154121,3.15042980237489));
#22534=CARTESIAN_POINT('Ctrl Pts',(2.62198323985695,6.50257016995387,3.15153136570051));
#22535=CARTESIAN_POINT('Ctrl Pts',(2.59947152634468,6.5116021575947,3.15263292902614));
#22536=CARTESIAN_POINT('Ctrl Pts',(2.5769140435464,6.52051689474641,3.15373449235176));
#22537=CARTESIAN_POINT('Ctrl Pts',(2.40219097573927,6.5895676056688,3.16226685056557));
#22538=CARTESIAN_POINT('Ctrl Pts',(2.22466146157776,6.65160311967304,3.17079920877938));
#22539=CARTESIAN_POINT('Ctrl Pts',(2.0449063016234,6.70641370481131,3.17933156699318));
#22540=CARTESIAN_POINT('Ctrl Pts',(1.86518480149153,6.76121402646358,3.18786232749117));
#22541=CARTESIAN_POINT('Ctrl Pts',(1.68323877982464,6.8087920299243,3.19639308798916));
#22542=CARTESIAN_POINT('Ctrl Pts',(1.49966469881372,6.84898768823773,3.20492384848714));
#22543=CARTESIAN_POINT('Ctrl Pts',(1.30818138049391,6.89091516510983,3.21382215438605));
#22544=CARTESIAN_POINT('Ctrl Pts',(1.11492694565757,6.9248099748863,3.22272046028496));
#22545=CARTESIAN_POINT('Ctrl Pts',(0.92059166891686,6.95054944170753,3.23161876618387));
#22546=CARTESIAN_POINT('Ctrl Pts',(0.734289178979928,6.97522497586103,3.24014926344093));
#22547=CARTESIAN_POINT('Ctrl Pts',(0.546993727132722,6.99240576608184,3.248679760698));
#22548=CARTESIAN_POINT('Ctrl Pts',(0.359320550293526,7.00203651123277,3.25721025795506));
#22549=CARTESIAN_POINT('Ctrl Pts',(0.171645452895992,7.01166735494018,3.26574084250919));
#22550=CARTESIAN_POINT('Ctrl Pts',(-0.0164070714756707,7.01374798673602,
3.27427142706331));
#22551=CARTESIAN_POINT('Ctrl Pts',(-0.204219476019748,7.00827517782473,
3.28280201161744));
#22552=CARTESIAN_POINT('Ctrl Pts',(-0.392069044302411,7.00280128597091,
3.2913342841773));
#22553=CARTESIAN_POINT('Ctrl Pts',(-0.579678092029639,6.98977097808267,
3.29986655673715));
#22554=CARTESIAN_POINT('Ctrl Pts',(-0.766431002904122,6.96923310560692,
3.30839882929701));
#22555=CARTESIAN_POINT('Ctrl Pts',(-0.790541831073335,6.96658155328623,
3.30950039262269));
#22556=CARTESIAN_POINT('Ctrl Pts',(-0.81463839579834,6.96380493402564,3.31060195594837));
#22557=CARTESIAN_POINT('Ctrl Pts',(-0.838719379193902,6.9609034158983,3.31170351927405));
#22558=CARTESIAN_POINT('Ctrl Pts',(-1.02524299674915,6.93842918182638,3.32023587748788));
#22559=CARTESIAN_POINT('Ctrl Pts',(-1.21089419386651,6.90844974878836,3.32876823570171));
#22560=CARTESIAN_POINT('Ctrl Pts',(-1.39506237180662,6.87105723606413,3.33730059391554));
#22561=CARTESIAN_POINT('Ctrl Pts',(-1.57919606356934,6.83367172522721,3.34583135441351));
#22562=CARTESIAN_POINT('Ctrl Pts',(-1.76184699060401,6.78887596575204,3.35436211491148));
#22563=CARTESIAN_POINT('Ctrl Pts',(-1.94241444908253,6.73681324295808,3.36289287540945));
#22564=CARTESIAN_POINT('Ctrl Pts',(-2.13076160538968,6.68250741249187,3.37179118130836));
#22565=CARTESIAN_POINT('Ctrl Pts',(-2.31684143976208,6.6202946328271,3.38068948720727));
#22566=CARTESIAN_POINT('Ctrl Pts',(-2.49998853805577,6.55039570347393,3.38958779310617));
#22567=CARTESIAN_POINT('Ctrl Pts',(-2.6755653093409,6.48338602411535,3.39811829036326));
#22568=CARTESIAN_POINT('Ctrl Pts',(-2.84844661213151,6.40931294546411,3.40664878762034));
#22569=CARTESIAN_POINT('Ctrl Pts',(-3.01806509828058,6.32842078444857,3.41517928487743));
#22570=CARTESIAN_POINT('Ctrl Pts',(-3.18768532022673,6.2475277956201,3.42370986943168));
#22571=CARTESIAN_POINT('Ctrl Pts',(-3.35404238402338,6.15981571961481,3.43224045398592));
#22572=CARTESIAN_POINT('Ctrl Pts',(-3.51659170468122,6.0655757636903,3.44077103854017));
#22573=CARTESIAN_POINT('Ctrl Pts',(-3.67917319009338,5.97131715985625,3.44930331109997));
#22574=CARTESIAN_POINT('Ctrl Pts',(-3.83794516327184,5.87052825051918,3.45783558365977));
#22575=CARTESIAN_POINT('Ctrl Pts',(-3.9923895349857,5.76354512114173,3.46636785621957));
#22576=CARTESIAN_POINT('Ctrl Pts',(-4.01232915301025,5.74973301059873,3.46746941954516));
#22577=CARTESIAN_POINT('Ctrl Pts',(-4.0321966773412,5.73581771243711,3.46857098287075));
#22578=CARTESIAN_POINT('Ctrl Pts',(-4.05199102910796,5.72180000196867,3.46967254619634));
#22579=CARTESIAN_POINT('Ctrl Pts',(-4.20531176515773,5.61322328715232,3.47820490441019));
#22580=CARTESIAN_POINT('Ctrl Pts',(-4.35429170696321,5.49846218600666,3.48673726262403));
#22581=CARTESIAN_POINT('Ctrl Pts',(-4.49843777963941,5.37788844298698,3.49526962083788));
#22582=CARTESIAN_POINT('Ctrl Pts',(-4.64255686042606,5.25733727785022,3.50380038133584));
#22583=CARTESIAN_POINT('Ctrl Pts',(-4.78184364384754,5.13097583920066,3.5123311418338));
#22584=CARTESIAN_POINT('Ctrl Pts',(-4.91583811907906,4.9992161535094,3.52086190233176));
#22585=CARTESIAN_POINT('Ctrl Pts',(-5.05560570834129,4.86177963906208,3.52976020823066));
#22586=CARTESIAN_POINT('Ctrl Pts',(-5.18961458465397,4.71846964016777,3.53865851412957));
#22587=CARTESIAN_POINT('Ctrl Pts',(-5.31738474194418,4.56979715836921,3.54755682002847));
#22588=CARTESIAN_POINT('Ctrl Pts',(-5.43987356045443,4.42727000628055,3.55608731728555));
#22589=CARTESIAN_POINT('Ctrl Pts',(-5.55662882843779,4.27981501913708,3.56461781454262));
#22590=CARTESIAN_POINT('Ctrl Pts',(-5.66726797327666,4.12791718443728,3.57314831179969));
#22591=CARTESIAN_POINT('Ctrl Pts',(-5.77790825034554,3.97601779528509,3.58167889635394));
#22592=CARTESIAN_POINT('Ctrl Pts',(-5.88243210166907,3.81967571695454,3.59020948090819));
#22593=CARTESIAN_POINT('Ctrl Pts',(-5.98049929865436,3.65940633181049,3.59874006546243));
#22594=CARTESIAN_POINT('Ctrl Pts',(-6.07858590087249,3.4991052330575,3.6072723380223));
#22595=CARTESIAN_POINT('Ctrl Pts',(-6.17021313812817,3.33487553688238,3.61580461058217));
#22596=CARTESIAN_POINT('Ctrl Pts',(-6.25508545008453,3.16725947384184,3.62433688314204));
#22597=CARTESIAN_POINT('Ctrl Pts',(-6.26604293246077,3.14561931800767,3.62543844646756));
#22598=CARTESIAN_POINT('Ctrl Pts',(-6.27688788527885,3.12392275043866,3.62654000979309));
#22599=CARTESIAN_POINT('Ctrl Pts',(-6.28761972898703,3.1021709666221,3.62764157311862));
#22600=CARTESIAN_POINT('Ctrl Pts',(-6.37051092536119,2.93416335927575,3.63614988766531));
#22601=CARTESIAN_POINT('Ctrl Pts',(-6.44667990653279,2.76280004359039,3.644658202212));
#22602=CARTESIAN_POINT('Ctrl Pts',(-6.51587084808528,2.58863934405171,3.65316651675868));
#22603=CARTESIAN_POINT('Ctrl Pts',(-6.58504816965121,2.41451292741672,3.66167315647443));
#22604=CARTESIAN_POINT('Ctrl Pts',(-6.64725007839304,2.2375905132263,3.67017979619017));
#22605=CARTESIAN_POINT('Ctrl Pts',(-6.70226898252104,2.05845015689872,3.67868643590592));
#22606=CARTESIAN_POINT('Ctrl Pts',(-6.75728864378276,1.87930733536022,3.68719319268441));
#22607=CARTESIAN_POINT('Ctrl Pts',(-6.80512500802915,1.69794680530732,3.69569994946289));
#22608=CARTESIAN_POINT('Ctrl Pts',(-6.84562017724716,1.51496235971942,3.70420670624138));
#22609=CARTESIAN_POINT('Ctrl Pts',(-6.88611314149592,1.33198787766744,3.71271299982543));
#22610=CARTESIAN_POINT('Ctrl Pts',(-6.91926564402742,1.14738995929416,3.72121929340949));
#22611=CARTESIAN_POINT('Ctrl Pts',(-6.94497071526182,0.961773531896027,
3.72972558699354));
#22612=CARTESIAN_POINT('Ctrl Pts',(-6.97068151815061,0.776115716197457,
3.73823377729029));
#22613=CARTESIAN_POINT('Ctrl Pts',(-6.98894152821702,0.589439244279225,
3.74674196758704));
#22614=CARTESIAN_POINT('Ctrl Pts',(-6.99969543066941,0.402356111381252,
3.75525015788378));
#22615=CARTESIAN_POINT('Ctrl Pts',(-7.00739885007534,0.26834152059714,3.76134489033384));
#22616=CARTESIAN_POINT('Ctrl Pts',(-7.01125167442655,0.1341184071921,3.7674396227839));
#22617=CARTESIAN_POINT('Ctrl Pts',(-7.01124999945394,-8.75047268976489E-5,
3.77353435523396));
#22618=CARTESIAN_POINT('Ctrl Pts',(-7.01174696422417,-8.75478460599835E-5,
3.77353435691035));
#22619=CARTESIAN_POINT('Ctrl Pts',(-7.01180261336239,-0.0887333921737332,
3.77755977128721));
#22620=CARTESIAN_POINT('Ctrl Pts',(-6.99636440224467,-0.919874595891691,
3.81530283634042));
#22621=CARTESIAN_POINT('Ctrl Pts',(-6.83009966285127,-1.7452908997936,3.85304590139378));
#22622=CARTESIAN_POINT('Ctrl Pts',(-6.57188903190969,-2.44175767753665,
3.88676355207028));
#22623=CARTESIAN_POINT('',(-7.01086833367197,0.000109686007034688,3.2264656355206));
#22624=CARTESIAN_POINT('Ctrl Pts',(-6.5722715952584,-2.44189939200197,3.33970491700474));
#22625=CARTESIAN_POINT('Ctrl Pts',(-6.61499340131524,-2.32691541134939,
3.33413514849053));
#22626=CARTESIAN_POINT('Ctrl Pts',(-6.6546932255011,-2.21082002405903,3.32856537997633));
#22627=CARTESIAN_POINT('Ctrl Pts',(-6.69131729331829,-2.0937763592704,3.32299561146213));
#22628=CARTESIAN_POINT('Ctrl Pts',(-6.74759831376839,-1.91391275361073,
3.31443642417538));
#22629=CARTESIAN_POINT('Ctrl Pts',(-6.79663212228337,-1.73174958693402,
3.30587723688862));
#22630=CARTESIAN_POINT('Ctrl Pts',(-6.83825110391958,-1.54788513858188,
3.29731804960187));
#22631=CARTESIAN_POINT('Ctrl Pts',(-6.87986114213862,-1.36406020048205,
3.28876070158123));
#22632=CARTESIAN_POINT('Ctrl Pts',(-6.91405946739486,-1.17853500489088,
3.28020335356059));
#22633=CARTESIAN_POINT('Ctrl Pts',(-6.94072919079019,-0.991919786380446,
3.27164600553994));
#22634=CARTESIAN_POINT('Ctrl Pts',(-6.96739714357071,-0.805316957337377,
3.26308922564544));
#22635=CARTESIAN_POINT('Ctrl Pts',(-6.98653744714038,-0.617624548411278,
3.25453244575094));
#22636=CARTESIAN_POINT('Ctrl Pts',(-6.99808475054815,-0.429460576357655,
3.24597566585644));
#22637=CARTESIAN_POINT('Ctrl Pts',(-7.0068609551157,-0.286451819016622,
3.23947232493417));
#22638=CARTESIAN_POINT('Ctrl Pts',(-7.01125223737829,-0.143170865468828,
3.2329689840119));
#22639=CARTESIAN_POINT('Ctrl Pts',(-7.01124999914453,0.00010952522091514,
3.22646564308963));
#22640=CARTESIAN_POINT('Ctrl Pts',(-7.01077666039611,0.000109724626693396,
3.22646563370257));
#22641=CARTESIAN_POINT('Ctrl Pts',(-7.01102961718175,0.451283813389737,
3.20598595064833));
#22642=CARTESIAN_POINT('Ctrl Pts',(-6.85785257182463,2.06232469578677,3.13284992528664));
#22643=CARTESIAN_POINT('Ctrl Pts',(-5.63772386156061,4.64629944776454,3.00705755761756));
#22644=CARTESIAN_POINT('Ctrl Pts',(-2.74525602695119,6.77019927653496,2.84908853069525));
#22645=CARTESIAN_POINT('Ctrl Pts',(0.809572652366525,7.26062125565349,2.69111950377297));
#22646=CARTESIAN_POINT('Ctrl Pts',(4.16907192684548,5.9992389655935,2.53315047685068));
#22647=CARTESIAN_POINT('Ctrl Pts',(6.52267959194278,3.29039204933995,2.37518144992839));
#22648=CARTESIAN_POINT('Ctrl Pts',(7.30252964686993,-0.212343245930207,
2.2172124230061));
#22649=CARTESIAN_POINT('Ctrl Pts',(6.32046399778932,-3.66384548666503,2.05924339608381));
#22650=CARTESIAN_POINT('Ctrl Pts',(3.81343024685451,-6.23135447955594,1.90127436916152));
#22651=CARTESIAN_POINT('Ctrl Pts',(0.386312228825965,-7.29539524353313,
1.74330534223923));
#22652=CARTESIAN_POINT('Ctrl Pts',(-3.13401315918718,-6.59924165458034,
1.58533631531694));
#22653=CARTESIAN_POINT('Ctrl Pts',(-5.48811015356693,-4.65034471123624,
1.45080234040949));
#22654=CARTESIAN_POINT('Ctrl Pts',(-6.34735191580087,-3.04510780294658,
1.36892470780946));
#22655=CARTESIAN_POINT('Ctrl Pts',(-6.57174751820247,-2.44170444323764,
1.33970341751688));
#22656=CARTESIAN_POINT('Origin',(0.,0.,0.));
#22657=CARTESIAN_POINT('',(-6.5722715952584,-2.44189939200198,-0.660303821598748));
#22658=CARTESIAN_POINT('',(-6.57227163891168,-2.44189927451098,-0.113051811211838));
#22659=CARTESIAN_POINT('',(-6.57227159525839,-2.441899392002,0.));
#22660=CARTESIAN_POINT('',(-7.01124999779487,0.000175845004380833,1.77353435691035));
#22661=CARTESIAN_POINT('Ctrl Pts',(-6.57227163891168,-2.44189927451098,
-0.113051811211839));
#22662=CARTESIAN_POINT('Ctrl Pts',(-6.51379048013646,-2.59929891226057,
-0.105346661399166));
#22663=CARTESIAN_POINT('Ctrl Pts',(-6.44965919248067,-2.75458629304454,
-0.0976675531015183));
#22664=CARTESIAN_POINT('Ctrl Pts',(-6.30177438124679,-3.07909809577218,
-0.0814412978830712));
#22665=CARTESIAN_POINT('Ctrl Pts',(-6.21665974009033,-3.24751422428018,
-0.0729127710991782));
#22666=CARTESIAN_POINT('Ctrl Pts',(-6.01680152855583,-3.60624728191609,
-0.0544264990385142));
#22667=CARTESIAN_POINT('Ctrl Pts',(-5.89959433231979,-3.79495816685282,
-0.0444946513980189));
#22668=CARTESIAN_POINT('Ctrl Pts',(-5.67134537880492,-4.12625400191001,
-0.0264653376106269));
#22669=CARTESIAN_POINT('Ctrl Pts',(-5.5633724974678,-4.27071604468818,-0.0183795479634319));
#22670=CARTESIAN_POINT('Ctrl Pts',(-5.38196222462781,-4.49486255913974,
-0.00532741689756344));
#22671=CARTESIAN_POINT('Ctrl Pts',(-5.31203897582476,-4.57728609272316,
-0.000405389684517453));
#22672=CARTESIAN_POINT('Ctrl Pts',(-5.04791538435022,-4.87442074824541,
0.0177810171590431));
#22673=CARTESIAN_POINT('Ctrl Pts',(-4.84237642232889,-5.07866300543721,
0.0311369266982347));
#22674=CARTESIAN_POINT('Ctrl Pts',(-4.46558505942067,-5.4093486242146,0.0541445575416953));
#22675=CARTESIAN_POINT('Ctrl Pts',(-4.30011501631266,-5.54179713015967,
0.0638205079324956));
#22676=CARTESIAN_POINT('Ctrl Pts',(-3.95709046738012,-5.79174002262208,
0.0830855683209048));
#22677=CARTESIAN_POINT('Ctrl Pts',(-3.77967410863643,-5.90905094017359,
0.0926643195028018));
#22678=CARTESIAN_POINT('Ctrl Pts',(-3.36346120301389,-6.15783313652653,
0.114435063300481));
#22679=CARTESIAN_POINT('Ctrl Pts',(-3.12178243662828,-6.2838088051756,0.126583180726194));
#22680=CARTESIAN_POINT('Ctrl Pts',(-2.76799658910346,-6.4427612088298,0.144043701559189));
#22681=CARTESIAN_POINT('Ctrl Pts',(-2.6614484738719,-6.48750097104497,0.149264869801388));
#22682=CARTESIAN_POINT('Ctrl Pts',(-2.35034634210553,-6.6091787839831,0.164467345759501));
#22683=CARTESIAN_POINT('Ctrl Pts',(-2.14324232001506,-6.6792127271797,0.174516156026655));
#22684=CARTESIAN_POINT('Ctrl Pts',(-1.6426784502937,-6.82279909339829,0.198472689701524));
#22685=CARTESIAN_POINT('Ctrl Pts',(-1.34705857149823,-6.88726492567702,
0.212349851066077));
#22686=CARTESIAN_POINT('Ctrl Pts',(-0.861236024399551,-6.96072221549327,
0.234704280016186));
#22687=CARTESIAN_POINT('Ctrl Pts',(-0.673203222455418,-6.98141677634236,
0.243252959396741));
#22688=CARTESIAN_POINT('Ctrl Pts',(-0.261265577008079,-7.00995488939356,
0.261840069161537));
#22689=CARTESIAN_POINT('Ctrl Pts',(-0.0373558298317422,-7.01472254986739,
0.271851739318829));
#22690=CARTESIAN_POINT('Ctrl Pts',(0.367065798118773,-7.00396695262904,
0.289983082135156));
#22691=CARTESIAN_POINT('Ctrl Pts',(0.547477948887577,-6.99217825859279,
0.298090263095312));
#22692=CARTESIAN_POINT('Ctrl Pts',(0.836614686634072,-6.96202538606241,
0.311253950360317));
#22693=CARTESIAN_POINT('Ctrl Pts',(0.945713287992123,-6.94804628486296,
0.316265662383899));
#22694=CARTESIAN_POINT('Ctrl Pts',(1.12922444502119,-6.92013015898074,0.324760691432349));
#22695=CARTESIAN_POINT('Ctrl Pts',(1.203823279825,-6.90754360712728,0.328231581556242));
#22696=CARTESIAN_POINT('Ctrl Pts',(1.68318192553285,-6.81866343687492,0.35062969928556));
#22697=CARTESIAN_POINT('Ctrl Pts',(2.08076607353137,-6.70803228930215,0.369588048055639));
#22698=CARTESIAN_POINT('Ctrl Pts',(2.65884688568928,-6.49079760841058,0.397632534543466));
#22699=CARTESIAN_POINT('Ctrl Pts',(2.84808301716799,-6.4100191331999,0.406906207846296));
#22700=CARTESIAN_POINT('Ctrl Pts',(3.1655757366444,-6.25765287957744,0.422725912084332));
#22701=CARTESIAN_POINT('Ctrl Pts',(3.29563640355392,-6.19014298728567,0.429286249465989));
#22702=CARTESIAN_POINT('Ctrl Pts',(3.61664409924359,-6.01053259762188,0.445766322371894));
#22703=CARTESIAN_POINT('Ctrl Pts',(3.80457288852243,-5.89337247774327,0.455678894857876));
#22704=CARTESIAN_POINT('Ctrl Pts',(4.08340943689875,-5.70063433761663,0.471045311444189));
#22705=CARTESIAN_POINT('Ctrl Pts',(4.17847651131669,-5.63132290016994,0.476414920780977));
#22706=CARTESIAN_POINT('Ctrl Pts',(4.41122355758142,-5.4524919920581,0.489863841851319));
#22707=CARTESIAN_POINT('Ctrl Pts',(4.54661161064246,-5.34012028570029,0.497960924407617));
#22708=CARTESIAN_POINT('Ctrl Pts',(4.86843309564754,-5.05189013463151,0.517831691158166));
#22709=CARTESIAN_POINT('Ctrl Pts',(5.0497304775803,-4.87067346811471,0.529577494975458));
#22710=CARTESIAN_POINT('Ctrl Pts',(5.34566795837694,-4.54054057475343,0.549755745055887));
#22711=CARTESIAN_POINT('Ctrl Pts',(5.46499738837264,-4.39618922258884,0.558223296853779));
#22712=CARTESIAN_POINT('Ctrl Pts',(5.70953561679692,-4.07500749496314,0.57640095972916));
#22713=CARTESIAN_POINT('Ctrl Pts',(5.83261775805606,-3.89680046723166,0.586087800144649));
#22714=CARTESIAN_POINT('Ctrl Pts',(6.05218242189192,-3.5451325863076,0.604664271504848));
#22715=CARTESIAN_POINT('Ctrl Pts',(6.14993486925177,-3.37271053492856,0.613544313471033));
#22716=CARTESIAN_POINT('Ctrl Pts',(6.29096259082812,-3.09738414210479,0.627555224997623));
#22717=CARTESIAN_POINT('Ctrl Pts',(6.33930794442124,-2.99719415308173,0.632625771398413));
#22718=CARTESIAN_POINT('Ctrl Pts',(6.41744039454165,-2.82491767512174,0.641285071597625));
#22719=CARTESIAN_POINT('Ctrl Pts',(6.44844618251633,-2.75340567747632,0.644861937113561));
#22720=CARTESIAN_POINT('Ctrl Pts',(6.63094349624851,-2.31249147471794,0.66678915431235));
#22721=CARTESIAN_POINT('Ctrl Pts',(6.75184801516868,-1.93121408346769,0.685163578727264));
#22722=CARTESIAN_POINT('Ctrl Pts',(6.88379637084582,-1.34584247504007,0.712424849648115));
#22723=CARTESIAN_POINT('Ctrl Pts',(6.9195147439769,-1.14815585810827,0.721484840716629));
#22724=CARTESIAN_POINT('Ctrl Pts',(6.98320203995558,-0.68206527646686,0.742626730668839));
#22725=CARTESIAN_POINT('Ctrl Pts',(7.00426442178689,-0.413041210143523,
0.754658315309748));
#22726=CARTESIAN_POINT('Ctrl Pts',(7.01246849324306,-0.0122125706970769,
0.772675701945629));
#22727=CARTESIAN_POINT('Ctrl Pts',(7.01146764743179,0.119097956915563,0.778594530890423));
#22728=CARTESIAN_POINT('Ctrl Pts',(7.00129066234927,0.403986015878096,0.791548813195998));
#22729=CARTESIAN_POINT('Ctrl Pts',(6.99074586380984,0.557446758404484,0.798594980744528));
#22730=CARTESIAN_POINT('Ctrl Pts',(6.93347914745049,1.11970085952642,0.824560061699123));
#22731=CARTESIAN_POINT('Ctrl Pts',(6.85585374680587,1.52451456157718,0.843495300485487));
#22732=CARTESIAN_POINT('Ctrl Pts',(6.68689510407699,2.11785316136084,0.871511712397881));
#22733=CARTESIAN_POINT('Ctrl Pts',(6.62194192000074,2.31295377337637,0.880779799361355));
#22734=CARTESIAN_POINT('Ctrl Pts',(6.41650278036058,2.85002486111788,0.906611143946151));
#22735=CARTESIAN_POINT('Ctrl Pts',(6.25742302352168,3.18414795801925,0.923033593896662));
#22736=CARTESIAN_POINT('Ctrl Pts',(6.01338813118964,3.60706274953789,0.945171474088692));
#22737=CARTESIAN_POINT('Ctrl Pts',(5.95141153384286,3.708428012476,0.950595039809579));
#22738=CARTESIAN_POINT('Ctrl Pts',(5.78917250790118,3.95922666655062,0.964283414428022));
#22739=CARTESIAN_POINT('Ctrl Pts',(5.68567649769621,4.10646764394342,0.972566799975525));
#22740=CARTESIAN_POINT('Ctrl Pts',(5.42543518029854,4.44797801056314,0.992313632627998));
#22741=CARTESIAN_POINT('Ctrl Pts',(5.263754551808,4.63818350970906,1.00375063794982));
#22742=CARTESIAN_POINT('Ctrl Pts',(4.96365066537529,4.95528166754589,1.0236213095988));
#22743=CARTESIAN_POINT('Ctrl Pts',(4.82963075185957,5.08599180451281,1.03208537602857));
#22744=CARTESIAN_POINT('Ctrl Pts',(4.52989208273937,5.35578390390235,1.0502451856365));
#22745=CARTESIAN_POINT('Ctrl Pts',(4.3626420268057,5.49287709725563,1.05991780976532));
#22746=CARTESIAN_POINT('Ctrl Pts',(4.02960451979685,5.7410443712721,1.07852773008465));
#22747=CARTESIAN_POINT('Ctrl Pts',(3.86488519773559,5.85320113806293,1.0874554928949));
#22748=CARTESIAN_POINT('Ctrl Pts',(3.60089399270991,6.01694385573736,1.10152611333106));
#22749=CARTESIAN_POINT('Ctrl Pts',(3.50478513799313,6.07342829086807,1.10660761948416));
#22750=CARTESIAN_POINT('Ctrl Pts',(3.33888889818418,6.16567819833357,1.11529721067078));
#22751=CARTESIAN_POINT('Ctrl Pts',(3.26977229165828,6.2026087886183,1.1188935011329));
#22752=CARTESIAN_POINT('Ctrl Pts',(2.84252173647579,6.42177231072161,1.14095893728608));
#22753=CARTESIAN_POINT('Ctrl Pts',(2.46987885139551,6.57410063911161,1.15944994906116));
#22754=CARTESIAN_POINT('Ctrl Pts',(1.89218828862413,6.75415167548213,1.18693426548889));
#22755=CARTESIAN_POINT('Ctrl Pts',(1.69559462082048,6.80616647034856,1.1961026518323));
#22756=CARTESIAN_POINT('Ctrl Pts',(1.22384362942314,6.90927070632869,1.2177994944551));
#22757=CARTESIAN_POINT('Ctrl Pts',(0.947344419517943,6.95257882587064,1.23027198563359));
#22758=CARTESIAN_POINT('Ctrl Pts',(0.548737309762689,6.99078751274997,1.24828400048376));
#22759=CARTESIAN_POINT('Ctrl Pts',(0.428197077049147,6.99920492306276,1.25373700365624));
#22760=CARTESIAN_POINT('Ctrl Pts',(0.133839260142499,7.01212735035969,1.26713460178215));
#22761=CARTESIAN_POINT('Ctrl Pts',(-0.0400437255557122,7.0132901082745,
1.27510979342304));
#22762=CARTESIAN_POINT('Ctrl Pts',(-0.588842850094366,6.99654828430897,
1.30035270897044));
#22763=CARTESIAN_POINT('Ctrl Pts',(-0.962382024109751,6.95501645697339,
1.31760840753119));
#22764=CARTESIAN_POINT('Ctrl Pts',(-1.52562683409449,6.84612769934643,1.34367692070361));
#22765=CARTESIAN_POINT('Ctrl Pts',(-1.71876625190528,6.80020925915605,1.35263330246511));
#22766=CARTESIAN_POINT('Ctrl Pts',(-2.16000731735223,6.67530296431773,1.37324820797228));
#22767=CARTESIAN_POINT('Ctrl Pts',(-2.40617696132,6.59057004050047,1.38486160845223));
#22768=CARTESIAN_POINT('Ctrl Pts',(-2.76869089556182,6.44276560460703,1.40244212312232));
#22769=CARTESIAN_POINT('Ctrl Pts',(-2.88889593140564,6.38976975176113,1.40835606004339));
#22770=CARTESIAN_POINT('Ctrl Pts',(-3.1193879371304,6.28031658599071,1.41993058842503));
#22771=CARTESIAN_POINT('Ctrl Pts',(-3.22980763527441,6.22425089625768,1.42558774449429));
#22772=CARTESIAN_POINT('Ctrl Pts',(-3.51253867514311,6.07114389917868,1.44033016396364));
#22773=CARTESIAN_POINT('Ctrl Pts',(-3.6823338936865,5.96968450062091,1.44943719768248));
#22774=CARTESIAN_POINT('Ctrl Pts',(-4.05289941509658,5.72642434443336,1.46981380593275));
#22775=CARTESIAN_POINT('Ctrl Pts',(-4.25096605565736,5.58096945780786,1.4810564867486));
#22776=CARTESIAN_POINT('Ctrl Pts',(-4.59321746301029,5.3008185832543,1.50115837571214));
#22777=CARTESIAN_POINT('Ctrl Pts',(-4.74013059600811,5.1698634318345,1.51003964146286));
#22778=CARTESIAN_POINT('Ctrl Pts',(-5.06321648100504,4.8565068317316,1.53027673730393));
#22779=CARTESIAN_POINT('Ctrl Pts',(-5.23539368083716,4.67038250404488,1.54159104914307));
#22780=CARTESIAN_POINT('Ctrl Pts',(-5.48939864600899,4.36406113378797,1.55945237351226));
#22781=CARTESIAN_POINT('Ctrl Pts',(-5.57821398391441,4.24994763216309,1.56595770228343));
#22782=CARTESIAN_POINT('Ctrl Pts',(-5.73751506703633,4.03166692716497,1.57821810049252));
#22783=CARTESIAN_POINT('Ctrl Pts',(-5.80884984573459,3.92819040919106,1.58396099058554));
#22784=CARTESIAN_POINT('Ctrl Pts',(-5.98915441136919,3.65098509479588,1.59912627575862));
#22785=CARTESIAN_POINT('Ctrl Pts',(-6.09335180602451,3.47429508306388,1.60857163925835));
#22786=CARTESIAN_POINT('Ctrl Pts',(-6.29312264193406,3.0988312280876,1.6281169753501));
#22787=CARTESIAN_POINT('Ctrl Pts',(-6.38736856202891,2.89959869798888,1.63820181520507));
#22788=CARTESIAN_POINT('Ctrl Pts',(-6.53856613128265,2.53666513588663,1.65608648002703));
#22789=CARTESIAN_POINT('Ctrl Pts',(-6.59912728896108,2.3746657192263,1.66390616530035));
#22790=CARTESIAN_POINT('Ctrl Pts',(-6.76468036029949,1.87636918106151,1.68755680402165));
#22791=CARTESIAN_POINT('Ctrl Pts',(-6.85038059533619,1.53425718069475,1.70323109943137));
#22792=CARTESIAN_POINT('Ctrl Pts',(-6.92785816130958,1.08328913852958,1.72383606851373));
#22793=CARTESIAN_POINT('Ctrl Pts',(-6.94335881845196,0.979031222269562,
1.72859848252526));
#22794=CARTESIAN_POINT('Ctrl Pts',(-6.99295834142992,0.584458581263378,
1.74668492580571));
#22795=CARTESIAN_POINT('Ctrl Pts',(-7.01124254080886,0.292460787846147,
1.76016286206212));
#22796=CARTESIAN_POINT('Ctrl Pts',(-7.01124999771819,0.000178876124116781,
1.77360028780278));
#22797=CARTESIAN_POINT('Ctrl Pts',(-7.01124999779487,0.000175845004380833,
1.77353435691035));
#22798=CARTESIAN_POINT('Ctrl Pts',(-7.01125469776653,-0.187220302170659,
1.78204174915585));
#22799=CARTESIAN_POINT('Ctrl Pts',(-7.00374199053544,-0.374635673529691,
1.79054914140135));
#22800=CARTESIAN_POINT('Ctrl Pts',(-6.98873332011083,-0.561456269777726,
1.79905653364685));
#22801=CARTESIAN_POINT('Ctrl Pts',(-6.97372411902929,-0.748283471383788,
1.80756422668558));
#22802=CARTESIAN_POINT('Ctrl Pts',(-6.95121844661908,-0.934515547269003,
1.81607191972432));
#22803=CARTESIAN_POINT('Ctrl Pts',(-6.92128973059513,-1.11954232955185,
1.82457961276305));
#22804=CARTESIAN_POINT('Ctrl Pts',(-6.89136184031077,-1.30456400690681,
1.83308707107274));
#22805=CARTESIAN_POINT('Ctrl Pts',(-6.85401136725828,-1.48838015211063,
1.84159452938244));
#22806=CARTESIAN_POINT('Ctrl Pts',(-6.80936316069837,-1.67038914873869,
1.85010198769213));
#22807=CARTESIAN_POINT('Ctrl Pts',(-6.76470558146594,-1.85243635318854,
1.85861123191052));
#22808=CARTESIAN_POINT('Ctrl Pts',(-6.71274728206629,-2.03267535073124,
1.86712047612892));
#22809=CARTESIAN_POINT('Ctrl Pts',(-6.65366367649957,-2.2105171889244,1.87562972034732));
#22810=CARTESIAN_POINT('Ctrl Pts',(-6.62788311018922,-2.28811677443237,
1.87934264769356));
#22811=CARTESIAN_POINT('Ctrl Pts',(-6.60074657699216,-2.36526015197544,
1.8830555750398));
#22812=CARTESIAN_POINT('Ctrl Pts',(-6.5722715952584,-2.44189939200199,1.88676850238605));
#22813=CARTESIAN_POINT('',(-7.01124999783523,-0.000174228519746755,1.22646564308963));
#22814=CARTESIAN_POINT('Ctrl Pts',(-6.57174751820247,-2.44170444323764,
1.33970341751688));
#22815=CARTESIAN_POINT('Ctrl Pts',(-6.75170954457185,-1.95778367933175,
1.31626836550204));
#22816=CARTESIAN_POINT('Ctrl Pts',(-6.95635145461453,-1.14674394506303,
1.27852244232832));
#22817=CARTESIAN_POINT('Ctrl Pts',(-7.01140638052565,-0.315405155950845,
1.24077651915461));
#22818=CARTESIAN_POINT('Ctrl Pts',(-7.01110477910546,-0.000174332979431822,
1.22646564799572));
#22819=CARTESIAN_POINT('Ctrl Pts',(-7.01124999783522,-0.000174228519746755,
1.22646564308963));
#22820=CARTESIAN_POINT('Ctrl Pts',(-7.01125465583345,0.187271490041512,
1.21795614517059));
#22821=CARTESIAN_POINT('Ctrl Pts',(-7.00373793128268,0.37473528203682,1.20944664725154));
#22822=CARTESIAN_POINT('Ctrl Pts',(-6.98872154284581,0.561602848161269,
1.2009371493325));
#22823=CARTESIAN_POINT('Ctrl Pts',(-6.9737043785875,0.748480068795355,1.19242721177039));
#22824=CARTESIAN_POINT('Ctrl Pts',(-6.95118679760751,0.934760693715983,
1.18391727420828));
#22825=CARTESIAN_POINT('Ctrl Pts',(-6.92124250286083,1.11983426411806,1.17540733664616));
#22826=CARTESIAN_POINT('Ctrl Pts',(-6.891298882398,1.30490366704444,1.16689759071032));
#22827=CARTESIAN_POINT('Ctrl Pts',(-6.8539289340877,1.48876576509718,1.15838784477448));
#22828=CARTESIAN_POINT('Ctrl Pts',(-6.80925778001219,1.6708186759321,1.14987809883864));
#22829=CARTESIAN_POINT('Ctrl Pts',(-6.76457640959323,1.85291322247357,1.14136640671428));
#22830=CARTESIAN_POINT('Ctrl Pts',(-6.71259057104574,2.03319745495257,1.13285471458992));
#22831=CARTESIAN_POINT('Ctrl Pts',(-6.65347595510241,2.21108215075199,1.12434302246556));
#22832=CARTESIAN_POINT('Ctrl Pts',(-6.62358007377258,2.30104331638169,1.12003842649373));
#22833=CARTESIAN_POINT('Ctrl Pts',(-6.59186172858171,2.39039101146068,1.1157338305219));
#22834=CARTESIAN_POINT('Ctrl Pts',(-6.5583484482587,2.47905066380715,1.11142923455007));
#22835=CARTESIAN_POINT('Ctrl Pts',(-6.49192007391006,2.65478746184447,1.10289687633624));
#22836=CARTESIAN_POINT('Ctrl Pts',(-6.41841290841537,2.82788232028147,1.09436451812241));
#22837=CARTESIAN_POINT('Ctrl Pts',(-6.3380624199563,2.99776438754578,1.08583215990858));
#22838=CARTESIAN_POINT('Ctrl Pts',(-6.25772697742553,3.1676146437601,1.07730139941061));
#22839=CARTESIAN_POINT('Ctrl Pts',(-6.1705508999817,3.33425303289975,1.06877063891265));
#22840=CARTESIAN_POINT('Ctrl Pts',(-6.07681697087871,3.49713054731168,1.06023987841468));
#22841=CARTESIAN_POINT('Ctrl Pts',(-5.97904454197702,3.66702559332035,1.05134157251577));
#22842=CARTESIAN_POINT('Ctrl Pts',(-5.87413681319125,3.83282819629963,1.04244326661686));
#22843=CARTESIAN_POINT('Ctrl Pts',(-5.76246730796888,3.99394505308847,1.03354496071795));
#22844=CARTESIAN_POINT('Ctrl Pts',(-5.6554136261984,4.14840219588844,1.02501446346088));
#22845=CARTESIAN_POINT('Ctrl Pts',(-5.54214610708143,4.29855290334076,1.01648396620381));
#22846=CARTESIAN_POINT('Ctrl Pts',(-5.42303765706886,4.44390471685804,1.00795346894674));
#22847=CARTESIAN_POINT('Ctrl Pts',(-5.30392798815565,4.58925801783836,0.999422884392513));
#22848=CARTESIAN_POINT('Ctrl Pts',(-5.17897746534402,4.72981209213407,0.990892299838288));
#22849=CARTESIAN_POINT('Ctrl Pts',(-5.04859908113031,4.86510779741931,0.982361715284064));
#22850=CARTESIAN_POINT('Ctrl Pts',(-4.91819489804679,5.00043027459859,0.973829442724257));
#22851=CARTESIAN_POINT('Ctrl Pts',(-4.78236092142949,5.13049208493782,0.96529717016445));
#22852=CARTESIAN_POINT('Ctrl Pts',(-4.64154738344617,5.25487054547722,0.956764897604643));
#22853=CARTESIAN_POINT('Ctrl Pts',(-4.62336758104229,5.27092848896965,0.955663334279022));
#22854=CARTESIAN_POINT('Ctrl Pts',(-4.60510482600696,5.28689175381491,0.954561770953402));
#22855=CARTESIAN_POINT('Ctrl Pts',(-4.58676012916224,5.30275947785939,0.953460207627781));
#22856=CARTESIAN_POINT('Ctrl Pts',(-4.44466795782465,5.42566580783316,0.944927849413946));
#22857=CARTESIAN_POINT('Ctrl Pts',(-4.29760892848704,5.54287832971843,0.93639549120011));
#22858=CARTESIAN_POINT('Ctrl Pts',(-4.14606191555579,5.65400717676214,0.927863132986275));
#22859=CARTESIAN_POINT('Ctrl Pts',(-3.99454328036692,5.76511521451553,0.919332372488281));
#22860=CARTESIAN_POINT('Ctrl Pts',(-3.8385385853446,5.87014166996735,0.910801611990286));
#22861=CARTESIAN_POINT('Ctrl Pts',(-3.67855791096258,5.96873841428778,0.902270851492292));
#22862=CARTESIAN_POINT('Ctrl Pts',(-3.51168451451707,6.07158317142346,0.893372545593392));
#22863=CARTESIAN_POINT('Ctrl Pts',(-3.34048522943482,6.16743169515204,0.884474239694491));
#22864=CARTESIAN_POINT('Ctrl Pts',(-3.1655710211493,6.25594011101128,0.875575933795591));
#22865=CARTESIAN_POINT('Ctrl Pts',(-2.9978868359848,6.34079005967487,0.867045436538524));
#22866=CARTESIAN_POINT('Ctrl Pts',(-2.82678895492625,6.41889435489977,0.858514939281457));
#22867=CARTESIAN_POINT('Ctrl Pts',(-2.65283978343348,6.48999750739032,0.849984442024389));
#22868=CARTESIAN_POINT('Ctrl Pts',(-2.47888883182517,6.56110138751773,0.84145385747015));
#22869=CARTESIAN_POINT('Ctrl Pts',(-2.30208681593066,6.62520386896563,0.832923272915911));
#22870=CARTESIAN_POINT('Ctrl Pts',(-2.1230155277549,6.68209784659067,0.824392688361672));
#22871=CARTESIAN_POINT('Ctrl Pts',(-1.94390880550797,6.73900308221955,0.815860415801817));
#22872=CARTESIAN_POINT('Ctrl Pts',(-1.76253220605297,6.78869687341039,0.807328143241962));
#22873=CARTESIAN_POINT('Ctrl Pts',(-1.57948290834741,6.83102190779231,0.798795870682106));
#22874=CARTESIAN_POINT('Ctrl Pts',(-1.5558502370159,6.83648630257109,0.797694307356568));
#22875=CARTESIAN_POINT('Ctrl Pts',(-1.53218970172665,6.84182794236975,0.79659274403103));
#22876=CARTESIAN_POINT('Ctrl Pts',(-1.50850260187556,6.84704655034816,0.795491180705493));
#22877=CARTESIAN_POINT('Ctrl Pts',(-1.32502988061606,6.8874682234532,0.786958822491666));
#22878=CARTESIAN_POINT('Ctrl Pts',(-1.13990061171332,6.92051799186226,0.77842646427784));
#22879=CARTESIAN_POINT('Ctrl Pts',(-0.95372153551622,6.94608103862837,0.769894106064014));
#22880=CARTESIAN_POINT('Ctrl Pts',(-0.767577322044346,6.9716392986188,0.761363345566032));
#22881=CARTESIAN_POINT('Ctrl Pts',(-0.580383996592522,6.98971359307129,
0.752832585068051));
#22882=CARTESIAN_POINT('Ctrl Pts',(-0.392755867337207,7.00024066666084,
0.744301824570069));
#22883=CARTESIAN_POINT('Ctrl Pts',(-0.197043833252064,7.0112212962357,0.735403518671163));
#22884=CARTESIAN_POINT('Ctrl Pts',(-0.00085904929266481,7.01398991619409,
0.726505212772258));
#22885=CARTESIAN_POINT('Ctrl Pts',(0.19509748762768,7.00853504898287,0.717606906873352));
#22886=CARTESIAN_POINT('Ctrl Pts',(0.382954223471156,7.00330565697144,0.709076409616276));
#22887=CARTESIAN_POINT('Ctrl Pts',(0.570600875278154,6.99051894899005,0.7005459123592));
#22888=CARTESIAN_POINT('Ctrl Pts',(0.757421232792699,6.97021804813987,0.692015415102123));
#22889=CARTESIAN_POINT('Ctrl Pts',(0.944243502139027,6.94991693953981,0.683484830547945));
#22890=CARTESIAN_POINT('Ctrl Pts',(1.13023915645784,6.92210152068343,0.674954245993767));
#22891=CARTESIAN_POINT('Ctrl Pts',(1.31479797593136,6.88686669284275,0.666423661439589));
#22892=CARTESIAN_POINT('Ctrl Pts',(1.49939331533318,6.85162489284332,0.657891388879727));
#22893=CARTESIAN_POINT('Ctrl Pts',(1.68255095165807,6.80896080995481,0.649359116319865));
#22894=CARTESIAN_POINT('Ctrl Pts',(1.86367084333698,6.75902045789149,0.640826843760003));
#22895=CARTESIAN_POINT('Ctrl Pts',(1.88705441773763,6.752572883706,0.639725280434402));
#22896=CARTESIAN_POINT('Ctrl Pts',(1.91040404455407,6.74600409587929,0.638623717108802));
#22897=CARTESIAN_POINT('Ctrl Pts',(1.93371844932792,6.7393144696793,0.637522153783201));
#22898=CARTESIAN_POINT('Ctrl Pts',(2.11430439336691,6.68749875856379,0.628989795569389));
#22899=CARTESIAN_POINT('Ctrl Pts',(2.2928368916444,6.62841170029351,0.620457437355577));
#22900=CARTESIAN_POINT('Ctrl Pts',(2.46872772896921,6.56224123015289,0.611925079141765));
#22901=CARTESIAN_POINT('Ctrl Pts',(2.64458563007975,6.49608315067921,0.603394318643801));
#22902=CARTESIAN_POINT('Ctrl Pts',(2.81780257113077,6.42284441402677,0.594863558145838));
#22903=CARTESIAN_POINT('Ctrl Pts',(2.98780823326861,6.34276190028542,0.586332797647874));
#22904=CARTESIAN_POINT('Ctrl Pts',(3.16513854123012,6.25922905411132,0.577434491748961));
#22905=CARTESIAN_POINT('Ctrl Pts',(3.33897439771579,6.16824977232899,0.568536185850047));
#22906=CARTESIAN_POINT('Ctrl Pts',(3.50869390715765,6.07014774353761,0.559637879951134));
#22907=CARTESIAN_POINT('Ctrl Pts',(3.67139811470115,5.97610073087889,0.55110738269408));
#22908=CARTESIAN_POINT('Ctrl Pts',(3.83031914624211,5.87550812891856,0.542576885437027));
#22909=CARTESIAN_POINT('Ctrl Pts',(3.98493566267762,5.76870126864099,0.534046388179973));
#22910=CARTESIAN_POINT('Ctrl Pts',(4.13955376138723,5.66189331535127,0.525515803625745));
#22911=CARTESIAN_POINT('Ctrl Pts',(4.28986700705451,5.54887115323685,0.516985219071517));
#22912=CARTESIAN_POINT('Ctrl Pts',(4.43538398265685,5.43000879270845,0.508454634517289));
#22913=CARTESIAN_POINT('Ctrl Pts',(4.58092975270658,5.31112291206515,0.499922361957472));
#22914=CARTESIAN_POINT('Ctrl Pts',(4.72167712078367,5.18639471921427,0.491390089397654));
#22915=CARTESIAN_POINT('Ctrl Pts',(4.85716795756154,5.05623832453905,0.482857816837836));
#22916=CARTESIAN_POINT('Ctrl Pts',(4.87466056995861,5.03943441796354,0.481756253512194));
#22917=CARTESIAN_POINT('Ctrl Pts',(4.89206561392294,5.02254008487155,0.480654690186552));
#22918=CARTESIAN_POINT('Ctrl Pts',(4.90938214742827,5.00555626209641,0.47955312686091));
#22919=CARTESIAN_POINT('Ctrl Pts',(5.04351049343434,4.87400498729954,0.471020768647081));
#22920=CARTESIAN_POINT('Ctrl Pts',(5.17237084479945,4.73703731504642,0.462488410433252));
#22921=CARTESIAN_POINT('Ctrl Pts',(5.29553543293831,4.5950985888221,0.453956052219423));
#22922=CARTESIAN_POINT('Ctrl Pts',(5.41867695804973,4.45318644115244,0.445425291721419));
#22923=CARTESIAN_POINT('Ctrl Pts',(5.53612464792779,4.30630532815229,0.436894531223415));
#22924=CARTESIAN_POINT('Ctrl Pts',(5.64748977655617,4.154935112152,0.428363770725412));
#22925=CARTESIAN_POINT('Ctrl Pts',(5.7636530402227,3.99704315325006,0.419465464826512));
#22926=CARTESIAN_POINT('Ctrl Pts',(5.87319777382074,3.83426696932088,0.410567158927613));
#22927=CARTESIAN_POINT('Ctrl Pts',(5.97573123079891,3.66718731724391,0.401668853028713));
#22928=CARTESIAN_POINT('Ctrl Pts',(6.07402649997131,3.50701384940077,0.393138355771637));
#22929=CARTESIAN_POINT('Ctrl Pts',(6.16587828585823,3.34288580406798,0.384607858514561));
#22930=CARTESIAN_POINT('Ctrl Pts',(6.25098590644932,3.17534277832678,0.376077361257485));
#22931=CARTESIAN_POINT('Ctrl Pts',(6.33609439799203,3.00779803802854,0.367546776703286));
#22932=CARTESIAN_POINT('Ctrl Pts',(6.41445845063592,2.8368385217534,0.359016192149087));
#22933=CARTESIAN_POINT('Ctrl Pts',(6.48582401665194,2.66302710979834,0.350485607594888));
#22934=CARTESIAN_POINT('Ctrl Pts',(6.55720370426484,2.48918130458011,0.341953335035072));
#22935=CARTESIAN_POINT('Ctrl Pts',(6.62158202404142,2.31248276000431,0.333421062475256));
#22936=CARTESIAN_POINT('Ctrl Pts',(6.67875329391682,2.13351376876158,0.32488878991544));
#22937=CARTESIAN_POINT('Ctrl Pts',(6.68613441937098,2.11040788743961,0.323787226589833));
#22938=CARTESIAN_POINT('Ctrl Pts',(6.69339548359188,2.08726418435723,0.322685663264226));
#22939=CARTESIAN_POINT('Ctrl Pts',(6.70053610427249,2.06408393187896,0.32158409993862));
#22940=CARTESIAN_POINT('Ctrl Pts',(6.75584507480538,1.88453708873849,0.313051741724777));
#22941=CARTESIAN_POINT('Ctrl Pts',(6.80394253568359,1.70273563755189,0.304519383510934));
#22942=CARTESIAN_POINT('Ctrl Pts',(6.84466437466792,1.51927487988572,0.295987025297092));
#22943=CARTESIAN_POINT('Ctrl Pts',(6.88537858833604,1.3358484759306,0.287456264799144));
#22944=CARTESIAN_POINT('Ctrl Pts',(6.91871987002713,1.15076368414967,0.278925504301196));
#22945=CARTESIAN_POINT('Ctrl Pts',(6.94457487631809,0.964627570470402,0.270394743803248));
#22946=CARTESIAN_POINT('Ctrl Pts',(6.97154383823544,0.770471835029124,0.261496437904338));
#22947=CARTESIAN_POINT('Ctrl Pts',(6.9903670753975,0.575172525106002,0.252598132005428));
#22948=CARTESIAN_POINT('Ctrl Pts',(7.00097575007869,0.3794273439146,0.243699826106518));
#22949=CARTESIAN_POINT('Ctrl Pts',(7.01114591856887,0.191773227478618,0.235169328849452));
#22950=CARTESIAN_POINT('Ctrl Pts',(7.01376694603514,0.00370968489178242,
0.226638831592386));
#22951=CARTESIAN_POINT('Ctrl Pts',(7.00883135452383,-0.18414561179569,0.218108334335321));
#22952=CARTESIAN_POINT('Ctrl Pts',(7.00389571250398,-0.372002830906788,
0.209577749781118));
#22953=CARTESIAN_POINT('Ctrl Pts',(6.99140330825087,-0.559651494072332,
0.201047165226916));
#22954=CARTESIAN_POINT('Ctrl Pts',(6.97139875862046,-0.746475659887957,
0.192516580672714));
#22955=CARTESIAN_POINT('Ctrl Pts',(6.95139025055174,-0.933336793890739,
0.183984308112868));
#22956=CARTESIAN_POINT('Ctrl Pts',(6.92386666175923,-1.11937280054723,0.175452035553022));
#22957=CARTESIAN_POINT('Ctrl Pts',(6.88892438331984,-1.30397369735794,0.166919762993175));
#22958=CARTESIAN_POINT('Ctrl Pts',(6.88441314294721,-1.32780668867135,0.16581819966756));
#22959=CARTESIAN_POINT('Ctrl Pts',(6.87977831627972,-1.35161577155493,0.164716636341944));
#22960=CARTESIAN_POINT('Ctrl Pts',(6.87502017297057,-1.37539964510236,0.163615073016328));
#22961=CARTESIAN_POINT('Ctrl Pts',(6.83816511234691,-1.559621944538,0.155082714802508));
#22962=CARTESIAN_POINT('Ctrl Pts',(6.79389498193691,-1.74239308271298,0.146550356588688));
#22963=CARTESIAN_POINT('Ctrl Pts',(6.74234892197997,-1.92311143119049,0.138017998374868));
#22964=CARTESIAN_POINT('Ctrl Pts',(6.69081251421497,-2.10379593948338,0.129487237876939));
#22965=CARTESIAN_POINT('Ctrl Pts',(6.63200297973483,-2.28242813106,0.12095647737901));
#22966=CARTESIAN_POINT('Ctrl Pts',(6.56610970461094,-2.45842020604981,0.112425716881081));
#22967=CARTESIAN_POINT('Ctrl Pts',(6.49737743638276,-2.64199484976712,0.103527410982161));
#22968=CARTESIAN_POINT('Ctrl Pts',(6.42093760606955,-2.82269650182234,0.0946291050832411));
#22969=CARTESIAN_POINT('Ctrl Pts',(6.3370618935737,-2.99987885080649,0.0857307991843212));
#22970=CARTESIAN_POINT('Ctrl Pts',(6.25665315695463,-3.16973742379592,0.0772003019272322));
#22971=CARTESIAN_POINT('Ctrl Pts',(6.16941103836503,-3.33636148742264,0.0686698046701432));
#22972=CARTESIAN_POINT('Ctrl Pts',(6.07562306814898,-3.49920432331065,0.0601393074130542));
#22973=CARTESIAN_POINT('Ctrl Pts',(5.9818341381507,-3.6620488256561,0.0516087228588453));
#22974=CARTESIAN_POINT('Ctrl Pts',(5.88149937818162,-3.82111175940824,0.0430781383046364));
#22975=CARTESIAN_POINT('Ctrl Pts',(5.77495130476384,-3.97587273313753,0.0345475537504275));
#22976=CARTESIAN_POINT('Ctrl Pts',(5.66838214794392,-4.13066433048805,0.0260152811906182));
#22977=CARTESIAN_POINT('Ctrl Pts',(5.55559739641577,-4.28115201614751,0.0174830086308088));
#22978=CARTESIAN_POINT('Ctrl Pts',(5.43697225766915,-4.42684529115667,0.00895073607099953));
#22979=CARTESIAN_POINT('Ctrl Pts',(5.42165709967018,-4.44565509445578,0.00784917274534623));
#22980=CARTESIAN_POINT('Ctrl Pts',(5.40624464856188,-4.46438502763424,0.00674760941969292));
#22981=CARTESIAN_POINT('Ctrl Pts',(5.39073576089718,-4.48303407511969,0.00564604609403962));
#22982=CARTESIAN_POINT('Ctrl Pts',(5.27060886308617,-4.62748364945361,-0.00288631211978283));
#22983=CARTESIAN_POINT('Ctrl Pts',(5.14465240415034,-4.76712642172868,-0.0114186703336053));
#22984=CARTESIAN_POINT('Ctrl Pts',(5.01327520578717,-4.9014995943629,-0.0199510285474277));
#22985=CARTESIAN_POINT('Ctrl Pts',(4.88192260829423,-5.03584760511953,-0.028481789045362));
#22986=CARTESIAN_POINT('Ctrl Pts',(4.74515151086828,-5.16492776673308,-0.0370125495432962));
#22987=CARTESIAN_POINT('Ctrl Pts',(4.60340833500619,-5.28831336663171,-0.0455433100412305));
#22988=CARTESIAN_POINT('Ctrl Pts',(4.45555819453976,-5.41701500017134,-0.0544416159401489));
#22989=CARTESIAN_POINT('Ctrl Pts',(4.30229829444563,-5.53952025612765,-0.0633399218390673));
#22990=CARTESIAN_POINT('Ctrl Pts',(4.14417528276514,-5.65539015349237,-0.0722382277379857));
#22991=CARTESIAN_POINT('Ctrl Pts',(3.99258823543917,-5.76647060553293,-0.0807687249950581));
#22992=CARTESIAN_POINT('Ctrl Pts',(3.83653228743178,-5.87145301799739,-0.0892992222521305));
#22993=CARTESIAN_POINT('Ctrl Pts',(3.67652060358513,-5.96999353550019,-0.0978297195092029));
#22994=CARTESIAN_POINT('Ctrl Pts',(3.51650728225407,-6.06853506142036,-0.106360304063377));
#22995=CARTESIAN_POINT('Ctrl Pts',(3.35253840642575,-6.16063440295548,-0.114890888617551));
#22996=CARTESIAN_POINT('Ctrl Pts',(3.18515416446187,-6.24599227594073,-0.123421473171726));
#22997=CARTESIAN_POINT('Ctrl Pts',(3.01773680102362,-6.33136703927699,-0.131953745731499));
#22998=CARTESIAN_POINT('Ctrl Pts',(2.84690299468735,-6.4099975316115,-0.140486018291272));
#22999=CARTESIAN_POINT('Ctrl Pts',(2.67321624127837,-6.48163108251816,-0.149018290851045));
#23000=CARTESIAN_POINT('Ctrl Pts',(2.65079232591689,-6.49087936801516,-0.15011985417678));
#23001=CARTESIAN_POINT('Ctrl Pts',(2.62832088499811,-6.50001109234066,-0.151221417502516));
#23002=CARTESIAN_POINT('Ctrl Pts',(2.60580315531013,-6.50902577028819,-0.152322980828251));
#23003=CARTESIAN_POINT('Ctrl Pts',(2.43138800243462,-6.57885059073544,-0.16085533904209));
#23004=CARTESIAN_POINT('Ctrl Pts',(2.25413532275062,-6.64167272808602,-0.169387697255928));
#23005=CARTESIAN_POINT('Ctrl Pts',(2.07462498107822,-6.69727987696395,-0.177920055469766));
#23006=CARTESIAN_POINT('Ctrl Pts',(1.89514825338543,-6.75287661319627,-0.186450815967772));
#23007=CARTESIAN_POINT('Ctrl Pts',(1.71341499952775,-6.80126096661933,-0.194981576465778));
#23008=CARTESIAN_POINT('Ctrl Pts',(1.53002096621149,-6.84227026691092,-0.203512336963784));
#23009=CARTESIAN_POINT('Ctrl Pts',(1.33872545289098,-6.88504644129532,-0.21241064286268));
#23010=CARTESIAN_POINT('Ctrl Pts',(1.1456232205715,-6.91979788136369,-0.221308948761577));
#23011=CARTESIAN_POINT('Ctrl Pts',(0.951403993087149,-6.94639885152284,
-0.230207254660473));
#23012=CARTESIAN_POINT('Ctrl Pts',(0.765212755547516,-6.97190027904801,
-0.238737751917524));
#23013=CARTESIAN_POINT('Ctrl Pts',(0.577995331319964,-6.98991143949831,
-0.247268249174574));
#23014=CARTESIAN_POINT('Ctrl Pts',(0.390366706047602,-7.00037430408614,
-0.255798746431625));
#23015=CARTESIAN_POINT('Ctrl Pts',(0.202736160669771,-7.01083727574615,
-0.264329330985879));
#23016=CARTESIAN_POINT('Ctrl Pts',(0.0146947115222116,-7.01375178338187,
-0.272859915540134));
#23017=CARTESIAN_POINT('Ctrl Pts',(-0.173140114982729,-7.00911185979249,
-0.281390500094389));
#23018=CARTESIAN_POINT('Ctrl Pts',(-0.361012109659622,-7.00447101806945,
-0.289922772654215));
#23019=CARTESIAN_POINT('Ctrl Pts',(-0.548677094163707,-6.99227276804658,
-0.298455045214041));
#23020=CARTESIAN_POINT('Ctrl Pts',(-0.735519241624514,-6.97256323081405,
-0.306987317773867));
#23021=CARTESIAN_POINT('Ctrl Pts',(-0.759641590725308,-6.97001862113043,
-0.308088881099424));
#23022=CARTESIAN_POINT('Ctrl Pts',(-0.783750231116449,-6.96734888248705,
-0.309190444424982));
#23023=CARTESIAN_POINT('Ctrl Pts',(-0.807843844180328,-6.96455417711141,
-0.310292007750539));
#23024=CARTESIAN_POINT('Ctrl Pts',(-0.994465287139578,-6.94290728054736,
-0.318824365964374));
#23025=CARTESIAN_POINT('Ctrl Pts',(-1.18024759914043,-6.91375139016416,
-0.327356724178208));
#23026=CARTESIAN_POINT('Ctrl Pts',(-1.36457977895502,-6.87717591670935,
-0.335889082392043));
#23027=CARTESIAN_POINT('Ctrl Pts',(-1.54887744188274,-6.8406072921481,-0.344419842890039));
#23028=CARTESIAN_POINT('Ctrl Pts',(-1.73172521451693,-6.79662191666365,
-0.352950603388035));
#23029=CARTESIAN_POINT('Ctrl Pts',(-1.91252176355406,-6.74536041041782,
-0.361481363886031));
#23030=CARTESIAN_POINT('Ctrl Pts',(-2.10110788072095,-6.6918903166881,-0.370379669784931));
#23031=CARTESIAN_POINT('Ctrl Pts',(-2.28746176066021,-6.63050329733387,
-0.37927797568383));
#23032=CARTESIAN_POINT('Ctrl Pts',(-2.47091701666132,-6.56141719899547,
-0.38817628158273));
#23033=CARTESIAN_POINT('Ctrl Pts',(-2.64678920805253,-6.49518675254061,
-0.39670677883978));
#23034=CARTESIAN_POINT('Ctrl Pts',(-2.81999727924531,-6.42188102350908,
-0.405237276096829));
#23035=CARTESIAN_POINT('Ctrl Pts',(-2.98997280427668,-6.34174181059004,
-0.413767773353879));
#23036=CARTESIAN_POINT('Ctrl Pts',(-3.15995006876101,-6.2616017775624,-0.422298357908195));
#23037=CARTESIAN_POINT('Ctrl Pts',(-3.32669444560058,-6.17462825432024,
-0.430828942462511));
#23038=CARTESIAN_POINT('Ctrl Pts',(-3.4896600638369,-6.08111003036139,-0.439359527016827));
#23039=CARTESIAN_POINT('Ctrl Pts',(-3.65265792920186,-5.98757330130783,
-0.447891799576629));
#23040=CARTESIAN_POINT('Ctrl Pts',(-3.81187527764207,-5.88748943813292,
-0.456424072136431));
#23041=CARTESIAN_POINT('Ctrl Pts',(-3.96679253468986,-5.78119222559056,
-0.464956344696233));
#23042=CARTESIAN_POINT('Ctrl Pts',(-3.98679320481144,-5.76746867068508,
-0.466057908021765));
#23043=CARTESIAN_POINT('Ctrl Pts',(-4.00672223952132,-5.75364160948471,
-0.467159471347298));
#23044=CARTESIAN_POINT('Ctrl Pts',(-4.02657855652151,-5.73971181250951,
-0.468261034672831));
#23045=CARTESIAN_POINT('Ctrl Pts',(-4.18037925551463,-5.63181604756988,
-0.476793392886621));
#23046=CARTESIAN_POINT('Ctrl Pts',(-4.32986662685901,-5.51771670837547,
-0.485325751100411));
#23047=CARTESIAN_POINT('Ctrl Pts',(-4.47454595206147,-5.39778334924535,
-0.493858109314201));
#23048=CARTESIAN_POINT('Ctrl Pts',(-4.61919818552228,-5.2778724480827,-0.502388869812187));
#23049=CARTESIAN_POINT('Ctrl Pts',(-4.75904393408753,-5.15212990229196,
-0.510919630310174));
#23050=CARTESIAN_POINT('Ctrl Pts',(-4.89362136437337,-5.02096569443056,
-0.51945039080816));
#23051=CARTESIAN_POINT('Ctrl Pts',(-5.03399702514309,-4.88415031380712,
-0.528348696707074));
#23052=CARTESIAN_POINT('Ctrl Pts',(-5.16864007484259,-4.74143597016446,
-0.537247002605987));
#23053=CARTESIAN_POINT('Ctrl Pts',(-5.29706824614347,-4.593331531492,-0.5461453085049));
#23054=CARTESIAN_POINT('Ctrl Pts',(-5.42018787986454,-4.45134894264784,
-0.554675805761967));
#23055=CARTESIAN_POINT('Ctrl Pts',(-5.53759587132219,-4.30441314245886,
-0.563206303019034));
#23056=CARTESIAN_POINT('Ctrl Pts',(-5.64890750104157,-4.15300741718291,
-0.571736800276102));
#23057=CARTESIAN_POINT('Ctrl Pts',(-5.76022026987218,-4.00160014249149,
-0.580267384830293));
#23058=CARTESIAN_POINT('Ctrl Pts',(-5.86543637366439,-3.84572309974774,
-0.588797969384485));
#23059=CARTESIAN_POINT('Ctrl Pts',(-5.96421330176928,-3.68589015754653,
-0.597328553938677));
#23060=CARTESIAN_POINT('Ctrl Pts',(-6.06300977554652,-3.52602558809817,
-0.605860826498497));
#23061=CARTESIAN_POINT('Ctrl Pts',(-6.15536436876196,-3.36220381657647,
-0.614393099058317));
#23062=CARTESIAN_POINT('Ctrl Pts',(-6.24097911952844,-3.19496575758021,
-0.622925371618137));
#23063=CARTESIAN_POINT('Ctrl Pts',(-6.25203245484078,-3.17337440414494,
-0.624026934943799));
#23064=CARTESIAN_POINT('Ctrl Pts',(-6.26297351185236,-3.15172614053068,
-0.625128498269461));
#23065=CARTESIAN_POINT('Ctrl Pts',(-6.27380170571591,-3.13002215964299,
-0.626230061595122));
#23066=CARTESIAN_POINT('Ctrl Pts',(-6.35745714771697,-2.9623435848758,-0.634740415959077));
#23067=CARTESIAN_POINT('Ctrl Pts',(-6.43440197266013,-2.79127817175156,
-0.643250770323033));
#23068=CARTESIAN_POINT('Ctrl Pts',(-6.50437781620031,-2.61738338548661,
-0.651761124686988));
#23069=CARTESIAN_POINT('Ctrl Pts',(-6.5277917422228,-2.55919816819849,-0.654608690324241));
#23070=CARTESIAN_POINT('Ctrl Pts',(-6.55042583092581,-2.50069636654977,
-0.657456255961495));
#23071=CARTESIAN_POINT('Ctrl Pts',(-6.5722715952584,-2.44189939200198,-0.660303821598748));
#23072=CARTESIAN_POINT('Origin',(0.,0.,0.));
#23073=CARTESIAN_POINT('',(-6.57261910096697,-2.44202878201564,-2.66029322980694));
#23074=CARTESIAN_POINT('',(-6.57227163721606,-2.44189927907465,-2.11302806574593));
#23075=CARTESIAN_POINT('',(-6.57227159525839,-2.441899392002,0.));
#23076=CARTESIAN_POINT('Ctrl Pts',(-6.57227163721606,-2.44189927907466,
-2.11302806574593));
#23077=CARTESIAN_POINT('Ctrl Pts',(-6.51953748579793,-2.5838310821789,-2.10622305876647));
#23078=CARTESIAN_POINT('Ctrl Pts',(-6.46220633364772,-2.72405292621106,
-2.09944006788617));
#23079=CARTESIAN_POINT('Ctrl Pts',(-6.33650509248318,-3.00512819872079,
-2.08564570072172));
#23080=CARTESIAN_POINT('Ctrl Pts',(-6.26788868974173,-3.1457372854464,-2.07863975024577));
#23081=CARTESIAN_POINT('Ctrl Pts',(-6.15383678120463,-3.36087845473853,
-2.06767142613725));
#23082=CARTESIAN_POINT('Ctrl Pts',(-6.11161603784971,-3.43705691998926,
-2.06373707023924));
#23083=CARTESIAN_POINT('Ctrl Pts',(-5.99986890027327,-3.63010861102319,
-2.05360831065317));
#23084=CARTESIAN_POINT('Ctrl Pts',(-5.92834201533009,-3.74578101905171,
-2.04738680115132));
#23085=CARTESIAN_POINT('Ctrl Pts',(-5.69016811754324,-4.10702550372183,
-2.02752645117635));
#23086=CARTESIAN_POINT('Ctrl Pts',(-5.51127520696392,-4.34413621110689,
-2.01384649718659));
#23087=CARTESIAN_POINT('Ctrl Pts',(-5.19460340716075,-4.71269729482426,
-1.99160728170246));
#23088=CARTESIAN_POINT('Ctrl Pts',(-5.06554858082755,-4.85114826985282,
-1.98299428255651));
#23089=CARTESIAN_POINT('Ctrl Pts',(-4.71483135622538,-5.19812482824586,
-1.96065680487294));
#23090=CARTESIAN_POINT('Ctrl Pts',(-4.48492016006575,-5.39774311405849,
-1.94704021335579));
#23091=CARTESIAN_POINT('Ctrl Pts',(-4.07276902366969,-5.71102252482692,
-1.92384579853699));
#23092=CARTESIAN_POINT('Ctrl Pts',(-3.89695293238659,-5.8324078513493,-1.91428098375394));
#23093=CARTESIAN_POINT('Ctrl Pts',(-3.62003185496311,-6.00547831241529,
-1.89948619697423));
#23094=CARTESIAN_POINT('Ctrl Pts',(-3.52275654162347,-6.0630508716118,-1.89433181645506));
#23095=CARTESIAN_POINT('Ctrl Pts',(-3.18463566105164,-6.25228339227409,
-1.87658940572744));
#23096=CARTESIAN_POINT('Ctrl Pts',(-2.93747413220861,-6.37214232036376,
-1.86393092679018));
#23097=CARTESIAN_POINT('Ctrl Pts',(-2.48580379030894,-6.55929853983847,
-1.84149219324628));
#23098=CARTESIAN_POINT('Ctrl Pts',(-2.28401871681013,-6.6322604385465,-1.83169692937167));
#23099=CARTESIAN_POINT('Ctrl Pts',(-1.87862206162202,-6.75814461970629,
-1.81243081495137));
#23100=CARTESIAN_POINT('Ctrl Pts',(-1.67533986993288,-6.81138588901042,
-1.80296694735822));
#23101=CARTESIAN_POINT('Ctrl Pts',(-1.18806296773287,-6.91587015740234,
-1.78059141505088));
#23102=CARTESIAN_POINT('Ctrl Pts',(-0.902695260293384,-6.95887151122777,
-1.76773609250292));
#23103=CARTESIAN_POINT('Ctrl Pts',(-0.50632953486355,-6.9938020064444,-1.74980433031526));
#23104=CARTESIAN_POINT('Ctrl Pts',(-0.39695619116797,-7.00086149172748,
-1.7448451267552));
#23105=CARTESIAN_POINT('Ctrl Pts',(-0.0704598280006472,-7.01425911832889,
-1.72995996183026));
#23106=CARTESIAN_POINT('Ctrl Pts',(0.146836526019976,-7.0130758563541,-1.71996890697031));
#23107=CARTESIAN_POINT('Ctrl Pts',(0.569885949331282,-6.99109961083581,
-1.70048068945671));
#23108=CARTESIAN_POINT('Ctrl Pts',(0.775475263538958,-6.97128991803752,
-1.69099278094508));
#23109=CARTESIAN_POINT('Ctrl Pts',(1.06527357053363,-6.93038628930513,-1.67761158148982));
#23110=CARTESIAN_POINT('Ctrl Pts',(1.15042649250193,-6.91676087008585,-1.67367830779049));
#23111=CARTESIAN_POINT('Ctrl Pts',(1.42088198533952,-6.8683522326076,-1.66117676076989));
#23112=CARTESIAN_POINT('Ctrl Pts',(1.60504366515428,-6.827664634724,-1.652652527281));
#23113=CARTESIAN_POINT('Ctrl Pts',(2.17672919603003,-6.67694812038725,-1.62603700615829));
#23114=CARTESIAN_POINT('Ctrl Pts',(2.55654114230817,-6.54093839122033,-1.60816388687753));
#23115=CARTESIAN_POINT('Ctrl Pts',(3.01940679865851,-6.32867748826894,-1.58511560681427));
#23116=CARTESIAN_POINT('Ctrl Pts',(3.11521786188344,-6.28206917467245,-1.58026433345328));
#23117=CARTESIAN_POINT('Ctrl Pts',(3.45492929911434,-6.1071297303324,-1.56278674522321));
#23118=CARTESIAN_POINT('Ctrl Pts',(3.69227790865397,-5.9666283192268,-1.55007586514755));
#23119=CARTESIAN_POINT('Ctrl Pts',(4.10506250509221,-5.68819143019162,-1.52721245076718));
#23120=CARTESIAN_POINT('Ctrl Pts',(4.28336906056868,-5.55516082737718,-1.51705058499257));
#23121=CARTESIAN_POINT('Ctrl Pts',(4.61560006042116,-5.28176968717741,-1.4975148638704));
#23122=CARTESIAN_POINT('Ctrl Pts',(4.770190878907,-5.14258065267075,-1.48814172755728));
#23123=CARTESIAN_POINT('Ctrl Pts',(5.1281382503437,-4.79024651914989,-1.46558351981212));
#23124=CARTESIAN_POINT('Ctrl Pts',(5.32469539334947,-4.57076365934437,-1.4524621633358));
#23125=CARTESIAN_POINT('Ctrl Pts',(5.57533038512504,-4.25271092174228,-1.43421715648585));
#23126=CARTESIAN_POINT('Ctrl Pts',(5.64171980018662,-4.16423540730412,-1.429213607102));
#23127=CARTESIAN_POINT('Ctrl Pts',(5.81936632704178,-3.91543988374907,-1.4152905826453));
#23128=CARTESIAN_POINT('Ctrl Pts',(5.9260651735649,-3.75199201605711,-1.40632367816575));
#23129=CARTESIAN_POINT('Ctrl Pts',(6.13693332561609,-3.39748833767617,-1.38734957803417));
#23130=CARTESIAN_POINT('Ctrl Pts',(6.23931191876503,-3.20559911688762,-1.37735167651129));
#23131=CARTESIAN_POINT('Ctrl Pts',(6.41306114104572,-2.83996606376113,-1.35883085801239));
#23132=CARTESIAN_POINT('Ctrl Pts',(6.48669087267177,-2.66750886342719,-1.35030100584811));
#23133=CARTESIAN_POINT('Ctrl Pts',(6.64787543344751,-2.24368692236273,-1.32977722671881));
#23134=CARTESIAN_POINT('Ctrl Pts',(6.72820443306059,-1.98988603124351,-1.31785105648502));
#23135=CARTESIAN_POINT('Ctrl Pts',(6.83598640412604,-1.56713457381781,-1.29830478262318));
#23136=CARTESIAN_POINT('Ctrl Pts',(6.87202848356104,-1.40065869672694,-1.29068356264488));
#23137=CARTESIAN_POINT('Ctrl Pts',(6.922376645178,-1.11883289029985,-1.2777962314217));
#23138=CARTESIAN_POINT('Ctrl Pts',(6.93994123689945,-1.00414181979542,-1.27255440448487));
#23139=CARTESIAN_POINT('Ctrl Pts',(6.97569617344906,-0.724451852747487,
-1.25972304350627));
#23140=CARTESIAN_POINT('Ctrl Pts',(6.99088876476121,-0.559142896839073,
-1.252108629037));
#23141=CARTESIAN_POINT('Ctrl Pts',(7.01345372084819,-0.157673539843914,
-1.23362207052769));
#23142=CARTESIAN_POINT('Ctrl Pts',(7.0147853281581,0.0786263206280219,-1.22274933931911));
#23143=CARTESIAN_POINT('Ctrl Pts',(6.99556447043618,0.506633699858591,-1.20313059071173));
#23144=CARTESIAN_POINT('Ctrl Pts',(6.97903946981141,0.698290572471308,-1.19437160873707));
#23145=CARTESIAN_POINT('Ctrl Pts',(6.906028430232,1.26943908542235,-1.16828904011256));
#23146=CARTESIAN_POINT('Ctrl Pts',(6.8262697841316,1.64521970948371,-1.15118534066737));
#23147=CARTESIAN_POINT('Ctrl Pts',(6.69383214117339,2.08717518292637,-1.130484971321));
#23148=CARTESIAN_POINT('Ctrl Pts',(6.67024108955778,2.16138212353261,-1.12698714340597));
#23149=CARTESIAN_POINT('Ctrl Pts',(6.60997288537854,2.34056563741783,-1.11847035518716));
#23150=CARTESIAN_POINT('Ctrl Pts',(6.57202555391534,2.4450907777513,-1.11344109812216));
#23151=CARTESIAN_POINT('Ctrl Pts',(6.45966058649541,2.73305427449377,-1.09936460835701));
#23152=CARTESIAN_POINT('Ctrl Pts',(6.37993814708852,2.9143075243136,-1.0902676665805));
#23153=CARTESIAN_POINT('Ctrl Pts',(6.19717111788147,3.28627105452563,-1.07120305700744));
#23154=CARTESIAN_POINT('Ctrl Pts',(6.09273529955224,3.47607323663455,-1.06124494652088));
#23155=CARTESIAN_POINT('Ctrl Pts',(5.88192895315215,3.82041774221988,-1.04277387146757));
#23156=CARTESIAN_POINT('Ctrl Pts',(5.77781639586997,3.97611860963083,-1.03425424626747));
#23157=CARTESIAN_POINT('Ctrl Pts',(5.51633433584106,4.33517044357127,-1.01415058180392));
#23158=CARTESIAN_POINT('Ctrl Pts',(5.35376855983176,4.53440314263139,-1.00262587369899));
#23159=CARTESIAN_POINT('Ctrl Pts',(5.06243592471743,4.85387882066213,-0.983253652586092));
#23160=CARTESIAN_POINT('Ctrl Pts',(4.93941696602262,4.97901159816298,-0.975404346216908));
#23161=CARTESIAN_POINT('Ctrl Pts',(4.72637753451685,5.18003742826861,-0.962221554904486));
#23162=CARTESIAN_POINT('Ctrl Pts',(4.6389071789761,5.25851426109885,-0.956914085935074));
#23163=CARTESIAN_POINT('Ctrl Pts',(4.44114884533163,5.42716351144375,-0.945088750833864));
#23164=CARTESIAN_POINT('Ctrl Pts',(4.33000280149616,5.51624707609266,-0.938562475106899));
#23165=CARTESIAN_POINT('Ctrl Pts',(4.01632625589052,5.75233377439716,-0.920525766494181));
#23166=CARTESIAN_POINT('Ctrl Pts',(3.80851901656226,5.89197798147266,-0.908999622644175));
#23167=CARTESIAN_POINT('Ctrl Pts',(3.42547694329479,6.12063019898576,-0.888561787861463));
#23168=CARTESIAN_POINT('Ctrl Pts',(3.25312430962182,6.21395126374646,-0.879632547332947));
#23169=CARTESIAN_POINT('Ctrl Pts',(2.85668838537808,6.40758322178479,-0.859638089324845));
#23170=CARTESIAN_POINT('Ctrl Pts',(2.63078947535102,6.50359442553203,-0.848617999075666));
#23171=CARTESIAN_POINT('Ctrl Pts',(2.21532642632959,6.6549772720127,-0.828796816384092));
#23172=CARTESIAN_POINT('Ctrl Pts',(2.02757430087945,6.7145614495574,-0.819993903164605));
#23173=CARTESIAN_POINT('Ctrl Pts',(1.71829410496459,6.79855622026545,-0.805580649543301));
#23174=CARTESIAN_POINT('Ctrl Pts',(1.59818849064993,6.82778840026634,-0.800003364071787));
#23175=CARTESIAN_POINT('Ctrl Pts',(1.34873321047896,6.88155960884435,-0.788400046508771));
#23176=CARTESIAN_POINT('Ctrl Pts',(1.21933840783383,6.90566123529639,-0.782374836239947));
#23177=CARTESIAN_POINT('Ctrl Pts',(0.832617388102664,6.96648502223349,-0.764400539666374));
#23178=CARTESIAN_POINT('Ctrl Pts',(0.573843077236756,6.99255822311188,-0.752423249359184));
#23179=CARTESIAN_POINT('Ctrl Pts',(0.11605306322733,7.01309542224427,-0.731422272237092));
#23180=CARTESIAN_POINT('Ctrl Pts',(-0.0824039055175498,7.01357163845523,
-0.722377798841256));
#23181=CARTESIAN_POINT('Ctrl Pts',(-0.655101838414206,6.99063180179189,
-0.696396248055746));
#23182=CARTESIAN_POINT('Ctrl Pts',(-1.02778326705308,6.94562860512029,-0.679662612450395));
#23183=CARTESIAN_POINT('Ctrl Pts',(-1.56570433335402,6.83641054771974,-0.655050768707296));
#23184=CARTESIAN_POINT('Ctrl Pts',(-1.73497665737009,6.79542446991993,-0.647230708071769));
#23185=CARTESIAN_POINT('Ctrl Pts',(-2.01876329756693,6.71541521806983,-0.633856319975324));
#23186=CARTESIAN_POINT('Ctrl Pts',(-2.13411374301414,6.67965301808382,-0.628340561556277));
#23187=CARTESIAN_POINT('Ctrl Pts',(-2.51340711941884,6.55123215530529,-0.609983091602798));
#23188=CARTESIAN_POINT('Ctrl Pts',(-2.7727283881231,6.44576110261613,-0.597083850232413));
#23189=CARTESIAN_POINT('Ctrl Pts',(-3.20844135660255,6.23737552779624,-0.574937859495651));
#23190=CARTESIAN_POINT('Ctrl Pts',(-3.38792802955432,6.14173387660556,-0.565663596643418));
#23191=CARTESIAN_POINT('Ctrl Pts',(-3.90916097761288,5.83417755729144,-0.538216858581451));
#23192=CARTESIAN_POINT('Ctrl Pts',(-4.23711154293978,5.60054074252687,-0.520292896684572));
#23193=CARTESIAN_POINT('Ctrl Pts',(-4.60289977383775,5.28933610627461,-0.498745982025865));
#23194=CARTESIAN_POINT('Ctrl Pts',(-4.66170747694175,5.23758017311961,-0.495227118306987));
#23195=CARTESIAN_POINT('Ctrl Pts',(-4.80205278176163,5.10982745900633,-0.486677628279994));
#23196=CARTESIAN_POINT('Ctrl Pts',(-4.88266817310611,5.03285195838024,-0.48163682753406));
#23197=CARTESIAN_POINT('Ctrl Pts',(-5.10211786256593,4.81307322170992,-0.467493951432141));
#23198=CARTESIAN_POINT('Ctrl Pts',(-5.23675217016614,4.66623035799095,-0.458341175817069));
#23199=CARTESIAN_POINT('Ctrl Pts',(-5.50411364112357,4.34845753317505,-0.439237595113581));
#23200=CARTESIAN_POINT('Ctrl Pts',(-5.63555286791056,4.17670863639256,-0.429296446644721));
#23201=CARTESIAN_POINT('Ctrl Pts',(-5.86558794953502,3.84545494795492,-0.410846564889966));
#23202=CARTESIAN_POINT('Ctrl Pts',(-5.9661322944301,3.68753478099821,-0.402331288097689));
#23203=CARTESIAN_POINT('Ctrl Pts',(-6.18591950332344,3.30975650239894,-0.382549926611484));
#23204=CARTESIAN_POINT('Ctrl Pts',(-6.2999600098488,3.08716606843899,-0.371336894420973));
#23205=CARTESIAN_POINT('Ctrl Pts',(-6.47511748331437,2.69494806530593,-0.35208947617182));
#23206=CARTESIAN_POINT('Ctrl Pts',(-6.54203221130213,2.52818223171317,-0.344053311846169));
#23207=CARTESIAN_POINT('Ctrl Pts',(-6.64241059628119,2.24724281384611,-0.330628628174148));
#23208=CARTESIAN_POINT('Ctrl Pts',(-6.67950624280283,2.13445890569617,-0.325267530957115));
#23209=CARTESIAN_POINT('Ctrl Pts',(-6.76622730642944,1.84634295529001,-0.311579604140177));
#23210=CARTESIAN_POINT('Ctrl Pts',(-6.81191448793027,1.66992033273699,-0.3032162317978));
#23211=CARTESIAN_POINT('Ctrl Pts',(-6.89944374467669,1.26799910238903,-0.284299975755273));
#23212=CARTESIAN_POINT('Ctrl Pts',(-6.93720115188294,1.04181915943751,-0.273752348830883));
#23213=CARTESIAN_POINT('Ctrl Pts',(-6.97413171097342,0.72595239414745,-0.259194191658068));
#23214=CARTESIAN_POINT('Ctrl Pts',(-6.98277083377061,0.637519914007879,
-0.25513616674583));
#23215=CARTESIAN_POINT('Ctrl Pts',(-7.00407233685088,0.366288335271892,
-0.242740651524406));
#23216=CARTESIAN_POINT('Ctrl Pts',(-7.0112523177922,0.183136087572746,-0.234442732772776));
#23217=CARTESIAN_POINT('Ctrl Pts',(-7.01124871528832,-0.101579106034701,
-0.221607777351206));
#23218=CARTESIAN_POINT('Ctrl Pts',(-7.00904376688205,-0.203057910238692,
-0.21704532616958));
#23219=CARTESIAN_POINT('Ctrl Pts',(-6.99269606217985,-0.579173637994724,
-0.200147900057931));
#23220=CARTESIAN_POINT('Ctrl Pts',(-6.96460424313232,-0.852951423398579,
-0.187881817746726));
#23221=CARTESIAN_POINT('Ctrl Pts',(-6.90275168889596,-1.23365491144146,
-0.170504260987112));
#23222=CARTESIAN_POINT('Ctrl Pts',(-6.88241021161708,-1.34250316286391,
-0.165495514278024));
#23223=CARTESIAN_POINT('Ctrl Pts',(-6.81424568765894,-1.66478500130876,
-0.15049327476538));
#23224=CARTESIAN_POINT('Ctrl Pts',(-6.75900633229958,-1.87650875306416,
-0.140433011724079));
#23225=CARTESIAN_POINT('Ctrl Pts',(-6.65659239076678,-2.2052646011545,-0.124592045835341));
#23226=CARTESIAN_POINT('Ctrl Pts',(-6.61601241605238,-2.32417276872652,
-0.118814850930105));
#23227=CARTESIAN_POINT('Ctrl Pts',(-6.57227163891168,-2.44189927451098,
-0.113051811211838));
#23228=CARTESIAN_POINT('',(-7.01138978795984,7.81656089707349E-5,-0.773534355761736));
#23229=CARTESIAN_POINT('Ctrl Pts',(-6.5722715952584,-2.44189939200198,-0.660303821598748));
#23230=CARTESIAN_POINT('Ctrl Pts',(-6.63754513530709,-2.26621834855315,
-0.668812138672701));
#23231=CARTESIAN_POINT('Ctrl Pts',(-6.69577709547641,-2.08790084462448,
-0.677320455746654));
#23232=CARTESIAN_POINT('Ctrl Pts',(-6.74677372834014,-1.9075300315013,-0.685828772820607));
#23233=CARTESIAN_POINT('Ctrl Pts',(-6.79777217374385,-1.7271528075762,-0.694337392300112));
#23234=CARTESIAN_POINT('Ctrl Pts',(-6.84153469067179,-1.54472242525412,
-0.702846011779617));
#23235=CARTESIAN_POINT('Ctrl Pts',(-6.87791759594143,-1.36083654637111,
-0.711354631259122));
#23236=CARTESIAN_POINT('Ctrl Pts',(-6.9142994945855,-1.17695575515848,-0.719863015326035));
#23237=CARTESIAN_POINT('Ctrl Pts',(-6.94330213173949,-0.991619851606324,
-0.728371399392948));
#23238=CARTESIAN_POINT('Ctrl Pts',(-6.96483300486484,-0.805436389074502,
-0.736879783459861));
#23239=CARTESIAN_POINT('Ctrl Pts',(-6.98636838000213,-0.619213996390389,
-0.745389946592879));
#23240=CARTESIAN_POINT('Ctrl Pts',(-7.00042883457153,-0.432143997917336,
-0.753900109725898));
#23241=CARTESIAN_POINT('Ctrl Pts',(-7.00697367561977,-0.244839685654932,
-0.762410272858916));
#23242=CARTESIAN_POINT('Ctrl Pts',(-7.00982537777381,-0.163227908256182,
-0.766118300350915));
#23243=CARTESIAN_POINT('Ctrl Pts',(-7.01125090971808,-0.0815716875323698,
-0.769826327842913));
#23244=CARTESIAN_POINT('Ctrl Pts',(-7.0112499995644,7.81546515054621E-5,
-0.773534355334912));
#23245=CARTESIAN_POINT('Ctrl Pts',(-7.01176597774635,7.81950970159262E-5,
-0.773534356910375));
#23246=CARTESIAN_POINT('Ctrl Pts',(-7.01181069762049,0.078362201253698,
-0.777089267446053));
#23247=CARTESIAN_POINT('Ctrl Pts',(-6.99150694704885,1.31618785766362,-0.833300520289124));
#23248=CARTESIAN_POINT('Ctrl Pts',(-6.30415497350669,3.69183680131228,-0.942168115439734));
#23249=CARTESIAN_POINT('Ctrl Pts',(-3.78576056174483,6.24820341111258,-1.10013714236197));
#23250=CARTESIAN_POINT('Ctrl Pts',(-0.35395787806857,7.29703657096924,-1.25810616928429));
#23251=CARTESIAN_POINT('Ctrl Pts',(3.16324588907938,6.58527936709808,-1.41607519620657));
#23252=CARTESIAN_POINT('Ctrl Pts',(5.91723842982768,4.28466081062169,-1.57404422312886));
#23253=CARTESIAN_POINT('Ctrl Pts',(7.24355099965782,0.950261970649094,-1.73201325005114));
#23254=CARTESIAN_POINT('Ctrl Pts',(6.82217792133075,-2.6134110482692,-1.88998227697345));
#23255=CARTESIAN_POINT('Ctrl Pts',(4.75478586103601,-5.5465340811355,-2.04795130389573));
#23256=CARTESIAN_POINT('Ctrl Pts',(1.54018423325358,-7.14141872635569,-2.20592033081802));
#23257=CARTESIAN_POINT('Ctrl Pts',(-2.04602489478722,-7.0132596577781,-2.36388935774031));
#23258=CARTESIAN_POINT('Ctrl Pts',(-5.01110659443209,-5.26800938017539,
-2.51534699073651));
#23259=CARTESIAN_POINT('Ctrl Pts',(-6.21784576943405,-3.39432725900993,
-2.61414828142529));
#23260=CARTESIAN_POINT('Ctrl Pts',(-6.5726191009646,-2.44202878202201,-2.66029322980663));
#23261=CARTESIAN_POINT('Origin',(0.,0.,0.));
#23262=CARTESIAN_POINT('',(-6.57227158383948,-2.44189942273553,-4.66062920490781));
#23263=CARTESIAN_POINT('',(-6.57227159525839,-2.44189939200201,-4.11323059144668));
#23264=CARTESIAN_POINT('',(-6.57227159525839,-2.441899392002,0.));
#23265=CARTESIAN_POINT('',(-7.01124999966544,-6.84931509963988E-5,-2.22646564448509));
#23266=CARTESIAN_POINT('Ctrl Pts',(-6.57227159525839,-2.44189939200201,
-4.11323059144668));
#23267=CARTESIAN_POINT('Ctrl Pts',(-6.57127504206402,-2.44458157386175,
-4.11310064298898));
#23268=CARTESIAN_POINT('Ctrl Pts',(-6.57027684974964,-2.447263138134,-4.11297069453128));
#23269=CARTESIAN_POINT('Ctrl Pts',(-6.5692770191055,-2.44994408278074,-4.11284074607358));
#23270=CARTESIAN_POINT('Ctrl Pts',(-6.50362858156447,-2.62597372162417,
-4.10430838785975));
#23271=CARTESIAN_POINT('Ctrl Pts',(-6.43088970711211,-2.79939283689036,
-4.09577602964593));
#23272=CARTESIAN_POINT('Ctrl Pts',(-6.35129333024236,-2.96962953846418,
-4.08724367143211));
#23273=CARTESIAN_POINT('Ctrl Pts',(-6.27171185809064,-3.13983436258157,
-4.07871291093415));
#23274=CARTESIAN_POINT('Ctrl Pts',(-6.1852755756442,-3.30685768517568,-4.07018215043618));
#23275=CARTESIAN_POINT('Ctrl Pts',(-6.09226482886828,-3.47014925002291,
-4.06165138993822));
#23276=CARTESIAN_POINT('Ctrl Pts',(-5.99524674039942,-3.64047618571277,
-4.05275308403931));
#23277=CARTESIAN_POINT('Ctrl Pts',(-5.89107527475381,-3.80674235923873,
-4.0438547781404));
#23278=CARTESIAN_POINT('Ctrl Pts',(-5.78012132077499,-3.96835281692825,
-4.03495647224149));
#23279=CARTESIAN_POINT('Ctrl Pts',(-5.67375361316515,-4.12328315779282,
-4.02642597498441));
#23280=CARTESIAN_POINT('Ctrl Pts',(-5.56115303293323,-4.27393466016442,
-4.01789547772733));
#23281=CARTESIAN_POINT('Ctrl Pts',(-5.44269029911535,-4.41981321668865,
-4.00936498047026));
#23282=CARTESIAN_POINT('Ctrl Pts',(-5.32422635300546,-4.56569326606555,
-4.00083439591608));
#23283=CARTESIAN_POINT('Ctrl Pts',(-5.19990032883057,-4.70680003650741,
-3.9923038113619));
#23284=CARTESIAN_POINT('Ctrl Pts',(-5.07012317901512,-4.84267255883707,
-3.98377322680771));
#23285=CARTESIAN_POINT('Ctrl Pts',(-4.94032034929951,-4.97857196720032,
-3.9752409542479));
#23286=CARTESIAN_POINT('Ctrl Pts',(-4.8050644516411,-5.10923483821213,-3.96670868168809));
#23287=CARTESIAN_POINT('Ctrl Pts',(-4.66480383944429,-5.23423649656813,
-3.95817640912828));
#23288=CARTESIAN_POINT('Ctrl Pts',(-4.64669542280057,-5.25037489832764,
-3.95707484580262));
#23289=CARTESIAN_POINT('Ctrl Pts',(-4.6285036344999,-5.26641899021432,-3.95597328247695));
#23290=CARTESIAN_POINT('Ctrl Pts',(-4.61022948153129,-5.28236790560064,
-3.95487171915129));
#23291=CARTESIAN_POINT('Ctrl Pts',(-4.4686837205656,-5.40590311781067,-3.94633936093745));
#23292=CARTESIAN_POINT('Ctrl Pts',(-4.32214590192658,-5.52376660284747,
-3.9378070027236));
#23293=CARTESIAN_POINT('Ctrl Pts',(-4.17109316649515,-5.63556637428018,
-3.92927464450976));
#23294=CARTESIAN_POINT('Ctrl Pts',(-4.02006871625134,-5.74734521078907,
-3.92074388401179));
#23295=CARTESIAN_POINT('Ctrl Pts',(-3.86453128223555,-5.85306241768264,
-3.91221312351381));
#23296=CARTESIAN_POINT('Ctrl Pts',(-3.70498939617103,-5.95236760766338,
-3.90368236301584));
#23297=CARTESIAN_POINT('Ctrl Pts',(-3.53857369311297,-6.05595133364036,
-3.89478405711694));
#23298=CARTESIAN_POINT('Ctrl Pts',(-3.36780111999451,-6.15255807762932,
-3.88588575121803));
#23299=CARTESIAN_POINT('Ctrl Pts',(-3.19328111137226,-6.24184125929627,
-3.87698744531913));
#23300=CARTESIAN_POINT('Ctrl Pts',(-3.02597483175353,-6.32743394906945,
-3.86845694806207));
#23301=CARTESIAN_POINT('Ctrl Pts',(-2.85522497701526,-6.40629618935039,
-3.859926450805));
#23302=CARTESIAN_POINT('Ctrl Pts',(-2.68159281415117,-6.47816999943602,
-3.85139595354794));
#23303=CARTESIAN_POINT('Ctrl Pts',(-2.50795887441577,-6.550044545045,-3.84286536899371));
#23304=CARTESIAN_POINT('Ctrl Pts',(-2.33144285156541,-6.61493040351321,
-3.83433478443948));
#23305=CARTESIAN_POINT('Ctrl Pts',(-2.15262561350206,-6.67261789184686,
-3.82580419988525));
#23306=CARTESIAN_POINT('Ctrl Pts',(-1.9737729916391,-6.73031679520152,-3.81727192732544));
#23307=CARTESIAN_POINT('Ctrl Pts',(-1.79261853660246,-6.78081439051791,
-3.80873965476564));
#23308=CARTESIAN_POINT('Ctrl Pts',(-1.60975872389551,-6.82395071885358,
-3.80020738220584));
#23309=CARTESIAN_POINT('Ctrl Pts',(-1.58615051611798,-6.82951985614533,
-3.79910581888022));
#23310=CARTESIAN_POINT('Ctrl Pts',(-1.56251390031448,-6.83496636322321,
-3.79800425555461));
#23311=CARTESIAN_POINT('Ctrl Pts',(-1.5388501746405,-6.84028995748783,-3.796902692229));
#23312=CARTESIAN_POINT('Ctrl Pts',(-1.35555850231488,-6.88152482088126,
-3.78837033401517));
#23313=CARTESIAN_POINT('Ctrl Pts',(-1.17057760880854,-6.91539519781984,
-3.77983797580134));
#23314=CARTESIAN_POINT('Ctrl Pts',(-0.984513719362953,-6.94178358196841,
-3.77130561758751));
#23315=CARTESIAN_POINT('Ctrl Pts',(-0.798484671074311,-6.96816702479367,
-3.76277485708957));
#23316=CARTESIAN_POINT('Ctrl Pts',(-0.611373334375636,-6.9870712278236,
-3.75424409659162));
#23317=CARTESIAN_POINT('Ctrl Pts',(-0.423793730905451,-6.99843021227941,
-3.74571333609368));
#23318=CARTESIAN_POINT('Ctrl Pts',(-0.228132313324107,-7.01027859536474,
-3.73681503019477));
#23319=CARTESIAN_POINT('Ctrl Pts',(-0.0319617353477988,-7.01391714592579,
-3.72791672429585));
#23320=CARTESIAN_POINT('Ctrl Pts',(0.164017063898131,-7.00933127803575,
-3.71901841839694));
#23321=CARTESIAN_POINT('Ctrl Pts',(0.351895141860959,-7.00493496553517,
-3.71048792113986));
#23322=CARTESIAN_POINT('Ctrl Pts',(0.539596649861354,-6.9929804797751,-3.70195742388278));
#23323=CARTESIAN_POINT('Ctrl Pts',(0.726505192477673,-6.97350821092246,
-3.6934269266257));
#23324=CARTESIAN_POINT('Ctrl Pts',(0.913415647828903,-6.9540357427997,-3.68489634207148));
#23325=CARTESIAN_POINT('Ctrl Pts',(1.09953281758467,-6.92704537277569,-3.67636575751727));
#23326=CARTESIAN_POINT('Ctrl Pts',(1.28424606709855,-6.89262929524299,-3.66783517296306));
#23327=CARTESIAN_POINT('Ctrl Pts',(1.46899586709716,-6.85820640756366,-3.65930290040324));
#23328=CARTESIAN_POINT('Ctrl Pts',(1.65234089137479,-6.81635493464919,-3.65077062784342));
#23329=CARTESIAN_POINT('Ctrl Pts',(1.83368045678168,-6.76721822796612,-3.6422383552836));
#23330=CARTESIAN_POINT('Ctrl Pts',(1.85709239226987,-6.76087440882006,-3.64113679195797));
#23331=CARTESIAN_POINT('Ctrl Pts',(1.88047091801492,-6.75440922668806,-3.64003522863234));
#23332=CARTESIAN_POINT('Ctrl Pts',(1.90381475790691,-6.74782305118294,-3.63893366530671));
#23333=CARTESIAN_POINT('Ctrl Pts',(2.08462869697889,-6.6968086361591,-3.63040130709289));
#23334=CARTESIAN_POINT('Ctrl Pts',(2.26342145439287,-6.6385138397135,-3.62186894887907));
#23335=CARTESIAN_POINT('Ctrl Pts',(2.43960398736454,-6.57312398691331,-3.61333659066524));
#23336=CARTESIAN_POINT('Ctrl Pts',(2.61575352950025,-6.50774637860677,-3.6048058301673));
#23337=CARTESIAN_POINT('Ctrl Pts',(2.78929353586459,-6.43527647171821,-3.59627506966935));
#23338=CARTESIAN_POINT('Ctrl Pts',(2.95965264279496,-6.35594861499814,-3.5877443091714));
#23339=CARTESIAN_POINT('Ctrl Pts',(3.13735162361824,-6.27320294002925,-3.57884600327249));
#23340=CARTESIAN_POINT('Ctrl Pts',(3.31158920764571,-6.18299540694012,-3.56994769737357));
#23341=CARTESIAN_POINT('Ctrl Pts',(3.48174207006567,-6.08564694342638,-3.56104939147466));
#23342=CARTESIAN_POINT('Ctrl Pts',(3.64486171808,-5.99232234766433,-3.55251889421759));
#23343=CARTESIAN_POINT('Ctrl Pts',(3.80422725291596,-5.89243545091744,-3.54398839696053));
#23344=CARTESIAN_POINT('Ctrl Pts',(3.95931587134899,-5.78631526909691,-3.53545789970347));
#23345=CARTESIAN_POINT('Ctrl Pts',(4.11440607688664,-5.68019400129191,-3.52692731514927));
#23346=CARTESIAN_POINT('Ctrl Pts',(4.26521902786838,-5.56783949640685,-3.51839673059508));
#23347=CARTESIAN_POINT('Ctrl Pts',(4.41126165359899,-5.44962358204556,-3.50986614604088));
#23348=CARTESIAN_POINT('Ctrl Pts',(4.5573331777919,-5.3313842754854,-3.50133387348104));
#23349=CARTESIAN_POINT('Ctrl Pts',(4.69863225422026,-5.20728143622244,-3.49280160092121));
#23350=CARTESIAN_POINT('Ctrl Pts',(4.83469892173909,-5.07772713904901,-3.48426932836137));
#23351=CARTESIAN_POINT('Ctrl Pts',(4.85226587705268,-5.0610009665732,-3.48316776503572));
#23352=CARTESIAN_POINT('Ctrl Pts',(4.86974566578001,-5.04418398015829,-3.48206620171007));
#23353=CARTESIAN_POINT('Ctrl Pts',(4.8871373417498,-5.02727711245111,-3.48096463838442));
#23354=CARTESIAN_POINT('Ctrl Pts',(5.02184771732065,-4.89632190706907,-3.47243228017058));
#23355=CARTESIAN_POINT('Ctrl Pts',(5.15131416840792,-4.75992699719581,-3.46389992195674));
#23356=CARTESIAN_POINT('Ctrl Pts',(5.27510695580997,-4.61853582504946,-3.4553675637429));
#23357=CARTESIAN_POINT('Ctrl Pts',(5.39887656255142,-4.47717112892681,-3.44683680324492));
#23358=CARTESIAN_POINT('Ctrl Pts',(5.51697442431981,-4.33081226770075,-3.43830604274694));
#23359=CARTESIAN_POINT('Ctrl Pts',(5.62900969102896,-4.17993737522491,-3.42977528224896));
#23360=CARTESIAN_POINT('Ctrl Pts',(5.74587196548612,-4.02256208072073,-3.42087697635006));
#23361=CARTESIAN_POINT('Ctrl Pts',(5.85613743345589,-3.86027326013519,-3.41197867045116));
#23362=CARTESIAN_POINT('Ctrl Pts',(5.95941077695181,-3.69364992305045,-3.40308036455226));
#23363=CARTESIAN_POINT('Ctrl Pts',(6.05841534966832,-3.53391390856453,-3.39454986729517));
#23364=CARTESIAN_POINT('Ctrl Pts',(6.15099403854922,-3.37019478261854,-3.38601937003809));
#23365=CARTESIAN_POINT('Ctrl Pts',(6.2368437717621,-3.20303080365024,-3.37748887278101));
#23366=CARTESIAN_POINT('Ctrl Pts',(6.32269438352104,-3.03586511400389,-3.3689582882268));
#23367=CARTESIAN_POINT('Ctrl Pts',(6.40181576510515,-2.86525477455143,-3.3604277036726));
#23368=CARTESIAN_POINT('Ctrl Pts',(6.47395137525816,-2.69176153351164,-3.3518971191184));
#23369=CARTESIAN_POINT('Ctrl Pts',(6.54610125938249,-2.51823396216619,-3.34336484655852));
#23370=CARTESIAN_POINT('Ctrl Pts',(6.61126249463669,-2.34182263278763,-3.33483257399864));
#23371=CARTESIAN_POINT('Ctrl Pts',(6.66922681887129,-2.16310892026914,-3.32630030143876));
#23372=CARTESIAN_POINT('Ctrl Pts',(6.67671033200553,-2.1400359968363,-3.32519873811322));
#23373=CARTESIAN_POINT('Ctrl Pts',(6.68407395280301,-2.11692471961782,-3.32409717478768));
#23374=CARTESIAN_POINT('Ctrl Pts',(6.69131729331829,-2.09377635927041,-3.32299561146213));
#23375=CARTESIAN_POINT('Ctrl Pts',(6.74742189893471,-1.91447654239467,-3.3144632532483));
#23376=CARTESIAN_POINT('Ctrl Pts',(6.79632506358751,-1.73289016106787,-3.30593089503446));
#23377=CARTESIAN_POINT('Ctrl Pts',(6.83786003685788,-1.54961178326768,-3.29739853682063));
#23378=CARTESIAN_POINT('Ctrl Pts',(6.87938723254975,-1.36636772502653,-3.28886777632266));
#23379=CARTESIAN_POINT('Ctrl Pts',(6.91354892267587,-1.1814326008848,-3.28033701582468));
#23380=CARTESIAN_POINT('Ctrl Pts',(6.94022907296669,-0.995412968193562,
-3.27180625532671));
#23381=CARTESIAN_POINT('Ctrl Pts',(6.96805872997944,-0.80137873229134,-3.26290794942781));
#23382=CARTESIAN_POINT('Ctrl Pts',(6.98774781336841,-0.606164811914298,
-3.2540096435289));
#23383=CARTESIAN_POINT('Ctrl Pts',(6.99922439220387,-0.410468598163639,
-3.24511133762999));
#23384=CARTESIAN_POINT('Ctrl Pts',(7.01022659030634,-0.222861425115102,
-3.23658084037295));
#23385=CARTESIAN_POINT('Ctrl Pts',(7.01368153715842,-0.0348113541834391,
-3.2280503431159));
#23386=CARTESIAN_POINT('Ctrl Pts',(7.00957901588756,0.153063981814104,-3.21951984585885));
#23387=CARTESIAN_POINT('Ctrl Pts',(7.0054764526334,0.340941240440978,-3.21098926130463));
#23388=CARTESIAN_POINT('Ctrl Pts',(6.99381627662711,0.528643454725836,-3.20245867675042));
#23389=CARTESIAN_POINT('Ctrl Pts',(6.97464037296792,0.715554491472127,-3.1939280921962));
#23390=CARTESIAN_POINT('Ctrl Pts',(6.9554606748404,0.902502513594548,-3.18539581963638));
#23391=CARTESIAN_POINT('Ctrl Pts',(6.92876231094879,1.08865874120466,-3.17686354707656));
#23392=CARTESIAN_POINT('Ctrl Pts',(6.89463896652825,1.27341277036565,-3.16833127451674));
#23393=CARTESIAN_POINT('Ctrl Pts',(6.89023345504253,1.29726553190831,-3.1672297111911));
#23394=CARTESIAN_POINT('Ctrl Pts',(6.88570425245799,1.32109493328478,-3.16612814786547));
#23395=CARTESIAN_POINT('Ctrl Pts',(6.88105162265645,1.34489967240575,-3.16502658453984));
#23396=CARTESIAN_POINT('Ctrl Pts',(6.84501383601325,1.52928358991725,-3.15649422632601));
#23397=CARTESIAN_POINT('Ctrl Pts',(6.80155461748795,1.71224924167072,-3.14796186811218));
#23398=CARTESIAN_POINT('Ctrl Pts',(6.75081043810302,1.89319438814383,-3.13942950989834));
#23399=CARTESIAN_POINT('Ctrl Pts',(6.70007576075442,2.07410565196526,-3.13089874940032));
#23400=CARTESIAN_POINT('Ctrl Pts',(6.64205892744768,2.25299687105402,-3.1223679889023));
#23401=CARTESIAN_POINT('Ctrl Pts',(6.57694671586432,2.42927941150901,-3.11383722840428));
#23402=CARTESIAN_POINT('Ctrl Pts',(6.50902916307913,2.61315703531129,-3.10493892250538));
#23403=CARTESIAN_POINT('Ctrl Pts',(6.43339138405314,2.79419587395531,-3.09604061660649));
#23404=CARTESIAN_POINT('Ctrl Pts',(6.35030219002736,2.97174841765478,-3.0871423107076));
#23405=CARTESIAN_POINT('Ctrl Pts',(6.27064746138764,3.14196188347907,-3.07861181345052));
#23406=CARTESIAN_POINT('Ctrl Pts',(6.18414507491995,3.30897117355236,-3.07008131619344));
#23407=CARTESIAN_POINT('Ctrl Pts',(6.09108013378454,3.47222829985521,-3.06155081893637));
#23408=CARTESIAN_POINT('Ctrl Pts',(5.99801424026553,3.63548709685601,-3.05302023438212));
#23409=CARTESIAN_POINT('Ctrl Pts',(5.89838581222268,3.79499338913906,-3.04448964982788));
#23410=CARTESIAN_POINT('Ctrl Pts',(5.79252505529564,3.95022531588672,-3.03595906527364));
#23411=CARTESIAN_POINT('Ctrl Pts',(5.68664335097022,4.10548795944676,-3.02742679271377));
#23412=CARTESIAN_POINT('Ctrl Pts',(5.57452702786904,4.25647429593832,-3.0188945201539));
#23413=CARTESIAN_POINT('Ctrl Pts',(5.45654911473421,4.40269216741227,-3.01036224759404));
#23414=CARTESIAN_POINT('Ctrl Pts',(5.44131751712455,4.42156969899809,-3.00926068426854));
#23415=CARTESIAN_POINT('Ctrl Pts',(5.42598827318772,4.44036779268315,-3.00815912094305));
#23416=CARTESIAN_POINT('Ctrl Pts',(5.41056223496481,4.4590854291068,-3.00705755761755));
#23417=CARTESIAN_POINT('Ctrl Pts',(5.2910770624906,4.60406627150271,-2.99852519940372));
#23418=CARTESIAN_POINT('Ctrl Pts',(5.16574107102182,4.74426620958732,-2.98999284118989));
#23419=CARTESIAN_POINT('Ctrl Pts',(5.03496102601622,4.87922063745817,-2.98146048297606));
#23420=CARTESIAN_POINT('Ctrl Pts',(4.90420547006126,5.01414979460965,-2.97292972247809));
#23421=CARTESIAN_POINT('Ctrl Pts',(4.76800810780415,5.14383518209711,-2.96439896198012));
#23422=CARTESIAN_POINT('Ctrl Pts',(4.62681346414701,5.26784811194172,-2.95586820148215));
#23423=CARTESIAN_POINT('Ctrl Pts',(4.47953548924109,5.39720410375976,-2.94696989558324));
#23424=CARTESIAN_POINT('Ctrl Pts',(4.32682033080478,5.52038776784499,-2.93807158968433));
#23425=CARTESIAN_POINT('Ctrl Pts',(4.16921268489638,5.63695770346019,-2.92917328378543));
#23426=CARTESIAN_POINT('Ctrl Pts',(4.01811970086244,5.7487092578929,-2.92064278652837));
#23427=CARTESIAN_POINT('Ctrl Pts',(3.86253081906203,5.85438264950738,-2.91211228927132));
#23428=CARTESIAN_POINT('Ctrl Pts',(3.70295767450657,5.95363175073105,-2.90358179201426));
#23429=CARTESIAN_POINT('Ctrl Pts',(3.54338289695334,6.05288186762413,-2.89505120746004));
#23430=CARTESIAN_POINT('Ctrl Pts',(3.37982403670182,6.14570740390164,-2.88652062290582));
#23431=CARTESIAN_POINT('Ctrl Pts',(3.21281994966298,6.23180668294096,-2.8779900383516));
#23432=CARTESIAN_POINT('Ctrl Pts',(3.0457828163744,6.31792299903804,-2.86945776579182));
#23433=CARTESIAN_POINT('Ctrl Pts',(2.87529936711953,6.39731026024745,-2.86092549323204));
#23434=CARTESIAN_POINT('Ctrl Pts',(2.70193197174684,6.4697132998729,-2.85239322067226));
#23435=CARTESIAN_POINT('Ctrl Pts',(2.67954928726617,6.47906093059604,-2.85129165734659));
#23436=CARTESIAN_POINT('Ctrl Pts',(2.65711856081897,6.48829221204009,-2.85019009402093));
#23437=CARTESIAN_POINT('Ctrl Pts',(2.63464102702961,6.49740665351896,-2.84908853069526));
#23438=CARTESIAN_POINT('Ctrl Pts',(2.46053721875456,6.5680042104681,-2.84055617248142));
#23439=CARTESIAN_POINT('Ctrl Pts',(2.28356485901358,6.6316117358416,-2.83202381426759));
#23440=CARTESIAN_POINT('Ctrl Pts',(2.1043028654829,6.68801435501005,-2.82349145605375));
#23441=CARTESIAN_POINT('Ctrl Pts',(1.92507443942696,6.74440641257837,-2.81496069555571));
#23442=CARTESIAN_POINT('Ctrl Pts',(1.74355752694815,6.79359616454269,-2.80642993505767));
#23443=CARTESIAN_POINT('Ctrl Pts',(1.56034714755351,6.83541830041305,-2.79789917455963));
#23444=CARTESIAN_POINT('Ctrl Pts',(1.36924320083274,6.8790423311668,-2.78900086866074));
#23445=CARTESIAN_POINT('Ctrl Pts',(1.17629696815757,6.91464971818105,-2.78010256276186));
#23446=CARTESIAN_POINT('Ctrl Pts',(0.982197609021416,6.94211166860147,-2.77120425686297));
#23447=CARTESIAN_POINT('Ctrl Pts',(0.796121285109166,6.96843848804298,-2.76267375960589));
#23448=CARTESIAN_POINT('Ctrl Pts',(0.608985569910114,6.98727966455462,-2.75414326234881));
#23449=CARTESIAN_POINT('Ctrl Pts',(0.421405185699195,6.99857444283947,-2.74561276509173));
#23450=CARTESIAN_POINT('Ctrl Pts',(0.233822881879344,7.00986933670975,-2.73708218053757));
#23451=CARTESIAN_POINT('Ctrl Pts',(0.045796205574106,7.01361766287508,-2.72855159598342));
#23452=CARTESIAN_POINT('Ctrl Pts',(-0.142057349336477,7.00981071584672,
-2.72002101142927));
#23453=CARTESIAN_POINT('Ctrl Pts',(-0.329948076126833,7.00600301551147,
-2.71148873886946));
#23454=CARTESIAN_POINT('Ctrl Pts',(-0.517665307197656,6.99463706321847,
-2.70295646630965));
#23455=CARTESIAN_POINT('Ctrl Pts',(-0.704593017214773,6.97575624879426,
-2.69442419374983));
#23456=CARTESIAN_POINT('Ctrl Pts',(-0.728726412913724,6.97331863178405,
-2.69332263042421));
#23457=CARTESIAN_POINT('Ctrl Pts',(-0.752846654907111,6.9707558262547,-2.69222106709859));
#23458=CARTESIAN_POINT('Ctrl Pts',(-0.776952423870934,6.96806798858486,
-2.69111950377297));
#23459=CARTESIAN_POINT('Ctrl Pts',(-0.963668022544028,6.94724885518932,
-2.68258714555912));
#23460=CARTESIAN_POINT('Ctrl Pts',(-1.14957779623874,6.91891708077707,-2.67405478734527));
#23461=CARTESIAN_POINT('Ctrl Pts',(-1.3340703532533,6.88315936580511,-2.66552242913141));
#23462=CARTESIAN_POINT('Ctrl Pts',(-1.51852836334871,6.8474083465986,-2.65699166863345));
#23463=CARTESIAN_POINT('Ctrl Pts',(-1.70156938609551,6.80423422002569,-2.64846090813548));
#23464=CARTESIAN_POINT('Ctrl Pts',(-1.88259147053926,6.75377493832544,-2.63993014763752));
#23465=CARTESIAN_POINT('Ctrl Pts',(-2.0714128402427,6.7011416327585,-2.63103184173861));
#23466=CARTESIAN_POINT('Ctrl Pts',(-2.25803710131995,6.64058158081811,-2.62213353583971));
#23467=CARTESIAN_POINT('Ctrl Pts',(-2.44179690759758,6.57230967199103,-2.61323522994081));
#23468=CARTESIAN_POINT('Ctrl Pts',(-2.61796106077668,6.50685976078319,-2.60470473268375));
#23469=CARTESIAN_POINT('Ctrl Pts',(-2.79149249444014,6.43432282284169,-2.59617423542669));
#23470=CARTESIAN_POINT('Ctrl Pts',(-2.96182171598655,6.35493813386177,-2.58764373816963));
#23471=CARTESIAN_POINT('Ctrl Pts',(-3.13215268060353,6.27555263249561,-2.57911315361541));
#23472=CARTESIAN_POINT('Ctrl Pts',(-3.2992810916516,6.18931937224999,-2.57058256906118));
#23473=CARTESIAN_POINT('Ctrl Pts',(-3.46265980293689,6.09652471918429,-2.56205198450695));
#23474=CARTESIAN_POINT('Ctrl Pts',(-3.62607084309448,6.00371170420065,-2.55351971194713));
#23475=CARTESIAN_POINT('Ctrl Pts',(-3.78573043597567,5.90433485521893,-2.54498743938731));
#23476=CARTESIAN_POINT('Ctrl Pts',(-3.94111753209282,5.79872564972086,-2.53645516682749));
#23477=CARTESIAN_POINT('Ctrl Pts',(-3.96117886102417,5.78509092030885,-2.53535360350189));
#23478=CARTESIAN_POINT('Ctrl Pts',(-3.98116901423432,5.77135236796101,-2.53425204017628));
#23479=CARTESIAN_POINT('Ctrl Pts',(-4.00108690601917,5.75751075839046,-2.53315047685068));
#23480=CARTESIAN_POINT('Ctrl Pts',(-4.15536454364832,5.6502980649691,-2.52461811863684));
#23481=CARTESIAN_POINT('Ctrl Pts',(-4.30535640504065,5.5368627313533,-2.516085760423));
#23482=CARTESIAN_POINT('Ctrl Pts',(-4.45056613782287,5.41757211445907,-2.50755340220916));
#23483=CARTESIAN_POINT('Ctrl Pts',(-4.59574867954287,5.29830383517625,-2.49902264171111));
#23484=CARTESIAN_POINT('Ctrl Pts',(-4.73615064335071,5.17318265482241,-2.49049188121306));
#23485=CARTESIAN_POINT('Ctrl Pts',(-4.87130838238491,5.04261650397951,-2.48196112071501));
#23486=CARTESIAN_POINT('Ctrl Pts',(-5.01228935433964,4.90642494749334,-2.47306281481613));
#23487=CARTESIAN_POINT('Ctrl Pts',(-5.14756392982854,4.76430906541191,-2.46416450891724));
#23488=CARTESIAN_POINT('Ctrl Pts',(-5.27664758975097,4.61677558216503,-2.45526620301836));
#23489=CARTESIAN_POINT('Ctrl Pts',(-5.40039561768075,4.47534034848493,-2.44673570576127));
#23490=CARTESIAN_POINT('Ctrl Pts',(-5.51845402392328,4.32892662456899,-2.43820520850419));
#23491=CARTESIAN_POINT('Ctrl Pts',(-5.63043594971143,4.17801598593126,-2.4296747112471));
#23492=CARTESIAN_POINT('Ctrl Pts',(-5.74241902147132,4.02710380294318,-2.42114412669281));
#23493=CARTESIAN_POINT('Ctrl Pts',(-5.84832530878325,3.87169486092134,-2.41261354213852));
#23494=CARTESIAN_POINT('Ctrl Pts',(-5.94781002567736,3.71230150458605,-2.40408295758424));
#23495=CARTESIAN_POINT('Ctrl Pts',(-6.04731442829802,3.55287660798887,-2.39555068502439));
#23496=CARTESIAN_POINT('Ctrl Pts',(-6.14039456142936,3.3894659824808,-2.38701841246455));
#23497=CARTESIAN_POINT('Ctrl Pts',(-6.22675006749305,3.22260921606627,-2.37848613990471));
#23498=CARTESIAN_POINT('Ctrl Pts',(-6.23789903838709,3.20106708960527,-2.37738457657927));
#23499=CARTESIAN_POINT('Ctrl Pts',(-6.24893598444566,3.1794675556402,-2.37628301325383));
#23500=CARTESIAN_POINT('Ctrl Pts',(-6.25986031553744,3.1578118044715,-2.37518144992838));
#23501=CARTESIAN_POINT('Ctrl Pts',(-6.34428116655006,2.99046087674696,-2.3666688085047));
#23502=CARTESIAN_POINT('Ctrl Pts',(-6.42200273866975,2.81969184675183,-2.35815616708101));
#23503=CARTESIAN_POINT('Ctrl Pts',(-6.49276411959083,2.64606134657796,-2.34964352565732));
#23504=CARTESIAN_POINT('Ctrl Pts',(-6.56351169396974,2.47246472416044,-2.34113254516988));
#23505=CARTESIAN_POINT('Ctrl Pts',(-6.62730167060251,2.296008031561,-2.33262156468244));
#23506=CARTESIAN_POINT('Ctrl Pts',(-6.68392119685633,2.11726805027485,-2.324110584195));
#23507=CARTESIAN_POINT('Ctrl Pts',(-6.74054189011732,1.93852438490915,-2.31559942828442));
#23508=CARTESIAN_POINT('Ctrl Pts',(-6.78999174023709,1.75749762994793,-2.30708827237384));
#23509=CARTESIAN_POINT('Ctrl Pts',(-6.83210744490193,1.57478075420538,-2.29857711646326));
#23510=CARTESIAN_POINT('Ctrl Pts',(-6.87422073043193,1.39207437375816,-2.29006644943524));
#23511=CARTESIAN_POINT('Ctrl Pts',(-6.90900064431342,1.20767836785345,-2.28155578240723));
#23512=CARTESIAN_POINT('Ctrl Pts',(-6.9363347135591,1.02219729209926,-2.27304511537921));
#23513=CARTESIAN_POINT('Ctrl Pts',(-6.96367525103699,0.836672324794936,
-2.26453243441869));
#23514=CARTESIAN_POINT('Ctrl Pts',(-6.98356637669238,0.650062080119472,
-2.25601975345816));
#23515=CARTESIAN_POINT('Ctrl Pts',(-6.99594720559743,0.462978680927659,
-2.24750707249764));
#23516=CARTESIAN_POINT('Ctrl Pts',(-7.00614807812903,0.30883602032161,-2.24049326316012));
#23517=CARTESIAN_POINT('Ctrl Pts',(-7.01125150840371,0.154372366967734,
-2.2334794538226));
#23518=CARTESIAN_POINT('Ctrl Pts',(-7.01124999966544,-6.84931509963988E-5,
-2.22646564448509));
#23519=CARTESIAN_POINT('Ctrl Pts',(-7.01124999951636,-8.23516846733779E-5,
-2.22677279634694));
#23520=CARTESIAN_POINT('Ctrl Pts',(-7.01124880883069,-0.101454836867331,
-2.22219948827291));
#23521=CARTESIAN_POINT('Ctrl Pts',(-7.00904910995193,-0.202813406512794,
-2.21760633059935));
#23522=CARTESIAN_POINT('Ctrl Pts',(-6.99729784000022,-0.473502170309707,
-2.20525735769209));
#23523=CARTESIAN_POINT('Ctrl Pts',(-6.98379961971893,-0.642591040978516,
-2.19746942105447));
#23524=CARTESIAN_POINT('Ctrl Pts',(-6.93583102485646,-1.054493625703,-2.17839760819467));
#23525=CARTESIAN_POINT('Ctrl Pts',(-6.89472871351082,-1.29631268506705,
-2.16711896464435));
#23526=CARTESIAN_POINT('Ctrl Pts',(-6.8029333810765,-1.70528906870794,-2.14795172209859));
#23527=CARTESIAN_POINT('Ctrl Pts',(-6.75851063828571,-1.87361912106811,
-2.14003340177884));
#23528=CARTESIAN_POINT('Ctrl Pts',(-6.66672192903047,-2.17541791283756,
-2.12575233329747));
#23529=CARTESIAN_POINT('Ctrl Pts',(-6.62149981133014,-2.3094036699173,-2.1193806486438));
#23530=CARTESIAN_POINT('Ctrl Pts',(-6.57227163721606,-2.44189927907466,
-2.11302806574593));
#23531=CARTESIAN_POINT('',(-7.01074934648484,9.37578675265012E-5,-2.77353775949927));
#23532=CARTESIAN_POINT('Ctrl Pts',(-6.5726191009646,-2.44202878202201,-2.66029322980663));
#23533=CARTESIAN_POINT('Ctrl Pts',(-6.62268024518726,-2.30765241502215,
-2.66680462373271));
#23534=CARTESIAN_POINT('Ctrl Pts',(-6.88878358359034,-1.51975160196419,
-2.70455166610063));
#23535=CARTESIAN_POINT('Ctrl Pts',(-7.01041463086307,-0.688046937181739,
-2.74229870846854));
#23536=CARTESIAN_POINT('Ctrl Pts',(-7.01074344146299,9.39112607581394E-5,
-2.77353435691037));
#23537=CARTESIAN_POINT('Ctrl Pts',(-7.01124999953497,8.07525321924046E-5,
-2.77382624556319));
#23538=CARTESIAN_POINT('Ctrl Pts',(-7.01124590840154,0.355288923246704,
-2.78984771974093));
#23539=CARTESIAN_POINT('Ctrl Pts',(-6.98424833394108,0.709982097587371,
-2.80566510602609));
#23540=CARTESIAN_POINT('Ctrl Pts',(-6.91597066131533,1.15593282800845,-2.82595038395769));
#23541=CARTESIAN_POINT('Ctrl Pts',(-6.89950613365193,1.25045820016344,-2.83027522025353));
#23542=CARTESIAN_POINT('Ctrl Pts',(-6.86186625834546,1.44308137055211,-2.83916825388826));
#23543=CARTESIAN_POINT('Ctrl Pts',(-6.8405143033683,1.54112161527904,-2.84374089258977));
#23544=CARTESIAN_POINT('Ctrl Pts',(-6.7310378686837,1.99655729969631,-2.86517247507147));
#23545=CARTESIAN_POINT('Ctrl Pts',(-6.61695979443096,2.34711706640564,-2.88217334921628));
#23546=CARTESIAN_POINT('Ctrl Pts',(-6.40928460343441,2.84761270848719,-2.90695326912895));
#23547=CARTESIAN_POINT('Ctrl Pts',(-6.33673573359343,3.00559624128286,-2.91486072610223));
#23548=CARTESIAN_POINT('Ctrl Pts',(-6.12058121892723,3.43359319367885,-2.93656920662926));
#23549=CARTESIAN_POINT('Ctrl Pts',(-5.96507201325998,3.69716048636172,-2.9502531876902));
#23550=CARTESIAN_POINT('Ctrl Pts',(-5.7085545283741,4.07338018707437,-2.97065443723908));
#23551=CARTESIAN_POINT('Ctrl Pts',(-5.62031524539495,4.19429099361423,-2.97736005047625));
#23552=CARTESIAN_POINT('Ctrl Pts',(-5.47329443792854,4.38276916253252,-2.98813117667118));
#23553=CARTESIAN_POINT('Ctrl Pts',(-5.41697090112093,4.45219536837568,-2.99217187593043));
#23554=CARTESIAN_POINT('Ctrl Pts',(-5.26723793930212,4.62971217807466,-3.00272606466486));
#23555=CARTESIAN_POINT('Ctrl Pts',(-5.17182587978082,4.7360581267113,-3.00926771045137));
#23556=CARTESIAN_POINT('Ctrl Pts',(-4.89653443268444,5.02465044725512,-3.02758473970247));
#23557=CARTESIAN_POINT('Ctrl Pts',(-4.70982173006713,5.20007134358355,-3.03938128910531));
#23558=CARTESIAN_POINT('Ctrl Pts',(-4.36289807132683,5.49196762218392,-3.06015693190967));
#23559=CARTESIAN_POINT('Ctrl Pts',(-4.20656074624372,5.6126140457021,-3.06915550734746));
#23560=CARTESIAN_POINT('Ctrl Pts',(-3.84119904084998,5.8707143072342,-3.08943122255127));
#23561=CARTESIAN_POINT('Ctrl Pts',(-3.62949137987601,6.00390634861941,-3.10065985685495));
#23562=CARTESIAN_POINT('Ctrl Pts',(-3.24022587235689,6.2206772305833,-3.12063134823794));
#23563=CARTESIAN_POINT('Ctrl Pts',(-3.06542261854953,6.30865060212891,-3.12937715772036));
#23564=CARTESIAN_POINT('Ctrl Pts',(-2.77487028879792,6.43994628684181,-3.14371708307237));
#23565=CARTESIAN_POINT('Ctrl Pts',(-2.66125173902792,6.48772318041217,-3.14927856377225));
#23566=CARTESIAN_POINT('Ctrl Pts',(-2.42324549258326,6.58050068012467,-3.16089431094035));
#23567=CARTESIAN_POINT('Ctrl Pts',(-2.29872442284727,6.62502628419134,-3.16694829616124));
#23568=CARTESIAN_POINT('Ctrl Pts',(-1.92645407201859,6.74638100654683,-3.18492674927493));
#23569=CARTESIAN_POINT('Ctrl Pts',(-1.67561647432196,6.81301640353276,-3.19687864983173));
#23570=CARTESIAN_POINT('Ctrl Pts',(-1.22755398574876,6.90579702552752,-3.21784800100911));
#23571=CARTESIAN_POINT('Ctrl Pts',(-1.03182343738932,6.93774196356555,-3.22688605427261));
#23572=CARTESIAN_POINT('Ctrl Pts',(-0.604916001749064,6.98894868852491,
-3.2463764626622));
#23573=CARTESIAN_POINT('Ctrl Pts',(-0.373602768797742,7.00512314699171,
-3.25679624392579));
#23574=CARTESIAN_POINT('Ctrl Pts',(0.0669087924883373,7.01404117675433,
-3.27655401677683));
#23575=CARTESIAN_POINT('Ctrl Pts',(0.275812978775597,7.00893550892242,-3.2858884782659));
#23576=CARTESIAN_POINT('Ctrl Pts',(0.610720721519649,6.98575243248526,-3.30098156573496));
#23577=CARTESIAN_POINT('Ctrl Pts',(0.737003415781903,6.97356023232605,-3.30670325664519));
#23578=CARTESIAN_POINT('Ctrl Pts',(1.01995213739006,6.93847056754246,-3.31966396866203));
#23579=CARTESIAN_POINT('Ctrl Pts',(1.17631346404718,6.91367932067892,-3.32691880099318));
#23580=CARTESIAN_POINT('Ctrl Pts',(1.57308583746265,6.83692003012535,-3.34548993018733));
#23581=CARTESIAN_POINT('Ctrl Pts',(1.81185013991261,6.77755670113293,-3.3568147244724));
#23582=CARTESIAN_POINT('Ctrl Pts',(2.23331267827011,6.64890120151752,-3.37700054401989));
#23583=CARTESIAN_POINT('Ctrl Pts',(2.417173939016,6.58428770560722,-3.38587769400206));
#23584=CARTESIAN_POINT('Ctrl Pts',(2.82317849638355,6.42230565229147,-3.40568503922625));
#23585=CARTESIAN_POINT('Ctrl Pts',(3.0434445300554,6.32090139619768,-3.41657212340553));
#23586=CARTESIAN_POINT('Ctrl Pts',(3.43282994590629,6.11655782431705,-3.43628437358597));
#23587=CARTESIAN_POINT('Ctrl Pts',(3.60368684859317,6.01747800099115,-3.44511064157775));
#23588=CARTESIAN_POINT('Ctrl Pts',(3.87445847834976,5.84478475332479,-3.45955387390316));
#23589=CARTESIAN_POINT('Ctrl Pts',(3.97700284751861,5.77549870053841,-3.46513761179685));
#23590=CARTESIAN_POINT('Ctrl Pts',(4.18458889671162,5.62708810785398,-3.47674063443582));
#23591=CARTESIAN_POINT('Ctrl Pts',(4.28934664858187,5.54764900331619,-3.48275894099708));
#23592=CARTESIAN_POINT('Ctrl Pts',(4.59451236575126,5.30242438790547,-3.5007335426723));
#23593=CARTESIAN_POINT('Ctrl Pts',(4.78799873685138,5.12838351370287,-3.51271826026345));
#23594=CARTESIAN_POINT('Ctrl Pts',(5.1112759687563,4.80331652796788,-3.53372849666487));
#23595=CARTESIAN_POINT('Ctrl Pts',(5.24514957391362,4.65675847143009,-3.54277485582992));
#23596=CARTESIAN_POINT('Ctrl Pts',(5.613603857019,4.21731528101331,-3.5687707326019));
#23597=CARTESIAN_POINT('Ctrl Pts',(5.83113005358908,3.911038544606,-3.58551637652729));
#23598=CARTESIAN_POINT('Ctrl Pts',(6.11214632647117,3.43941097107539,-3.61013305077131));
#23599=CARTESIAN_POINT('Ctrl Pts',(6.19558667963229,3.28672857628575,-3.61794562952778));
#23600=CARTESIAN_POINT('Ctrl Pts',(6.32720452154977,3.02302822755733,-3.63131428558462));
#23601=CARTESIAN_POINT('Ctrl Pts',(6.37834442382916,2.91357825372106,-3.63683195242053));
#23602=CARTESIAN_POINT('Ctrl Pts',(6.53842567600284,2.54653112494688,-3.65518917141804));
#23603=CARTESIAN_POINT('Ctrl Pts',(6.63478458503777,2.28373934758444,-3.66808616614431));
#23604=CARTESIAN_POINT('Ctrl Pts',(6.77363529379773,1.8212109716682,-3.69022936149848));
#23605=CARTESIAN_POINT('Ctrl Pts',(6.82358617795048,1.62407453630684,-3.69950305917718));
#23606=CARTESIAN_POINT('Ctrl Pts',(6.9465810154549,1.03156856503938,-3.72694663545437));
#23607=CARTESIAN_POINT('Ctrl Pts',(6.99428024190498,0.631798167362091,-3.74486810024395));
#23608=CARTESIAN_POINT('Ctrl Pts',(7.01004353802653,0.151838302369994,-3.76641314522748));
#23609=CARTESIAN_POINT('Ctrl Pts',(7.01130258281483,0.0734932960740408,
-3.76993271995863));
#23610=CARTESIAN_POINT('Ctrl Pts',(7.01117112255727,-0.116314552547843,
-3.77848332036554));
#23611=CARTESIAN_POINT('Ctrl Pts',(7.00843618512526,-0.227753304968802,
-3.78352451643272));
#23612=CARTESIAN_POINT('Ctrl Pts',(6.99425056386765,-0.520729752687469,
-3.79688132570966));
#23613=CARTESIAN_POINT('Ctrl Pts',(6.97839108675056,-0.701966537763913,
-3.80523424939673));
#23614=CARTESIAN_POINT('Ctrl Pts',(6.92723979238907,-1.10517522002605,-3.82392767453972));
#23615=CARTESIAN_POINT('Ctrl Pts',(6.88828713330589,-1.32648597921271,-3.83426151654963));
#23616=CARTESIAN_POINT('Ctrl Pts',(6.79705512902356,-1.73017226468217,-3.85320338147652));
#23617=CARTESIAN_POINT('Ctrl Pts',(6.74787020651669,-1.91303522731362,-3.8618206509253));
#23618=CARTESIAN_POINT('Ctrl Pts',(6.60002304218254,-2.38554959743193,-3.88423786293243));
#23619=CARTESIAN_POINT('Ctrl Pts',(6.48970196677333,-2.67112758261271,-3.89792798567451));
#23620=CARTESIAN_POINT('Ctrl Pts',(6.27058880968273,-3.14382724641097,-3.92127111415586));
#23621=CARTESIAN_POINT('Ctrl Pts',(6.17115064055129,-3.33479102023564,-3.93091041485874));
#23622=CARTESIAN_POINT('Ctrl Pts',(6.00518975336127,-3.62058231883819,-3.94588798894772));
#23623=CARTESIAN_POINT('Ctrl Pts',(5.94484009525226,-3.71884332088699,-3.95114871237711));
#23624=CARTESIAN_POINT('Ctrl Pts',(5.72524171716036,-4.05737695954606,-3.96963228348334));
#23625=CARTESIAN_POINT('Ctrl Pts',(5.55362604195964,-4.28928186450089,-3.98292821331062));
#23626=CARTESIAN_POINT('Ctrl Pts',(5.23607603510089,-4.66726260484389,-4.00556885570729));
#23627=CARTESIAN_POINT('Ctrl Pts',(5.09707575743117,-4.8186775336576,-4.01494398407426));
#23628=CARTESIAN_POINT('Ctrl Pts',(4.66061568935461,-5.25406965953527,-4.04290743849807));
#23629=CARTESIAN_POINT('Ctrl Pts',(4.3446403335694,-5.51821441551957,-4.06123111974664));
#23630=CARTESIAN_POINT('Ctrl Pts',(3.88101915321531,-5.8411487479271,-4.08658577877555));
#23631=CARTESIAN_POINT('Ctrl Pts',(3.75182812168114,-5.92495679019439,-4.09351132361659));
#23632=CARTESIAN_POINT('Ctrl Pts',(3.50762965018205,-6.07218023984643,-4.10645361136492));
#23633=CARTESIAN_POINT('Ctrl Pts',(3.39339663625125,-6.13674970732486,-4.11245308486267));
#23634=CARTESIAN_POINT('Ctrl Pts',(3.03898543253231,-6.3241554297724,-4.13084726117303));
#23635=CARTESIAN_POINT('Ctrl Pts',(2.79347267554831,-6.4363720950731,-4.14328214501769));
#23636=CARTESIAN_POINT('Ctrl Pts',(2.35495418029332,-6.60697696924434,-4.16485208389484));
#23637=CARTESIAN_POINT('Ctrl Pts',(2.16475852466024,-6.67171464216146,-4.17401121538921));
#23638=CARTESIAN_POINT('Ctrl Pts',(1.58879316350656,-6.84053089277647,-4.20122486106248));
#23639=CARTESIAN_POINT('Ctrl Pts',(1.19664427648142,-6.91991130224887,-4.21903446986866));
#23640=CARTESIAN_POINT('Ctrl Pts',(0.722474742964915,-6.97436207109186,
-4.24044874187128));
#23641=CARTESIAN_POINT('Ctrl Pts',(0.644934006514725,-6.98195932946982,
-4.24394859196465));
#23642=CARTESIAN_POINT('Ctrl Pts',(0.456435757829557,-6.99726096939189,
-4.25246852491921));
#23643=CARTESIAN_POINT('Ctrl Pts',(0.345392108645162,-7.00362040021651,
-4.25749889277586));
#23644=CARTESIAN_POINT('Ctrl Pts',(0.0363132898915868,-7.01395237971942,
-4.27158177342206));
#23645=CARTESIAN_POINT('Ctrl Pts',(-0.161806438995436,-7.01217967974589,
-4.28068409025098));
#23646=CARTESIAN_POINT('Ctrl Pts',(-0.575782563090936,-6.99092029973489,
-4.29975245772036));
#23647=CARTESIAN_POINT('Ctrl Pts',(-0.791353721284571,-6.96981009452171,
-4.30970894112332));
#23648=CARTESIAN_POINT('Ctrl Pts',(-1.19088429473961,-6.91190793591781,
-4.32817799076764));
#23649=CARTESIAN_POINT('Ctrl Pts',(-1.37501749591971,-6.8776453216945,-4.33669720632862));
#23650=CARTESIAN_POINT('Ctrl Pts',(-1.79533658134681,-6.78187774416473,
-4.35620866809789));
#23651=CARTESIAN_POINT('Ctrl Pts',(-2.03012599702565,-6.71533243912823,
-4.36715313937824));
#23652=CARTESIAN_POINT('Ctrl Pts',(-2.43481472181455,-6.57746399831273,
-4.38631128582253));
#23653=CARTESIAN_POINT('Ctrl Pts',(-2.60626245536179,-6.51143231088565,
-4.39452635026103));
#23654=CARTESIAN_POINT('Ctrl Pts',(-2.88499622565634,-6.39130589228717,
-4.40818236147793));
#23655=CARTESIAN_POINT('Ctrl Pts',(-2.99383735568591,-6.3410513144667,-4.41359454885594));
#23656=CARTESIAN_POINT('Ctrl Pts',(-3.43256220124429,-6.12466663274223,
-4.435845953407));
#23657=CARTESIAN_POINT('Ctrl Pts',(-3.75036053482541,-5.93538707445485,
-4.45291872314849));
#23658=CARTESIAN_POINT('Ctrl Pts',(-4.21994097535676,-5.60287325244001,
-4.47930874630594));
#23659=CARTESIAN_POINT('Ctrl Pts',(-4.38278519575835,-5.47643008206499,
-4.48871313522633));
#23660=CARTESIAN_POINT('Ctrl Pts',(-4.71158148882153,-5.19705921583717,
-4.50828449058583));
#23661=CARTESIAN_POINT('Ctrl Pts',(-4.87620253288263,-5.04292332122871,
-4.51842816277566));
#23662=CARTESIAN_POINT('Ctrl Pts',(-5.2269186453325,-4.68128650424208,-4.54102913560914));
#23663=CARTESIAN_POINT('Ctrl Pts',(-5.40864681169705,-4.4700848913034,-4.55344650508219));
#23664=CARTESIAN_POINT('Ctrl Pts',(-5.60648153205455,-4.21038060508412,
-4.56817596372438));
#23665=CARTESIAN_POINT('Ctrl Pts',(-5.63523327615461,-4.17182045272179,
-4.57035015071541));
#23666=CARTESIAN_POINT('Ctrl Pts',(-5.73152086507164,-4.03987337155385,
-4.57775287863013));
#23667=CARTESIAN_POINT('Ctrl Pts',(-5.79714901358844,-3.94511985899341,
-4.58301117054901));
#23668=CARTESIAN_POINT('Ctrl Pts',(-6.01867157118361,-3.60781592309585,
-4.60149561129016));
#23669=CARTESIAN_POINT('Ctrl Pts',(-6.16191836365588,-3.35730634733075,
-4.61479498720285));
#23670=CARTESIAN_POINT('Ctrl Pts',(-6.38014051035421,-2.91438625547387,
-4.63743992604504));
#23671=CARTESIAN_POINT('Ctrl Pts',(-6.46280109794801,-2.72617756743884,
-4.64681593004686));
#23672=CARTESIAN_POINT('Ctrl Pts',(-6.54902910051275,-2.5037846095666,-4.65763515361273));
#23673=CARTESIAN_POINT('Ctrl Pts',(-6.56076062700498,-2.47288068830357,
-4.6591330043543));
#23674=CARTESIAN_POINT('Ctrl Pts',(-6.57227158383948,-2.44189942273553,
-4.6606292049078));
#23675=CARTESIAN_POINT('Origin',(0.,0.,0.));
#23676=CARTESIAN_POINT('',(-6.5722714983487,-2.44189965283043,-6.66023848729892));
#23677=CARTESIAN_POINT('',(-6.57227174271038,-2.44189899514102,-6.11302261786463));
#23678=CARTESIAN_POINT('',(-6.57227159525839,-2.441899392002,0.));
#23679=CARTESIAN_POINT('',(-7.0112499978881,0.00017208778304258,-4.22646564308965));
#23680=CARTESIAN_POINT('Ctrl Pts',(-6.57227174271038,-2.44189899514102,
-6.11302261786463));
#23681=CARTESIAN_POINT('Ctrl Pts',(-6.51134619784151,-2.60587761905121,
-6.105001908522));
#23682=CARTESIAN_POINT('Ctrl Pts',(-6.44427743276589,-2.76759301087802,
-6.09701124066779));
#23683=CARTESIAN_POINT('Ctrl Pts',(-6.28674107852913,-3.11053720106985,
-6.07986803322655));
#23684=CARTESIAN_POINT('Ctrl Pts',(-6.19437377980903,-3.29063676100689,
-6.07074150759056));
#23685=CARTESIAN_POINT('Ctrl Pts',(-5.95799008587052,-3.70621667689436,
-6.04925757833389));
#23686=CARTESIAN_POINT('Ctrl Pts',(-5.80760812360777,-3.93768648618198,
-6.03695396159107));
#23687=CARTESIAN_POINT('Ctrl Pts',(-5.56958851842973,-4.26063780837813,
-6.01891451978956));
#23688=CARTESIAN_POINT('Ctrl Pts',(-5.49249818474332,-4.35956580711916,
-6.01325719512312));
#23689=CARTESIAN_POINT('Ctrl Pts',(-5.30648224427145,-4.58550440909404,
-5.99995194459492));
#23690=CARTESIAN_POINT('Ctrl Pts',(-5.1955815240398,-4.71078931039558,-5.99228093501358));
#23691=CARTESIAN_POINT('Ctrl Pts',(-4.81412592909629,-5.11184836173482,
-5.96683880431027));
#23692=CARTESIAN_POINT('Ctrl Pts',(-4.5252675167531,-5.36924260197459,-5.94907212635811));
#23693=CARTESIAN_POINT('Ctrl Pts',(-4.05674090527729,-5.72193647333492,
-5.92242814067287));
#23694=CARTESIAN_POINT('Ctrl Pts',(-3.89171492337875,-5.83543147044556,
-5.91339449686395));
#23695=CARTESIAN_POINT('Ctrl Pts',(-3.49561843034168,-6.08355763852672,
-5.89238727747053));
#23696=CARTESIAN_POINT('Ctrl Pts',(-3.26125702234848,-6.21234447314634,
-5.88046267125955));
#23697=CARTESIAN_POINT('Ctrl Pts',(-2.89939337099132,-6.38506380215797,
-5.86244632528071));
#23698=CARTESIAN_POINT('Ctrl Pts',(-2.77704432500597,-6.4392193469182,-5.85641724528001));
#23699=CARTESIAN_POINT('Ctrl Pts',(-2.51462695486597,-6.54650266054002,
-5.84353642877551));
#23700=CARTESIAN_POINT('Ctrl Pts',(-2.37425336995916,-6.59870940216665,
-5.83667800574024));
#23701=CARTESIAN_POINT('Ctrl Pts',(-1.83443645159856,-6.7800175360291,-5.81052087636864));
#23702=CARTESIAN_POINT('Ctrl Pts',(-1.4253481344753,-6.87765879366356,-5.79119796203726));
#23703=CARTESIAN_POINT('Ctrl Pts',(-0.804366687127787,-6.96805541337416,
-5.76270493355499));
#23704=CARTESIAN_POINT('Ctrl Pts',(-0.597516053346675,-6.98883240744239,
-5.75333740374891));
#23705=CARTESIAN_POINT('Ctrl Pts',(-0.0324883748679699,-7.0203145014224,
-5.72792049107774));
#23706=CARTESIAN_POINT('Ctrl Pts',(0.326064777081194,-7.01281295085359,
-5.71199564948401));
#23707=CARTESIAN_POINT('Ctrl Pts',(0.795427355416544,-6.96690778708516,
-5.69062793359969));
#23708=CARTESIAN_POINT('Ctrl Pts',(0.908101270318745,-6.95311872462858,
-5.68545118332169));
#23709=CARTESIAN_POINT('Ctrl Pts',(1.18023373432557,-6.91308745378104,-5.67285514064947));
#23710=CARTESIAN_POINT('Ctrl Pts',(1.33921736221832,-6.88405594359876,-5.66542121935758));
#23711=CARTESIAN_POINT('Ctrl Pts',(1.7730509725222,-6.78923628398118,-5.64499243357249));
#23712=CARTESIAN_POINT('Ctrl Pts',(2.0451523321977,-6.71228688025453,-5.63202805724349));
#23713=CARTESIAN_POINT('Ctrl Pts',(2.48942172737593,-6.55711645661793,-5.61061408389849));
#23714=CARTESIAN_POINT('Ctrl Pts',(2.66440775694261,-6.48798347592862,-5.60210950660562));
#23715=CARTESIAN_POINT('Ctrl Pts',(3.03746506549949,-6.32295570218357,-5.58374371965392));
#23716=CARTESIAN_POINT('Ctrl Pts',(3.23423170374685,-6.22460511456047,-5.57390738015286));
#23717=CARTESIAN_POINT('Ctrl Pts',(3.58928652142074,-6.02574911621908,-5.55567139031329));
#23718=CARTESIAN_POINT('Ctrl Pts',(3.7487942857898,-5.92783012312946,-5.54728236116348));
#23719=CARTESIAN_POINT('Ctrl Pts',(3.99483419768763,-5.7628842387067,-5.5338715206011));
#23720=CARTESIAN_POINT('Ctrl Pts',(4.08404295284515,-5.70001117422567,-5.5288998898695));
#23721=CARTESIAN_POINT('Ctrl Pts',(4.23125463770712,-5.59102788116846,-5.52051892836126));
#23722=CARTESIAN_POINT('Ctrl Pts',(4.29006077082934,-5.54603345388105,-5.51712243361233));
#23723=CARTESIAN_POINT('Ctrl Pts',(4.67617982355893,-5.24078520970028,-5.49451277806392));
#23724=CARTESIAN_POINT('Ctrl Pts',(4.98036689096504,-4.95262008893787,-5.47526240477633));
#23725=CARTESIAN_POINT('Ctrl Pts',(5.39424980759214,-4.48360195891624,-5.44685950732038));
#23726=CARTESIAN_POINT('Ctrl Pts',(5.52447759238921,-4.32212525020034,-5.43751154359048));
#23727=CARTESIAN_POINT('Ctrl Pts',(5.8607718425196,-3.86505605412114,-5.41202401306825));
#23728=CARTESIAN_POINT('Ctrl Pts',(6.05151775956992,-3.55899284298793,-5.39601181822503));
#23729=CARTESIAN_POINT('Ctrl Pts',(6.27069321898006,-3.1383251110126,-5.37451772065111));
#23730=CARTESIAN_POINT('Ctrl Pts',(6.32099542095487,-3.03573614658974,-5.36930627359539));
#23731=CARTESIAN_POINT('Ctrl Pts',(6.43741146221111,-2.78285913337723,-5.35655646586825));
#23732=CARTESIAN_POINT('Ctrl Pts',(6.50079729942602,-2.63138847996865,-5.34900287562634));
#23733=CARTESIAN_POINT('Ctrl Pts',(6.65686626467081,-2.21827505774401,-5.32868784701643));
#23734=CARTESIAN_POINT('Ctrl Pts',(6.73943138833716,-1.95312089102667,-5.31595676936915));
#23735=CARTESIAN_POINT('Ctrl Pts',(6.85117915692958,-1.50141863815789,-5.29478165095512));
#23736=CARTESIAN_POINT('Ctrl Pts',(6.8889452941563,-1.31732608523719,-5.28628660733263));
#23737=CARTESIAN_POINT('Ctrl Pts',(6.9546279799784,-0.915822948130322,-5.26796901957214));
#23738=CARTESIAN_POINT('Ctrl Pts',(6.97983819041424,-0.698170157146178,
-5.2581709353385));
#23739=CARTESIAN_POINT('Ctrl Pts',(7.00781143127827,-0.290269127143199,
-5.23984979167635));
#23740=CARTESIAN_POINT('Ctrl Pts',(7.01310174712942,-0.100396500618003,
-5.2313370143895));
#23741=CARTESIAN_POINT('Ctrl Pts',(7.00928089057375,0.199051880567814,-5.21777728906797));
#23742=CARTESIAN_POINT('Ctrl Pts',(7.00531266557363,0.30859991953487,-5.21278300268002));
#23743=CARTESIAN_POINT('Ctrl Pts',(6.98158728758654,0.705837637291974,-5.19457236717849));
#23744=CARTESIAN_POINT('Ctrl Pts',(6.94665710998975,0.992332074562671,-5.18126963967956));
#23745=CARTESIAN_POINT('Ctrl Pts',(6.85597364790044,1.48234554062127,-5.15840232062872));
#23746=CARTESIAN_POINT('Ctrl Pts',(6.80850316320757,1.68701206812089,-5.14881242820551));
#23747=CARTESIAN_POINT('Ctrl Pts',(6.69411925160376,2.09580625252878,-5.12954641415351));
#23748=CARTESIAN_POINT('Ctrl Pts',(6.62687127628842,2.29961202115196,-5.11988312154751));
#23749=CARTESIAN_POINT('Ctrl Pts',(6.45251862516887,2.756439942648,-5.09793245849722));
#23750=CARTESIAN_POINT('Ctrl Pts',(6.3396799790906,3.00689437778745,-5.08568917062978));
#23751=CARTESIAN_POINT('Ctrl Pts',(6.16007886246485,3.35019700701687,-5.0682400307183));
#23752=CARTESIAN_POINT('Ctrl Pts',(6.10529438365007,3.44902476145725,-5.06313182744073));
#23753=CARTESIAN_POINT('Ctrl Pts',(5.93912073600712,3.73241578671817,-5.04817582179967));
#23754=CARTESIAN_POINT('Ctrl Pts',(5.82158146460825,3.91321737801238,-5.03826343675899));
#23755=CARTESIAN_POINT('Ctrl Pts',(5.51996940853453,4.33342785555409,-5.01446796623745));
#23756=CARTESIAN_POINT('Ctrl Pts',(5.32839521754225,4.56693208006331,-5.00061537900585));
#23757=CARTESIAN_POINT('Ctrl Pts',(4.99328129453979,4.92549613841691,-4.97828631747505));
#23758=CARTESIAN_POINT('Ctrl Pts',(4.8586533818069,5.05834549469446,-4.96973889305962));
#23759=CARTESIAN_POINT('Ctrl Pts',(4.55335442338125,5.33616345512455,-4.95115805038667));
#23760=CARTESIAN_POINT('Ctrl Pts',(4.3807770225186,5.47872889107436,-4.94115133866499));
#23761=CARTESIAN_POINT('Ctrl Pts',(4.05716400257742,5.72098198394382,-4.92303450322575));
#23762=CARTESIAN_POINT('Ctrl Pts',(3.90852624558663,5.82354151113776,-4.91493682758702));
#23763=CARTESIAN_POINT('Ctrl Pts',(3.66342411535084,5.97904641016079,-4.90179339501776));
#23764=CARTESIAN_POINT('Ctrl Pts',(3.56938370746226,6.03565832098991,-4.8967922520089));
#23765=CARTESIAN_POINT('Ctrl Pts',(3.40871001119445,6.12731442169353,-4.88832709939066));
#23766=CARTESIAN_POINT('Ctrl Pts',(3.34276994090111,6.16353591655151,-4.88487562078499));
#23767=CARTESIAN_POINT('Ctrl Pts',(2.91068531912496,6.39191026605421,-4.86242337175407));
#23768=CARTESIAN_POINT('Ctrl Pts',(2.5287247133862,6.55241707554525,-4.84338993644098));
#23769=CARTESIAN_POINT('Ctrl Pts',(1.93856019464885,6.74107389614773,-4.81525394774652));
#23770=CARTESIAN_POINT('Ctrl Pts',(1.73959909928719,6.79513720893601,-4.8059618347278));
#23771=CARTESIAN_POINT('Ctrl Pts',(1.17827430318887,6.92139124222625,-4.78011706316965));
#23772=CARTESIAN_POINT('Ctrl Pts',(0.812172143355865,6.97383358486175,-4.76370414853906));
#23773=CARTESIAN_POINT('Ctrl Pts',(0.324072299708876,7.00478128660869,-4.74152719440797));
#23774=CARTESIAN_POINT('Ctrl Pts',(0.204318291362056,7.00929645774514,-4.73605580997046));
#23775=CARTESIAN_POINT('Ctrl Pts',(-0.0989748059805782,7.01295244028332,
-4.72215425318536));
#23776=CARTESIAN_POINT('Ctrl Pts',(-0.282474672911588,7.00796016287849,
-4.7137048124347));
#23777=CARTESIAN_POINT('Ctrl Pts',(-0.708992712108262,6.97957554126962,
-4.6940471780958));
#23778=CARTESIAN_POINT('Ctrl Pts',(-0.951410426440865,6.95068100315977,
-4.68286401330344));
#23779=CARTESIAN_POINT('Ctrl Pts',(-1.37627961892231,6.87739157466336,-4.66324151956071));
#23780=CARTESIAN_POINT('Ctrl Pts',(-1.55938259890341,6.83820063129862,-4.65477559786249));
#23781=CARTESIAN_POINT('Ctrl Pts',(-1.9502396885087,6.73802515195734,-4.63660628141201));
#23782=CARTESIAN_POINT('Ctrl Pts',(-2.15718274362952,6.67465213721348,-4.62692608644044));
#23783=CARTESIAN_POINT('Ctrl Pts',(-2.54788460171998,6.53493380206192,-4.60833400214877));
#23784=CARTESIAN_POINT('Ctrl Pts',(-2.73197552733957,6.46013804580409,-4.59943167485397));
#23785=CARTESIAN_POINT('Ctrl Pts',(-3.01391716052841,6.33137633869536,-4.58539291192272));
#23786=CARTESIAN_POINT('Ctrl Pts',(-3.11407640382979,6.2827183849206,-4.58031727872298));
#23787=CARTESIAN_POINT('Ctrl Pts',(-3.28247985232057,6.1958903767336,-4.57164390928719));
#23788=CARTESIAN_POINT('Ctrl Pts',(-3.35132310281836,6.15892562923275,-4.56805801760813));
#23789=CARTESIAN_POINT('Ctrl Pts',(-3.77103344811813,5.92444492914084,-4.54596606919803));
#23790=CARTESIAN_POINT('Ctrl Pts',(-4.10497246511925,5.69815351094268,-4.52743742372748));
#23791=CARTESIAN_POINT('Ctrl Pts',(-4.57561920977808,5.31626968473013,-4.49990856148787));
#23792=CARTESIAN_POINT('Ctrl Pts',(-4.72794437893988,5.18126994390225,-4.49073226988463));
#23793=CARTESIAN_POINT('Ctrl Pts',(-5.0756926188213,4.8449516462406,-4.46899584952018));
#23794=CARTESIAN_POINT('Ctrl Pts',(-5.26533000746845,4.63815811979918,-4.45649208908233));
#23795=CARTESIAN_POINT('Ctrl Pts',(-5.51787367553666,4.32725653558499,-4.43847376052746));
#23796=CARTESIAN_POINT('Ctrl Pts',(-5.5912572939989,4.23201140327411,-4.43304720976354));
#23797=CARTESIAN_POINT('Ctrl Pts',(-5.7159541582044,4.06125792598364,-4.4234323640533));
#23798=CARTESIAN_POINT('Ctrl Pts',(-5.76830919154459,3.98654696326831,-4.41926401880285));
#23799=CARTESIAN_POINT('Ctrl Pts',(-5.91832603620198,3.76332701830764,-4.4069400660947));
#23800=CARTESIAN_POINT('Ctrl Pts',(-6.01181602556229,3.61210202038548,-4.39875774161554));
#23801=CARTESIAN_POINT('Ctrl Pts',(-6.22424303243211,3.2373532685571,-4.37894546442074));
#23802=CARTESIAN_POINT('Ctrl Pts',(-6.33702003603994,3.01062081028342,-4.36734276624509));
#23803=CARTESIAN_POINT('Ctrl Pts',(-6.50676703027325,2.61731678805357,-4.34784642969746));
#23804=CARTESIAN_POINT('Ctrl Pts',(-6.57017874608918,2.45379641593338,-4.33991294832414));
#23805=CARTESIAN_POINT('Ctrl Pts',(-6.74448595619915,1.948915497106,-4.31584706652881));
#23806=CARTESIAN_POINT('Ctrl Pts',(-6.83536941741902,1.60127606293307,-4.29988137936741));
#23807=CARTESIAN_POINT('Ctrl Pts',(-6.91800407317094,1.14452974964774,-4.27897974113059));
#23808=CARTESIAN_POINT('Ctrl Pts',(-6.93442260486219,1.04043817544725,-4.27421844970426));
#23809=CARTESIAN_POINT('Ctrl Pts',(-6.99027522850461,0.625817670587475,
-4.25519105535893));
#23810=CARTESIAN_POINT('Ctrl Pts',(-7.01124210805982,0.313172090659878,
-4.2407473831395));
#23811=CARTESIAN_POINT('Ctrl Pts',(-7.01124999777253,0.000176733446466751,
-4.22636455703907));
#23812=CARTESIAN_POINT('Ctrl Pts',(-7.0112499978881,0.00017208778304258,
-4.22646564308965));
#23813=CARTESIAN_POINT('Ctrl Pts',(-7.01125459996624,-0.187327104922663,
-4.2179538597749));
#23814=CARTESIAN_POINT('Ctrl Pts',(-7.00373353003433,-0.374843190662422,
-4.20944207646015));
#23815=CARTESIAN_POINT('Ctrl Pts',(-6.98870878823683,-0.561761547029809,
-4.2009302931454));
#23816=CARTESIAN_POINT('Ctrl Pts',(-6.97368319756446,-0.748690463997657,
-4.19241802892795));
#23817=CARTESIAN_POINT('Ctrl Pts',(-6.9511531095221,-0.93502127618761,-4.1839057647105));
#23818=CARTESIAN_POINT('Ctrl Pts',(-6.9211925057364,-1.12014323237624,-4.17539350049304));
#23819=CARTESIAN_POINT('Ctrl Pts',(-6.89123239521493,-1.30526214076115,
-4.16688137641948));
#23820=CARTESIAN_POINT('Ctrl Pts',(-6.85384206526541,-1.48917192862319,
-4.15836925234591));
#23821=CARTESIAN_POINT('Ctrl Pts',(-6.80914691169823,-1.67127044412639,
-4.14985712827235));
#23822=CARTESIAN_POINT('Ctrl Pts',(-6.76444180092798,-1.85340952760519,
-4.14134310786459));
#23823=CARTESIAN_POINT('Ctrl Pts',(-6.71242868925155,-2.03373623281141,
-4.13282908745683));
#23824=CARTESIAN_POINT('Ctrl Pts',(-6.65328352886334,-2.21166110583331,
-4.12431506704907));
#23825=CARTESIAN_POINT('Ctrl Pts',(-6.62761633303324,-2.28887507446445,
-4.12062024184827));
#23826=CARTESIAN_POINT('Ctrl Pts',(-6.60060659762498,-2.36563690067436,
-4.11692541664747));
#23827=CARTESIAN_POINT('Ctrl Pts',(-6.57227159525839,-2.44189939200201,
-4.11323059144668));
#23828=CARTESIAN_POINT('Ctrl Pts',(-6.57227158383948,-2.44189942273553,
-4.6606292049078));
#23829=CARTESIAN_POINT('Ctrl Pts',(-6.70390621728781,-2.08761023588097,
-4.67773914757001));
#23830=CARTESIAN_POINT('Ctrl Pts',(-6.80669705592026,-1.72320489332983,
-4.69459415246904));
#23831=CARTESIAN_POINT('Ctrl Pts',(-6.8942421135184,-1.27781271705034,-4.71496363186487));
#23832=CARTESIAN_POINT('Ctrl Pts',(-6.90766216320481,-1.20315543525653,
-4.7183718645118));
#23833=CARTESIAN_POINT('Ctrl Pts',(-6.93758375007867,-1.01964549419006,
-4.72675020208282));
#23834=CARTESIAN_POINT('Ctrl Pts',(-6.95273764935542,-0.910595489399886,
-4.73173114360371));
#23835=CARTESIAN_POINT('Ctrl Pts',(-6.99590754101394,-0.535308904302658,
-4.74893736830413));
#23836=CARTESIAN_POINT('Ctrl Pts',(-7.01124315989833,-0.267853137209664,
-4.76127380578758));
#23837=CARTESIAN_POINT('Ctrl Pts',(-7.01125616410567,0.241211380042968,
-4.78468215521764));
#23838=CARTESIAN_POINT('Ctrl Pts',(-6.99879608154224,0.482443869538131,
-4.79574490275203));
#23839=CARTESIAN_POINT('Ctrl Pts',(-6.95454963225591,0.909499595056456,
-4.81528242823844));
#23840=CARTESIAN_POINT('Ctrl Pts',(-6.92767134590944,1.09559177564294,-4.82378164659587));
#23841=CARTESIAN_POINT('Ctrl Pts',(-6.85328797825378,1.49605893575086,-4.84212032646349));
#23842=CARTESIAN_POINT('Ctrl Pts',(-6.80312743939344,1.7097386383162,-4.85193514871219));
#23843=CARTESIAN_POINT('Ctrl Pts',(-6.69135122731386,2.10215003965919,-4.87021889566688));
#23844=CARTESIAN_POINT('Ctrl Pts',(-6.63236935521845,2.28142305464891,-4.87867739602326));
#23845=CARTESIAN_POINT('Ctrl Pts',(-6.52787863739525,2.56054559408591,-4.89217164560283));
#23846=CARTESIAN_POINT('Ctrl Pts',(-6.48713477867009,2.66208091752975,-4.89715582769753));
#23847=CARTESIAN_POINT('Ctrl Pts',(-6.38618840884508,2.89754642513058,-4.90887903910264));
#23848=CARTESIAN_POINT('Ctrl Pts',(-6.32412098437491,3.03062221629724,-4.91562892313301));
#23849=CARTESIAN_POINT('Ctrl Pts',(-6.11679971881715,3.44097761944665,-4.93677868961053));
#23850=CARTESIAN_POINT('Ctrl Pts',(-5.95713126674611,3.71054690471241,-4.95115154162357));
#23851=CARTESIAN_POINT('Ctrl Pts',(-5.67263970273283,4.12489429513226,-4.97401646496258));
#23852=CARTESIAN_POINT('Ctrl Pts',(-5.5589918147202,4.27682191451809,-4.98258951225769));
#23853=CARTESIAN_POINT('Ctrl Pts',(-5.29671652139686,4.59929346983292,-5.00129800651448));
#23854=CARTESIAN_POINT('Ctrl Pts',(-5.14571502500059,4.76763293840727,-5.01140565108458));
#23855=CARTESIAN_POINT('Ctrl Pts',(-4.85820073886254,5.05855778491549,-5.02973830064952));
#23856=CARTESIAN_POINT('Ctrl Pts',(-4.72450834552819,5.18364163316081,-5.0379498830824));
#23857=CARTESIAN_POINT('Ctrl Pts',(-4.4997412231803,5.37800924921345,-5.05141469837085));
#23858=CARTESIAN_POINT('Ctrl Pts',(-4.41159619883565,5.45054792240292,-5.05662136292772));
#23859=CARTESIAN_POINT('Ctrl Pts',(-4.19274521403411,5.62186287422926,-5.06934998955121));
#23860=CARTESIAN_POINT('Ctrl Pts',(-4.06027139790908,5.71827337155505,-5.0768870993764));
#23861=CARTESIAN_POINT('Ctrl Pts',(-3.69404964851037,5.96565104395998,-5.09721749249556));
#23862=CARTESIAN_POINT('Ctrl Pts',(-3.45449158594315,6.10749433473452,-5.1099803871655));
#23863=CARTESIAN_POINT('Ctrl Pts',(-3.04006933351791,6.32067268306784,-5.13118804424986));
#23864=CARTESIAN_POINT('Ctrl Pts',(-2.86961096598136,6.39986399361892,-5.13968434669682));
#23865=CARTESIAN_POINT('Ctrl Pts',(-2.49392285582217,6.55636948057832,-5.15800827483852));
#23866=CARTESIAN_POINT('Ctrl Pts',(-2.28783068562546,6.63109820841612,-5.16781138680754));
#23867=CARTESIAN_POINT('Ctrl Pts',(-1.89759290916194,6.7522351463715,-5.18612128988212));
#23868=CARTESIAN_POINT('Ctrl Pts',(-1.71440687784977,6.80105475186465,-5.19461775716185));
#23869=CARTESIAN_POINT('Ctrl Pts',(-1.4225672291869,6.86628928141453,-5.20815778505994));
#23870=CARTESIAN_POINT('Ctrl Pts',(-1.31512015945449,6.8876762543057,-5.21314901403829));
#23871=CARTESIAN_POINT('Ctrl Pts',(-1.06205205194053,6.9319109140208,-5.22490524125236));
#23872=CARTESIAN_POINT('Ctrl Pts',(-0.916123168975142,6.95270173267984,
-5.23168125048848));
#23873=CARTESIAN_POINT('Ctrl Pts',(-0.459758082269938,7.00310306459452,
-5.25280287560086));
#23874=CARTESIAN_POINT('Ctrl Pts',(-0.147925049822086,7.01661981552651,
-5.26712116522719));
#23875=CARTESIAN_POINT('Ctrl Pts',(0.353314907659504,7.00490833466094,-5.28993009385463));
#23876=CARTESIAN_POINT('Ctrl Pts',(0.542600648481804,6.99279331011027,-5.29850063154806));
#23877=CARTESIAN_POINT('Ctrl Pts',(0.955717812126998,6.94947542758775,-5.31719664334724));
#23878=CARTESIAN_POINT('Ctrl Pts',(1.17900327353281,6.91509632353111,-5.32729442246173));
#23879=CARTESIAN_POINT('Ctrl Pts',(1.57946014632695,6.83347540813823,-5.34561190263004));
#23880=CARTESIAN_POINT('Ctrl Pts',(1.75717955787997,6.78994837413825,-5.35381828449975));
#23881=CARTESIAN_POINT('Ctrl Pts',(2.04231668194139,6.70816699631933,-5.36725884042856));
#23882=CARTESIAN_POINT('Ctrl Pts',(2.15086121074734,6.67415590566567,-5.37244650716258));
#23883=CARTESIAN_POINT('Ctrl Pts',(2.41225178430267,6.58521333907708,-5.38509096611195));
#23884=CARTESIAN_POINT('Ctrl Pts',(2.56411081606651,6.52758214676201,-5.39256257809965));
#23885=CARTESIAN_POINT('Ctrl Pts',(2.9728435641803,6.35600012754387,-5.41295498145386));
#23886=CARTESIAN_POINT('Ctrl Pts',(3.22509093691513,6.23179982166028,-5.42584530572912));
#23887=CARTESIAN_POINT('Ctrl Pts',(3.63257878684362,5.99977841309522,-5.44718338554033));
#23888=CARTESIAN_POINT('Ctrl Pts',(3.79214334581374,5.90022203051291,-5.45568484932166));
#23889=CARTESIAN_POINT('Ctrl Pts',(4.12897764336816,5.67074790180028,-5.47403487931341));
#23890=CARTESIAN_POINT('Ctrl Pts',(4.30453298717051,5.53866722424426,-5.48385870964967));
#23891=CARTESIAN_POINT('Ctrl Pts',(4.61835709735215,5.27861227506268,-5.50212242281259));
#23892=CARTESIAN_POINT('Ctrl Pts',(4.75822823513098,5.15288582155602,-5.51055180079543));
#23893=CARTESIAN_POINT('Ctrl Pts',(4.97114535632935,4.94543045900397,-5.52401103294801));
#23894=CARTESIAN_POINT('Ctrl Pts',(5.04761981505703,4.86735061284432,-5.52898990317804));
#23895=CARTESIAN_POINT('Ctrl Pts',(5.28531488702843,4.61303702173026,-5.54491845710866));
#23896=CARTESIAN_POINT('Ctrl Pts',(5.43937069638893,4.43033969889257,-5.55592567941762));
#23897=CARTESIAN_POINT('Ctrl Pts',(5.71800133490058,4.06341341139405,-5.57710026901083));
#23898=CARTESIAN_POINT('Ctrl Pts',(5.84373613370387,3.88041467470019,-5.58726057644863));
#23899=CARTESIAN_POINT('Ctrl Pts',(6.06056948761918,3.53032340841884,-5.60599358800878));
#23900=CARTESIAN_POINT('Ctrl Pts',(6.15395836412213,3.36488987640865,-5.61457712308354));
#23901=CARTESIAN_POINT('Ctrl Pts',(6.34396198930457,2.9938730092555,-5.63333773553946));
#23902=CARTESIAN_POINT('Ctrl Pts',(6.43753861109095,2.78697444509421,-5.64348656152049));
#23903=CARTESIAN_POINT('Ctrl Pts',(6.58824561808943,2.40545848224129,-5.66187265736131));
#23904=CARTESIAN_POINT('Ctrl Pts',(6.64886531533272,2.2324424354922,-5.67009605360231));
#23905=CARTESIAN_POINT('Ctrl Pts',(6.73660825648486,1.94657141526927,-5.68364913403675));
#23906=CARTESIAN_POINT('Ctrl Pts',(6.76783262889296,1.83506721414836,-5.68893221611056));
#23907=CARTESIAN_POINT('Ctrl Pts',(6.83792256297493,1.55857601904308,-5.70199859010682));
#23908=CARTESIAN_POINT('Ctrl Pts',(6.87359451254463,1.39285399253202,-5.70979829890135));
#23909=CARTESIAN_POINT('Ctrl Pts',(6.94999793375986,0.962651139356424,-5.72989698975842));
#23910=CARTESIAN_POINT('Ctrl Pts',(6.98166120249297,0.696834938462023,-5.74216638201182));
#23911=CARTESIAN_POINT('Ctrl Pts',(7.00955502099417,0.242725585568709,-5.76287175551013));
#23912=CARTESIAN_POINT('Ctrl Pts',(7.01353913261123,0.0552054826433945,
-5.77135111488268));
#23913=CARTESIAN_POINT('Ctrl Pts',(7.00589901430265,-0.349762775455823,
-5.78958902682646));
#23914=CARTESIAN_POINT('Ctrl Pts',(6.99167393646226,-0.566966754980128,
-5.79932379705014));
#23915=CARTESIAN_POINT('Ctrl Pts',(6.94564379190608,-0.976474418599964,
-5.81778888747249));
#23916=CARTESIAN_POINT('Ctrl Pts',(6.91587835810513,-1.16880055450405,-5.82650937513558));
#23917=CARTESIAN_POINT('Ctrl Pts',(6.85672868373382,-1.46802792137355,-5.84032251187271));
#23918=CARTESIAN_POINT('Ctrl Pts',(6.83274382423929,-1.57589505695686,-5.84535822128053));
#23919=CARTESIAN_POINT('Ctrl Pts',(6.735689642359,-1.96835720429491,-5.86386222842968));
#23920=CARTESIAN_POINT('Ctrl Pts',(6.64730156138577,-2.24885022792779,-5.87741782164038));
#23921=CARTESIAN_POINT('Ctrl Pts',(6.46662001669965,-2.71732296584495,-5.90045136230478));
#23922=CARTESIAN_POINT('Ctrl Pts',(6.38303640796235,-2.90824118798729,-5.90996020281285));
#23923=CARTESIAN_POINT('Ctrl Pts',(6.19318611573004,-3.29412236647469,-5.92947115545108));
#23924=CARTESIAN_POINT('Ctrl Pts',(6.08591182043921,-3.48833424810144,-5.93945405321215));
#23925=CARTESIAN_POINT('Ctrl Pts',(5.82510822334941,-3.91173334406615,-5.96176801844721));
#23926=CARTESIAN_POINT('Ctrl Pts',(5.66690089155583,-4.13760505953238,-5.97405882283894));
#23927=CARTESIAN_POINT('Ctrl Pts',(5.42947375803411,-4.43732532204864,-5.99129752003615));
#23928=CARTESIAN_POINT('Ctrl Pts',(5.36122825266725,-4.51954341314763,-5.99613485629221));
#23929=CARTESIAN_POINT('Ctrl Pts',(5.02288070966675,-4.90871178621462,-6.01963184827458));
#23930=CARTESIAN_POINT('Ctrl Pts',(4.72815728289039,-5.19319881463183,-6.0385459037528));
#23931=CARTESIAN_POINT('Ctrl Pts',(4.27894856406941,-5.5566885261447,-6.06498223518058));
#23932=CARTESIAN_POINT('Ctrl Pts',(4.14376853386443,-5.65821276367141,-6.07267733515801));
#23933=CARTESIAN_POINT('Ctrl Pts',(3.78012610677635,-5.9112916003396,-6.0927513643439));
#23934=CARTESIAN_POINT('Ctrl Pts',(3.54621572088584,-6.05450896422114,-6.10504501523413));
#23935=CARTESIAN_POINT('Ctrl Pts',(3.08610916948512,-6.30038761924725,-6.12841946046126));
#23936=CARTESIAN_POINT('Ctrl Pts',(2.86166855482467,-6.40545111666512,-6.13948895318468));
#23937=CARTESIAN_POINT('Ctrl Pts',(2.5316105293928,-6.53913907747908,-6.15560895566176));
#23938=CARTESIAN_POINT('Ctrl Pts',(2.43014745855055,-6.57752037678161,-6.16054952415093));
#23939=CARTESIAN_POINT('Ctrl Pts',(2.05568743160319,-6.70932311625542,-6.17871129988722));
#23940=CARTESIAN_POINT('Ctrl Pts',(1.77788575318046,-6.7882243442581,-6.19202222402473));
#23941=CARTESIAN_POINT('Ctrl Pts',(1.28922590751124,-6.89494920809898,-6.21497704368261));
#23942=CARTESIAN_POINT('Ctrl Pts',(1.08049549130856,-6.93072576545548,-6.22464480964778));
#23943=CARTESIAN_POINT('Ctrl Pts',(0.659355031407631,-6.98341910910548,
-6.24390958938615));
#23944=CARTESIAN_POINT('Ctrl Pts',(0.447150726398731,-7.00021068726772,
-6.25349601558817));
#23945=CARTESIAN_POINT('Ctrl Pts',(-0.0479150094512006,-7.01677872881925,
-6.27573545400535));
#23946=CARTESIAN_POINT('Ctrl Pts',(-0.330650687769794,-7.0091474322944,
-6.28833750190172));
#23947=CARTESIAN_POINT('Ctrl Pts',(-0.722904410143011,-6.97476855196262,
-6.30607670790614));
#23948=CARTESIAN_POINT('Ctrl Pts',(-0.833409285102849,-6.96242887557347,
-6.311105588362));
#23949=CARTESIAN_POINT('Ctrl Pts',(-1.38274308358209,-6.88782073617079,
-6.33635129730869));
#23950=CARTESIAN_POINT('Ctrl Pts',(-1.81526823350533,-6.786667836431,-6.35686880016417));
#23951=CARTESIAN_POINT('Ctrl Pts',(-2.4082933198585,-6.58718793621379,-6.3854507255645));
#23952=CARTESIAN_POINT('Ctrl Pts',(-2.57890510103155,-6.52228269564939,
-6.39374013815183));
#23953=CARTESIAN_POINT('Ctrl Pts',(-2.82933461806604,-6.41564811689309,
-6.40604262781619));
#23954=CARTESIAN_POINT('Ctrl Pts',(-2.9111952322872,-6.37891978400674,-6.41008673270239));
#23955=CARTESIAN_POINT('Ctrl Pts',(-3.20607472588871,-6.2397575338227,-6.42475624235216));
#23956=CARTESIAN_POINT('Ctrl Pts',(-3.41458332433729,-6.1281408589003,-6.4353201318437));
#23957=CARTESIAN_POINT('Ctrl Pts',(-3.7586230823732,-5.92095334177488,-6.45332838543319));
#23958=CARTESIAN_POINT('Ctrl Pts',(-3.89712972844991,-5.8307216173014,-6.46075112571011));
#23959=CARTESIAN_POINT('Ctrl Pts',(-4.12700081411852,-5.66911693031274,
-6.47348647246354));
#23960=CARTESIAN_POINT('Ctrl Pts',(-4.2200202129524,-5.60021883402846,-6.47876782501162));
#23961=CARTESIAN_POINT('Ctrl Pts',(-4.44482669160317,-5.42492547707781,
-6.49182656067331));
#23962=CARTESIAN_POINT('Ctrl Pts',(-4.57454684955087,-5.31599675076628,
-6.49962033275064));
#23963=CARTESIAN_POINT('Ctrl Pts',(-4.89883956243725,-5.02301353446546,
-6.51972395108936));
#23964=CARTESIAN_POINT('Ctrl Pts',(-5.0870445420839,-4.83231574338115,-6.53200418158846));
#23965=CARTESIAN_POINT('Ctrl Pts',(-5.38135978233284,-4.49780184072536,
-6.55228135748184));
#23966=CARTESIAN_POINT('Ctrl Pts',(-5.49371302340107,-4.35985928930604,
-6.5603275647837));
#23967=CARTESIAN_POINT('Ctrl Pts',(-5.72660556133383,-4.05060716273615,
-6.57776759697057));
#23968=CARTESIAN_POINT('Ctrl Pts',(-5.84496164891105,-3.87786716922929,
-6.58713843404064));
#23969=CARTESIAN_POINT('Ctrl Pts',(-6.06481104935635,-3.52401262702012,
-6.60580253501089));
#23970=CARTESIAN_POINT('Ctrl Pts',(-6.16634450597322,-3.34317087659181,
-6.61508683885542));
#23971=CARTESIAN_POINT('Ctrl Pts',(-6.3069702654834,-3.06443449918892,-6.62921800477762));
#23972=CARTESIAN_POINT('Ctrl Pts',(-6.35211616926502,-2.9697225814325,-6.63399490891892));
#23973=CARTESIAN_POINT('Ctrl Pts',(-6.45898223987877,-2.73193097941898,
-6.64591800053814));
#23974=CARTESIAN_POINT('Ctrl Pts',(-6.5180611244172,-2.58780462279585,-6.65307815376513));
#23975=CARTESIAN_POINT('Ctrl Pts',(-6.5722714983487,-2.44189965283043,-6.66023848729892));
#23976=CARTESIAN_POINT('Origin',(0.,0.,0.));
#23977=CARTESIAN_POINT('',(-6.57227159525839,-2.44189939200199,-8.66029439624775));
#23978=CARTESIAN_POINT('',(-6.57227165853301,-2.44189922170096,-8.11305756739085));
#23979=CARTESIAN_POINT('',(-6.57227159525839,-2.441899392002,0.));
#23980=CARTESIAN_POINT('Ctrl Pts',(-6.57227165853301,-2.44189922170096,
-8.11305756739085));
#23981=CARTESIAN_POINT('Ctrl Pts',(-6.51817519271005,-2.58749764197787,
-8.10608231724909));
#23982=CARTESIAN_POINT('Ctrl Pts',(-6.45923882215988,-2.73130286006209,
-8.0991275279903));
#23983=CARTESIAN_POINT('Ctrl Pts',(-6.33712037052739,-3.00314237969816,
-8.08577404493706));
#23984=CARTESIAN_POINT('Ctrl Pts',(-6.27473543286156,-3.13139800508645,
-8.0793815528912));
#23985=CARTESIAN_POINT('Ctrl Pts',(-6.16355711632633,-3.34328277427315,
-8.06859486435757));
#23986=CARTESIAN_POINT('Ctrl Pts',(-6.11686483163985,-3.4279644824695,-8.06422004891531));
#23987=CARTESIAN_POINT('Ctrl Pts',(-5.99274121333451,-3.64246061971337,
-8.05294144285684));
#23988=CARTESIAN_POINT('Ctrl Pts',(-5.9128377489431,-3.77078446643113,-8.04601158176694));
#23989=CARTESIAN_POINT('Ctrl Pts',(-5.68078292142082,-4.11792658014196,
-8.02682113598621));
#23990=CARTESIAN_POINT('Ctrl Pts',(-5.52020798851787,-4.3308105001367,-8.01454987363125));
#23991=CARTESIAN_POINT('Ctrl Pts',(-5.22641443800212,-4.67734054736446,
-7.99376276196743));
#23992=CARTESIAN_POINT('Ctrl Pts',(-5.09920929828207,-4.81570229432193,
-7.98521238398094));
#23993=CARTESIAN_POINT('Ctrl Pts',(-4.77036319129291,-5.14573188995945,
-7.96412293838842));
#23994=CARTESIAN_POINT('Ctrl Pts',(-4.56258523254715,-5.33082923970444,
-7.95166344456971));
#23995=CARTESIAN_POINT('Ctrl Pts',(-4.21575006671975,-5.60463457235991,
-7.93186652732066));
#23996=CARTESIAN_POINT('Ctrl Pts',(-4.08361626691444,-5.70162738977248,
-7.92453006375508));
#23997=CARTESIAN_POINT('Ctrl Pts',(-3.85386888447544,-5.85818687811532,
-7.91201145782549));
#23998=CARTESIAN_POINT('Ctrl Pts',(-3.75797669565571,-5.92015791706546,
-7.90685140890572));
#23999=CARTESIAN_POINT('Ctrl Pts',(-3.35368857734603,-6.16764986481274,
-7.88527471484278));
#24000=CARTESIAN_POINT('Ctrl Pts',(-3.03275446176226,-6.3316294580092,-7.86864324095011));
#24001=CARTESIAN_POINT('Ctrl Pts',(-2.50925959838254,-6.5501341291496,-7.84262266007155));
#24002=CARTESIAN_POINT('Ctrl Pts',(-2.31441160311268,-6.62149090484725,
-7.83315618534303));
#24003=CARTESIAN_POINT('Ctrl Pts',(-1.71783496608031,-6.81041146448286,
-7.80476754391258));
#24004=CARTESIAN_POINT('Ctrl Pts',(-1.30847988470247,-6.90076408149348,
-7.78612330577171));
#24005=CARTESIAN_POINT('Ctrl Pts',(-0.820128773837127,-6.96351132196717,
-7.76402426653175));
#24006=CARTESIAN_POINT('Ctrl Pts',(-0.746597344149629,-6.97177835629235,
-7.76069878717101));
#24007=CARTESIAN_POINT('Ctrl Pts',(-0.564354023764458,-6.98935144802316,
-7.75244684525943));
#24008=CARTESIAN_POINT('Ctrl Pts',(-0.455531393873775,-6.99728661804769,
-7.74750901691098));
#24009=CARTESIAN_POINT('Ctrl Pts',(-0.166941845043998,-7.01156909937355,
-7.73434570204032));
#24010=CARTESIAN_POINT('Ctrl Pts',(0.0129573714319099,-7.01354416492444,
-7.72608435581353));
#24011=CARTESIAN_POINT('Ctrl Pts',(0.416039609820819,-7.00245970656703,
-7.7075377941428));
#24012=CARTESIAN_POINT('Ctrl Pts',(0.638928484736241,-6.98564975975726,
-7.69725933870154));
#24013=CARTESIAN_POINT('Ctrl Pts',(1.04818172256356,-6.93503090250718,-7.67838699514727));
#24014=CARTESIAN_POINT('Ctrl Pts',(1.2347160983123,-6.90426073555607,-7.66978424118245));
#24015=CARTESIAN_POINT('Ctrl Pts',(1.71374568405082,-6.80520480935842,-7.64763715745567));
#24016=CARTESIAN_POINT('Ctrl Pts',(2.00350447835029,-6.72560106154017,-7.63419616636894));
#24017=CARTESIAN_POINT('Ctrl Pts',(2.48964951866254,-6.55782793963812,-7.61115532333263));
#24018=CARTESIAN_POINT('Ctrl Pts',(2.68872121877613,-6.47875280894356,-7.60156725238652));
#24019=CARTESIAN_POINT('Ctrl Pts',(2.98525083369218,-6.34494110385861,-7.58683255586316));
#24020=CARTESIAN_POINT('Ctrl Pts',(3.08553692081057,-6.29678181487987,-7.5817617336861));
#24021=CARTESIAN_POINT('Ctrl Pts',(3.436369340257,-6.11791110360568,-7.56373508888826));
#24022=CARTESIAN_POINT('Ctrl Pts',(3.68011604037794,-5.97446370742416,-7.55070040509004));
#24023=CARTESIAN_POINT('Ctrl Pts',(4.09098900750442,-5.6979531826868,-7.52797353176129));
#24024=CARTESIAN_POINT('Ctrl Pts',(4.26194496183058,-5.57123763934641,-7.51826070876749));
#24025=CARTESIAN_POINT('Ctrl Pts',(4.59106903748204,-5.30325776469124,-7.49899969670924));
#24026=CARTESIAN_POINT('Ctrl Pts',(4.74912157020259,-5.16219953346053,-7.48946075461461));
#24027=CARTESIAN_POINT('Ctrl Pts',(5.10716828169107,-4.81226847836516,-7.46698482479571));
#24028=CARTESIAN_POINT('Ctrl Pts',(5.3011061557193,-4.59775672716515,-7.45410331544837));
#24029=CARTESIAN_POINT('Ctrl Pts',(5.5487896495945,-4.28722406604433,-7.43619722595163));
#24030=CARTESIAN_POINT('Ctrl Pts',(5.61435203948097,-4.20100079446446,-7.43129396117637));
#24031=CARTESIAN_POINT('Ctrl Pts',(5.78460655947834,-3.96598551284471,-7.41807084366292));
#24032=CARTESIAN_POINT('Ctrl Pts',(5.88554790328168,-3.81458239403292,-7.40971370741527));
#24033=CARTESIAN_POINT('Ctrl Pts',(6.09609552605055,-3.47049107377572,-7.39115883803676));
#24034=CARTESIAN_POINT('Ctrl Pts',(6.2026871626226,-3.27618103792163,-7.38096856961922));
#24035=CARTESIAN_POINT('Ctrl Pts',(6.38262817790572,-2.90778483295969,-7.36220684332091));
#24036=CARTESIAN_POINT('Ctrl Pts',(6.45849151211225,-2.7351497354249,-7.35362712588235));
#24037=CARTESIAN_POINT('Ctrl Pts',(6.63357967465798,-2.28866405948016,-7.33191541296364));
#24038=CARTESIAN_POINT('Ctrl Pts',(6.72287263719483,-2.01130527664654,-7.31887668513947));
#24039=CARTESIAN_POINT('Ctrl Pts',(6.84884588211138,-1.51630923499633,-7.29599354187019));
#24040=CARTESIAN_POINT('Ctrl Pts',(6.892988858788,-1.30099417499752,-7.28615915682875));
#24041=CARTESIAN_POINT('Ctrl Pts',(6.94396998395295,-0.975205561409179,
-7.27122696245657));
#24042=CARTESIAN_POINT('Ctrl Pts',(6.9584252124808,-0.866061645879403,-7.26621024907983));
#24043=CARTESIAN_POINT('Ctrl Pts',(7.00082706162474,-0.475440040128734,
-7.24822800460087));
#24044=CARTESIAN_POINT('Ctrl Pts',(7.01430697306611,-0.192666848376906,
-7.23518066190373));
#24045=CARTESIAN_POINT('Ctrl Pts',(7.00791699459066,0.30428356830222,-7.21237153645258));
#24046=CARTESIAN_POINT('Ctrl Pts',(6.99535385784562,0.51818499952154,-7.2025902543283));
#24047=CARTESIAN_POINT('Ctrl Pts',(6.95064379059364,0.94457130352698,-7.18313239595964));
#24048=CARTESIAN_POINT('Ctrl Pts',(6.91848372796387,1.15682708978907,-7.1734662618088));
#24049=CARTESIAN_POINT('Ctrl Pts',(6.82117084362721,1.64625709416158,-7.15106490792058));
#24050=CARTESIAN_POINT('Ctrl Pts',(6.74877593285378,1.92160227799906,-7.13838069462069));
#24051=CARTESIAN_POINT('Ctrl Pts',(6.64385062179033,2.2404234805491,-7.12325361596668));
#24052=CARTESIAN_POINT('Ctrl Pts',(6.62731134533452,2.2888846063367,-7.12094161123295));
#24053=CARTESIAN_POINT('Ctrl Pts',(6.57400369553663,2.43965584654816,-7.11370212319582));
#24054=CARTESIAN_POINT('Ctrl Pts',(6.53538634295797,2.54129294053583,-7.10874992640004));
#24055=CARTESIAN_POINT('Ctrl Pts',(6.39065146904711,2.89707380426187,-7.09117661951697));
#24056=CARTESIAN_POINT('Ctrl Pts',(6.27194272407044,3.1458221597177,-7.07847472992205));
#24057=CARTESIAN_POINT('Ctrl Pts',(6.03249746006562,3.57982230837531,-7.05571703294241));
#24058=CARTESIAN_POINT('Ctrl Pts',(5.9170501266622,3.76758191939754,-7.04565040359384));
#24059=CARTESIAN_POINT('Ctrl Pts',(5.67503961797406,4.12254368379534,-7.02614580139638));
#24060=CARTESIAN_POINT('Ctrl Pts',(5.54943852748492,4.29012528818939,-7.01671079925425));
#24061=CARTESIAN_POINT('Ctrl Pts',(5.23107653002378,4.67747461441378,-6.99419410083532));
#24062=CARTESIAN_POINT('Ctrl Pts',(5.0317095340301,4.89130119970314,-6.98117314653623));
#24063=CARTESIAN_POINT('Ctrl Pts',(4.73946237932808,5.1679101678667,-6.96304180099587));
#24064=CARTESIAN_POINT('Ctrl Pts',(4.65755588733432,5.24184815195318,-6.95805014302439));
#24065=CARTESIAN_POINT('Ctrl Pts',(4.43672915741739,5.43192745495537,-6.94477961869521));
#24066=CARTESIAN_POINT('Ctrl Pts',(4.29499849107725,5.54467205903683,-6.93646401459017));
#24067=CARTESIAN_POINT('Ctrl Pts',(3.96849114943427,5.78436549426352,-6.9178345626302));
#24068=CARTESIAN_POINT('Ctrl Pts',(3.78166660262041,5.908198131128,-6.9075274383583));
#24069=CARTESIAN_POINT('Ctrl Pts',(3.42676215032734,6.11969767484504,-6.88861911683933));
#24070=CARTESIAN_POINT('Ctrl Pts',(3.26043690729395,6.20990750729763,-6.88000885666077));
#24071=CARTESIAN_POINT('Ctrl Pts',(2.81861347951256,6.42688945506487,-6.85772241496385));
#24072=CARTESIAN_POINT('Ctrl Pts',(2.53818201931679,6.54271542689402,-6.84415289199739));
#24073=CARTESIAN_POINT('Ctrl Pts',(2.05757120596388,6.70565436760548,-6.82141645457886));
#24074=CARTESIAN_POINT('Ctrl Pts',(1.86123291250805,6.76278122571477,-6.81226151026225));
#24075=CARTESIAN_POINT('Ctrl Pts',(1.55943660990965,6.83645222220464,-6.79820135841265));
#24076=CARTESIAN_POINT('Ctrl Pts',(1.45563287447383,6.85930417364746,-6.79336227335932));
#24077=CARTESIAN_POINT('Ctrl Pts',(1.08090125771741,6.93291022512691,-6.77589587002869));
#24078=CARTESIAN_POINT('Ctrl Pts',(0.807554912700613,6.97003919652783,-6.76318318159885));
#24079=CARTESIAN_POINT('Ctrl Pts',(0.310520245701929,7.00791478987115,-6.74029328680237));
#24080=CARTESIAN_POINT('Ctrl Pts',(0.0876223906700351,7.01424388409346,
-6.73010713012611));
#24081=CARTESIAN_POINT('Ctrl Pts',(-0.342739865064623,7.00594352479632,
-6.71056247626169));
#24082=CARTESIAN_POINT('Ctrl Pts',(-0.550001215201553,6.99272591980853,
-6.70120413859114));
#24083=CARTESIAN_POINT('Ctrl Pts',(-1.04945901861334,6.93852819869003,-6.67863951195789));
#24084=CARTESIAN_POINT('Ctrl Pts',(-1.34024571486383,6.88827097736807,-6.66549759879253));
#24085=CARTESIAN_POINT('Ctrl Pts',(-1.73467865652842,6.79417182040374,-6.64722756787435));
#24086=CARTESIAN_POINT('Ctrl Pts',(-1.84172999618833,6.76593756488301,-6.64221972285008));
#24087=CARTESIAN_POINT('Ctrl Pts',(-2.12226240203206,6.68479698662707,-6.62891983133171));
#24088=CARTESIAN_POINT('Ctrl Pts',(-2.2944342593525,6.62767520792402,-6.62059083729334));
#24089=CARTESIAN_POINT('Ctrl Pts',(-2.67408710196292,6.48514825080581,-6.60193933390689));
#24090=CARTESIAN_POINT('Ctrl Pts',(-2.88007950768366,6.39632964823763,-6.59162353032621));
#24091=CARTESIAN_POINT('Ctrl Pts',(-3.25139434267168,6.21464813663892,-6.5727043152711));
#24092=CARTESIAN_POINT('Ctrl Pts',(-3.41789282565394,6.12465728644501,-6.56409178119931));
#24093=CARTESIAN_POINT('Ctrl Pts',(-3.84189576222056,5.87280710540862,-6.54176298274265));
#24094=CARTESIAN_POINT('Ctrl Pts',(-4.09287151809201,5.70073961859469,-6.52815439597193));
#24095=CARTESIAN_POINT('Ctrl Pts',(-4.50262227913299,5.37877003992366,-6.50480700081698));
#24096=CARTESIAN_POINT('Ctrl Pts',(-4.66702908684039,5.2367558254219,-6.49508142677324));
#24097=CARTESIAN_POINT('Ctrl Pts',(-4.90846581330569,5.00778953466546,-6.48000090135578));
#24098=CARTESIAN_POINT('Ctrl Pts',(-4.9903714161686,4.92617345323335,-6.47472556069264));
#24099=CARTESIAN_POINT('Ctrl Pts',(-5.25826271359213,4.64568858880247,-6.45695840972673));
#24100=CARTESIAN_POINT('Ctrl Pts',(-5.43467776796553,4.43802062151827,-6.44440223021673));
#24101=CARTESIAN_POINT('Ctrl Pts',(-5.72651142781564,4.05090913540504,-6.42215566534128));
#24102=CARTESIAN_POINT('Ctrl Pts',(-5.84667166910733,3.87546519868902,-6.41244980528081));
#24103=CARTESIAN_POINT('Ctrl Pts',(-6.07033880171417,3.514755915509,-6.39318884680505));
#24104=CARTESIAN_POINT('Ctrl Pts',(-6.17378039797205,3.32970866586246,-6.38364319269721));
#24105=CARTESIAN_POINT('Ctrl Pts',(-6.3984520465339,2.88121212588124,-6.36112372107576));
#24106=CARTESIAN_POINT('Ctrl Pts',(-6.51203712877862,2.61437218374742,-6.34820587646107));
#24107=CARTESIAN_POINT('Ctrl Pts',(-6.64484320577531,2.23949640543405,-6.3302760460809));
#24108=CARTESIAN_POINT('Ctrl Pts',(-6.67854312086716,2.13690123503765,-6.3253871362613));
#24109=CARTESIAN_POINT('Ctrl Pts',(-6.76984834968026,1.83563500788081,-6.31104229493326));
#24110=CARTESIAN_POINT('Ctrl Pts',(-6.82104814237988,1.63514627549764,-6.30153036791633));
#24111=CARTESIAN_POINT('Ctrl Pts',(-6.90610487471028,1.22768153889449,-6.28238133669502));
#24112=CARTESIAN_POINT('Ctrl Pts',(-6.93969300269204,1.02085688592325,-6.27275397964097));
#24113=CARTESIAN_POINT('Ctrl Pts',(-6.97400667889152,0.726875324778639,
-6.25921896890452));
#24114=CARTESIAN_POINT('Ctrl Pts',(-6.98244783564724,0.640733382814972,
-6.25527035484034));
#24115=CARTESIAN_POINT('Ctrl Pts',(-7.00392758728411,0.369967034499953,
-6.24290898893682));
#24116=CARTESIAN_POINT('Ctrl Pts',(-7.01125277045169,0.184968370858522,
-6.23453801484205));
#24117=CARTESIAN_POINT('Ctrl Pts',(-7.01124677665848,-0.215320004964521,
-6.21651180210464));
#24118=CARTESIAN_POINT('Ctrl Pts',(-7.00133432271619,-0.430421342449451,
-6.20687998953804));
#24119=CARTESIAN_POINT('Ctrl Pts',(-6.96294211853579,-0.846158790037305,
-6.18817303064746));
#24120=CARTESIAN_POINT('Ctrl Pts',(-6.93563167370119,-1.04668951243584,
-6.17910730173908));
#24121=CARTESIAN_POINT('Ctrl Pts',(-6.87975920415703,-1.35614245711543,
-6.16486257391386));
#24122=CARTESIAN_POINT('Ctrl Pts',(-6.85718273817151,-1.46603312094027,
-6.15974794181732));
#24123=CARTESIAN_POINT('Ctrl Pts',(-6.81409091533509,-1.65291580623209,
-6.15096724362044));
#24124=CARTESIAN_POINT('Ctrl Pts',(-6.79488156059996,-1.73018789276738,
-6.14731269945627));
#24125=CARTESIAN_POINT('Ctrl Pts',(-6.71706876478634,-2.02188583155679,
-6.13343855391773));
#24126=CARTESIAN_POINT('Ctrl Pts',(-6.64962111007924,-2.23371632153885,
-6.12320548606609));
#24127=CARTESIAN_POINT('Ctrl Pts',(-6.57227174271038,-2.44189899514102,
-6.11302261786463));
#24128=CARTESIAN_POINT('',(-7.01124999933522,9.65497915988582E-5,-6.77353435691037));
#24129=CARTESIAN_POINT('Ctrl Pts',(-6.5722714983487,-2.44189965283043,-6.66023848729892));
#24130=CARTESIAN_POINT('Ctrl Pts',(-6.66318645252301,-2.19720582956012,
-6.67224691572112));
#24131=CARTESIAN_POINT('Ctrl Pts',(-6.74040831275645,-1.94750920134252,
-6.6842496182875));
#24132=CARTESIAN_POINT('Ctrl Pts',(-6.84556497205163,-1.52516452324806,
-6.70410727531474));
#24133=CARTESIAN_POINT('Ctrl Pts',(-6.88129720898833,-1.35485666965225,
-6.71200071435652));
#24134=CARTESIAN_POINT('Ctrl Pts',(-6.97760540239254,-0.792446624908524,
-6.73777021356879));
#24135=CARTESIAN_POINT('Ctrl Pts',(-7.011256159715,-0.396526017179738,-6.75540657027142));
#24136=CARTESIAN_POINT('Ctrl Pts',(-7.01124999915429,0.000108899215703687,
-6.77325998610253));
#24137=CARTESIAN_POINT('Ctrl Pts',(-7.01124999933522,9.65497915988582E-5,
-6.77353435691037));
#24138=CARTESIAN_POINT('Ctrl Pts',(-7.01124863601993,0.0990977407168242,
-6.77803027512839));
#24139=CARTESIAN_POINT('Ctrl Pts',(-7.00915014456632,0.198092936793512,
-6.78252619334641));
#24140=CARTESIAN_POINT('Ctrl Pts',(-7.00495668404128,0.296999018862735,
-6.78702211156443));
#24141=CARTESIAN_POINT('Ctrl Pts',(-6.99699833034792,0.484703083043638,
-6.79555446977832));
#24142=CARTESIAN_POINT('Ctrl Pts',(-6.98148974930442,0.672118710222703,
-6.80408682799221));
#24143=CARTESIAN_POINT('Ctrl Pts',(-6.95847548566115,0.858630000613053,
-6.8126191862061));
#24144=CARTESIAN_POINT('Ctrl Pts',(-6.93546553152443,1.04510636606995,-6.82114994670415));
#24145=CARTESIAN_POINT('Ctrl Pts',(-6.90495273703956,1.23067842912626,-6.8296807072022));
#24146=CARTESIAN_POINT('Ctrl Pts',(-6.86703342573335,1.41473619179017,-6.83821146770025));
#24147=CARTESIAN_POINT('Ctrl Pts',(-6.82748037163525,1.60672403104786,-6.84710977359913));
#24148=CARTESIAN_POINT('Ctrl Pts',(-6.77986849624805,1.79706384305653,-6.856008079498));
#24149=CARTESIAN_POINT('Ctrl Pts',(-6.72436639184499,1.985075109593,-6.86490638539687));
#24150=CARTESIAN_POINT('Ctrl Pts',(-6.67115844925952,2.16531499027655,-6.873436882654));
#24151=CARTESIAN_POINT('Ctrl Pts',(-6.61069953595977,2.34341464114204,-6.88196737991113));
#24152=CARTESIAN_POINT('Ctrl Pts',(-6.54318928729106,2.5187894936218,-6.89049787716825));
#24153=CARTESIAN_POINT('Ctrl Pts',(-6.47567834775357,2.69416614080698,-6.89902846172256));
#24154=CARTESIAN_POINT('Ctrl Pts',(-6.4011160415954,2.86681764949735,-6.90755904627686));
#24155=CARTESIAN_POINT('Ctrl Pts',(-6.31975051686545,3.03617851370417,-6.91608963083117));
#24156=CARTESIAN_POINT('Ctrl Pts',(-6.23836889177823,3.20557289051269,-6.92462190339104));
#24157=CARTESIAN_POINT('Ctrl Pts',(-6.1501814927871,3.37167504694702,-6.93315417595092));
#24158=CARTESIAN_POINT('Ctrl Pts',(-6.05548326369799,3.53394241684462,-6.9416864485108));
#24159=CARTESIAN_POINT('Ctrl Pts',(-6.0432572013677,3.55489202696535,-6.9427880118361));
#24160=CARTESIAN_POINT('Ctrl Pts',(-6.03092267699221,3.57577775305031,-6.94388957516141));
#24161=CARTESIAN_POINT('Ctrl Pts',(-6.01848037998311,3.59659845941388,-6.94499113848672));
#24162=CARTESIAN_POINT('Ctrl Pts',(-5.92210631537392,3.75786901089051,-6.95352349670053));
#24163=CARTESIAN_POINT('Ctrl Pts',(-5.81923020290197,3.91529086095874,-6.96205585491435));
#24164=CARTESIAN_POINT('Ctrl Pts',(-5.71018447586611,4.06834362045263,-6.97058821312816));
#24165=CARTESIAN_POINT('Ctrl Pts',(-5.60115916804912,4.22136772024681,-6.9791189736261));
#24166=CARTESIAN_POINT('Ctrl Pts',(-5.48596672866419,4.37002411305193,-6.98764973412403));
#24167=CARTESIAN_POINT('Ctrl Pts',(-5.36498231317679,4.51382225412125,-6.99618049462197));
#24168=CARTESIAN_POINT('Ctrl Pts',(-5.23878531839894,4.66381589738911,-7.00507880052089));
#24169=CARTESIAN_POINT('Ctrl Pts',(-5.10628640973121,4.80852309802423,-7.01397710641981));
#24170=CARTESIAN_POINT('Ctrl Pts',(-4.9679578714695,4.94742570937697,-7.02287541231873));
#24171=CARTESIAN_POINT('Ctrl Pts',(-4.83534709930489,5.08058682550413,-7.03140590957577));
#24172=CARTESIAN_POINT('Ctrl Pts',(-4.69737917042236,5.2084133346288,-7.03993640683282));
#24173=CARTESIAN_POINT('Ctrl Pts',(-4.55450798055408,5.33048624588501,-7.04846690408987));
#24174=CARTESIAN_POINT('Ctrl Pts',(-4.41163532860805,5.45256040637898,-7.05699748864408));
#24175=CARTESIAN_POINT('Ctrl Pts',(-4.26385955013853,5.56888065504471,-7.06552807319829));
#24176=CARTESIAN_POINT('Ctrl Pts',(-4.11166812443973,5.67906786338799,-7.0740586577525));
#24177=CARTESIAN_POINT('Ctrl Pts',(-3.95944658357395,5.7892768752341,-7.08259093031231));
#24178=CARTESIAN_POINT('Ctrl Pts',(-3.80280789877975,5.8933502442502,-7.09112320287213));
#24179=CARTESIAN_POINT('Ctrl Pts',(-3.64226977693333,5.9909512962916,-7.09965547543194));
#24180=CARTESIAN_POINT('Ctrl Pts',(-3.62154342224158,6.00355212903856,-7.10075703875763));
#24181=CARTESIAN_POINT('Ctrl Pts',(-3.60075210863097,6.01604514006157,-7.10185860208332));
#24182=CARTESIAN_POINT('Ctrl Pts',(-3.579896983104,6.02842965894626,-7.10296016540901));
#24183=CARTESIAN_POINT('Ctrl Pts',(-3.41835983181976,6.12435619259727,-7.11149252362288));
#24184=CARTESIAN_POINT('Ctrl Pts',(-3.25293759185572,6.21380235473948,-7.12002488183674));
#24185=CARTESIAN_POINT('Ctrl Pts',(-3.08417037731232,6.29646882357161,-7.12855724005061));
#24186=CARTESIAN_POINT('Ctrl Pts',(-2.91543476505835,6.37911981279959,-7.13708800054863));
#24187=CARTESIAN_POINT('Ctrl Pts',(-2.74335570288113,6.45499350767575,-7.14561876104664));
#24188=CARTESIAN_POINT('Ctrl Pts',(-2.5684966626596,6.52383717273864,-7.15414952154466));
#24189=CARTESIAN_POINT('Ctrl Pts',(-2.38610387019533,6.5956469476201,-7.16304782744355));
#24190=CARTESIAN_POINT('Ctrl Pts',(-2.20068656367054,6.65980734938466,-7.17194613334243));
#24191=CARTESIAN_POINT('Ctrl Pts',(-2.01290676914844,6.71608761863754,-7.18084443924132));
#24192=CARTESIAN_POINT('Ctrl Pts',(-1.8328887926581,6.77004156087621,-7.18937493649842));
#24193=CARTESIAN_POINT('Ctrl Pts',(-1.65070001986582,6.81675362467153,-7.19790543375552));
#24194=CARTESIAN_POINT('Ctrl Pts',(-1.46693909333062,6.85607148875786,-7.20643593101262));
#24195=CARTESIAN_POINT('Ctrl Pts',(-1.28317628627086,6.89538975520507,-7.21496651556689));
#24196=CARTESIAN_POINT('Ctrl Pts',(-1.09784159320205,6.92731360988333,-7.22349710012117));
#24197=CARTESIAN_POINT('Ctrl Pts',(-0.911544208239695,6.95174177590945,
-7.23202768467544));
#24198=CARTESIAN_POINT('Ctrl Pts',(-0.725209959329071,6.97617477570524,
-7.24055995723531));
#24199=CARTESIAN_POINT('Ctrl Pts',(-0.53791294157442,6.99310908564372,-7.24909222979517));
#24200=CARTESIAN_POINT('Ctrl Pts',(-0.350268715347124,7.00249515455377,
-7.25762450235504));
#24201=CARTESIAN_POINT('Ctrl Pts',(-0.326042813468306,7.00370694768493,
-7.25872606568046));
#24202=CARTESIAN_POINT('Ctrl Pts',(-0.301811128741185,7.00479299605895,
-7.25982762900588));
#24203=CARTESIAN_POINT('Ctrl Pts',(-0.277574989016474,7.00575325628676,
-7.2609291923313));
#24204=CARTESIAN_POINT('Ctrl Pts',(-0.0898495799762465,7.01319112577006,
-7.26946155054498));
#24205=CARTESIAN_POINT('Ctrl Pts',(0.0982065849262575,7.01308050338434,
-7.27799390875866));
#24206=CARTESIAN_POINT('Ctrl Pts',(0.285976026660581,7.00541535347301,-7.28652626697234));
#24207=CARTESIAN_POINT('Ctrl Pts',(0.473710307867381,6.99775163888957,-7.29505702747016));
#24208=CARTESIAN_POINT('Ctrl Pts',(0.661157667450691,6.98253623230385,-7.30358778796797));
#24209=CARTESIAN_POINT('Ctrl Pts',(0.847702268630839,6.95981518621423,-7.31211854846579));
#24210=CARTESIAN_POINT('Ctrl Pts',(1.04228409114593,6.93611521028568,-7.32101685436477));
#24211=CARTESIAN_POINT('Ctrl Pts',(1.23588328914722,6.90424853101664,-7.32991516026376));
#24212=CARTESIAN_POINT('Ctrl Pts',(1.42780782494883,6.86432745267261,-7.33881346616274));
#24213=CARTESIAN_POINT('Ctrl Pts',(1.6117992211513,6.82605649939534,-7.34734396341966));
#24214=CARTESIAN_POINT('Ctrl Pts',(1.79425129499713,6.78038367833687,-7.35587446067657));
#24215=CARTESIAN_POINT('Ctrl Pts',(1.97456509440875,6.72746008910068,-7.36440495793349));
#24216=CARTESIAN_POINT('Ctrl Pts',(2.15488073906813,6.67453595826904,-7.37293554248756));
#24217=CARTESIAN_POINT('Ctrl Pts',(2.33305777288524,6.6143610002643,-7.38146612704163));
#24218=CARTESIAN_POINT('Ctrl Pts',(2.50851227005532,6.54713622536464,-7.38999671159569));
#24219=CARTESIAN_POINT('Ctrl Pts',(2.68400148561692,6.4798981482351,-7.39852898415537));
#24220=CARTESIAN_POINT('Ctrl Pts',(2.85676680316711,6.40560757842274,-7.40706125671504));
#24221=CARTESIAN_POINT('Ctrl Pts',(3.02624332798783,6.32451404317432,-7.41559352927471));
#24222=CARTESIAN_POINT('Ctrl Pts',(3.04812367968835,6.31404442165151,-7.41669509260101));
#24223=CARTESIAN_POINT('Ctrl Pts',(3.06994924291153,6.30346147136764,-7.4177966559273));
#24224=CARTESIAN_POINT('Ctrl Pts',(3.09171882933523,6.29276578642762,-7.4188982192536));
#24225=CARTESIAN_POINT('Ctrl Pts',(3.2603391030037,6.20992042195642,-7.42743057746784));
#24226=CARTESIAN_POINT('Ctrl Pts',(3.42565599669263,6.12027970542203,-7.43596293568208));
#24227=CARTESIAN_POINT('Ctrl Pts',(3.58712364851388,6.02413234356388,-7.44449529389633));
#24228=CARTESIAN_POINT('Ctrl Pts',(3.74856106491592,5.92800298565736,-7.45302605439471));
#24229=CARTESIAN_POINT('Ctrl Pts',(3.90615041507801,5.82536957037538,-7.4615568148931));
#24230=CARTESIAN_POINT('Ctrl Pts',(4.0593720831585,5.71656582687311,-7.47008757539149));
#24231=CARTESIAN_POINT('Ctrl Pts',(4.21919526341856,5.60307430489335,-7.47898588129019));
#24232=CARTESIAN_POINT('Ctrl Pts',(4.37426576303269,5.48286916830926,-7.48788418718889));
#24233=CARTESIAN_POINT('Ctrl Pts',(4.52402850388267,5.3563786888678,-7.49678249308758));
#24234=CARTESIAN_POINT('Ctrl Pts',(4.66760084952214,5.23511665312112,-7.50531299034507));
#24235=CARTESIAN_POINT('Ctrl Pts',(4.80629515369704,5.10807864373767,-7.51384348760255));
#24236=CARTESIAN_POINT('Ctrl Pts',(4.93965666679844,4.97568272467746,-7.52237398486003));
#24237=CARTESIAN_POINT('Ctrl Pts',(5.07301954465978,4.84328545073876,-7.53090456941467));
#24238=CARTESIAN_POINT('Ctrl Pts',(5.20104930753212,4.70553037542654,-7.53943515396931));
#24239=CARTESIAN_POINT('Ctrl Pts',(5.32332818444906,4.56287229748437,-7.54796573852394));
#24240=CARTESIAN_POINT('Ctrl Pts',(5.44563125753062,4.42018599080453,-7.55649801108418));
#24241=CARTESIAN_POINT('Ctrl Pts',(5.56218097344032,4.27259497672405,-7.56503028364441));
#24242=CARTESIAN_POINT('Ctrl Pts',(5.67259939792121,4.12058765629418,-7.57356255620464));
#24243=CARTESIAN_POINT('Ctrl Pts',(5.68685502393588,4.10096267503106,-7.57466411952838));
#24244=CARTESIAN_POINT('Ctrl Pts',(5.70100850922188,4.08126412436716,-7.57576568285213));
#24245=CARTESIAN_POINT('Ctrl Pts',(5.71505909169771,4.06149309255886,-7.57686724617588));
#24246=CARTESIAN_POINT('Ctrl Pts',(5.82389042277079,3.90835298522979,-7.58539960438884));
#24247=CARTESIAN_POINT('Ctrl Pts',(5.92658126006258,3.75081021222637,-7.59393196260179));
#24248=CARTESIAN_POINT('Ctrl Pts',(6.02278906149478,3.58937856504978,-7.60246432081475));
#24249=CARTESIAN_POINT('Ctrl Pts',(6.11897884765776,3.4279771465505,-7.61099508131185));
#24250=CARTESIAN_POINT('Ctrl Pts',(6.20868786402269,3.26268856984488,-7.61952584180895));
#24251=CARTESIAN_POINT('Ctrl Pts',(6.29161808584625,3.09405372034042,-7.62805660230605));
#24252=CARTESIAN_POINT('Ctrl Pts',(6.37812133281203,2.91815328606017,-7.63695490820539));
#24253=CARTESIAN_POINT('Ctrl Pts',(6.45724854463107,2.73861215130986,-7.64585321410474));
#24254=CARTESIAN_POINT('Ctrl Pts',(6.52871552906318,2.5560712241777,-7.65475152000408));
#24255=CARTESIAN_POINT('Ctrl Pts',(6.59722844843272,2.38107556818878,-7.66328201726028));
#24256=CARTESIAN_POINT('Ctrl Pts',(6.65870155525924,2.20332342905852,-7.67181251451649));
#24257=CARTESIAN_POINT('Ctrl Pts',(6.71293402198145,2.02339896684367,-7.68034301177269));
#24258=CARTESIAN_POINT('Ctrl Pts',(6.76716704369365,1.84347266336501,-7.68887359632606));
#24259=CARTESIAN_POINT('Ctrl Pts',(6.8141591920312,1.66137428627281,-7.69740418087943));
#24260=CARTESIAN_POINT('Ctrl Pts',(6.85375964843389,1.47770269134199,-7.7059347654328));
#24261=CARTESIAN_POINT('Ctrl Pts',(6.89336794085206,1.29399475204569,-7.71446703799178));
#24262=CARTESIAN_POINT('Ctrl Pts',(6.92558155650885,1.10871327247536,-7.72299931055076));
#24263=CARTESIAN_POINT('Ctrl Pts',(6.95030070758579,0.9224676886658,-7.73153158310974));
#24264=CARTESIAN_POINT('Ctrl Pts',(6.9534920859875,0.898422359126289,-7.73263314643922));
#24265=CARTESIAN_POINT('Ctrl Pts',(6.95655861538205,0.874360969981249,-7.73373470976869));
#24266=CARTESIAN_POINT('Ctrl Pts',(6.95950014379962,0.85028484106981,-7.73483627309817));
#24267=CARTESIAN_POINT('Ctrl Pts',(6.98228428474481,0.663798825413119,-7.74336863131337));
#24268=CARTESIAN_POINT('Ctrl Pts',(6.99757236394241,0.476365082341321,-7.75190098952856));
#24269=CARTESIAN_POINT('Ctrl Pts',(7.00530780586358,0.288598523223641,-7.76043334774376));
#24270=CARTESIAN_POINT('Ctrl Pts',(7.01304179929443,0.100867124093482,-7.7689641082431));
#24271=CARTESIAN_POINT('Ctrl Pts',(7.01322596520084,-0.0871966611166099,
-7.77749486874244));
#24272=CARTESIAN_POINT('Ctrl Pts',(7.00585577577047,-0.274975292714809,
-7.78602562924178));
#24273=CARTESIAN_POINT('Ctrl Pts',(6.99816804381687,-0.470844313447413,
-7.79492393514001));
#24274=CARTESIAN_POINT('Ctrl Pts',(6.98226057294049,-0.666402711573646,
-7.80382224103823));
#24275=CARTESIAN_POINT('Ctrl Pts',(6.95818862517891,-0.860951577576125,
-7.81272054693645));
#24276=CARTESIAN_POINT('Ctrl Pts',(6.93511168371009,-1.04745882817475,-7.82125104419488));
#24277=CARTESIAN_POINT('Ctrl Pts',(6.90453168732619,-1.23303800175695,-7.82978154145329));
#24278=CARTESIAN_POINT('Ctrl Pts',(6.8665501851245,-1.41707978521563,-7.83831203871172));
#24279=CARTESIAN_POINT('Ctrl Pts',(6.82856829423773,-1.60112345207257,-7.84684262326729));
#24280=CARTESIAN_POINT('Ctrl Pts',(6.78318481119027,-1.78362939835818,-7.85537320782286));
#24281=CARTESIAN_POINT('Ctrl Pts',(6.730552258532,-1.96399920001761,-7.86390379237844));
#24282=CARTESIAN_POINT('Ctrl Pts',(6.67790929110769,-2.14440469269313,-7.87243606493959));
#24283=CARTESIAN_POINT('Ctrl Pts',(6.61801447579919,-2.32267290304711,-7.88096833750074));
#24284=CARTESIAN_POINT('Ctrl Pts',(6.55107024750312,-2.49822040156176,-7.88950061006189));
#24285=CARTESIAN_POINT('Ctrl Pts',(6.54242737940247,-2.52088454922139,-7.89060217338141));
#24286=CARTESIAN_POINT('Ctrl Pts',(6.53366707692705,-2.54350337191474,-7.89170373670093));
#24287=CARTESIAN_POINT('Ctrl Pts',(6.52478983488515,-2.56607563666377,-7.89280530002046));
#24288=CARTESIAN_POINT('Ctrl Pts',(6.45602954875569,-2.74091320168762,-7.90133765823293));
#24289=CARTESIAN_POINT('Ctrl Pts',(6.38022624302496,-2.91301489321258,-7.90987001644539));
#24290=CARTESIAN_POINT('Ctrl Pts',(6.29762295895764,-3.08181304256271,-7.91840237465786));
#24291=CARTESIAN_POINT('Ctrl Pts',(6.21503514266295,-3.25057958383062,-7.92693313515447));
#24292=CARTESIAN_POINT('Ctrl Pts',(6.12565002355203,-3.41604354269852,-7.93546389565108));
#24293=CARTESIAN_POINT('Ctrl Pts',(6.02975766319005,-3.57765972189934,-7.9439946561477));
#24294=CARTESIAN_POINT('Ctrl Pts',(5.92973380760608,-3.74623908846612,-7.95289296204728));
#24295=CARTESIAN_POINT('Ctrl Pts',(5.82262972442264,-3.9106314547288,-7.96179126794687));
#24296=CARTESIAN_POINT('Ctrl Pts',(5.7088267966233,-4.07024853892925,-7.97068957384646));
#24297=CARTESIAN_POINT('Ctrl Pts',(5.59972787664448,-4.22326790172758,-7.97922007110219));
#24298=CARTESIAN_POINT('Ctrl Pts',(5.48447295676529,-4.37189854886369,-7.98775056835792));
#24299=CARTESIAN_POINT('Ctrl Pts',(5.36344146151282,-4.5156530260224,-7.99628106561365));
#24300=CARTESIAN_POINT('Ctrl Pts',(5.24240872767983,-4.65940897429815,-8.00481165016655));
#24301=CARTESIAN_POINT('Ctrl Pts',(5.11559949989041,-4.7982884209006,-8.01334223471946));
#24302=CARTESIAN_POINT('Ctrl Pts',(4.98343284197084,-4.93183775808434,-8.02187281927236));
#24303=CARTESIAN_POINT('Ctrl Pts',(4.85124003132286,-5.06541352159678,-8.03040509183089));
#24304=CARTESIAN_POINT('Ctrl Pts',(4.71368788915149,-5.19365685236146,-8.03893736438941));
#24305=CARTESIAN_POINT('Ctrl Pts',(4.57123223064792,-5.31615109416443,-8.04746963694793));
#24306=CARTESIAN_POINT('Ctrl Pts',(4.55284042134847,-5.33196577474073,-8.04857120027954));
#24307=CARTESIAN_POINT('Ctrl Pts',(4.53436692624702,-5.34768468154511,-8.04967276361114));
#24308=CARTESIAN_POINT('Ctrl Pts',(4.51581276754526,-5.36330696594696,-8.05077432694275));
#24309=CARTESIAN_POINT('Ctrl Pts',(4.37209817225324,-5.48431219805896,-8.05930668515607));
#24310=CARTESIAN_POINT('Ctrl Pts',(4.22349290199429,-5.59955805283533,-8.0678390433694));
#24311=CARTESIAN_POINT('Ctrl Pts',(4.0704809751167,-5.70866106838662,-8.07637140158272));
#24312=CARTESIAN_POINT('Ctrl Pts',(3.9174977002926,-5.81774365399168,-8.08490216208018));
#24313=CARTESIAN_POINT('Ctrl Pts',(3.76010966460322,-5.92068551831789,-8.09343292257763));
#24314=CARTESIAN_POINT('Ctrl Pts',(3.59883153447204,-6.01714534883358,-8.10196368307508));
#24315=CARTESIAN_POINT('Ctrl Pts',(3.4306047817481,-6.11776112384758,-8.11086198897425));
#24316=CARTESIAN_POINT('Ctrl Pts',(3.25814559259368,-6.21132373813366,-8.11976029487341));
#24317=CARTESIAN_POINT('Ctrl Pts',(3.08206945287029,-6.29749747520266,-8.12865860077257));
#24318=CARTESIAN_POINT('Ctrl Pts',(2.91327136434961,-6.380109248273,-8.1371890980291));
#24319=CARTESIAN_POINT('Ctrl Pts',(2.74114961801278,-6.45593055312099,-8.14571959528563));
#24320=CARTESIAN_POINT('Ctrl Pts',(2.56626996827503,-6.52471340462013,-8.15425009254217));
#24321=CARTESIAN_POINT('Ctrl Pts',(2.39138852890024,-6.593496960011,-8.16278067709584));
#24322=CARTESIAN_POINT('Ctrl Pts',(2.21374941565735,-6.65524180913895,-8.17131126164952));
#24323=CARTESIAN_POINT('Ctrl Pts',(2.03393712414705,-6.70974860464358,-8.17984184620319));
#24324=CARTESIAN_POINT('Ctrl Pts',(1.85408925193832,-6.76426618578381,-8.18837411876248));
#24325=CARTESIAN_POINT('Ctrl Pts',(1.67206763570726,-6.81154276489854,-8.19690639132176));
#24326=CARTESIAN_POINT('Ctrl Pts',(1.48847149426284,-6.8514289876833,-8.20543866388105));
#24327=CARTESIAN_POINT('Ctrl Pts',(1.4647682223418,-6.85657851848025,-8.20654022720904));
#24328=CARTESIAN_POINT('Ctrl Pts',(1.44103872191223,-6.86160493449024,-8.20764179053704));
#24329=CARTESIAN_POINT('Ctrl Pts',(1.41728429593782,-6.86650797618324,-8.20874335386504));
#24330=CARTESIAN_POINT('Ctrl Pts',(1.23329008826146,-6.90448537342617,-8.21727571208572));
#24331=CARTESIAN_POINT('Ctrl Pts',(1.04773754642442,-6.93506948156557,-8.2258080703064));
#24332=CARTESIAN_POINT('Ctrl Pts',(0.861234884474282,-6.95815356515395,
-8.23434042852708));
#24333=CARTESIAN_POINT('Ctrl Pts',(0.674767145841206,-6.98123332616182,
-8.24287118903195));
#24334=CARTESIAN_POINT('Ctrl Pts',(0.487349945684015,-6.99681582772935,
-8.25140194953683));
#24335=CARTESIAN_POINT('Ctrl Pts',(0.299598379294797,-7.00484599214172,
-8.2599327100417));
#24336=CARTESIAN_POINT('Ctrl Pts',(0.103757590055591,-7.0132221339044,-8.26883101593717));
#24337=CARTESIAN_POINT('Ctrl Pts',(-0.0924466645823951,-7.01338070381287,
-8.27772932183264));
#24338=CARTESIAN_POINT('Ctrl Pts',(-0.288313297052236,-7.00531955054464,
-8.28662762772811));
#24339=CARTESIAN_POINT('Ctrl Pts',(-0.476083844840867,-6.99759160247151,
-8.29515812499206));
#24340=CARTESIAN_POINT('Ctrl Pts',(-0.663543793791819,-6.98230980183732,
-8.30368862225601));
#24341=CARTESIAN_POINT('Ctrl Pts',(-0.850077561831749,-6.95952546524332,
-8.31221911951996));
#24342=CARTESIAN_POINT('Ctrl Pts',(-1.03661323877084,-6.93674089548509,
-8.32074970408102));
#24343=CARTESIAN_POINT('Ctrl Pts',(-1.22222241253063,-6.90645367665657,
-8.32928028864208));
#24344=CARTESIAN_POINT('Ctrl Pts',(-1.40629617974004,-6.86876681925865,
-8.33781087320314));
#24345=CARTESIAN_POINT('Ctrl Pts',(-1.59040637089355,-6.8310725045027,-8.34634314576972));
#24346=CARTESIAN_POINT('Ctrl Pts',(-1.77298024911097,-6.78597568907706,
-8.3548754183363));
#24347=CARTESIAN_POINT('Ctrl Pts',(-1.95341976830739,-6.73363035600306,
-8.36340769090288));
#24348=CARTESIAN_POINT('Ctrl Pts',(-1.97671550220829,-6.72687228573289,
-8.3645092541977));
#24349=CARTESIAN_POINT('Ctrl Pts',(-1.99997567905117,-6.71999346415156,
-8.36561081749251));
#24350=CARTESIAN_POINT('Ctrl Pts',(-2.02319902948267,-6.71299428344762,
-8.36671238078733));
#24351=CARTESIAN_POINT('Ctrl Pts',(-2.20307970019863,-6.65878086048782,
-8.37524473897966));
#24352=CARTESIAN_POINT('Ctrl Pts',(-2.38081037766226,-6.59732405037942,
-8.38377709717198));
#24353=CARTESIAN_POINT('Ctrl Pts',(-2.5558053987975,-6.52881959667883,-8.39230945536431));
#24354=CARTESIAN_POINT('Ctrl Pts',(-2.73076765146093,-6.46032797069327,
-8.40084021584067));
#24355=CARTESIAN_POINT('Ctrl Pts',(-2.90299498527226,-6.3847914462397,-8.40937097631704));
#24356=CARTESIAN_POINT('Ctrl Pts',(-3.07192028301177,-6.3024544692779,-8.4179017367934));
#24357=CARTESIAN_POINT('Ctrl Pts',(-3.24812368004017,-6.2165700266523,-8.42680004270309));
#24358=CARTESIAN_POINT('Ctrl Pts',(-3.4207338764258,-6.12328629325861,-8.43569834861277));
#24359=CARTESIAN_POINT('Ctrl Pts',(-3.58913333758728,-6.02293520200239,
-8.44459665452246));
#24360=CARTESIAN_POINT('Ctrl Pts',(-3.7505720600242,-5.92673209151845,-8.45312715175804));
#24361=CARTESIAN_POINT('Ctrl Pts',(-3.90814086663486,-5.82403429775449,
-8.46165764899363));
#24362=CARTESIAN_POINT('Ctrl Pts',(-4.06132287207676,-5.71518005764002,
-8.47018814622922));
#24363=CARTESIAN_POINT('Ctrl Pts',(-4.21450644511474,-5.60632470355998,
-8.4787187307621));
#24364=CARTESIAN_POINT('Ctrl Pts',(-4.36330287973525,-5.49131295711294,
-8.48724931529497));
#24365=CARTESIAN_POINT('Ctrl Pts',(-4.50722577778393,-5.37052533283105,
-8.49577989982785));
#24366=CARTESIAN_POINT('Ctrl Pts',(-4.65117715485464,-5.24971380746421,
-8.50431217236666));
#24367=CARTESIAN_POINT('Ctrl Pts',(-4.79025283551472,-5.12312431901584,
-8.51284444490546));
#24368=CARTESIAN_POINT('Ctrl Pts',(-4.92400023980192,-4.99117703562303,
-8.52137671744426));
#24369=CARTESIAN_POINT('Ctrl Pts',(-4.94126776702301,-4.97414191393317,
-8.52247828086605));
#24370=CARTESIAN_POINT('Ctrl Pts',(-4.95844653061949,-4.95701753861724,
-8.52357984428784));
#24371=CARTESIAN_POINT('Ctrl Pts',(-4.9755356011107,-4.93980485895749,-8.52468140770962));
#24372=CARTESIAN_POINT('Ctrl Pts',(-5.10790102723548,-4.80648200332974,
-8.53321369808804));
#24373=CARTESIAN_POINT('Ctrl Pts',(-5.23492695661218,-4.66781339360536,
-8.54174598846645));
#24374=CARTESIAN_POINT('Ctrl Pts',(-5.35619159273083,-4.52425001347843,
-8.55027827884486));
#24375=CARTESIAN_POINT('Ctrl Pts',(-5.47743312604602,-4.38071398441329,
-8.55880894368895));
#24376=CARTESIAN_POINT('Ctrl Pts',(-5.59291535928422,-4.2322852796589,-8.56733960853305));
#24377=CARTESIAN_POINT('Ctrl Pts',(-5.70225599664267,-4.07944887346964,
-8.57587027337714));
#24378=CARTESIAN_POINT('Ctrl Pts',(-5.81159359130132,-3.92661672036792,
-8.58440070083235));
#24379=CARTESIAN_POINT('Ctrl Pts',(-5.91478975087791,-3.76937735782259,
-8.59293112828756));
#24380=CARTESIAN_POINT('Ctrl Pts',(-6.01150434705256,-3.60824639511609,
-8.60146155574276));
#24381=CARTESIAN_POINT('Ctrl Pts',(-6.10821283211414,-3.44712561380484,
-8.60999144418516));
#24382=CARTESIAN_POINT('Ctrl Pts',(-6.19844041559358,-3.28211398657138,
-8.61852133262755));
#24383=CARTESIAN_POINT('Ctrl Pts',(-6.2818917023905,-3.11375387626213,-8.62705122106994));
#24384=CARTESIAN_POINT('Ctrl Pts',(-6.36535301325014,-2.94537354274997,
-8.63558213411172));
#24385=CARTESIAN_POINT('Ctrl Pts',(-6.44203626553885,-2.77364419685501,
-8.64411304715349));
#24386=CARTESIAN_POINT('Ctrl Pts',(-6.51169282550364,-2.59913122192483,
-8.65264396019526));
#24387=CARTESIAN_POINT('Ctrl Pts',(-6.53251525701584,-2.54696406824526,
-8.65519410554609));
#24388=CARTESIAN_POINT('Ctrl Pts',(-6.55271011457438,-2.49454831123339,
-8.65774425089692));
#24389=CARTESIAN_POINT('Ctrl Pts',(-6.57227159525839,-2.441899392002,-8.66029439624775));
#24390=CARTESIAN_POINT('Origin',(0.,0.,0.));
#24391=CARTESIAN_POINT('',(-6.57172397189,-2.44169584043396,-10.6602982140525));
#24392=CARTESIAN_POINT('',(-6.57227159525839,-2.44189939200199,-10.1135674911542));
#24393=CARTESIAN_POINT('',(-6.57227159525839,-2.441899392002,0.));
#24394=CARTESIAN_POINT('',(-7.01124021554704,-0.000177496958404323,-10.7735343566727));
#24395=CARTESIAN_POINT('Ctrl Pts',(-6.57172397189039,-2.44169584043291,
-10.6602982140526));
#24396=CARTESIAN_POINT('Ctrl Pts',(-6.766036100056,-1.91888078236536,-10.6856147375756));
#24397=CARTESIAN_POINT('Ctrl Pts',(-6.96373099417918,-1.10522974870895,
-10.7233601182964));
#24398=CARTESIAN_POINT('Ctrl Pts',(-7.01150624902316,-0.273937984959162,
-10.7611054990171));
#24399=CARTESIAN_POINT('Ctrl Pts',(-7.01123043334559,-0.000177506793261869,
-10.7735343562149));
#24400=CARTESIAN_POINT('',(5.31037376991254,-4.57794244025905,-12.));
#24401=CARTESIAN_POINT('Ctrl Pts',(-7.01124999775337,-0.0001774919695956,
-10.7735343569104));
#24402=CARTESIAN_POINT('Ctrl Pts',(-7.01125473885781,0.187104606374703,
-10.7820370306241));
#24403=CARTESIAN_POINT('Ctrl Pts',(-7.00375121472552,0.374409186281723,
-10.7905397043379));
#24404=CARTESIAN_POINT('Ctrl Pts',(-6.98876009213104,0.561122925156835,
-10.7990423780516));
#24405=CARTESIAN_POINT('Ctrl Pts',(-6.97376854100906,0.747842001322058,
-10.8075452948179));
#24406=CARTESIAN_POINT('Ctrl Pts',(-6.95128898438519,0.933969893314279,
-10.8160482115841));
#24407=CARTESIAN_POINT('Ctrl Pts',(-6.92139408241581,1.11889700973748,-10.8245511283503));
#24408=CARTESIAN_POINT('Ctrl Pts',(-6.89150055657391,1.30381561356252,-10.8330536537088));
#24409=CARTESIAN_POINT('Ctrl Pts',(-6.8541924186819,1.48753324643887,-10.8415561790672));
#24410=CARTESIAN_POINT('Ctrl Pts',(-6.80959376620514,1.66944880177863,-10.8500587044256));
#24411=CARTESIAN_POINT('Ctrl Pts',(-6.76498431048066,1.85140842299707,-10.8585632893729));
#24412=CARTESIAN_POINT('Ctrl Pts',(-6.71308088446669,2.03156479294153,-10.8670678743202));
#24413=CARTESIAN_POINT('Ctrl Pts',(-6.65405819721535,2.20932932596551,-10.8755724592675));
#24414=CARTESIAN_POINT('Ctrl Pts',(-6.61092696152564,2.33923198421757,-10.8817872433597));
#24415=CARTESIAN_POINT('Ctrl Pts',(-6.56399505794186,2.46785764044409,-10.8880020274518));
#24416=CARTESIAN_POINT('Ctrl Pts',(-6.51334730152521,2.59498236838215,-10.894216811544));
#24417=CARTESIAN_POINT('Ctrl Pts',(-6.44381562976938,2.7695052985259,-10.9027487655356));
#24418=CARTESIAN_POINT('Ctrl Pts',(-6.36725376840712,2.94126144775786,-10.9112807195273));
#24419=CARTESIAN_POINT('Ctrl Pts',(-6.2839072441766,3.10968427803931,-10.919812673519));
#24420=CARTESIAN_POINT('Ctrl Pts',(-6.2005763275957,3.27807556909886,-10.9283430297986));
#24421=CARTESIAN_POINT('Ctrl Pts',(-6.11046341929546,3.44313451271079,-10.9368733860782));
#24422=CARTESIAN_POINT('Ctrl Pts',(-6.01386096649161,3.6043172499391,-10.9454037423578));
#24423=CARTESIAN_POINT('Ctrl Pts',(-5.91308936073532,3.77245628553556,-10.9543022503668));
#24424=CARTESIAN_POINT('Ctrl Pts',(-5.80525579364537,3.93637679919713,-10.9632007583758));
#24425=CARTESIAN_POINT('Ctrl Pts',(-5.69074430248391,4.09549213724638,-10.9720992663849));
#24426=CARTESIAN_POINT('Ctrl Pts',(-5.58097371801334,4.24801991833405,-10.9806293659859));
#24427=CARTESIAN_POINT('Ctrl Pts',(-5.46506721216166,4.39613212525469,-10.9891594655869));
#24428=CARTESIAN_POINT('Ctrl Pts',(-5.34340634120211,4.53934304005559,-10.9976895651879));
#24429=CARTESIAN_POINT('Ctrl Pts',(-5.22174416957121,4.68255548591846,-11.0062197559839));
#24430=CARTESIAN_POINT('Ctrl Pts',(-5.09432771051767,4.82086630382314,-11.0147499467799));
#24431=CARTESIAN_POINT('Ctrl Pts',(-4.96157800818184,4.95382379896846,-11.0232801375758));
#24432=CARTESIAN_POINT('Ctrl Pts',(-4.82880191749833,5.08680772376708,-11.0318120240263));
#24433=CARTESIAN_POINT('Ctrl Pts',(-4.6906906830514,5.21443598453826,-11.0403439104769));
#24434=CARTESIAN_POINT('Ctrl Pts',(-4.54770193502134,5.3362940017116,-11.0488757969274));
#24435=CARTESIAN_POINT('Ctrl Pts',(-4.52921056939334,5.35205273225019,-11.049979144107));
#24436=CARTESIAN_POINT('Ctrl Pts',(-4.51063768039098,5.3677150163051,-11.0510824912866));
#24437=CARTESIAN_POINT('Ctrl Pts',(-4.49198429904447,5.38328000568779,-11.0521858384662));
#24438=CARTESIAN_POINT('Ctrl Pts',(-4.34773747733382,5.50364425529522,-11.0607180354414));
#24439=CARTESIAN_POINT('Ctrl Pts',(-4.19862571394932,5.61822778014426,-11.0692502324165));
#24440=CARTESIAN_POINT('Ctrl Pts',(-4.04513469379083,5.72664927087296,-11.0777824293916));
#24441=CARTESIAN_POINT('Ctrl Pts',(-3.89167247929069,5.83505041414148,-11.0863130251294));
#24442=CARTESIAN_POINT('Ctrl Pts',(-3.7338328979712,5.93729165461563,-11.0948436208673));
#24443=CARTESIAN_POINT('Ctrl Pts',(-3.57213209683775,6.03303396685628,-11.1033742166051));
#24444=CARTESIAN_POINT('Ctrl Pts',(-3.40345965995557,6.13290415305923,-11.1122726040037));
#24445=CARTESIAN_POINT('Ctrl Pts',(-3.23058596600869,6.2257023943694,-11.1211709914023));
#24446=CARTESIAN_POINT('Ctrl Pts',(-3.05412800691252,6.31109567982396,-11.1300693788009));
#24447=CARTESIAN_POINT('Ctrl Pts',(-2.88496881527845,6.39295687334823,-11.1385997053836));
#24448=CARTESIAN_POINT('Ctrl Pts',(-2.71251619643036,6.46801322098118,-11.1471300319662));
#24449=CARTESIAN_POINT('Ctrl Pts',(-2.53733697359699,6.53601925065385,-11.1556603585489));
#24450=CARTESIAN_POINT('Ctrl Pts',(-2.36215598521096,6.60402596572873,-11.1641907711049));
#24451=CARTESIAN_POINT('Ctrl Pts',(-2.18424862435887,6.66498211312519,-11.1727211836608));
#24452=CARTESIAN_POINT('Ctrl Pts',(-2.00420024027551,6.71869094090356,-11.1812515962168));
#24453=CARTESIAN_POINT('Ctrl Pts',(-1.82411624572041,6.77241039136374,-11.1897836959416));
#24454=CARTESIAN_POINT('Ctrl Pts',(-1.64189067569975,6.81887957279563,-11.1983157956663));
#24455=CARTESIAN_POINT('Ctrl Pts',(-1.4581233812625,6.85795179098801,-11.2068478953911));
#24456=CARTESIAN_POINT('Ctrl Pts',(-1.4343811627069,6.86299981189193,-11.2079502187236));
#24457=CARTESIAN_POINT('Ctrl Pts',(-1.41061322557452,6.86792443286042,-11.2090525420561));
#24458=CARTESIAN_POINT('Ctrl Pts',(-1.38682087669682,6.87272539961098,-11.2101548653885));
#24459=CARTESIAN_POINT('Ctrl Pts',(-1.20261507129361,6.90989558198963,-11.2186893046874));
#24460=CARTESIAN_POINT('Ctrl Pts',(-1.01688339423534,6.93966194091266,-11.2272237439862));
#24461=CARTESIAN_POINT('Ctrl Pts',(-0.830234829243166,6.96192047432399,
-11.235758183285));
#24462=CARTESIAN_POINT('Ctrl Pts',(-0.643620942919284,6.98417487217555,
-11.244291036914));
#24463=CARTESIAN_POINT('Ctrl Pts',(-0.456090812032652,6.99892419212788,
-11.252823890543));
#24464=CARTESIAN_POINT('Ctrl Pts',(-0.268260064727012,7.00611612094552,
-11.2613567441721));
#24465=CARTESIAN_POINT('Ctrl Pts',(-0.0724077147546187,7.01361519221033,
-11.270254006517));
#24466=CARTESIAN_POINT('Ctrl Pts',(0.123771141487748,7.01289715947273,-11.2791512688619));
#24467=CARTESIAN_POINT('Ctrl Pts',(0.319575848457633,7.00396300958126,-11.2880485312068));
#24468=CARTESIAN_POINT('Ctrl Pts',(0.507355008166848,6.99539504824214,-11.296581116928));
#24469=CARTESIAN_POINT('Ctrl Pts',(0.69478975221258,6.97927107636034,-11.3051137026492));
#24470=CARTESIAN_POINT('Ctrl Pts',(0.881264443551761,6.95564515649206,-11.3136462883704));
#24471=CARTESIAN_POINT('Ctrl Pts',(1.06774081813107,6.93201902336107,-11.3221789511122));
#24472=CARTESIAN_POINT('Ctrl Pts',(1.25325681983915,6.90089084851375,-11.330711613854));
#24473=CARTESIAN_POINT('Ctrl Pts',(1.43720371639759,6.86236635863118,-11.3392442765958));
#24474=CARTESIAN_POINT('Ctrl Pts',(1.62118643860935,6.82383436568634,-11.3477786011662));
#24475=CARTESIAN_POINT('Ctrl Pts',(1.80359914631097,6.77790324421311,-11.3563129257366));
#24476=CARTESIAN_POINT('Ctrl Pts',(1.98384418620484,6.72472964567062,-11.3648472503071));
#24477=CARTESIAN_POINT('Ctrl Pts',(2.00691175934491,6.71792454371485,-11.3659394643083));
#24478=CARTESIAN_POINT('Ctrl Pts',(2.02994384797711,6.71100088741002,-11.3670316783096));
#24479=CARTESIAN_POINT('Ctrl Pts',(2.05293921673861,6.70395906423038,-11.3681238923108));
#24480=CARTESIAN_POINT('Ctrl Pts',(2.23244130289167,6.64899051973013,-11.37664972609));
#24481=CARTESIAN_POINT('Ctrl Pts',(2.40976571285594,6.58679883635617,-11.3851755598692));
#24482=CARTESIAN_POINT('Ctrl Pts',(2.58432844263528,6.51758184168686,-11.3937013936483));
#24483=CARTESIAN_POINT('Ctrl Pts',(2.75885790085022,6.44837803974031,-11.4022256024081));
#24484=CARTESIAN_POINT('Ctrl Pts',(2.9306264441014,6.37215171169286,-11.4107498111678));
#24485=CARTESIAN_POINT('Ctrl Pts',(3.09906881065696,6.28914931205432,-11.4192740199276));
#24486=CARTESIAN_POINT('Ctrl Pts',(3.27496811012105,6.2024724014361,-11.4281755948697));
#24487=CARTESIAN_POINT('Ctrl Pts',(3.44723970573288,6.10840595515281,-11.4370771698118));
#24488=CARTESIAN_POINT('Ctrl Pts',(3.61526631523908,6.00728524646514,-11.445978744754));
#24489=CARTESIAN_POINT('Ctrl Pts',(3.77616550589435,5.91045391579584,-11.4545027291869));
#24490=CARTESIAN_POINT('Ctrl Pts',(3.93317212461599,5.80715459675497,-11.4630267136198));
#24491=CARTESIAN_POINT('Ctrl Pts',(4.08577157516053,5.69772737133941,-11.4715506980527));
#24492=CARTESIAN_POINT('Ctrl Pts',(4.23837330556009,5.58829851106731,-11.480074809835));
#24493=CARTESIAN_POINT('Ctrl Pts',(4.38656748876948,5.47274174310529,-11.4885989216173));
#24494=CARTESIAN_POINT('Ctrl Pts',(4.52987021406729,5.3514392836139,-11.4971230333996));
#24495=CARTESIAN_POINT('Ctrl Pts',(4.67320287130983,5.23011148742004,-11.5056489256313));
#24496=CARTESIAN_POINT('Ctrl Pts',(4.81164179646588,5.10303580186513,-11.514174817863));
#24497=CARTESIAN_POINT('Ctrl Pts',(4.94473708522744,4.97063393547306,-11.5227007100946));
#24498=CARTESIAN_POINT('Ctrl Pts',(4.96238869057907,4.95307429444356,-11.5238314464741));
#24499=CARTESIAN_POINT('Ctrl Pts',(4.97994635858858,4.93542102467172,-11.5249621828536));
#24500=CARTESIAN_POINT('Ctrl Pts',(4.99740908835378,4.9176751586638,-11.5260929192331));
#24501=CARTESIAN_POINT('Ctrl Pts',(5.12940952880526,4.78353449676653,-11.534640133909));
#24502=CARTESIAN_POINT('Ctrl Pts',(5.25602657606199,4.64405509543233,-11.5431873485848));
#24503=CARTESIAN_POINT('Ctrl Pts',(5.37683936972328,4.49969165106831,-11.5517345632607));
#24504=CARTESIAN_POINT('Ctrl Pts',(5.49763025943708,4.35535438049936,-11.5602802282849));
#24505=CARTESIAN_POINT('Ctrl Pts',(5.61261880087413,4.20613506705435,-11.5688258933091));
#24506=CARTESIAN_POINT('Ctrl Pts',(5.72142380932097,4.05252219693306,-11.5773715583333));
#24507=CARTESIAN_POINT('Ctrl Pts',(5.83462397684529,3.89270416208481,-11.5862624239852));
#24508=CARTESIAN_POINT('Ctrl Pts',(5.94113043624094,3.72813050389469,-11.595153289637));
#24509=CARTESIAN_POINT('Ctrl Pts',(6.04056253881339,3.55938629221167,-11.6040441552888));
#24510=CARTESIAN_POINT('Ctrl Pts',(6.13612965882716,3.39720126431498,-11.6125894279201));
#24511=CARTESIAN_POINT('Ctrl Pts',(6.22516184564189,3.23116406529217,-11.6211347005513));
#24512=CARTESIAN_POINT('Ctrl Pts',(6.30736689750766,3.06182125257576,-11.6296799731825));
#24513=CARTESIAN_POINT('Ctrl Pts',(6.38957175909986,2.89247883182385,-11.6382252260346));
#24514=CARTESIAN_POINT('Ctrl Pts',(6.46494938717006,2.71983108719843,-11.6467704788867));
#24515=CARTESIAN_POINT('Ctrl Pts',(6.53325460348441,2.54444706145555,-11.6553157317389));
#24516=CARTESIAN_POINT('Ctrl Pts',(6.60157144856407,2.36903317709009,-11.6638624393956));
#24517=CARTESIAN_POINT('Ctrl Pts',(6.66281336753809,2.19088236457828,-11.6724091470523));
#24518=CARTESIAN_POINT('Ctrl Pts',(6.71678386931552,2.01058225780566,-11.680955854709));
#24519=CARTESIAN_POINT('Ctrl Pts',(6.72332195472672,1.98874037272202,-11.6819912185245));
#24520=CARTESIAN_POINT('Ctrl Pts',(6.72975338948023,1.96686696498067,-11.6830265823399));
#24521=CARTESIAN_POINT('Ctrl Pts',(6.73607787396623,1.94496309434462,-11.6840619461554));
#24522=CARTESIAN_POINT('Ctrl Pts',(6.78803206725332,1.76502780771706,-11.6925672230537));
#24523=CARTESIAN_POINT('Ctrl Pts',(6.832782121241,1.58297591034739,-11.701072499952));
#24524=CARTESIAN_POINT('Ctrl Pts',(6.87017476756959,1.39940173844046,-11.7095777768503));
#24525=CARTESIAN_POINT('Ctrl Pts',(6.90756022416318,1.21586286357125,-11.7180814183819));
#24526=CARTESIAN_POINT('Ctrl Pts',(6.93759103410159,1.03080260171472,-11.7265850599135));
#24527=CARTESIAN_POINT('Ctrl Pts',(6.96016488598172,0.844826208428179,-11.7350887014451));
#24528=CARTESIAN_POINT('Ctrl Pts',(6.9838223879921,0.649922081236072,-11.7440005574145));
#24529=CARTESIAN_POINT('Ctrl Pts',(6.99928929715512,0.454012056972497,-11.7529124133839));
#24530=CARTESIAN_POINT('Ctrl Pts',(7.00650878861348,0.257800615945896,-11.7618242693533));
#24531=CARTESIAN_POINT('Ctrl Pts',(7.01339764590694,0.0705751549320466,
-11.7703279852101));
#24532=CARTESIAN_POINT('Ctrl Pts',(7.01277762320226,-0.116924398607505,
-11.778831701067));
#24533=CARTESIAN_POINT('Ctrl Pts',(7.00465270090815,-0.304084037989905,
-11.7873354169239));
#24534=CARTESIAN_POINT('Ctrl Pts',(6.99652748248866,-0.491250498695174,
-11.7958394427118));
#24535=CARTESIAN_POINT('Ctrl Pts',(6.9808968355076,-0.678076711090961,-11.8043434684998));
#24536=CARTESIAN_POINT('Ctrl Pts',(6.95781679305076,-0.863951408842418,
-11.8128474942878));
#24537=CARTESIAN_POINT('Ctrl Pts',(6.93473092359782,-1.04987303419992,-11.8213536670789));
#24538=CARTESIAN_POINT('Ctrl Pts',(6.90419194189063,-1.23484235776442,-11.8298598398701));
#24539=CARTESIAN_POINT('Ctrl Pts',(6.86630752895882,-1.41825508293234,-11.8383660126613));
#24540=CARTESIAN_POINT('Ctrl Pts',(6.86086658322036,-1.44459675245163,-11.8395876661334));
#24541=CARTESIAN_POINT('Ctrl Pts',(6.85527421229141,-1.47090633170256,-11.8408093196056));
#24542=CARTESIAN_POINT('Ctrl Pts',(6.84953082152621,-1.49718204887129,-11.8420309730777));
#24543=CARTESIAN_POINT('Ctrl Pts',(6.80917135818051,-1.68182451658929,-11.850615671655));
#24544=CARTESIAN_POINT('Ctrl Pts',(6.76133572224075,-1.86486078725442,-11.8592003702323));
#24545=CARTESIAN_POINT('Ctrl Pts',(6.70617623540106,-2.04568493718903,-11.8677850688095));
#24546=CARTESIAN_POINT('Ctrl Pts',(6.65102750995593,-2.22647380905754,-11.8763680925466));
#24547=CARTESIAN_POINT('Ctrl Pts',(6.58855787255442,-2.40505113644434,-11.8849511162836));
#24548=CARTESIAN_POINT('Ctrl Pts',(6.51896962033777,-2.58082576932524,-11.8935341400206));
#24549=CARTESIAN_POINT('Ctrl Pts',(6.44703718968831,-2.7625216186516,-11.9024062950189));
#24550=CARTESIAN_POINT('Ctrl Pts',(6.36749828660038,-2.94122233992901,-11.9112784500172));
#24551=CARTESIAN_POINT('Ctrl Pts',(6.28063099339152,-3.1162960204945,-11.9201506050155));
#24552=CARTESIAN_POINT('Ctrl Pts',(6.19660794304912,-3.28563737018311,-11.9287322644471));
#24553=CARTESIAN_POINT('Ctrl Pts',(6.10572894942552,-3.45158515555319,-11.9373139238787));
#24554=CARTESIAN_POINT('Ctrl Pts',(6.00829329235825,-3.6135907731096,-11.9458955833104));
#24555=CARTESIAN_POINT('Ctrl Pts',(5.90591023089262,-3.78382240698266,-11.954912986092));
#24556=CARTESIAN_POINT('Ctrl Pts',(5.79628751298796,-3.94970081146458,-11.9639303888736));
#24557=CARTESIAN_POINT('Ctrl Pts',(5.67982548128847,-4.11062149371676,-11.9729477916552));
#24558=CARTESIAN_POINT('Ctrl Pts',(5.56336344958899,-4.27154217596894,-11.9819651944368));
#24559=CARTESIAN_POINT('Ctrl Pts',(5.44006233029551,-4.42750482809971,-11.9909825972184));
#24560=CARTESIAN_POINT('Ctrl Pts',(5.31037376991253,-4.57794244025905,-12.));
#24561=CARTESIAN_POINT('',(-5.30612006659788,-4.5828720690575,-12.));
#24562=CARTESIAN_POINT('Origin',(0.,0.,-12.));
#24563=CARTESIAN_POINT('Ctrl Pts',(-5.30612006659788,-4.5828720690575,-12.));
#24564=CARTESIAN_POINT('Ctrl Pts',(-5.03347260351227,-4.89854751301181,
-11.9809094032564));
#24565=CARTESIAN_POINT('Ctrl Pts',(-4.73319340804265,-5.18926879016435,
-11.961640649704));
#24566=CARTESIAN_POINT('Ctrl Pts',(-4.26928721805366,-5.56444336543857,
-11.934434282125));
#24567=CARTESIAN_POINT('Ctrl Pts',(-4.12544111385343,-5.67191152130197,
-11.9262961500531));
#24568=CARTESIAN_POINT('Ctrl Pts',(-3.6470612840599,-6.00147544434351,-11.9000812266326));
#24569=CARTESIAN_POINT('Ctrl Pts',(-3.29755039688922,-6.20039684214918,
-11.8822436608555));
#24570=CARTESIAN_POINT('Ctrl Pts',(-2.84327523265843,-6.4096145726469,-11.8596945470418));
#24571=CARTESIAN_POINT('Ctrl Pts',(-2.75274343167674,-6.44901360156294,
-11.8552267223847));
#24572=CARTESIAN_POINT('Ctrl Pts',(-2.51138791433897,-6.54804188864338,
-11.8433498403589));
#24573=CARTESIAN_POINT('Ctrl Pts',(-2.35927765702271,-6.60437201916886,
-11.8359092031642));
#24574=CARTESIAN_POINT('Ctrl Pts',(-1.98152840657345,-6.72954456640903,
-11.8176136683002));
#24575=CARTESIAN_POINT('Ctrl Pts',(-1.75410314623136,-6.79237427609974,
-11.8067576240749));
#24576=CARTESIAN_POINT('Ctrl Pts',(-1.36036524116173,-6.88005218881468,
-11.7882865299175));
#24577=CARTESIAN_POINT('Ctrl Pts',(-1.19553075121103,-6.91060193019187,
-11.7806467369069));
#24578=CARTESIAN_POINT('Ctrl Pts',(-0.615042517245142,-6.99679430867117,
-11.7540249259773));
#24579=CARTESIAN_POINT('Ctrl Pts',(-0.195638850546006,-7.02104953336165,
-11.7353431450287));
#24580=CARTESIAN_POINT('Ctrl Pts',(0.297165582144061,-7.00533824086339,
-11.7132142035408));
#24581=CARTESIAN_POINT('Ctrl Pts',(0.370874232377533,-7.00182286714805,
-11.7098979420791));
#24582=CARTESIAN_POINT('Ctrl Pts',(0.553165261822067,-6.9902423168726,-11.7016656930351));
#24583=CARTESIAN_POINT('Ctrl Pts',(0.661639547676978,-6.9808102898942,-11.6967383421722));
#24584=CARTESIAN_POINT('Ctrl Pts',(0.948828547277942,-6.94908445857838,
-11.6835757905944));
#24585=CARTESIAN_POINT('Ctrl Pts',(1.12697637330927,-6.92242540608268,-11.6753043121028));
#24586=CARTESIAN_POINT('Ctrl Pts',(1.52354478053644,-6.84736524831524,-11.6567404154643));
#24587=CARTESIAN_POINT('Ctrl Pts',(1.74107898270743,-6.79531050024874,-11.6464547558566));
#24588=CARTESIAN_POINT('Ctrl Pts',(2.13731763355941,-6.68021304921843,-11.6275709920011));
#24589=CARTESIAN_POINT('Ctrl Pts',(2.31667464301831,-6.62015054629303,-11.6189639974111));
#24590=CARTESIAN_POINT('Ctrl Pts',(2.77281340618289,-6.44658950593237,-11.5968674463903));
#24591=CARTESIAN_POINT('Ctrl Pts',(3.0451553181144,-6.32250287310991,-11.583479759843));
#24592=CARTESIAN_POINT('Ctrl Pts',(3.50228552551207,-6.07781315501453,-11.5602494497656));
#24593=CARTESIAN_POINT('Ctrl Pts',(3.69085097825893,-5.96518509499422,-11.550418783469));
#24594=CARTESIAN_POINT('Ctrl Pts',(3.96923164540474,-5.7806513947774,-11.5352842242218));
#24595=CARTESIAN_POINT('Ctrl Pts',(4.06307942085906,-5.71507787643148,-11.5300621540794));
#24596=CARTESIAN_POINT('Ctrl Pts',(4.37525483738569,-5.48537694098302,-11.5123111649174));
#24597=CARTESIAN_POINT('Ctrl Pts',(4.58558599868548,-5.31080185230311,-11.4997152980757));
#24598=CARTESIAN_POINT('Ctrl Pts',(4.94119644040959,-4.97873084231838,-11.4773866669656));
#24599=CARTESIAN_POINT('Ctrl Pts',(5.09046426918637,-4.82600857499741,-11.4676387417521));
#24600=CARTESIAN_POINT('Ctrl Pts',(5.37585245043567,-4.5060182196124,-11.4481798621427));
#24601=CARTESIAN_POINT('Ctrl Pts',(5.51169357637629,-4.33880463449659,-11.4384803286146));
#24602=CARTESIAN_POINT('Ctrl Pts',(5.80865010291946,-3.93676839718646,-11.4160439734009));
#24603=CARTESIAN_POINT('Ctrl Pts',(5.96358892251378,-3.69785969844857,-11.4033576605807));
#24604=CARTESIAN_POINT('Ctrl Pts',(6.15712521063663,-3.35548416189856,-11.3856306398269));
#24605=CARTESIAN_POINT('Ctrl Pts',(6.20845391045076,-3.25953441426689,-11.3807057284765));
#24606=CARTESIAN_POINT('Ctrl Pts',(6.34113915322826,-2.99698876308996,-11.3673035355086));
#24607=CARTESIAN_POINT('Ctrl Pts',(6.41815438112904,-2.82829993380119,-11.3587863707568));
#24608=CARTESIAN_POINT('Ctrl Pts',(6.57190190074028,-2.45281454952298,-11.3401230891118));
#24609=CARTESIAN_POINT('Ctrl Pts',(6.64574844918732,-2.24504401544025,-11.3299850128475));
#24610=CARTESIAN_POINT('Ctrl Pts',(6.76428428973349,-1.85404916061724,-11.3112895403224));
#24611=CARTESIAN_POINT('Ctrl Pts',(6.81160939606699,-1.67183111176069,-11.3027242322513));
#24612=CARTESIAN_POINT('Ctrl Pts',(6.90028627141531,-1.26349571513071,-11.2838083175218));
#24613=CARTESIAN_POINT('Ctrl Pts',(6.93796908099293,-1.03680230611507,-11.2734934561395));
#24614=CARTESIAN_POINT('Ctrl Pts',(6.98695277138019,-0.614941517490937,
-11.2544572438967));
#24615=CARTESIAN_POINT('Ctrl Pts',(7.00135391097328,-0.420362762101538,
-11.2457372445639));
#24616=CARTESIAN_POINT('Ctrl Pts',(7.01158185917485,-0.102432630642884,
-11.2314306546495));
#24617=CARTESIAN_POINT('Ctrl Pts',(7.01229959221733,0.0206550579174754,
-11.2258765123003));
#24618=CARTESIAN_POINT('Ctrl Pts',(7.0071533386387,0.271698113049057,-11.2144586100377));
#24619=CARTESIAN_POINT('Ctrl Pts',(7.00102386176057,0.399602346535745,-11.2085975989526));
#24620=CARTESIAN_POINT('Ctrl Pts',(6.97170942873689,0.788303666061847,-11.1907023277934));
#24621=CARTESIAN_POINT('Ctrl Pts',(6.93741857339419,1.04803609012085,-11.1786367683149));
#24622=CARTESIAN_POINT('Ctrl Pts',(6.85166451550499,1.50062109112961,-11.1575252467956));
#24623=CARTESIAN_POINT('Ctrl Pts',(6.80634892865225,1.69433951177183,-11.1484578660865));
#24624=CARTESIAN_POINT('Ctrl Pts',(6.69065690626181,2.10860529922559,-11.1289594846385));
#24625=CARTESIAN_POINT('Ctrl Pts',(6.61747176167516,2.32812710568623,-11.1185603431471));
#24626=CARTESIAN_POINT('Ctrl Pts',(6.45743457771486,2.73919845193073,-11.0987783253905));
#24627=CARTESIAN_POINT('Ctrl Pts',(6.37255542273968,2.9312465304788,-11.0893993783134));
#24628=CARTESIAN_POINT('Ctrl Pts',(6.22263804584527,3.23304210756713,-11.0742494700491));
#24629=CARTESIAN_POINT('Ctrl Pts',(6.16300002990119,3.34532743459506,-11.0685157621435));
#24630=CARTESIAN_POINT('Ctrl Pts',(6.0227182027061,3.59295041541811,-11.0555788379607));
#24631=CARTESIAN_POINT('Ctrl Pts',(5.94049956697817,3.72731687383393,-11.0483604982724));
#24632=CARTESIAN_POINT('Ctrl Pts',(5.71821977316415,4.0645170075794,-11.0298017335497));
#24633=CARTESIAN_POINT('Ctrl Pts',(5.57186124643667,4.26294491431963,-11.0184522234398));
#24634=CARTESIAN_POINT('Ctrl Pts',(5.2915524413866,4.60381313895361,-10.9982358323555));
#24635=CARTESIAN_POINT('Ctrl Pts',(5.16151752863195,4.74914320674079,-10.9893526475353));
#24636=CARTESIAN_POINT('Ctrl Pts',(4.8851564413371,5.0332333106444,-10.971393227088));
#24637=CARTESIAN_POINT('Ctrl Pts',(4.73856164040789,5.17148200532207,-10.9623288878831));
#24638=CARTESIAN_POINT('Ctrl Pts',(4.41542054660129,5.45093351673867,-10.9431587770593));
#24639=CARTESIAN_POINT('Ctrl Pts',(4.23758849946023,5.59030034277817,-10.9330718027781));
#24640=CARTESIAN_POINT('Ctrl Pts',(3.94625283975758,5.79671807991351,-10.9170256210937));
#24641=CARTESIAN_POINT('Ctrl Pts',(3.83705426030064,5.86957119018013,-10.9111087588167));
#24642=CARTESIAN_POINT('Ctrl Pts',(3.60534262314025,6.01492950884022,-10.8986788063955));
#24643=CARTESIAN_POINT('Ctrl Pts',(3.48253608698529,6.08685583711557,-10.8921630678228));
#24644=CARTESIAN_POINT('Ctrl Pts',(3.08960177350754,6.30120648873547,-10.8716076955209));
#24645=CARTESIAN_POINT('Ctrl Pts',(2.81230846483226,6.42975632135445,-10.8575366136582));
#24646=CARTESIAN_POINT('Ctrl Pts',(2.44718246039113,6.57087077794948,-10.8396404812248));
#24647=CARTESIAN_POINT('Ctrl Pts',(2.36627894206668,6.60043702284669,-10.8357120186529));
#24648=CARTESIAN_POINT('Ctrl Pts',(2.1062307121032,6.69007584689251,-10.8231972306517));
#24649=CARTESIAN_POINT('Ctrl Pts',(1.92519316392614,6.74440178678913,-10.8146552479193));
#24650=CARTESIAN_POINT('Ctrl Pts',(1.35311364546076,6.89115700034329,-10.7880694490012));
#24651=CARTESIAN_POINT('Ctrl Pts',(0.956195485671111,6.95734453454538,-10.7702412035067));
#24652=CARTESIAN_POINT('Ctrl Pts',(0.44937464068031,6.99764875429134,-10.7472274565676));
#24653=CARTESIAN_POINT('Ctrl Pts',(0.342766797865227,7.00368016451697,-10.7423651910949));
#24654=CARTESIAN_POINT('Ctrl Pts',(-0.039320008195268,7.01655207627336,
-10.724877655996));
#24655=CARTESIAN_POINT('Ctrl Pts',(-0.315011029876103,7.00958749346482,
-10.71216852385));
#24656=CARTESIAN_POINT('Ctrl Pts',(-0.810675321235539,6.96775900726511,
-10.6893281019996));
#24657=CARTESIAN_POINT('Ctrl Pts',(-1.03076777960181,6.93861515305332,-10.6791871536366));
#24658=CARTESIAN_POINT('Ctrl Pts',(-1.45398296333813,6.86199017205336,-10.6596591086824));
#24659=CARTESIAN_POINT('Ctrl Pts',(-1.65710424665962,6.81578923852454,-10.6502732128743));
#24660=CARTESIAN_POINT('Ctrl Pts',(-2.14130607810876,6.68272681845155,-10.6277204005744));
#24661=CARTESIAN_POINT('Ctrl Pts',(-2.41956113953147,6.58708973449629,-10.6146166352803));
#24662=CARTESIAN_POINT('Ctrl Pts',(-2.79304087099005,6.43185533820519,-10.5963930743974));
#24663=CARTESIAN_POINT('Ctrl Pts',(-2.89407372683863,6.387031971596,-10.5913932342474));
#24664=CARTESIAN_POINT('Ctrl Pts',(-3.15784811867006,6.26246381801166,-10.5781075853874));
#24665=CARTESIAN_POINT('Ctrl Pts',(-3.31862810849199,6.17876719680774,-10.5697849256581));
#24666=CARTESIAN_POINT('Ctrl Pts',(-3.67060749139187,5.9778332146982,-10.5511439421458));
#24667=CARTESIAN_POINT('Ctrl Pts',(-3.85979395696704,5.85746030153534,-10.5408323331279));
#24668=CARTESIAN_POINT('Ctrl Pts',(-4.19743532854404,5.61915870521632,-10.521918377674));
#24669=CARTESIAN_POINT('Ctrl Pts',(-4.34750389885634,5.50387312271211,-10.5133069374932));
#24670=CARTESIAN_POINT('Ctrl Pts',(-4.7257601169692,5.18815511995088,-10.4909989556166));
#24671=CARTESIAN_POINT('Ctrl Pts',(-4.94591634291057,4.97872241369126,-10.4774095892723));
#24672=CARTESIAN_POINT('Ctrl Pts',(-5.29023740070518,4.60572096020231,-10.4546664246096));
#24673=CARTESIAN_POINT('Ctrl Pts',(-5.42205176708675,4.44978988892693,-10.4455247372652));
#24674=CARTESIAN_POINT('Ctrl Pts',(-5.61189601397819,4.20423011722575,-10.4314767152607));
#24675=CARTESIAN_POINT('Ctrl Pts',(-5.67499471690442,4.11866021873803,-10.4266362406227));
#24676=CARTESIAN_POINT('Ctrl Pts',(-5.89460916821788,3.80620180057507,-10.4091685497005));
#24677=CARTESIAN_POINT('Ctrl Pts',(-6.03966144402538,3.57156529511606,-10.3964560552845));
#24678=CARTESIAN_POINT('Ctrl Pts',(-6.27631161660821,3.13291851302716,-10.3735691741923));
#24679=CARTESIAN_POINT('Ctrl Pts',(-6.3726930321161,2.93190242993521,-10.3633857936126));
#24680=CARTESIAN_POINT('Ctrl Pts',(-6.54008166079987,2.53536257424353,-10.3438421304199));
#24681=CARTESIAN_POINT('Ctrl Pts',(-6.61228777266003,2.34059474568933,-10.3344820717728));
#24682=CARTESIAN_POINT('Ctrl Pts',(-6.7658330343885,1.86225927027523,-10.3119181647198));
#24683=CARTESIAN_POINT('Ctrl Pts',(-6.83813304456533,1.57621081751037,-10.2987786156168));
#24684=CARTESIAN_POINT('Ctrl Pts',(-6.912525049042,1.17765687240146,-10.28051146429));
#24685=CARTESIAN_POINT('Ctrl Pts',(-6.93025477348721,1.06838512787543,-10.2755041151218));
#24686=CARTESIAN_POINT('Ctrl Pts',(-6.97212850224025,0.765039264511157,
-10.2615578922025));
#24687=CARTESIAN_POINT('Ctrl Pts',(-6.99075163635057,0.570307879520168,
-10.2525712455192));
#24688=CARTESIAN_POINT('Ctrl Pts',(-7.01283237363221,0.158123628128352,
-10.2335834381316));
#24689=CARTESIAN_POINT('Ctrl Pts',(-7.01436481487391,-0.0592325604935013,
-10.2235916143769));
#24690=CARTESIAN_POINT('Ctrl Pts',(-6.99841766858817,-0.463571089965065,
-10.2050784079148));
#24691=CARTESIAN_POINT('Ctrl Pts',(-6.98352685073223,-0.650463154832566,
-10.1965501317857));
#24692=CARTESIAN_POINT('Ctrl Pts',(-6.92956514944857,-1.0995011646996,-10.176079382904));
#24693=CARTESIAN_POINT('Ctrl Pts',(-6.88308868415413,-1.36046633352886,
-10.1642035884737));
#24694=CARTESIAN_POINT('Ctrl Pts',(-6.78251461914111,-1.78446933768445,
-10.1446799121039));
#24695=CARTESIAN_POINT('Ctrl Pts',(-6.73700313116651,-1.94926231142541,
-10.1370307867779));
#24696=CARTESIAN_POINT('Ctrl Pts',(-6.65051118328972,-2.22302242034616,
-10.1241073063752));
#24697=CARTESIAN_POINT('Ctrl Pts',(-6.612758016824,-2.33292923210549,-10.1188574485144));
#24698=CARTESIAN_POINT('Ctrl Pts',(-6.5722843992401,-2.44186493044116,-10.11356916409));
#24699=CARTESIAN_POINT('Ctrl Pts',(-6.57227799727717,-2.44188216123224,
-10.1135683276261));
#24700=CARTESIAN_POINT('Ctrl Pts',(-6.57227159525839,-2.44189939200199,
-10.1135674911542));
#24701=CARTESIAN_POINT('Origin',(0.,0.,0.));
#24702=CARTESIAN_POINT('',(-7.01125010206304,-6.30148839881794E-5,-8.22678883376454));
#24703=CARTESIAN_POINT('Ctrl Pts',(-6.57227159525839,-2.44189939200199,
-10.1135674911542));
#24704=CARTESIAN_POINT('Ctrl Pts',(-6.55563335767533,-2.48668052287923,
-10.111393580184));
#24705=CARTESIAN_POINT('Ctrl Pts',(-6.53853794377912,-2.53129023612478,
-10.1092142556917));
#24706=CARTESIAN_POINT('Ctrl Pts',(-6.41893712906644,-2.83408518985237,
-10.0943340971301));
#24707=CARTESIAN_POINT('Ctrl Pts',(-6.3016220842915,-3.08615476115843,-10.0815210439367));
#24708=CARTESIAN_POINT('Ctrl Pts',(-6.06202586012092,-3.52998740057746,
-10.0583555983445));
#24709=CARTESIAN_POINT('Ctrl Pts',(-5.94478479856127,-3.72404414589833,
-10.0479961152748));
#24710=CARTESIAN_POINT('Ctrl Pts',(-5.70373976967903,-4.08254476599991,
-10.0283774784473));
#24711=CARTESIAN_POINT('Ctrl Pts',(-5.58169100795926,-4.24788728897974,
-10.0191146389423));
#24712=CARTESIAN_POINT('Ctrl Pts',(-5.27144447599857,-4.63168439768932,
-9.99694473763417));
#24713=CARTESIAN_POINT('Ctrl Pts',(-5.07669470879712,-4.84435717107434,
-9.98409851500608));
#24714=CARTESIAN_POINT('Ctrl Pts',(-4.78639664337701,-5.12458273860975,
-9.96593391436084));
#24715=CARTESIAN_POINT('Ctrl Pts',(-4.7014129183229,-5.20265868213545,-9.96071963443434));
#24716=CARTESIAN_POINT('Ctrl Pts',(-4.4549021696597,-5.41815774778652,-9.94581838120971));
#24717=CARTESIAN_POINT('Ctrl Pts',(-4.2890166544668,-5.5503982846688,-9.93606963252502));
#24718=CARTESIAN_POINT('Ctrl Pts',(-3.86676039241555,-5.8567633677391,-9.91207036463691));
#24719=CARTESIAN_POINT('Ctrl Pts',(-3.60434923938149,-6.02180911091854,
-9.89785023588188));
#24720=CARTESIAN_POINT('Ctrl Pts',(-3.1651642018583,-6.25901484236853,-9.87514223515454));
#24721=CARTESIAN_POINT('Ctrl Pts',(-2.99485896822553,-6.34226714362656,
-9.86657638642382));
#24722=CARTESIAN_POINT('Ctrl Pts',(-2.61507429412999,-6.50920912463532,
-9.84790366541906));
#24723=CARTESIAN_POINT('Ctrl Pts',(-2.40450649183683,-6.58989879715603,
-9.83782428806167));
#24724=CARTESIAN_POINT('Ctrl Pts',(-2.01692711283363,-6.71736453849948,
-9.81953794502612));
#24725=CARTESIAN_POINT('Ctrl Pts',(-1.84127461696467,-6.76762052275582,
-9.81134411052068));
#24726=CARTESIAN_POINT('Ctrl Pts',(-1.55412979117488,-6.83776770478043,
-9.7979524202195));
#24727=CARTESIAN_POINT('Ctrl Pts',(-1.44376664335993,-6.86191836181938,
-9.79280089508966));
#24728=CARTESIAN_POINT('Ctrl Pts',(-1.25334026162923,-6.89879169823925,
-9.78391936223826));
#24729=CARTESIAN_POINT('Ctrl Pts',(-1.17354982764886,-6.91281197550355,
-9.7802005893264));
#24730=CARTESIAN_POINT('Ctrl Pts',(-0.705750967202534,-6.98667787123912,
-9.75843382213963));
#24731=CARTESIAN_POINT('Ctrl Pts',(-0.313500584881129,-7.01523200327381,
-9.74037191885143));
#24732=CARTESIAN_POINT('Ctrl Pts',(0.280420151652584,-7.00853306035149,
-9.71338916156268));
#24733=CARTESIAN_POINT('Ctrl Pts',(0.481574664993027,-6.99758949172561,
-9.70430441878386));
#24734=CARTESIAN_POINT('Ctrl Pts',(0.95260313791147,-6.9515544839368,-9.68303561153323));
#24735=CARTESIAN_POINT('Ctrl Pts',(1.22145652174268,-6.90938533445735,-9.67090314030905));
#24736=CARTESIAN_POINT('Ctrl Pts',(1.61327646506455,-6.82433990681331,-9.65288084223265));
#24737=CARTESIAN_POINT('Ctrl Pts',(1.73859288307059,-6.79349470790795,-9.64706217086139));
#24738=CARTESIAN_POINT('Ctrl Pts',(2.01545571210786,-6.71718527644208,-9.63400956044661));
#24739=CARTESIAN_POINT('Ctrl Pts',(2.16645881854833,-6.67001460852423,-9.62676075780371));
#24740=CARTESIAN_POINT('Ctrl Pts',(2.69208767817669,-6.48608318937639,-9.60117141413292));
#24741=CARTESIAN_POINT('Ctrl Pts',(3.05652837817457,-6.32251978427163,-9.58282128894232));
#24742=CARTESIAN_POINT('Ctrl Pts',(3.5805204509342,-6.03139919028621,-9.55558821791589));
#24743=CARTESIAN_POINT('Ctrl Pts',(3.75168865020004,-5.92644386509312,-9.54653277069493));
#24744=CARTESIAN_POINT('Ctrl Pts',(4.14136661308595,-5.66384856685306,-9.52541413758718));
#24745=CARTESIAN_POINT('Ctrl Pts',(4.35576251628872,-5.50067543964145,-9.51340103279229));
#24746=CARTESIAN_POINT('Ctrl Pts',(4.66028882435961,-5.23991246658184,-9.49538413119836));
#24747=CARTESIAN_POINT('Ctrl Pts',(4.75789932949773,-5.15144328518606,-9.48944655333741));
#24748=CARTESIAN_POINT('Ctrl Pts',(4.96341591729386,-4.9543467014069,-9.47650705728897));
#24749=CARTESIAN_POINT('Ctrl Pts',(5.0703737113548,-4.84482798698939,-9.46949514487592));
#24750=CARTESIAN_POINT('Ctrl Pts',(5.45231069957782,-4.42723400922561,-9.4434963473546));
#24751=CARTESIAN_POINT('Ctrl Pts',(5.70351170441368,-4.09854357678903,-9.42449176193967));
#24752=CARTESIAN_POINT('Ctrl Pts',(6.03445099074402,-3.57567158865056,-9.39639098283425));
#24753=CARTESIAN_POINT('Ctrl Pts',(6.1368564923759,-3.39691334474483,-9.38710600788273));
#24754=CARTESIAN_POINT('Ctrl Pts',(6.37386387744646,-2.93739410744932,-9.36388012990598));
#24755=CARTESIAN_POINT('Ctrl Pts',(6.49791627700228,-2.65169869899579,-9.35001900094283));
#24756=CARTESIAN_POINT('Ctrl Pts',(6.63853016122665,-2.25808803434898,-9.33116932537813));
#24757=CARTESIAN_POINT('Ctrl Pts',(6.67217196427409,-2.15665603610392,-9.32632901535657));
#24758=CARTESIAN_POINT('Ctrl Pts',(6.76615056285521,-1.8500190400043,-9.31171019861519));
#24759=CARTESIAN_POINT('Ctrl Pts',(6.81942950598095,-1.64278532518974,-9.30187078375111));
#24760=CARTESIAN_POINT('Ctrl Pts',(6.9222311681217,-1.15058339330296,-9.27873901870707));
#24761=CARTESIAN_POINT('Ctrl Pts',(6.96376700641256,-0.864337889488257,
-9.26547632847848));
#24762=CARTESIAN_POINT('Ctrl Pts',(7.00300674771778,-0.388600837142123,
-9.24375578175975));
#24763=CARTESIAN_POINT('Ctrl Pts',(7.01091952486046,-0.200307405732222,
-9.23523773149981));
#24764=CARTESIAN_POINT('Ctrl Pts',(7.01161579047083,0.209153460630078,-9.21680406891329));
#24765=CARTESIAN_POINT('Ctrl Pts',(7.00153522190699,0.430123696089627,-9.20691390519347));
#24766=CARTESIAN_POINT('Ctrl Pts',(6.96403781339354,0.832693826912152,-9.18879542482949));
#24767=CARTESIAN_POINT('Ctrl Pts',(6.93989847695447,1.014400966877,-9.18057828843107));
#24768=CARTESIAN_POINT('Ctrl Pts',(6.89017627245457,1.30187235700103,-9.16737181638197));
#24769=CARTESIAN_POINT('Ctrl Pts',(6.86920351563081,1.40834760948636,-9.16242929894401));
#24770=CARTESIAN_POINT('Ctrl Pts',(6.78347668282857,1.79589911175014,-9.14427005405975));
#24771=CARTESIAN_POINT('Ctrl Pts',(6.70386803052358,2.07339406830289,-9.13096379629836));
#24772=CARTESIAN_POINT('Ctrl Pts',(6.53588682206941,2.54666731055961,-9.10791621983581));
#24773=CARTESIAN_POINT('Ctrl Pts',(6.45519931774765,2.74476499860548,-9.0981521436679));
#24774=CARTESIAN_POINT('Ctrl Pts',(6.27548975344534,3.13401577183411,-9.07869431602202));
#24775=CARTESIAN_POINT('Ctrl Pts',(6.17646680089845,3.32491899544151,-9.06901150243526));
#24776=CARTESIAN_POINT('Ctrl Pts',(5.93134215313975,3.74862480713826,-9.04703752610336));
#24777=CARTESIAN_POINT('Ctrl Pts',(5.78001485511577,3.97799374004855,-9.03479021895633));
#24778=CARTESIAN_POINT('Ctrl Pts',(5.54821455374222,4.28807877898038,-9.01735324692611));
#24779=CARTESIAN_POINT('Ctrl Pts',(5.47863802335601,4.37662307020571,-9.01226206298247));
#24780=CARTESIAN_POINT('Ctrl Pts',(5.37570018846381,4.50132036251301,-9.00490030870556));
#24781=CARTESIAN_POINT('Ctrl Pts',(5.34404473071823,4.53885705819345,-9.00265923001823));
#24782=CARTESIAN_POINT('Ctrl Pts',(5.12694212953571,4.79087496069243,-8.98744851412553));
#24783=CARTESIAN_POINT('Ctrl Pts',(4.92902658467874,4.99426822366104,-8.97436853820447));
#24784=CARTESIAN_POINT('Ctrl Pts',(4.55674781695201,5.33310535803238,-8.95125703918073));
#24785=CARTESIAN_POINT('Ctrl Pts',(4.38728197398616,5.47336483820739,-8.94121047947184));
#24786=CARTESIAN_POINT('Ctrl Pts',(4.04390378753554,5.73135369943985,-8.92171158334063));
#24787=CARTESIAN_POINT('Ctrl Pts',(3.87073839523873,5.84969736142594,-8.91226270498881));
#24788=CARTESIAN_POINT('Ctrl Pts',(3.43350890392148,6.12057893841721,-8.88916505283293));
#24789=CARTESIAN_POINT('Ctrl Pts',(3.16430536709535,6.26399541566597,-8.87558698468384));
#24790=CARTESIAN_POINT('Ctrl Pts',(2.789634337494,6.43326475561664,-8.85704322678649));
#24791=CARTESIAN_POINT('Ctrl Pts',(2.69165471315347,6.47487063609521,-8.8522208972402));
#24792=CARTESIAN_POINT('Ctrl Pts',(2.38880518474176,6.5954094766982,-8.83736128479388));
#24793=CARTESIAN_POINT('Ctrl Pts',(2.18114659618961,6.66696440665183,-8.82725894919786));
#24794=CARTESIAN_POINT('Ctrl Pts',(1.70104760554312,6.80756055696294,-8.80424551429163));
#24795=CARTESIAN_POINT('Ctrl Pts',(1.42711977915363,6.87020937909845,-8.79136282604805));
#24796=CARTESIAN_POINT('Ctrl Pts',(0.964729005599117,6.94710477029025,-8.77003258608758));
#24797=CARTESIAN_POINT('Ctrl Pts',(0.778118931541352,6.97047338331969,-8.7615314565525));
#24798=CARTESIAN_POINT('Ctrl Pts',(0.372032776105765,7.00481382531203,-8.74318308313487));
#24799=CARTESIAN_POINT('Ctrl Pts',(0.152523207717786,7.01302805488468,-8.73336056114841));
#24800=CARTESIAN_POINT('Ctrl Pts',(-0.255093735997572,7.00913207491632,
-8.71509397123718));
#24801=CARTESIAN_POINT('Ctrl Pts',(-0.443026827528892,6.99976648781566,
-8.70666039633668));
#24802=CARTESIAN_POINT('Ctrl Pts',(-0.739205899390721,6.97302995026178,
-8.69319613520645));
#24803=CARTESIAN_POINT('Ctrl Pts',(-0.847811881451378,6.96065990185586,
-8.68821651691027));
#24804=CARTESIAN_POINT('Ctrl Pts',(-1.10115160496994,6.92578771184345,-8.67651474288063));
#24805=CARTESIAN_POINT('Ctrl Pts',(-1.24555854211707,6.90127914005917,-8.66978183452009));
#24806=CARTESIAN_POINT('Ctrl Pts',(-1.6965882160546,6.81011252961119,-8.64861386731157));
#24807=CARTESIAN_POINT('Ctrl Pts',(-1.99957181749221,6.72738896653651,-8.6342056381497));
#24808=CARTESIAN_POINT('Ctrl Pts',(-2.47522606033523,6.56253486470539,-8.61130446702736));
#24809=CARTESIAN_POINT('Ctrl Pts',(-2.6518612157142,6.4931688361686,-8.60272984697376));
#24810=CARTESIAN_POINT('Ctrl Pts',(-3.03244035341468,6.32558894609971,-8.58401350154332));
#24811=CARTESIAN_POINT('Ctrl Pts',(-3.23488275015577,6.22449228667035,-8.57389964625463));
#24812=CARTESIAN_POINT('Ctrl Pts',(-3.59172571577048,6.02417207540035,-8.55555795444338));
#24813=CARTESIAN_POINT('Ctrl Pts',(-3.74779294308549,5.92833781657103,-8.54734360653233));
#24814=CARTESIAN_POINT('Ctrl Pts',(-3.9949918017487,5.76287713868979,-8.53386417815342));
#24815=CARTESIAN_POINT('Ctrl Pts',(-4.0884820789298,5.69693126292727,-8.5286456931841));
#24816=CARTESIAN_POINT('Ctrl Pts',(-4.31251610888672,5.53054681420163,-8.51586474445184));
#24817=CARTESIAN_POINT('Ctrl Pts',(-4.44121611984323,5.42773822158121,-8.50828693144187));
#24818=CARTESIAN_POINT('Ctrl Pts',(-4.77596570287999,5.14044808101262,-8.48799427053341));
#24819=CARTESIAN_POINT('Ctrl Pts',(-4.97492530895604,4.94814884130974,-8.47530973672958));
#24820=CARTESIAN_POINT('Ctrl Pts',(-5.2802353770552,4.61597897585171,-8.4547785319961));
#24821=CARTESIAN_POINT('Ctrl Pts',(-5.39361110877686,4.48297981094963,-8.44687395943722));
#24822=CARTESIAN_POINT('Ctrl Pts',(-5.63059353851227,4.18295934452165,-8.42964890297838));
#24823=CARTESIAN_POINT('Ctrl Pts',(-5.75198548675074,4.01439861804166,-8.42035171723981));
#24824=CARTESIAN_POINT('Ctrl Pts',(-5.98243789605577,3.66243952240189,-8.40150402343384));
#24825=CARTESIAN_POINT('Ctrl Pts',(-6.09096905111159,3.47895390888411,-8.39196295792931));
#24826=CARTESIAN_POINT('Ctrl Pts',(-6.23954140183416,3.19944627405982,-8.37763249214173));
#24827=CARTESIAN_POINT('Ctrl Pts',(-6.28607848509906,3.10701624938916,-8.3729202728785));
#24828=CARTESIAN_POINT('Ctrl Pts',(-6.48211764129864,2.69520323707306,-8.35206011545531));
#24829=CARTESIAN_POINT('Ctrl Pts',(-6.60944788205276,2.36583402036228,-8.33577429286849));
#24830=CARTESIAN_POINT('Ctrl Pts',(-6.76653161101002,1.84605459556445,-8.31091754506932));
#24831=CARTESIAN_POINT('Ctrl Pts',(-6.81415978112026,1.66165451476764,-8.30224882221859));
#24832=CARTESIAN_POINT('Ctrl Pts',(-6.95861947812567,0.990607171095191,
-8.27116381837615));
#24833=CARTESIAN_POINT('Ctrl Pts',(-7.01125445605145,0.495969930371231,
-8.24920677116425));
#24834=CARTESIAN_POINT('Ctrl Pts',(-7.01124999971706,-6.29887116476713E-5,
-8.22678901229957));
#24835=CARTESIAN_POINT('Ctrl Pts',(-7.01124999971675,-6.30228819856011E-5,
-8.22678901075528));
#24836=CARTESIAN_POINT('Ctrl Pts',(-7.01124918132822,-0.0911081541651411,
-8.22267430843915));
#24837=CARTESIAN_POINT('Ctrl Pts',(-7.00947497633958,-0.182142925889114,
-8.21854073419977));
#24838=CARTESIAN_POINT('Ctrl Pts',(-6.99953685041428,-0.437072884344599,
-8.20690147196852));
#24839=CARTESIAN_POINT('Ctrl Pts',(-6.98739183713415,-0.600752281441517,
-8.19936374275353));
#24840=CARTESIAN_POINT('Ctrl Pts',(-6.94396893096349,-0.996949710207563,
-8.18103189759171));
#24841=CARTESIAN_POINT('Ctrl Pts',(-6.90674368593749,-1.22861973404632,
-8.17024318619145));
#24842=CARTESIAN_POINT('Ctrl Pts',(-6.82218699227048,-1.62635116379858,
-8.15164360482691));
#24843=CARTESIAN_POINT('Ctrl Pts',(-6.78020561589611,-1.7933394799414,-8.14380870973982));
#24844=CARTESIAN_POINT('Ctrl Pts',(-6.6846911651413,-2.12164026690506,-8.12832257698379));
#24845=CARTESIAN_POINT('Ctrl Pts',(-6.63136950661576,-2.28283978608511,
-8.12067770055383));
#24846=CARTESIAN_POINT('Ctrl Pts',(-6.57227165853301,-2.44189922170096,
-8.11305756739085));
#24847=CARTESIAN_POINT('',(-7.01083548104182,7.7386374966269E-5,-8.77353436264612));
#24848=CARTESIAN_POINT('Ctrl Pts',(-6.57227159525839,-2.441899392002,-8.66029439624775));
#24849=CARTESIAN_POINT('Ctrl Pts',(-6.62943398574475,-2.28804917338076,
-8.66774640904247));
#24850=CARTESIAN_POINT('Ctrl Pts',(-6.6811857121734,-2.13220727019073,-8.67519842183719));
#24851=CARTESIAN_POINT('Ctrl Pts',(-6.72740127611852,-1.97476546267625,
-8.68265043463192));
#24852=CARTESIAN_POINT('Ctrl Pts',(-6.78061673854497,-1.79347721523458,
-8.6912311436621));
#24853=CARTESIAN_POINT('Ctrl Pts',(-6.82650811549892,-1.61000928425161,
-8.69981185269229));
#24854=CARTESIAN_POINT('Ctrl Pts',(-6.86491797772433,-1.42496586682535,
-8.70839256172248));
#24855=CARTESIAN_POINT('Ctrl Pts',(-6.90331958581666,-1.23996221452462,
-8.71697142679098));
#24856=CARTESIAN_POINT('Ctrl Pts',(-6.93424282786693,-1.05338404397609,
-8.72555029185948));
#24857=CARTESIAN_POINT('Ctrl Pts',(-6.9575812067861,-0.865846587726097,
-8.73412915692798));
#24858=CARTESIAN_POINT('Ctrl Pts',(-6.98091698638194,-0.678330018551714,
-8.74270706652121));
#24859=CARTESIAN_POINT('Ctrl Pts',(-6.99666955104869,-0.489854673144777,
-8.75128497611443));
#24860=CARTESIAN_POINT('Ctrl Pts',(-7.004784073487,-0.301042598850843,-8.75986288570765));
#24861=CARTESIAN_POINT('Ctrl Pts',(-7.00909504842534,-0.200733045636199,
-8.76442004277522));
#24862=CARTESIAN_POINT('Ctrl Pts',(-7.01125110605494,-0.100328544295878,
-8.7689771998428));
#24863=CARTESIAN_POINT('Ctrl Pts',(-7.01124999957427,7.72645793954891E-5,
-8.77353435691037));
#24864=CARTESIAN_POINT('Ctrl Pts',(-7.01071564309632,7.7421586253174E-5,
-8.77353436430433));
#24865=CARTESIAN_POINT('Ctrl Pts',(-7.01090830760592,0.492725215260218,
-8.79589606338762));
#24866=CARTESIAN_POINT('Ctrl Pts',(-6.83913257993509,2.14530585228538,-8.87091410477835));
#24867=CARTESIAN_POINT('Ctrl Pts',(-5.55442723662985,4.7455628683187,-8.99858848847648));
#24868=CARTESIAN_POINT('Ctrl Pts',(-2.62474354776125,6.81782592049443,-9.1565575153988));
#24869=CARTESIAN_POINT('Ctrl Pts',(0.938224379280063,7.24511999742928,-9.31452654232106));
#24870=CARTESIAN_POINT('Ctrl Pts',(4.2748224808499,5.92434990752088,-9.47249556924337));
#24871=CARTESIAN_POINT('Ctrl Pts',(6.58001406404274,3.17418394776362,-9.63046459616565));
#24872=CARTESIAN_POINT('Ctrl Pts',(7.29761463056158,-0.341832161412208,
-9.78843362308794));
#24873=CARTESIAN_POINT('Ctrl Pts',(6.25448545643946,-3.77537311475419,-9.94640265001023));
#24874=CARTESIAN_POINT('Ctrl Pts',(3.70230695067219,-6.29801144386563,-10.1043716769325));
#24875=CARTESIAN_POINT('Ctrl Pts',(0.256855774125145,-7.30110003209896,
-10.2623407038548));
#24876=CARTESIAN_POINT('Ctrl Pts',(-3.25056889473619,-6.54261565608652,
-10.4203097307771));
#24877=CARTESIAN_POINT('Ctrl Pts',(-5.53729420238302,-4.5801091614773,-10.5529622341764));
#24878=CARTESIAN_POINT('Ctrl Pts',(-6.36188242840926,-3.00629425112275,
-10.6329583952682));
#24879=CARTESIAN_POINT('Ctrl Pts',(-6.57172397189039,-2.44169584043291,
-10.6602982140526));
#24880=CARTESIAN_POINT('Origin',(0.,0.,-16.4167025567876));
#24881=CARTESIAN_POINT('',(-8.12521368785635,8.95665403536892E-5,-9.41670255780532));
#24882=CARTESIAN_POINT('Ctrl Pts',(4.94675008185374,-6.44587862049698,-10.7083437636031));
#24883=CARTESIAN_POINT('Ctrl Pts',(5.11324386102303,-6.31810657199534,-10.7001223210038));
#24884=CARTESIAN_POINT('Ctrl Pts',(5.27479811987266,-6.18387000071871,-10.6919008784046));
#24885=CARTESIAN_POINT('Ctrl Pts',(5.43091827111027,-6.04357628354442,-10.6836794358054));
#24886=CARTESIAN_POINT('Ctrl Pts',(5.58704849341192,-5.90327351624432,-10.6754574628539));
#24887=CARTESIAN_POINT('Ctrl Pts',(5.73774368584835,-5.75691301674722,-10.6672354899024));
#24888=CARTESIAN_POINT('Ctrl Pts',(5.88254383657361,-5.60494117482867,-10.659013516951));
#24889=CARTESIAN_POINT('Ctrl Pts',(6.0273393179283,-5.45297423354623,-10.6507918091335));
#24890=CARTESIAN_POINT('Ctrl Pts',(6.16623993542932,-5.29539652637689,-10.6425701013159));
#24891=CARTESIAN_POINT('Ctrl Pts',(6.29882356643554,-5.13269025379637,-10.6343483934984));
#24892=CARTESIAN_POINT('Ctrl Pts',(6.43143852287547,-4.96994553872851,-10.6261247431443));
#24893=CARTESIAN_POINT('Ctrl Pts',(6.55773332306666,-4.80207006492447,-10.6179010927901));
#24894=CARTESIAN_POINT('Ctrl Pts',(6.67732631326922,-4.6295789083482,-10.6096774424359));
#24895=CARTESIAN_POINT('Ctrl Pts',(6.77479347290812,-4.48900024177382,-10.6029752449198));
#24896=CARTESIAN_POINT('Ctrl Pts',(6.86780994836343,-4.34535645822659,-10.5962730474036));
#24897=CARTESIAN_POINT('Ctrl Pts',(6.95619037540507,-4.19894070256081,-10.5895708498875));
#24898=CARTESIAN_POINT('Ctrl Pts',(7.06463232354457,-4.01928995505725,-10.5813473169199));
#24899=CARTESIAN_POINT('Ctrl Pts',(7.16612867057859,-3.83540684465529,-10.5731237839523));
#24900=CARTESIAN_POINT('Ctrl Pts',(7.26036397147166,-3.64784903254729,-10.5649002509847));
#24901=CARTESIAN_POINT('Ctrl Pts',(7.35458213776429,-3.46032532366962,-10.5566782132843));
#24902=CARTESIAN_POINT('Ctrl Pts',(7.44154176065796,-3.26912851007378,-10.5484561755839));
#24903=CARTESIAN_POINT('Ctrl Pts',(7.52097373826056,-3.07484009192265,-10.5402341378835));
#24904=CARTESIAN_POINT('Ctrl Pts',(7.60039694531601,-2.88057312628707,-10.5320130080261));
#24905=CARTESIAN_POINT('Ctrl Pts',(7.67229405491373,-2.68321551050786,-10.5237918781687));
#24906=CARTESIAN_POINT('Ctrl Pts',(7.73644411056134,-2.48336869728615,-10.5155707483114));
#24907=CARTESIAN_POINT('Ctrl Pts',(7.80059925389462,-2.28350603438582,-10.5073489664433));
#24908=CARTESIAN_POINT('Ctrl Pts',(7.85700602295709,-2.08115405960809,-10.4991271845752));
#24909=CARTESIAN_POINT('Ctrl Pts',(7.90549302236132,-1.87693037587877,-10.4909054027071));
#24910=CARTESIAN_POINT('Ctrl Pts',(7.95397988712744,-1.67270725923533,-10.4826836436692));
#24911=CARTESIAN_POINT('Ctrl Pts',(7.99454696072024,-1.46661273161586,-10.4744618846312));
#24912=CARTESIAN_POINT('Ctrl Pts',(8.02707363735951,-1.25927613449469,-10.4662401255933));
#24913=CARTESIAN_POINT('Ctrl Pts',(8.05960709533697,-1.05189631071383,-10.4580166524384));
#24914=CARTESIAN_POINT('Ctrl Pts',(8.08409676186509,-0.843274191539016,
-10.4497931792834));
#24915=CARTESIAN_POINT('Ctrl Pts',(8.10047357116718,-0.634046910978997,
-10.4415697061285));
#24916=CARTESIAN_POINT('Ctrl Pts',(8.1070904883195,-0.549510322933475,-10.4382470784074));
#24917=CARTESIAN_POINT('Ctrl Pts',(8.11238357345324,-0.464875002095556,
-10.4349244506863));
#24918=CARTESIAN_POINT('Ctrl Pts',(8.11635067845989,-0.380183148973766,
-10.4316018229652));
#24919=CARTESIAN_POINT('Ctrl Pts',(8.12616931096018,-0.170569796118993,
-10.4233782794809));
#24920=CARTESIAN_POINT('Ctrl Pts',(8.12786496895076,0.039458169528622,-10.4151547359967));
#24921=CARTESIAN_POINT('Ctrl Pts',(8.12142579447583,0.249260159918624,-10.4069311925124));
#24922=CARTESIAN_POINT('Ctrl Pts',(8.11498779070991,0.459024006120668,-10.3987091441541));
#24923=CARTESIAN_POINT('Ctrl Pts',(8.10041791543133,0.668561664416116,-10.3904870957957));
#24924=CARTESIAN_POINT('Ctrl Pts',(8.07775641410193,0.877233650138387,-10.3822650474373));
#24925=CARTESIAN_POINT('Ctrl Pts',(8.0550974146648,1.08588259789764,-10.3740439068158));
#24926=CARTESIAN_POINT('Ctrl Pts',(8.02434860452279,1.29366577079501,-10.3658227661942));
#24927=CARTESIAN_POINT('Ctrl Pts',(7.98560206685205,1.49994906326457,-10.3576016255727));
#24928=CARTESIAN_POINT('Ctrl Pts',(7.94685245586464,1.70624871781239,-10.3493798328627));
#24929=CARTESIAN_POINT('Ctrl Pts',(7.90010390166676,1.91104796386036,-10.3411580401528));
#24930=CARTESIAN_POINT('Ctrl Pts',(7.84549975958371,2.11372209262994,-10.3329362474428));
#24931=CARTESIAN_POINT('Ctrl Pts',(7.7908957689595,2.31639565922995,-10.3247144775382));
#24932=CARTESIAN_POINT('Ctrl Pts',(7.72843631336478,2.51694383626728,-10.3164927076335));
#24933=CARTESIAN_POINT('Ctrl Pts',(7.658314999941,2.71475577615717,-10.3082709377288));
#24934=CARTESIAN_POINT('Ctrl Pts',(7.58817906754253,2.91260895611515,-10.3000474537398));
#24935=CARTESIAN_POINT('Ctrl Pts',(7.5103781848199,3.10772448128915,-10.2918239697508));
#24936=CARTESIAN_POINT('Ctrl Pts',(7.42515499169712,3.29950919255808,-10.2836004857617));
#24937=CARTESIAN_POINT('Ctrl Pts',(7.39072196440478,3.37699664586041,-10.2802779225221));
#24938=CARTESIAN_POINT('Ctrl Pts',(7.35507784413455,3.45394059557975,-10.2769553592825));
#24939=CARTESIAN_POINT('Ctrl Pts',(7.31824083470829,3.53030291160804,-10.2736327960429));
#24940=CARTESIAN_POINT('Ctrl Pts',(7.22706710013741,3.71930407215873,-10.2654092593437));
#24941=CARTESIAN_POINT('Ctrl Pts',(7.12855291764284,3.90480206002756,-10.2571857226446));
#24942=CARTESIAN_POINT('Ctrl Pts',(7.02299287655094,4.08622792051726,-10.2489621859455));
#24943=CARTESIAN_POINT('Ctrl Pts',(6.91745202847966,4.26762079399552,-10.2407401444571));
#24944=CARTESIAN_POINT('Ctrl Pts',(6.80486802695956,4.44494276304557,-10.2325181029687));
#24945=CARTESIAN_POINT('Ctrl Pts',(6.68558075375882,4.61765065238479,-10.2242960614803));
#24946=CARTESIAN_POINT('Ctrl Pts',(6.5663066511169,4.79033947297213,-10.2160749277911));
#24947=CARTESIAN_POINT('Ctrl Pts',(6.44033092194771,4.95841498834916,-10.2078537941018));
#24948=CARTESIAN_POINT('Ctrl Pts',(6.3080364709158,5.12136343604866,-10.1996326604125));
#24949=CARTESIAN_POINT('Ctrl Pts',(6.17573152713792,5.28432480777221,-10.1914108746758));
#24950=CARTESIAN_POINT('Ctrl Pts',(6.03710704397904,5.44215806865236,-10.183189088939));
#24951=CARTESIAN_POINT('Ctrl Pts',(5.89258653862695,5.59438213275536,-10.1749673032022));
#24952=CARTESIAN_POINT('Ctrl Pts',(5.7480664343292,5.74660577442613,-10.1667455402815));
#24953=CARTESIAN_POINT('Ctrl Pts',(5.59765054558968,5.89322003842304,-10.1585237773607));
#24954=CARTESIAN_POINT('Ctrl Pts',(5.44179997913404,6.0337799553511,-10.15030201444));
#24955=CARTESIAN_POINT('Ctrl Pts',(5.2859169201942,6.17436917689437,-10.1420785374061));
#24956=CARTESIAN_POINT('Ctrl Pts',(5.12459713908876,6.30890133221201,-10.1338550603722));
#24957=CARTESIAN_POINT('Ctrl Pts',(4.95833643774039,6.43697035356509,-10.1256315833383));
#24958=CARTESIAN_POINT('Ctrl Pts',(4.89116064434143,6.48871522201236,-10.1223089785991));
#24959=CARTESIAN_POINT('Ctrl Pts',(4.82317863122845,6.53940546242915,-10.1189863738598));
#24960=CARTESIAN_POINT('Ctrl Pts',(4.75442456323024,6.58901621147292,-10.1156637691206));
#24961=CARTESIAN_POINT('Ctrl Pts',(4.58425631376351,6.71180420882794,-10.1074402290653));
#24962=CARTESIAN_POINT('Ctrl Pts',(4.40930119041436,6.82801646716751,-10.0992166890101));
#24963=CARTESIAN_POINT('Ctrl Pts',(4.23008915387307,6.93729293837196,-10.0909931489548));
#24964=CARTESIAN_POINT('Ctrl Pts',(4.05090970095194,7.04654954136275,-10.0827711040709));
#24965=CARTESIAN_POINT('Ctrl Pts',(3.86747513129313,7.14887272063463,-10.074549059187));
#24966=CARTESIAN_POINT('Ctrl Pts',(3.6803429591141,7.24394666364954,-10.0663270143031));
#24967=CARTESIAN_POINT('Ctrl Pts',(3.49323144762652,7.33901010984084,-10.0581058771901));
#24968=CARTESIAN_POINT('Ctrl Pts',(3.30242341149901,7.42682578413742,-10.049884740077));
#24969=CARTESIAN_POINT('Ctrl Pts',(3.10850019267276,7.50712422400571,-10.041663602964));
#24970=CARTESIAN_POINT('Ctrl Pts',(2.91456159272127,7.5874290327883,-10.033441813787));
#24971=CARTESIAN_POINT('Ctrl Pts',(2.71750758786926,7.6602153005277,-10.02522002461));
#24972=CARTESIAN_POINT('Ctrl Pts',(2.51793967416545,7.72526163697797,-10.016998235433));
#24973=CARTESIAN_POINT('Ctrl Pts',(2.31837231420016,7.79030779294501,-10.0087764690689));
#24974=CARTESIAN_POINT('Ctrl Pts',(2.11629134058487,7.84761397174942,-10.0005547027048));
#24975=CARTESIAN_POINT('Ctrl Pts',(1.91231410721149,7.89700844104018,-9.99233293634071));
#24976=CARTESIAN_POINT('Ctrl Pts',(1.70829434812204,7.94641320822127,-9.9841094558809));
#24977=CARTESIAN_POINT('Ctrl Pts',(1.50237782620332,7.98790290132602,-9.97588597542108));
#24978=CARTESIAN_POINT('Ctrl Pts',(1.29519388187691,8.02135651687722,-9.96766249496127));
#24979=CARTESIAN_POINT('Ctrl Pts',(1.21148405675715,8.03487299044624,-9.96433991070695));
#24980=CARTESIAN_POINT('Ctrl Pts',(1.1275674387783,8.04707819603545,-9.96101732645263));
#24981=CARTESIAN_POINT('Ctrl Pts',(1.04348590916681,8.05796653752486,-9.95769474219831));
#24982=CARTESIAN_POINT('Ctrl Pts',(0.835380510040261,8.08491565062911,-9.9494712033834));
#24983=CARTESIAN_POINT('Ctrl Pts',(0.62619676826291,8.10380302437128,-9.9412476645685));
#24984=CARTESIAN_POINT('Ctrl Pts',(0.416572149134518,8.11456438800417,-9.93302412575359));
#24985=CARTESIAN_POINT('Ctrl Pts',(0.206985643462719,8.12532379503116,-9.92480208212323));
#24986=CARTESIAN_POINT('Ctrl Pts',(-0.0030412851703448,8.12796012566084,
-9.91658003849286));
#24987=CARTESIAN_POINT('Ctrl Pts',(-0.212868004803957,8.12246112794828,
-9.9083579948625));
#24988=CARTESIAN_POINT('Ctrl Pts',(-0.422671557875082,8.11696273736942,
-9.90013685901207));
#24989=CARTESIAN_POINT('Ctrl Pts',(-0.632274651359207,8.103330819407,-9.89191572316165));
#24990=CARTESIAN_POINT('Ctrl Pts',(-0.841037769756865,8.08160522621233,
-9.88369458731123));
#24991=CARTESIAN_POINT('Ctrl Pts',(-1.04981744621454,8.05987790985084,-9.87547279940089));
#24992=CARTESIAN_POINT('Ctrl Pts',(-1.25775672083429,8.03005566347492,-9.86725101149056));
#24993=CARTESIAN_POINT('Ctrl Pts',(-1.46422124509005,7.99223020864182,-9.85902922358022));
#24994=CARTESIAN_POINT('Ctrl Pts',(-1.67068519647114,7.95440485876257,-9.85080745848278));
#24995=CARTESIAN_POINT('Ctrl Pts',(-1.87567411605584,7.90857640064783,-9.84258569338535));
#24996=CARTESIAN_POINT('Ctrl Pts',(-2.07856335525882,7.85488777390709,-9.83436392828791));
#24997=CARTESIAN_POINT('Ctrl Pts',(-2.28149489355781,7.80118795396367,-9.82614044908659));
#24998=CARTESIAN_POINT('Ctrl Pts',(-2.4823255918076,7.73962476716973,-9.81791696988528));
#24999=CARTESIAN_POINT('Ctrl Pts',(-2.68044441560244,7.67039146962954,-9.80969349068397));
#25000=CARTESIAN_POINT('Ctrl Pts',(-2.76049179746798,7.64241863948722,-9.80637089888132));
#25001=CARTESIAN_POINT('Ctrl Pts',(-2.84009665958289,7.61319425858774,-9.80304830707867));
#25002=CARTESIAN_POINT('Ctrl Pts',(-2.91921950827893,7.58273334787553,-9.79972571527603));
#25003=CARTESIAN_POINT('Ctrl Pts',(-3.1150515197089,7.5073414539654,-9.79150217622762));
#25004=CARTESIAN_POINT('Ctrl Pts',(-3.30799316668953,7.42434691148092,-9.78327863717921));
#25005=CARTESIAN_POINT('Ctrl Pts',(-3.49745328333352,7.33399673393707,-9.7750550981308));
#25006=CARTESIAN_POINT('Ctrl Pts',(-3.68687895281885,7.24366298363371,-9.76683305426544));
#25007=CARTESIAN_POINT('Ctrl Pts',(-3.87282408928764,7.14597639442396,-9.75861101040008));
#25008=CARTESIAN_POINT('Ctrl Pts',(-4.05471951110016,7.04123123102797,-9.75038896653472));
#25009=CARTESIAN_POINT('Ctrl Pts',(-4.23659485020781,6.93649763233317,-9.74216783044855));
#25010=CARTESIAN_POINT('Ctrl Pts',(-4.41442111183242,6.82470716246459,-9.73394669436239));
#25011=CARTESIAN_POINT('Ctrl Pts',(-4.58765490561207,6.706199372932,-9.72572555827623));
#25012=CARTESIAN_POINT('Ctrl Pts',(-4.76090243942555,6.58768218395718,-9.71750377013087));
#25013=CARTESIAN_POINT('Ctrl Pts',(-4.92955653265772,6.46244677510975,-9.70928198198552));
#25014=CARTESIAN_POINT('Ctrl Pts',(-5.09310303634507,6.33087584964929,-9.70106019384016));
#25015=CARTESIAN_POINT('Ctrl Pts',(-5.25664908622561,6.1993052892702,-9.69283842850852));
#25016=CARTESIAN_POINT('Ctrl Pts',(-5.41508734680205,6.0613994344153,-9.68461666317688));
#25017=CARTESIAN_POINT('Ctrl Pts',(-5.56793658648711,5.91758140893374,-9.67639489784523));
#25018=CARTESIAN_POINT('Ctrl Pts',(-5.72081769269233,5.77373339978974,-9.66817141841249));
#25019=CARTESIAN_POINT('Ctrl Pts',(-5.86810723539858,5.62397095980253,-9.65994793897975));
#25020=CARTESIAN_POINT('Ctrl Pts',(-6.00935991315134,5.46875497683977,-9.651724459547));
#25021=CARTESIAN_POINT('Ctrl Pts',(-6.06643122883918,5.40604196846076,-9.64840186914924));
#25022=CARTESIAN_POINT('Ctrl Pts',(-6.12251748081821,5.34243910080151,-9.64507927875149));
#25023=CARTESIAN_POINT('Ctrl Pts',(-6.17759109212944,5.27797838769192,-9.64175668835373));
#25024=CARTESIAN_POINT('Ctrl Pts',(-6.31390040065081,5.11843564078345,-9.63353314918797));
#25025=CARTESIAN_POINT('Ctrl Pts',(-6.44404800923583,4.95358366325013,-9.6253096100222));
#25026=CARTESIAN_POINT('Ctrl Pts',(-6.56763168481993,4.7839211547693,-9.61708607085644));
#25027=CARTESIAN_POINT('Ctrl Pts',(-6.69119289076534,4.61428949385187,-9.6088640268716));
#25028=CARTESIAN_POINT('Ctrl Pts',(-6.80819237210817,4.43984928594032,-9.60064198288675));
#25029=CARTESIAN_POINT('Ctrl Pts',(-6.91826972669666,4.2611303137985,-9.59241993890191));
#25030=CARTESIAN_POINT('Ctrl Pts',(-7.02833492789097,4.08243107361812,-9.58419880269453));
#25031=CARTESIAN_POINT('Ctrl Pts',(-7.13147937352829,3.89945426337947,-9.57597766648715));
#25032=CARTESIAN_POINT('Ctrl Pts',(-7.22738690476808,3.71275720877178,-9.56775653027977));
#25033=CARTESIAN_POINT('Ctrl Pts',(-7.32330204293134,3.52604534625292,-9.55953474201146));
#25034=CARTESIAN_POINT('Ctrl Pts',(-7.41197898266931,3.33561291092459,-9.55131295374316));
#25035=CARTESIAN_POINT('Ctrl Pts',(-7.49314782575478,3.14204125114334,-9.54309116547485));
#25036=CARTESIAN_POINT('Ctrl Pts',(-7.57431644362136,2.94847012846468,-9.53486940001951));
#25037=CARTESIAN_POINT('Ctrl Pts',(-7.64797689494447,2.7517600717876,-9.52664763456417));
#25038=CARTESIAN_POINT('Ctrl Pts',(-7.71390747417866,2.55251230012914,-9.51842586910882));
#25039=CARTESIAN_POINT('Ctrl Pts',(-7.77985179884272,2.35322298862219,-9.51020238955205));
#25040=CARTESIAN_POINT('Ctrl Pts',(-7.83806293933497,2.15139518525295,-9.50197890999527));
#25041=CARTESIAN_POINT('Ctrl Pts',(-7.88836876716378,1.94764620907776,-9.49375543043849));
#25042=CARTESIAN_POINT('Ctrl Pts',(-7.90869418083824,1.86532409243151,-9.49043284076948));
#25043=CARTESIAN_POINT('Ctrl Pts',(-7.9277296580035,1.7826885076049,-9.48711025110047));
#25044=CARTESIAN_POINT('Ctrl Pts',(-7.94546619198763,1.69978073717808,-9.48378766143146));
#25045=CARTESIAN_POINT('Ctrl Pts',(-7.9902909041595,1.49025180951269,-9.47539063607622));
#25046=CARTESIAN_POINT('Ctrl Pts',(-8.02682757236947,1.27892832382411,-9.46699361072099));
#25047=CARTESIAN_POINT('Ctrl Pts',(-8.05495717630292,1.06646727583459,-9.45859658536576));
#25048=CARTESIAN_POINT('Ctrl Pts',(-8.08307984587844,0.85405860259438,-9.45020162999983));
#25049=CARTESIAN_POINT('Ctrl Pts',(-8.10279955479153,0.64051319213268,-9.44180667463391));
#25050=CARTESIAN_POINT('Ctrl Pts',(-8.11404888660069,0.426495285265938,
-9.43341171926798));
#25051=CARTESIAN_POINT('Ctrl Pts',(-8.12151237281116,0.284502878624238,
-9.42784199880156));
#25052=CARTESIAN_POINT('Ctrl Pts',(-8.12524843182286,0.142302641431262,
-9.42227227833514));
#25053=CARTESIAN_POINT('Ctrl Pts',(-8.12524999950632,8.95685591188772E-5,
-9.41670255786871));
#25054=CARTESIAN_POINT('Ctrl Pts',(-8.12463074038876,8.95341310840764E-5,
-9.41670255678762));
#25055=CARTESIAN_POINT('Ctrl Pts',(-8.124328237486,-0.773372194525053,-9.38640791602813));
#25056=CARTESIAN_POINT('Ctrl Pts',(-7.8241694511866,-2.89144900506152,-9.30345693296121));
#25057=CARTESIAN_POINT('Ctrl Pts',(-6.00817426353592,-5.96502784783864,
-9.16784960758686));
#25058=CARTESIAN_POINT('Ctrl Pts',(-2.44310026360785,-8.10623070945008,
-9.00988058066457));
#25059=CARTESIAN_POINT('Ctrl Pts',(1.58509684317598,-8.28596807580914,-8.85671523469708));
#25060=CARTESIAN_POINT('Ctrl Pts',(3.97770688061432,-7.18910576064169,-8.75620623103704));
#25061=CARTESIAN_POINT('Ctrl Pts',(4.94707560569883,-6.44630337359169,-8.70835356968441));
#25062=CARTESIAN_POINT('',(-8.12524999771476,0.000192707558782804,-9.58329744321239));
#25063=CARTESIAN_POINT('Ctrl Pts',(-8.12524999771476,0.000192707558782804,
-9.58329744321239));
#25064=CARTESIAN_POINT('Ctrl Pts',(-8.12525496787522,-0.20936729363032,
-9.57508874610108));
#25065=CARTESIAN_POINT('Ctrl Pts',(-8.11714838747745,-0.418942865113511,
-9.56688004898976));
#25066=CARTESIAN_POINT('Ctrl Pts',(-8.10095270917323,-0.62789550582793,
-9.55867135187845));
#25067=CARTESIAN_POINT('Ctrl Pts',(-8.08475586360825,-0.836863206252313,
-9.55046206314696));
#25068=CARTESIAN_POINT('Ctrl Pts',(-8.06046877518818,-1.04520759010267,
-9.54225277441548));
#25069=CARTESIAN_POINT('Ctrl Pts',(-8.02816588827779,-1.25229390831103,
-9.53404348568399));
#25070=CARTESIAN_POINT('Ctrl Pts',(-7.99586328014076,-1.45937843936803,
-9.52583426779852));
#25071=CARTESIAN_POINT('Ctrl Pts',(-7.9555450600785,-1.66520463367737,-9.51762504991305));
#25072=CARTESIAN_POINT('Ctrl Pts',(-7.90733713346637,-1.86914606711297,
-9.50941583202759));
#25073=CARTESIAN_POINT('Ctrl Pts',(-7.85911838623119,-2.07313327670053,
-9.5012047715229));
#25074=CARTESIAN_POINT('Ctrl Pts',(-7.80300646254863,-2.27523459131867,
-9.49299371101821));
#25075=CARTESIAN_POINT('Ctrl Pts',(-7.73917793735757,-2.47483583625619,
-9.48478265051352));
#25076=CARTESIAN_POINT('Ctrl Pts',(-7.70734013857672,-2.57439734505975,
-9.4806869567568));
#25077=CARTESIAN_POINT('Ctrl Pts',(-7.67358320372099,-2.67333705226453,
-9.47659126300008));
#25078=CARTESIAN_POINT('Ctrl Pts',(-7.63793365164408,-2.77158025241609,
-9.47249556924336));
#25079=CARTESIAN_POINT('Ctrl Pts',(-7.56635468679208,-2.96883789412297,
-9.46427202918809));
#25080=CARTESIAN_POINT('Ctrl Pts',(-7.48711843473188,-3.16335319052398,
-9.45604848913282));
#25081=CARTESIAN_POINT('Ctrl Pts',(-7.40046039517722,-3.35453029527434,
-9.44782494907755));
#25082=CARTESIAN_POINT('Ctrl Pts',(-7.31381811144289,-3.54567264096337,
-9.43960290419365));
#25083=CARTESIAN_POINT('Ctrl Pts',(-7.2197568551662,-3.73347773788535,-9.43138085930975));
#25084=CARTESIAN_POINT('Ctrl Pts',(-7.11855979482363,-3.91737080323277,
-9.42315881442585));
#25085=CARTESIAN_POINT('Ctrl Pts',(-7.01737390733895,-4.10124356550934,
-9.41493767731277));
#25086=CARTESIAN_POINT('Ctrl Pts',(-6.9090539308259,-4.28120490022198,-9.4067165401997));
#25087=CARTESIAN_POINT('Ctrl Pts',(-6.7939288123268,-4.45670493251862,-9.39849540308663));
#25088=CARTESIAN_POINT('Ctrl Pts',(-6.67879456261701,-4.6322188846947,-9.39027361390964));
#25089=CARTESIAN_POINT('Ctrl Pts',(-6.5568542520048,-4.80327057935863,-9.38205182473265));
#25090=CARTESIAN_POINT('Ctrl Pts',(-6.42848053838611,-4.96933854049922,
-9.37383003555567));
#25091=CARTESIAN_POINT('Ctrl Pts',(-6.30010718096393,-5.13540604085369,
-9.36560826919155));
#25092=CARTESIAN_POINT('Ctrl Pts',(-6.16530063875436,-5.2964896036532,-9.35738650282743));
#25093=CARTESIAN_POINT('Ctrl Pts',(-6.02447462116785,-5.45209987999161,
-9.34916473646332));
#25094=CARTESIAN_POINT('Ctrl Pts',(-5.88361924379905,-5.60774259837384,
-9.3409412560035));
#25095=CARTESIAN_POINT('Ctrl Pts',(-5.7367420819481,-5.75790953201645,-9.33271777554369));
#25096=CARTESIAN_POINT('Ctrl Pts',(-5.5842952989107,-5.90214652283929,-9.32449429508388));
#25097=CARTESIAN_POINT('Ctrl Pts',(-5.52270127149018,-5.9604234965529,-9.32117171082961));
#25098=CARTESIAN_POINT('Ctrl Pts',(-5.46019844734465,-6.01773285695843,
-9.31784912657534));
#25099=CARTESIAN_POINT('Ctrl Pts',(-5.39681829916226,-6.07404641144002,
-9.31452654232107));
#25100=CARTESIAN_POINT('Ctrl Pts',(-5.239949708696,-6.21342487881518,-9.30630300350617));
#25101=CARTESIAN_POINT('Ctrl Pts',(-5.07765336222313,-6.34674579477515,
-9.29807946469126));
#25102=CARTESIAN_POINT('Ctrl Pts',(-4.91042006300688,-6.4735973281723,-9.28985592587636));
#25103=CARTESIAN_POINT('Ctrl Pts',(-4.74321716975749,-6.60042579772068,
-9.28163388224602));
#25104=CARTESIAN_POINT('Ctrl Pts',(-4.57107935018773,-6.72078705420987,
-9.27341183861569));
#25105=CARTESIAN_POINT('Ctrl Pts',(-4.39452929623703,-6.83431048658272,
-9.26518979498536));
#25106=CARTESIAN_POINT('Ctrl Pts',(-4.21799873483613,-6.94782138505308,
-9.25696865913495));
#25107=CARTESIAN_POINT('Ctrl Pts',(-4.03705715960278,-7.05449580718584,
-9.24874752328454));
#25108=CARTESIAN_POINT('Ctrl Pts',(-3.85225565845309,-7.15400684263135,
-9.24052638743413));
#25109=CARTESIAN_POINT('Ctrl Pts',(-3.66743949975987,-7.25352577080135,
-9.23230459952378));
#25110=CARTESIAN_POINT('Ctrl Pts',(-3.47876306186508,-7.34588003487075,
-9.22408281161343));
#25111=CARTESIAN_POINT('Ctrl Pts',(-3.28680234819714,-7.43078851040626,
-9.21586102370307));
#25112=CARTESIAN_POINT('Ctrl Pts',(-3.09484216716088,-7.51569675034699,
-9.20763925860564));
#25113=CARTESIAN_POINT('Ctrl Pts',(-2.89959799939557,-7.59315912624164,
-9.19941749350821));
#25114=CARTESIAN_POINT('Ctrl Pts',(-2.70166665009423,-7.66294231181918,
-9.19119572841078));
#25115=CARTESIAN_POINT('Ctrl Pts',(-2.50369403533593,-7.73274004605235,
-9.18297224920947));
#25116=CARTESIAN_POINT('Ctrl Pts',(-2.30303339805748,-7.79485529357421,
-9.17474877000816));
#25117=CARTESIAN_POINT('Ctrl Pts',(-2.10029860215858,-7.84910398353027,
-9.16652529080685));
#25118=CARTESIAN_POINT('Ctrl Pts',(-2.01838619568401,-7.87102247424959,
-9.16320269900416));
#25119=CARTESIAN_POINT('Ctrl Pts',(-1.93613535735116,-7.89165735018837,
-9.15988010720147));
#25120=CARTESIAN_POINT('Ctrl Pts',(-1.85358718734212,-7.91099880555048,
-9.15655751539878));
#25121=CARTESIAN_POINT('Ctrl Pts',(-1.64927737748347,-7.95886963136031,
-9.14833397635037));
#25122=CARTESIAN_POINT('Ctrl Pts',(-1.44307892078272,-7.99882923191098,
-9.14011043730195));
#25123=CARTESIAN_POINT('Ctrl Pts',(-1.23561950582139,-8.03074915554792,
-9.13188689825353));
#25124=CARTESIAN_POINT('Ctrl Pts',(-1.02819781060594,-8.06266327558512,
-9.12366485438817));
#25125=CARTESIAN_POINT('Ctrl Pts',(-0.819515906075216,-8.08654059137286,
-9.11544281052281));
#25126=CARTESIAN_POINT('Ctrl Pts',(-0.610209895465547,-8.10230408254195,
-9.10722076665745));
#25127=CARTESIAN_POINT('Ctrl Pts',(-0.400926993910222,-8.11806583329578,
-9.09899963057137));
#25128=CARTESIAN_POINT('Ctrl Pts',(-0.191020417832148,-8.12571552578341,
-9.09077849448529));
#25129=CARTESIAN_POINT('Ctrl Pts',(0.01886956737902,-8.12522808922475,-9.0825573583992));
#25130=CARTESIAN_POINT('Ctrl Pts',(0.228776200010718,-8.12474061400507,
-9.07433557025385));
#25131=CARTESIAN_POINT('Ctrl Pts',(0.438665944197674,-8.11611471821314,
-9.0661137821085));
#25132=CARTESIAN_POINT('Ctrl Pts',(0.647898425864787,-8.09937745708038,
-9.05789199396315));
#25133=CARTESIAN_POINT('Ctrl Pts',(0.857130326957093,-8.0826402423899,-9.04967022863148));
#25134=CARTESIAN_POINT('Ctrl Pts',(1.0657046753998,-8.05779173358663,-9.04144846329982));
#25135=CARTESIAN_POINT('Ctrl Pts',(1.27298556404421,-8.02491092263553,-9.03322669796815));
#25136=CARTESIAN_POINT('Ctrl Pts',(1.48030966730031,-7.99202325658319,-9.0250032185354));
#25137=CARTESIAN_POINT('Ctrl Pts',(1.6863394807022,-7.95109998922567,-9.01677973910264));
#25138=CARTESIAN_POINT('Ctrl Pts',(1.8904475494082,-7.90227154844963,-9.00855625966988));
#25139=CARTESIAN_POINT('Ctrl Pts',(1.97291477204086,-7.88254304912174,-9.00523366927209));
#25140=CARTESIAN_POINT('Ctrl Pts',(2.05506840269879,-7.86152464277297,-9.00191107887428));
#25141=CARTESIAN_POINT('Ctrl Pts',(2.13686763041419,-7.83922727649786,-8.99858848847649));
#25142=CARTESIAN_POINT('Ctrl Pts',(2.33932188973639,-7.78404097584268,-8.99036502968837));
#25143=CARTESIAN_POINT('Ctrl Pts',(2.53967004483497,-7.72099870846218,-8.98214157090025));
#25144=CARTESIAN_POINT('Ctrl Pts',(2.73729898511362,-7.6502863886652,-8.97391811211213));
#25145=CARTESIAN_POINT('Ctrl Pts',(2.93550376974204,-7.57936802976403,-8.96567069209509));
#25146=CARTESIAN_POINT('Ctrl Pts',(3.13097317892045,-7.50073492507245,-8.95742327207806));
#25147=CARTESIAN_POINT('Ctrl Pts',(3.32310566778239,-7.4146244870022,-8.94917585206102));
#25148=CARTESIAN_POINT('Ctrl Pts',(3.5146335017164,-7.32878504474859,-8.94095438727511));
#25149=CARTESIAN_POINT('Ctrl Pts',(3.70284512438198,-7.23551540107621,-8.93273292248921));
#25150=CARTESIAN_POINT('Ctrl Pts',(3.88716557477536,-7.13509855270278,-8.9245114577033));
#25151=CARTESIAN_POINT('Ctrl Pts',(4.07235887690803,-7.03420617912002,-8.9162510600707));
#25152=CARTESIAN_POINT('Ctrl Pts',(4.25362378264773,-6.92609885551256,-8.9079906624381));
#25153=CARTESIAN_POINT('Ctrl Pts',(4.43040241461211,-6.81111018902933,-8.89973026480549));
#25154=CARTESIAN_POINT('Ctrl Pts',(4.60718104657649,-6.6961215225461,-8.89146986717289));
#25155=CARTESIAN_POINT('Ctrl Pts',(4.77947315318472,-6.57425168013767,-8.88320946954029));
#25156=CARTESIAN_POINT('Ctrl Pts',(4.94675008185375,-6.44587862049697,-8.87494907190769));
#25157=CARTESIAN_POINT('Ctrl Pts',(4.94701442880054,-6.44622255101802,-10.8749380057189));
#25158=CARTESIAN_POINT('Ctrl Pts',(5.88239992671177,-5.72708597335159,-10.8287079320199));
#25159=CARTESIAN_POINT('Ctrl Pts',(7.54661450291582,-3.74878751104997,-10.7298215160133));
#25160=CARTESIAN_POINT('Ctrl Pts',(8.46533576428991,0.133483448085083,-10.5782787576994));
#25161=CARTESIAN_POINT('Ctrl Pts',(7.38054169264561,4.14816882234201,-10.4203097307771));
#25162=CARTESIAN_POINT('Ctrl Pts',(4.51501107248497,7.16201092752528,-10.2623407038548));
#25163=CARTESIAN_POINT('Ctrl Pts',(0.560121710166043,8.44783839312321,-10.1043716769325));
#25164=CARTESIAN_POINT('Ctrl Pts',(-3.52991045919384,7.69541743414669,-9.94640265001023));
#25165=CARTESIAN_POINT('Ctrl Pts',(-6.76826471849102,5.08628620969646,-9.78843362308794));
#25166=CARTESIAN_POINT('Ctrl Pts',(-7.99827042167485,2.14691493907655,-9.66739855694933));
#25167=CARTESIAN_POINT('Ctrl Pts',(-8.1253377544992,0.401556537849047,-9.59901983311814));
#25168=CARTESIAN_POINT('Ctrl Pts',(-8.1249788462242,0.000192915105033694,
-9.58329745159439));
#25169=CARTESIAN_POINT('Ctrl Pts',(5.30944861964463,-4.57791378026326,-11.9996110935251));
#25170=CARTESIAN_POINT('Ctrl Pts',(6.06687727096382,-3.6994534565604,-11.9469459372515));
#25171=CARTESIAN_POINT('Ctrl Pts',(7.13654022615018,-1.56045331767952,-11.8416244386703));
#25172=CARTESIAN_POINT('Ctrl Pts',(7.01811917762224,2.02657116595001,-11.6836465977818));
#25173=CARTESIAN_POINT('Ctrl Pts',(5.20670544824235,5.12353011424085,-11.5256775708595));
#25174=CARTESIAN_POINT('Ctrl Pts',(2.1389031829018,6.98475869103201,-11.3677085439372));
#25175=CARTESIAN_POINT('Ctrl Pts',(-1.44489008506026,7.16051286830259,-11.209739517015));
#25176=CARTESIAN_POINT('Ctrl Pts',(-4.68010501547651,5.60873401464311,-11.0517704900927));
#25177=CARTESIAN_POINT('Ctrl Pts',(-6.7861098885743,2.70364896469204,-10.8938014631704));
#25178=CARTESIAN_POINT('Ctrl Pts',(-7.25480791088177,-0.85372703166743,
-10.7358324362481));
#25179=CARTESIAN_POINT('Ctrl Pts',(-5.97309921761341,-4.20513633432643,
-10.5778634093258));
#25180=CARTESIAN_POINT('Ctrl Pts',(-3.2502353630771,-6.54194433684208,-10.4198943824035));
#25181=CARTESIAN_POINT('Ctrl Pts',(0.256829418882314,-7.30035088692297,
-10.2619253554812));
#25182=CARTESIAN_POINT('Ctrl Pts',(3.70192706745187,-6.29736522276595,-10.1039563285589));
#25183=CARTESIAN_POINT('Ctrl Pts',(6.25384370141796,-3.77498573442189,-9.94598730163663));
#25184=CARTESIAN_POINT('Ctrl Pts',(7.29686584301275,-0.341797086983226,
-9.78801827471434));
#25185=CARTESIAN_POINT('Ctrl Pts',(6.57933890745369,3.1738582537474,-9.63004924779205));
#25186=CARTESIAN_POINT('Ctrl Pts',(4.27438385343404,5.92374202677216,-9.47208022086977));
#25187=CARTESIAN_POINT('Ctrl Pts',(0.938128110736348,7.24437659620591,-9.31411119394746));
#25188=CARTESIAN_POINT('Ctrl Pts',(-2.62447423026687,6.81712636270503,-9.15614216702519));
#25189=CARTESIAN_POINT('Ctrl Pts',(-5.55385731259764,4.74507593956608,-8.99817314010289));
#25190=CARTESIAN_POINT('Ctrl Pts',(-7.14323510016274,1.52815871821299,-8.8402041131806));
#25191=CARTESIAN_POINT('Ctrl Pts',(-7.00913092711596,-2.05746455634189,
-8.68223508625831));
#25192=CARTESIAN_POINT('Ctrl Pts',(-5.18390074123243,-5.14667366916295,
-8.52426605933603));
#25193=CARTESIAN_POINT('Ctrl Pts',(-2.10792642022479,-6.99412059972256,
-8.36629703241372));
#25194=CARTESIAN_POINT('Ctrl Pts',(1.47663723085556,-7.15406312813223,-8.20832800549144));
#25195=CARTESIAN_POINT('Ctrl Pts',(4.70492566621234,-5.58791116879607,-8.05035897856915));
#25196=CARTESIAN_POINT('Ctrl Pts',(6.7980345379359,-2.67353757689276,-7.89238995164686));
#25197=CARTESIAN_POINT('Ctrl Pts',(7.25094961548956,0.885893011560273,-7.73442092472457));
#25198=CARTESIAN_POINT('Ctrl Pts',(5.95439394599882,4.23158002289299,-7.57645189780228));
#25199=CARTESIAN_POINT('Ctrl Pts',(3.22119361930529,6.55629380223107,-7.41848287087999));
#25200=CARTESIAN_POINT('Ctrl Pts',(-0.289199255448484,7.29913971266049,
-7.2605138439577));
#25201=CARTESIAN_POINT('Ctrl Pts',(-3.72981566445424,6.28088782445941,-7.10254481703542));
#25202=CARTESIAN_POINT('Ctrl Pts',(-6.27052189027239,3.74721656404909,-6.94457579011312));
#25203=CARTESIAN_POINT('Ctrl Pts',(-7.29830978161512,0.309436723489391,
-6.78660676319084));
#25204=CARTESIAN_POINT('Ctrl Pts',(-6.56520011570507,-3.20300237199563,
-6.62863773626853));
#25205=CARTESIAN_POINT('Ctrl Pts',(-4.2480737126944,-5.94263800729771,-6.47066870934626));
#25206=CARTESIAN_POINT('Ctrl Pts',(-0.905994567535462,-7.24846539605864,
-6.31269968242396));
#25207=CARTESIAN_POINT('Ctrl Pts',(2.65467815183388,-6.80542141710856,-6.15473065550168));
#25208=CARTESIAN_POINT('Ctrl Pts',(5.57484417681311,-4.72040137684464,-5.99676162857937));
#25209=CARTESIAN_POINT('Ctrl Pts',(7.14994130409419,-1.49646787545602,-5.8387926016571));
#25210=CARTESIAN_POINT('Ctrl Pts',(6.99993843512708,2.08852547475353,-5.68082357473479));
#25211=CARTESIAN_POINT('Ctrl Pts',(5.16102746823472,5.16961045209313,-5.52285454781251));
#25212=CARTESIAN_POINT('Ctrl Pts',(2.07689110893385,7.00339918010501,-5.36488552089022));
#25213=CARTESIAN_POINT('Ctrl Pts',(-1.50834654502773,7.14744481995956,-5.20691649396793));
#25214=CARTESIAN_POINT('Ctrl Pts',(-4.7296583276429,5.56699280204512,-5.04894746704564));
#25215=CARTESIAN_POINT('Ctrl Pts',(-6.80982318103781,2.64336622458256,-4.89097844012335));
#25216=CARTESIAN_POINT('Ctrl Pts',(-7.2469499388148,-0.918037765332133,
-4.73300941320106));
#25217=CARTESIAN_POINT('Ctrl Pts',(-5.93557097038376,-4.25794246201161,
-4.57504038627877));
#25218=CARTESIAN_POINT('Ctrl Pts',(-3.19208885267558,-6.57051333693862,
-4.41707135935648));
#25219=CARTESIAN_POINT('Ctrl Pts',(0.321563569035109,-7.29778552886649,
-4.2591023324342));
#25220=CARTESIAN_POINT('Ctrl Pts',(3.75763083470845,-6.26428665246988,-4.1011333055119));
#25221=CARTESIAN_POINT('Ctrl Pts',(6.28707682012798,-3.71937384677495,-3.94316427858961));
#25222=CARTESIAN_POINT('Ctrl Pts',(7.29961018521532,-0.277070204396804,
-3.78519525166732));
#25223=CARTESIAN_POINT('Ctrl Pts',(6.55093223855146,3.23208347048326,-3.62722622474503));
#25224=CARTESIAN_POINT('Ctrl Pts',(4.22168003267289,5.96141715165068,-3.46925719782274));
#25225=CARTESIAN_POINT('Ctrl Pts',(0.87384321207103,7.25241165371776,-3.31128817090045));
#25226=CARTESIAN_POINT('Ctrl Pts',(-2.68482987385822,6.79358265591156,-3.15331914397816));
#25227=CARTESIAN_POINT('Ctrl Pts',(-5.59572141748757,4.69563399043567,-2.99535011705587));
#25228=CARTESIAN_POINT('Ctrl Pts',(-7.15650691328321,1.46474760774455,-2.83738109013358));
#25229=CARTESIAN_POINT('Ctrl Pts',(-6.99060829739456,-2.11954532545598,
-2.67941206321129));
#25230=CARTESIAN_POINT('Ctrl Pts',(-5.13805270983225,-5.19244558038399,
-2.521443036289));
#25231=CARTESIAN_POINT('Ctrl Pts',(-2.04581495797315,-7.01254004708689,
-2.36347400936671));
#25232=CARTESIAN_POINT('Ctrl Pts',(1.54002619931572,-7.14068596562577,-2.20550498244442));
#25233=CARTESIAN_POINT('Ctrl Pts',(4.75429798593852,-5.54596496699761,-2.04753595552213));
#25234=CARTESIAN_POINT('Ctrl Pts',(6.82147791699478,-2.61314289357019,-1.88956692859984));
#25235=CARTESIAN_POINT('Ctrl Pts',(7.24280775942499,0.95016446696199,-1.73159790167755));
#25236=CARTESIAN_POINT('Ctrl Pts',(5.9166312787675,4.2842211737227,-1.57362887475526));
#25237=CARTESIAN_POINT('Ctrl Pts',(3.16292131738634,6.5846036702513,-1.41565984783297));
#25238=CARTESIAN_POINT('Ctrl Pts',(-0.353921559454153,7.29628784273328,
-1.25769082091068));
#25239=CARTESIAN_POINT('Ctrl Pts',(-3.78537211558607,6.24756230067434,-1.09972179398839));
#25240=CARTESIAN_POINT('Ctrl Pts',(-6.30350812203686,3.69145799240344,-0.9417527670661));
#25241=CARTESIAN_POINT('Ctrl Pts',(-7.3007670505948,0.24469823704531,-0.783783740143811));
#25242=CARTESIAN_POINT('Ctrl Pts',(-6.53653554504556,-3.26110101386324,
-0.625814713221519));
#25243=CARTESIAN_POINT('Ctrl Pts',(-4.19520333829513,-5.98007907176997,
-0.46784568629923));
#25244=CARTESIAN_POINT('Ctrl Pts',(-0.841674673510988,-7.2562153012596,
-0.309876659376941));
#25245=CARTESIAN_POINT('Ctrl Pts',(2.71492880187119,-6.78161030692815,-0.151907632454651));
#25246=CARTESIAN_POINT('Ctrl Pts',(5.61648862490336,-4.67077426992517,0.00606139446763901));
#25247=CARTESIAN_POINT('Ctrl Pts',(7.16293179820857,-1.43299853749978,0.164030421389929));
#25248=CARTESIAN_POINT('Ctrl Pts',(6.98114069759885,2.15052349780071,0.32199944831222));
#25249=CARTESIAN_POINT('Ctrl Pts',(5.1149769176862,5.21517860535967,0.479968475234509));
#25250=CARTESIAN_POINT('Ctrl Pts',(2.01469857847539,7.0215430207436,0.637937502156801));
#25251=CARTESIAN_POINT('Ctrl Pts',(-1.57167557080576,7.13378669812858,0.795906529079091));
#25252=CARTESIAN_POINT('Ctrl Pts',(-4.77884415657439,5.52482807709332,0.953875556001379));
#25253=CARTESIAN_POINT('Ctrl Pts',(-6.83299851663795,2.58286817818632,1.11184458292367));
#25254=CARTESIAN_POINT('Ctrl Pts',(-7.23852315876716,-0.982272484728826,
1.26981360984596));
#25255=CARTESIAN_POINT('Ctrl Pts',(-5.89757524357886,-4.31041564127981,
1.42778263676825));
#25256=CARTESIAN_POINT('Ctrl Pts',(-3.13369158698168,-6.59856452510272,
1.58575166369054));
#25257=CARTESIAN_POINT('Ctrl Pts',(0.386272590423321,-7.29464668370932,
1.74372069061283));
#25258=CARTESIAN_POINT('Ctrl Pts',(3.81303896158782,-6.23071509793838,1.90168971753512));
#25259=CARTESIAN_POINT('Ctrl Pts',(6.31981547289674,-3.66346954986648,2.05965874445741));
#25260=CARTESIAN_POINT('Ctrl Pts',(7.30178035500521,-0.212321457991736,
2.2176277713797));
#25261=CARTESIAN_POINT('Ctrl Pts',(6.52201031828136,3.29005443153991,2.37559679830199));
#25262=CARTESIAN_POINT('Ctrl Pts',(4.16864415019414,5.99862340069086,2.53356582522428));
#25263=CARTESIAN_POINT('Ctrl Pts',(0.809489584411698,7.25987626388997,2.69153485214657));
#25264=CARTESIAN_POINT('Ctrl Pts',(-2.74497434401292,6.76950460558043,2.84950387906886));
#25265=CARTESIAN_POINT('Ctrl Pts',(-5.63714539069788,4.6458227041502,3.00747290599115));
#25266=CARTESIAN_POINT('Ctrl Pts',(-7.16921583253243,1.40122128902973,3.16544193291344));
#25267=CARTESIAN_POINT('Ctrl Pts',(-6.97153582190914,-2.18145938263847,
3.32341095983573));
#25268=CARTESIAN_POINT('Ctrl Pts',(-5.09180054555483,-5.23780908000201,
3.48137998675802));
#25269=CARTESIAN_POINT('Ctrl Pts',(-1.9835425823075,-7.03040792404231,3.63934901368031));
#25270=CARTESIAN_POINT('Ctrl Pts',(1.60329403715025,-7.12674715313392,3.7973180406026));
#25271=CARTESIAN_POINT('Ctrl Pts',(4.80329635687901,-5.50358254796425,3.95528706752489));
#25272=CARTESIAN_POINT('Ctrl Pts',(6.8443847534283,-2.55254267374754,4.11325609444718));
#25273=CARTESIAN_POINT('Ctrl Pts',(7.23409622109297,1.01436118726632,4.27122512136948));
#25274=CARTESIAN_POINT('Ctrl Pts',(5.87840323953227,4.33652534959965,4.42919414829176));
#25275=CARTESIAN_POINT('Ctrl Pts',(3.1044002362298,6.61239562696911,4.58716317521405));
#25276=CARTESIAN_POINT('Ctrl Pts',(-0.418616025797768,7.29286208406613,
4.74513220213634));
#25277=CARTESIAN_POINT('Ctrl Pts',(-3.84063082867778,6.21374537554234,4.90310122905863));
#25278=CARTESIAN_POINT('Ctrl Pts',(-6.33599855204275,3.6354090695238,5.06107025598092));
#25279=CARTESIAN_POINT('Ctrl Pts',(-7.30265007852114,0.179940503887283,
5.21903928290322));
#25280=CARTESIAN_POINT('Ctrl Pts',(-6.50735684388029,-3.31894315417848,
5.37700830982549));
#25281=CARTESIAN_POINT('Ctrl Pts',(-4.14200299062497,-6.01704977376103,
5.53497733674779));
#25282=CARTESIAN_POINT('Ctrl Pts',(-0.777288577654901,-7.26339446962033,
5.69294636367007));
#25283=CARTESIAN_POINT('Ctrl Pts',(2.77496590947331,-6.75726578991273,5.85091539059238));
#25284=CARTESIAN_POINT('Ctrl Pts',(5.65769130868017,-4.62077978375391,6.00888441751465));
#25285=CARTESIAN_POINT('Ctrl Pts',(7.17535889268669,-1.3694164871965,6.16685344443696));
#25286=CARTESIAN_POINT('Ctrl Pts',(6.96179385919402,2.2123523716516,6.32482247135923));
#25287=CARTESIAN_POINT('Ctrl Pts',(5.0685240491741,5.26033655930945,6.48279149828153));
#25288=CARTESIAN_POINT('Ctrl Pts',(1.95234758211533,7.03913458266513,6.64076052520383));
#25289=CARTESIAN_POINT('Ctrl Pts',(-1.63488097660941,7.11956746906613,6.7987295521261));
#25290=CARTESIAN_POINT('Ctrl Pts',(-4.82765410602868,5.48222879737866,6.95669857904841));
#25291=CARTESIAN_POINT('Ctrl Pts',(-6.85563640346892,2.52216697656922,7.11466760597069));
#25292=CARTESIAN_POINT('Ctrl Pts',(-7.22952703345286,-1.04642994358814,
7.27263663289298));
#25293=CARTESIAN_POINT('Ctrl Pts',(-5.85911564362261,-4.36254978526544,
7.43060565981527));
#25294=CARTESIAN_POINT('Ctrl Pts',(-3.07504784111029,-6.6260967038787,7.58857468673756));
#25295=CARTESIAN_POINT('Ctrl Pts',(0.450951229581866,-7.29093407889477,
7.74654371365985));
#25296=CARTESIAN_POINT('Ctrl Pts',(3.86814717429503,-6.19665346717748,7.90451274058214));
#25297=CARTESIAN_POINT('Ctrl Pts',(6.3520570412528,-3.60727710314822,8.06248176750443));
#25298=CARTESIAN_POINT('Ctrl Pts',(7.30337620404243,-0.147556011471691,
8.22045079442672));
#25299=CARTESIAN_POINT('Ctrl Pts',(6.49257540998184,3.34776661372899,8.37841982134901));
#25300=CARTESIAN_POINT('Ctrl Pts',(4.11528038346205,6.03535782862288,8.5363888482713));
#25301=CARTESIAN_POINT('Ctrl Pts',(0.745072286421063,7.26676984931728,8.69435787519359));
#25302=CARTESIAN_POINT('Ctrl Pts',(-2.8049029084755,6.74489410049378,8.85232690211588));
#25303=CARTESIAN_POINT('Ctrl Pts',(-5.67812597489344,4.59564600135665,9.01029592903816));
#25304=CARTESIAN_POINT('Ctrl Pts',(-7.18136085776966,1.3375847570525,9.16826495596046));
#25305=CARTESIAN_POINT('Ctrl Pts',(-6.95191500122292,-2.24320185668345,
9.32623398288275));
#25306=CARTESIAN_POINT('Ctrl Pts',(-5.04514788584998,-5.28276060163157,
9.48420300980505));
#25307=CARTESIAN_POINT('Ctrl Pts',(-1.92111419208628,-7.04772282243763,
9.64217203672733));
#25308=CARTESIAN_POINT('Ctrl Pts',(1.66643576956794,-7.11224779210674,9.80014106364964));
#25309=CARTESIAN_POINT('Ctrl Pts',(4.8519169221348,-5.46076723551842,9.95811009057189));
#25310=CARTESIAN_POINT('Ctrl Pts',(6.86675325118528,-2.49174170282171,10.1160791174942));
#25311=CARTESIAN_POINT('Ctrl Pts',(7.22481567467034,1.07847815974748,10.2740481444165));
#25312=CARTESIAN_POINT('Ctrl Pts',(5.83971285652996,4.38848836535715,10.4320171713388));
#25313=CARTESIAN_POINT('Ctrl Pts',(3.04563493721469,6.63966762466851,10.5899861982611));
#25314=CARTESIAN_POINT('Ctrl Pts',(-0.483277485164237,7.28886243758024,
10.7479552251834));
#25315=CARTESIAN_POINT('Ctrl Pts',(-3.89558761425688,6.17944023049411,10.9059242521057));
#25316=CARTESIAN_POINT('Ctrl Pts',(-6.36799032002207,3.57907319090321,11.063893279028));
#25317=CARTESIAN_POINT('Ctrl Pts',(-7.30395930917253,0.115170585126009,
11.2218623059502));
#25318=CARTESIAN_POINT('Ctrl Pts',(-6.47766515763742,-3.37652806502809,
11.3798313328725));
#25319=CARTESIAN_POINT('Ctrl Pts',(-4.08847908705193,-6.05353978254256,
11.5378003597948));
#25320=CARTESIAN_POINT('Ctrl Pts',(-0.712837007271165,-7.27001675403624,
11.6957693867171));
#25321=CARTESIAN_POINT('Ctrl Pts',(2.83477632842898,-6.73236177450462,11.8537384136394));
#25322=CARTESIAN_POINT('Ctrl Pts',(5.69846535245322,-4.57047627984927,12.0117074405617));
#25323=CARTESIAN_POINT('Ctrl Pts',(7.18718979160324,-1.3056206783609,12.169676467484));
#25324=CARTESIAN_POINT('Ctrl Pts',(6.94196157239741,2.27379792622975,12.3276454944063));
#25325=CARTESIAN_POINT('Ctrl Pts',(5.02154850583196,5.30552096540472,12.4856145213286));
#25326=CARTESIAN_POINT('Ctrl Pts',(2.93392826290545,6.47182695586933,12.5909272059434));
#25327=CARTESIAN_POINT('Ctrl Pts',(1.81369530454163,6.7718570992692,12.6435835482508));
#25328=CARTESIAN_POINT('Ctrl Pts',(5.59099055985781,-4.82066492452619,-12.214237887564));
#25329=CARTESIAN_POINT('Ctrl Pts',(6.38858306760391,-3.89562284786681,-12.1615727312903));
#25330=CARTESIAN_POINT('Ctrl Pts',(7.51496659875801,-1.64319883160089,-12.0562512327092));
#25331=CARTESIAN_POINT('Ctrl Pts',(7.39026608617398,2.13403331859815,-11.8982733918206));
#25332=CARTESIAN_POINT('Ctrl Pts',(5.48279926871797,5.39521343061514,-11.7403043648983));
#25333=CARTESIAN_POINT('Ctrl Pts',(2.25232191904217,7.35513660683255,-11.582335337976));
#25334=CARTESIAN_POINT('Ctrl Pts',(-1.52150767515003,7.54021042830991,-11.4243663110537));
#25335=CARTESIAN_POINT('Ctrl Pts',(-4.92827501218454,5.90614603795184,-11.2663972841314));
#25336=CARTESIAN_POINT('Ctrl Pts',(-7.14595413632915,2.8470142422763,-11.1084282572091));
#25337=CARTESIAN_POINT('Ctrl Pts',(-7.63950561518693,-0.898997262557083,
-10.9504592302869));
#25338=CARTESIAN_POINT('Ctrl Pts',(-6.28983228413006,-4.42812036284623,
-10.7924902033646));
#25339=CARTESIAN_POINT('Ctrl Pts',(-3.42258425197763,-6.88884131867677,
-10.6345211764423));
#25340=CARTESIAN_POINT('Ctrl Pts',(0.270448206458184,-7.68746357981854,
-10.47655214952));
#25341=CARTESIAN_POINT('Ctrl Pts',(3.89822762590192,-6.63129300888081,-10.3185831225977));
#25342=CARTESIAN_POINT('Ctrl Pts',(6.58546368978599,-3.97516034464673,-10.1606140956754));
#25343=CARTESIAN_POINT('Ctrl Pts',(7.68379373592351,-0.359921420020828,
-10.0026450687531));
#25344=CARTESIAN_POINT('Ctrl Pts',(6.92821879574774,3.34215712519999,-9.84467604183086));
#25345=CARTESIAN_POINT('Ctrl Pts',(4.50103984156416,6.23785784990473,-9.68670701490859));
#25346=CARTESIAN_POINT('Ctrl Pts',(0.987873842805025,7.6285211634938,-9.52873798798628));
#25347=CARTESIAN_POINT('Ctrl Pts',(-2.76364114189211,7.17861530823001,-9.37076896106401));
#25348=CARTESIAN_POINT('Ctrl Pts',(-5.84835941168012,4.99669112264581,-9.2127999341417));
#25349=CARTESIAN_POINT('Ctrl Pts',(-7.52201647909117,1.60919175973965,-9.05483090721943));
#25350=CARTESIAN_POINT('Ctrl Pts',(-7.38080121941844,-2.16656488004954,
-8.89686188029712));
#25351=CARTESIAN_POINT('Ctrl Pts',(-5.45878530592322,-5.41958420927045,
-8.73889285337486));
#25352=CARTESIAN_POINT('Ctrl Pts',(-2.21970256435789,-7.36499494559062,
-8.58092382645254));
#25353=CARTESIAN_POINT('Ctrl Pts',(1.5549382637402,-7.53341868043001,-8.42295479953027));
#25354=CARTESIAN_POINT('Ctrl Pts',(4.95441181732098,-5.88421902765374,-8.26498577260798));
#25355=CARTESIAN_POINT('Ctrl Pts',(7.15851110914994,-2.81530615034617,-8.10701674568568));
#25356=CARTESIAN_POINT('Ctrl Pts',(7.63544272755767,0.932868894587585,-7.94904771876339));
#25357=CARTESIAN_POINT('Ctrl Pts',(6.27013513579911,4.45596626997045,-7.7910786918411));
#25358=CARTESIAN_POINT('Ctrl Pts',(3.39200252364726,6.90395168724349,-7.63310966491881));
#25359=CARTESIAN_POINT('Ctrl Pts',(-0.304534504985681,7.68618818111842,
-7.47514063799653));
#25360=CARTESIAN_POINT('Ctrl Pts',(-3.92759506002511,6.61394187037614,-7.31717161107423));
#25361=CARTESIAN_POINT('Ctrl Pts',(-6.60302626607604,3.94591866993969,-7.15920258415194));
#25362=CARTESIAN_POINT('Ctrl Pts',(-7.6853142416621,0.325845096890364,-7.00123355722965));
#25363=CARTESIAN_POINT('Ctrl Pts',(-6.91333027212556,-3.37284665657586,
-6.84326453030737));
#25364=CARTESIAN_POINT('Ctrl Pts',(-4.47333456385235,-6.25775581978934,
-6.68529550338507));
#25365=CARTESIAN_POINT('Ctrl Pts',(-0.954036367473559,-7.63282677844849,
-6.52732647646279));
#25366=CARTESIAN_POINT('Ctrl Pts',(2.79544667433989,-7.16628968931519,-6.36935744954049));
#25367=CARTESIAN_POINT('Ctrl Pts',(5.87045913768095,-4.9707081520726,-6.2113884226182));
#25368=CARTESIAN_POINT('Ctrl Pts',(7.52907829013018,-1.57582045974579,-6.05341939569592));
#25369=CARTESIAN_POINT('Ctrl Pts',(7.37112128095155,2.19927285295983,-5.89545036877362));
#25370=CARTESIAN_POINT('Ctrl Pts',(5.43469914132034,5.44373725152078,-5.73748134185133));
#25371=CARTESIAN_POINT('Ctrl Pts',(2.1870215564265,7.37476553742481,-5.57951231492904));
#25372=CARTESIAN_POINT('Ctrl Pts',(-1.58832901462538,7.5264494259619,-5.42154328800675));
#25373=CARTESIAN_POINT('Ctrl Pts',(-4.98045596737956,5.86219143130419,-5.26357426108446));
#25374=CARTESIAN_POINT('Ctrl Pts',(-7.17092486376328,2.78353491419177,-5.10560523416217));
#25375=CARTESIAN_POINT('Ctrl Pts',(-7.63123096167894,-0.966718174948357,
-4.94763620723988));
#25376=CARTESIAN_POINT('Ctrl Pts',(-6.25031404202623,-4.48372661926579,
-4.78966718031759));
#25377=CARTESIAN_POINT('Ctrl Pts',(-3.36135443057194,-6.91892523534814,
-4.6316981533953));
#25378=CARTESIAN_POINT('Ctrl Pts',(0.338614987668868,-7.6847621895794,-4.47372912647301));
#25379=CARTESIAN_POINT('Ctrl Pts',(3.95688517383029,-6.59646039489246,-4.31576009955072));
#25380=CARTESIAN_POINT('Ctrl Pts',(6.62045904736319,-3.91659954839013,-4.15779107262843));
#25381=CARTESIAN_POINT('Ctrl Pts',(7.68668360122721,-0.291762291750758,
-3.99982204570614));
#25382=CARTESIAN_POINT('Ctrl Pts',(6.8983058181399,3.40346982646831,-3.84185301878385));
#25383=CARTESIAN_POINT('Ctrl Pts',(4.44554131705566,6.27753075807789,-3.68388399186156));
#25384=CARTESIAN_POINT('Ctrl Pts',(0.920180135354985,7.63698229268348,-3.52591496493927));
#25385=CARTESIAN_POINT('Ctrl Pts',(-2.82719723928136,7.15382315901524,-3.36794593801698));
#25386=CARTESIAN_POINT('Ctrl Pts',(-5.89244342717854,4.9446274356885,-3.20997691109469));
#25387=CARTESIAN_POINT('Ctrl Pts',(-7.53599205116739,1.54241817449251,-3.0520078841724));
#25388=CARTESIAN_POINT('Ctrl Pts',(-7.36129639785696,-2.23193758048048,
-2.89403885725011));
#25389=CARTESIAN_POINT('Ctrl Pts',(-5.41050610988806,-5.46778324873317,
-2.73606983032782));
#25390=CARTESIAN_POINT('Ctrl Pts',(-2.15429754323705,-7.38439111338679,
-2.57810080340553));
#25391=CARTESIAN_POINT('Ctrl Pts',(1.62168853286391,-7.51933217264942,-2.42013177648324));
#25392=CARTESIAN_POINT('Ctrl Pts',(5.00640218266438,-5.84004856192791,-2.26216274956095));
#25393=CARTESIAN_POINT('Ctrl Pts',(7.18319761059275,-2.751708943082,-2.10419372263866));
#25394=CARTESIAN_POINT('Ctrl Pts',(7.62686913665253,1.00054844592363,-1.94622469571637));
#25395=CARTESIAN_POINT('Ctrl Pts',(6.23037004320095,4.51139880137492,-1.78825566879408));
#25396=CARTESIAN_POINT('Ctrl Pts',(3.33064024042927,6.93376273094893,-1.63028664187179));
#25397=CARTESIAN_POINT('Ctrl Pts',(-0.372688811888484,7.68318508626183,
-1.4723176149495));
#25398=CARTESIAN_POINT('Ctrl Pts',(-3.98609748015743,6.57884920779809,-1.31434858802721));
#25399=CARTESIAN_POINT('Ctrl Pts',(-6.63776164513556,3.88720341153253,-1.15637956110492));
#25400=CARTESIAN_POINT('Ctrl Pts',(-7.68790181122962,0.257673749449668,
-0.998410534182634));
#25401=CARTESIAN_POINT('Ctrl Pts',(-6.88314571711041,-3.43402607114267,
-0.840441507260343));
#25402=CARTESIAN_POINT('Ctrl Pts',(-4.41766065393471,-6.29718225613171,
-0.682472480338053));
#25403=CARTESIAN_POINT('Ctrl Pts',(-0.886305808979903,-7.64098763467338,
-0.524503453415764));
#25404=CARTESIAN_POINT('Ctrl Pts',(2.85889221072524,-7.14121595722447,-0.366534426493473));
#25405=CARTESIAN_POINT('Ctrl Pts',(5.91431184872925,-4.91844948904059,-0.208565399571184));
#25406=CARTESIAN_POINT('Ctrl Pts',(7.54275762581348,-1.50898555940589,-0.050596372648894));
#25407=CARTESIAN_POINT('Ctrl Pts',(7.35132676355511,2.26455841958236,0.107372654273397));
#25408=CARTESIAN_POINT('Ctrl Pts',(5.38620668723756,5.49172172844002,0.265341681195686));
#25409=CARTESIAN_POINT('Ctrl Pts',(2.1215311683285,7.39387148401118,0.423310708117978));
#25410=CARTESIAN_POINT('Ctrl Pts',(-1.6550161625111,7.51206706054266,0.581279735040268));
#25411=CARTESIAN_POINT('Ctrl Pts',(-5.0322499529579,5.81779085488797,0.739248761962557));
#25412=CARTESIAN_POINT('Ctrl Pts',(-7.1953291083175,2.71982886286287,0.897217788884847));
#25413=CARTESIAN_POINT('Ctrl Pts',(-7.62235733824431,-1.03435904229439,
1.05518681580714));
#25414=CARTESIAN_POINT('Ctrl Pts',(-6.21030353150069,-4.53898227215012,
1.21315584272943));
#25415=CARTESIAN_POINT('Ctrl Pts',(-3.29986055717648,-6.9484638822875,1.37112486965172));
#25416=CARTESIAN_POINT('Ctrl Pts',(0.40675530762235,-7.68145690217578,1.52909389657401));
#25417=CARTESIAN_POINT('Ctrl Pts',(4.01523140458121,-6.56110865539718,1.6870629234963));
#25418=CARTESIAN_POINT('Ctrl Pts',(6.65493371915781,-3.8577308374068,1.84503195041859));
#25419=CARTESIAN_POINT('Ctrl Pts',(7.68896884771471,-0.223580140298352,
2.00300097734088));
#25420=CARTESIAN_POINT('Ctrl Pts',(6.8678502671426,3.46451478974651,2.16097000426317));
#25421=CARTESIAN_POINT('Ctrl Pts',(4.38969312272992,6.31670992752719,2.31893903118546));
#25422=CARTESIAN_POINT('Ctrl Pts',(0.852414054446948,7.64484272565788,2.47690805810775));
#25423=CARTESIAN_POINT('Ctrl Pts',(-2.89053096542732,7.12846833184862,2.63487708503004));
#25424=CARTESIAN_POINT('Ctrl Pts',(-5.93606397231646,4.89217482688728,2.79284611195233));
#25425=CARTESIAN_POINT('Ctrl Pts',(-7.54937488103139,1.47552327189886,2.95081513887462));
#25426=CARTESIAN_POINT('Ctrl Pts',(-7.3412125740871,-2.29713472881507,3.10878416579691));
#25427=CARTESIAN_POINT('Ctrl Pts',(-5.36180135118839,-5.51555221991937,
3.2667531927192));
#25428=CARTESIAN_POINT('Ctrl Pts',(-2.08872307601302,-7.40320646287767,
3.42472221964149));
#25429=CARTESIAN_POINT('Ctrl Pts',(1.68831124821834,-7.50465423250149,3.58269124656378));
#25430=CARTESIAN_POINT('Ctrl Pts',(5.05799876999421,-5.79541874785593,3.74066027348607));
#25431=CARTESIAN_POINT('Ctrl Pts',(7.20731911838588,-2.68789530041857,3.89862930040836));
#25432=CARTESIAN_POINT('Ctrl Pts',(7.6176956551735,1.06814929921513,4.05659832733065));
#25433=CARTESIAN_POINT('Ctrl Pts',(6.19011490150972,4.56647648919493,4.21456735425294));
#25434=CARTESIAN_POINT('Ctrl Pts',(3.26901598605976,6.96302840028308,4.37253638117523));
#25435=CARTESIAN_POINT('Ctrl Pts',(-0.440813804993028,7.67957767130397,
4.53050540809751));
#25436=CARTESIAN_POINT('Ctrl Pts',(-4.04428637421744,6.54323908653675,4.68847443501981));
#25437=CARTESIAN_POINT('Ctrl Pts',(-6.67197493176133,3.82818240555635,4.84644346194209));
#25438=CARTESIAN_POINT('Ctrl Pts',(-7.68988468970048,0.189482134707461,
5.0044124888644));
#25439=CARTESIAN_POINT('Ctrl Pts',(-6.85241976900343,-3.49493538275516,
5.16238151578668));
#25440=CARTESIAN_POINT('Ctrl Pts',(-4.36163927338976,-6.33611338827574,
5.32035054270897));
#25441=CARTESIAN_POINT('Ctrl Pts',(-0.818505538197435,-7.6485474898312,
5.47831956963126));
#25442=CARTESIAN_POINT('Ctrl Pts',(2.92211288124885,-7.1155805335547,5.63628859655355));
#25443=CARTESIAN_POINT('Ctrl Pts',(5.95769937021023,-4.86580396588883,5.79425762347584));
#25444=CARTESIAN_POINT('Ctrl Pts',(7.5558436867006,-1.44203196996787,5.95222665039812));
#25445=CARTESIAN_POINT('Ctrl Pts',(7.33095402833655,2.32966586760398,6.11019567732041));
#25446=CARTESIAN_POINT('Ctrl Pts',(5.33729058164263,5.5392742545727,6.26816470424272));
#25447=CARTESIAN_POINT('Ctrl Pts',(2.05587391142296,7.41239586642492,6.42613373116499));
#25448=CARTESIAN_POINT('Ctrl Pts',(-1.7215731352771,7.49709383429043,6.58410275808729));
#25449=CARTESIAN_POINT('Ctrl Pts',(-5.08364812745316,5.77293268075287,6.74207178500957));
#25450=CARTESIAN_POINT('Ctrl Pts',(-7.21916740502853,2.65590888368507,6.90004081193188));
#25451=CARTESIAN_POINT('Ctrl Pts',(-7.61288417910656,-1.10191855224044,
7.05800983885415));
#25452=CARTESIAN_POINT('Ctrl Pts',(-6.16980455021368,-4.59388091186788,
7.21597886577645));
#25453=CARTESIAN_POINT('Ctrl Pts',(-3.2381071336009,-6.97745599854215,7.37394789269874));
#25454=CARTESIAN_POINT('Ctrl Pts',(0.474863634280211,-7.67754743059828,
7.53191691962102));
#25455=CARTESIAN_POINT('Ctrl Pts',(4.07326181773498,-6.52524085260257,7.68988594654333));
#25456=CARTESIAN_POINT('Ctrl Pts',(6.68888494784978,-3.79855869701265,7.84785497346561));
#25457=CARTESIAN_POINT('Ctrl Pts',(7.69064931918003,-0.155380403180869,
8.00582400038789));
#25458=CARTESIAN_POINT('Ctrl Pts',(6.83685452611142,3.52528725199694,8.1637930273102));
#25459=CARTESIAN_POINT('Ctrl Pts',(4.3334996575679,6.35539225680518,8.32176205423247));
#25460=CARTESIAN_POINT('Ctrl Pts',(0.784580926987224,7.65210185439399,8.47973108115477));
#25461=CARTESIAN_POINT('Ctrl Pts',(-2.95363733713913,7.10255281566796,8.63770010807706));
#25462=CARTESIAN_POINT('Ctrl Pts',(-5.97921761703337,4.83933742478764,8.79566913499935));
#25463=CARTESIAN_POINT('Ctrl Pts',(-7.5621639155084,1.40851231180965,8.95363816192163));
#25464=CARTESIAN_POINT('Ctrl Pts',(-7.32055132824183,-2.36215119554395,
9.11160718884394));
#25465=CARTESIAN_POINT('Ctrl Pts',(-5.3126748601556,-5.56288736733038,9.26957621576621));
#25466=CARTESIAN_POINT('Ctrl Pts',(-2.02298432131397,-7.4214395112426,9.42754524268851));
#25467=CARTESIAN_POINT('Ctrl Pts',(1.75480117121603,-7.48938601984247,9.5855142696108));
#25468=CARTESIAN_POINT('Ctrl Pts',(5.10919751789325,-5.75033308551119,9.74348329653307));
#25469=CARTESIAN_POINT('Ctrl Pts',(7.23087374123971,-2.62387026150611,9.90145232345539));
#25470=CARTESIAN_POINT('Ctrl Pts',(7.60792299304672,1.13566617592857,10.0594213503777));
#25471=CARTESIAN_POINT('Ctrl Pts',(6.14937289953934,4.62119492633867,10.2173903773));
#25472=CARTESIAN_POINT('Ctrl Pts',(3.20713456379208,6.99174653894661,10.3753594042223));
#25473=CARTESIAN_POINT('Ctrl Pts',(-0.508904040873067,7.67536593721493,
10.5333284311446));
#25474=CARTESIAN_POINT('Ctrl Pts',(-4.10215733057928,6.50711485672321,10.6912974580669));
#25475=CARTESIAN_POINT('Ctrl Pts',(-6.70566311401509,3.7688592275556,10.8492664849892));
#25476=CARTESIAN_POINT('Ctrl Pts',(-7.69126334438516,0.121277688201066,
11.0072355119115));
#25477=CARTESIAN_POINT('Ctrl Pts',(-6.82115363397089,-3.55557382490135,
11.1652045388337));
#25478=CARTESIAN_POINT('Ctrl Pts',(-4.30527717987661,-6.37453833768985,
11.323173565756));
#25479=CARTESIAN_POINT('Ctrl Pts',(-0.750636320996575,-7.65552093138916,
11.4811425926783));
#25480=CARTESIAN_POINT('Ctrl Pts',(2.98509484260074,-7.08935594320191,11.6391116196006));
#25481=CARTESIAN_POINT('Ctrl Pts',(6.00063552237091,-4.81283303884795,11.7970806465229));
#25482=CARTESIAN_POINT('Ctrl Pts',(7.56830193781019,-1.37485328711205,11.9550496734452));
#25483=CARTESIAN_POINT('Ctrl Pts',(7.31007010305476,2.39436967024001,12.1130187003675));
#25484=CARTESIAN_POINT('Ctrl Pts',(5.28782408555519,5.58685463551785,12.2709877272898));
#25485=CARTESIAN_POINT('Ctrl Pts',(3.08950446577676,6.81500585228764,12.3763004119046));
#25486=CARTESIAN_POINT('Ctrl Pts',(1.90986937676202,7.13094557024913,12.4289567542121));
#25487=CARTESIAN_POINT('Ctrl Pts',(5.87253250007098,-5.06341606878912,-12.4288646816028));
#25488=CARTESIAN_POINT('Ctrl Pts',(6.71028886424398,-4.09179223917321,-12.376199525329));
#25489=CARTESIAN_POINT('Ctrl Pts',(7.89339297136583,-1.72594434552226,-12.270878026748));
#25490=CARTESIAN_POINT('Ctrl Pts',(7.76241299472572,2.24149547124628,-12.1129001858595));
#25491=CARTESIAN_POINT('Ctrl Pts',(5.75889308919358,5.66689674698945,-11.9549311589372));
#25492=CARTESIAN_POINT('Ctrl Pts',(2.36574065518254,7.72551452263309,-11.7969621320149));
#25493=CARTESIAN_POINT('Ctrl Pts',(-1.59812526523981,7.91990798831724,-11.6389931050926));
#25494=CARTESIAN_POINT('Ctrl Pts',(-5.17644500889257,6.20355806126057,-11.4810240781703));
#25495=CARTESIAN_POINT('Ctrl Pts',(-7.505798384084,2.99037951986057,-11.323055051248));
#25496=CARTESIAN_POINT('Ctrl Pts',(-8.02420331949211,-0.944267493446741,
-11.1650860243257));
#25497=CARTESIAN_POINT('Ctrl Pts',(-6.60656535064672,-4.65110439136602,
-11.0071169974035));
#25498=CARTESIAN_POINT('Ctrl Pts',(-3.59493314087816,-7.23573830051147,
-10.8491479704812));
#25499=CARTESIAN_POINT('Ctrl Pts',(0.28406699403406,-8.07457627271411,-10.6911789435589));
#25500=CARTESIAN_POINT('Ctrl Pts',(4.09452818435197,-6.96522079499565,-10.5332099166366));
#25501=CARTESIAN_POINT('Ctrl Pts',(6.91708367815401,-4.17533495487158,-10.3752408897143));
#25502=CARTESIAN_POINT('Ctrl Pts',(8.07072162883429,-0.378045753058428,
-10.217271862792));
#25503=CARTESIAN_POINT('Ctrl Pts',(7.27709868404176,3.51045599665256,-10.0593028358697));
#25504=CARTESIAN_POINT('Ctrl Pts',(4.7276958296943,6.5519736730373,-9.90133380894741));
#25505=CARTESIAN_POINT('Ctrl Pts',(1.0376195748737,8.01266573078172,-9.7433647820251));
#25506=CARTESIAN_POINT('Ctrl Pts',(-2.90280805351734,7.54010425375498,-9.58539575510284));
#25507=CARTESIAN_POINT('Ctrl Pts',(-6.1428615107626,5.24830630572554,-9.42742672818051));
#25508=CARTESIAN_POINT('Ctrl Pts',(-7.90079785801961,1.69022480126632,-9.26945770125828));
#25509=CARTESIAN_POINT('Ctrl Pts',(-7.75247151172096,-2.27566520375718,
-9.11148867433593));
#25510=CARTESIAN_POINT('Ctrl Pts',(-5.733669870614,-5.69249474937794,-8.95351964741368));
#25511=CARTESIAN_POINT('Ctrl Pts',(-2.33147870849099,-7.7358692914587,-8.79555062049136));
#25512=CARTESIAN_POINT('Ctrl Pts',(1.63323929662484,-7.91277423272776,-8.63758159356908));
#25513=CARTESIAN_POINT('Ctrl Pts',(5.20389796842962,-6.18052688651141,-8.47961256664679));
#25514=CARTESIAN_POINT('Ctrl Pts',(7.518987680364,-2.95707472379959,-8.3216435397245));
#25515=CARTESIAN_POINT('Ctrl Pts',(8.01993583962579,0.9798447776149,-8.16367451280222));
#25516=CARTESIAN_POINT('Ctrl Pts',(6.5858763255994,4.68035251704791,-8.00570548587992));
#25517=CARTESIAN_POINT('Ctrl Pts',(3.56281142798924,7.2516095722559,-7.84773645895763));
#25518=CARTESIAN_POINT('Ctrl Pts',(-0.319869754522884,8.07323664957635,
-7.68976743203535));
#25519=CARTESIAN_POINT('Ctrl Pts',(-4.12537445559599,6.94699591629286,-7.53179840511305));
#25520=CARTESIAN_POINT('Ctrl Pts',(-6.9355306418797,4.1446207758303,-7.37382937819076));
#25521=CARTESIAN_POINT('Ctrl Pts',(-8.07231870170907,0.342253470291336,
-7.21586035126847));
#25522=CARTESIAN_POINT('Ctrl Pts',(-7.26146042854604,-3.5426909411561,-7.05789132434619));
#25523=CARTESIAN_POINT('Ctrl Pts',(-4.69859541501031,-6.57287363228098,
-6.8999222974239));
#25524=CARTESIAN_POINT('Ctrl Pts',(-1.00207816741164,-8.01718816083833,
-6.7419532705016));
#25525=CARTESIAN_POINT('Ctrl Pts',(2.93621519684588,-7.52715796152183,-6.58398424357932));
#25526=CARTESIAN_POINT('Ctrl Pts',(6.16607409854881,-5.22101492730056,-6.42601521665703));
#25527=CARTESIAN_POINT('Ctrl Pts',(7.90821527616617,-1.65517304403557,-6.26804618973472));
#25528=CARTESIAN_POINT('Ctrl Pts',(7.74230412677602,2.31002023116615,-6.11007716281246));
#25529=CARTESIAN_POINT('Ctrl Pts',(5.70837081440596,5.7178640509484,-5.95210813589015));
#25530=CARTESIAN_POINT('Ctrl Pts',(2.29715200391916,7.74613189474464,-5.79413910896788));
#25531=CARTESIAN_POINT('Ctrl Pts',(-1.66831148422301,7.90545403196422,-5.63617008204558));
#25532=CARTESIAN_POINT('Ctrl Pts',(-5.23125360711624,6.15739006056327,-5.4782010551233));
#25533=CARTESIAN_POINT('Ctrl Pts',(-7.53202654648873,2.92370360380095,-5.32023202820099));
#25534=CARTESIAN_POINT('Ctrl Pts',(-8.0155119845431,-1.01539858456457,-5.16226300127872));
#25535=CARTESIAN_POINT('Ctrl Pts',(-6.56505711366871,-4.70951077651998,
-5.00429397435641));
#25536=CARTESIAN_POINT('Ctrl Pts',(-3.5306200084683,-7.26733713375767,-4.84632494743412));
#25537=CARTESIAN_POINT('Ctrl Pts',(0.355666406302637,-8.07173885029227,
-4.68835592051184));
#25538=CARTESIAN_POINT('Ctrl Pts',(4.15613951295213,-6.92863413731507,-4.53038689358954));
#25539=CARTESIAN_POINT('Ctrl Pts',(6.95384127459843,-4.11382525000531,-4.37241786666726));
#25540=CARTESIAN_POINT('Ctrl Pts',(8.07375701723909,-0.30645437910471,-4.21444883974496));
#25541=CARTESIAN_POINT('Ctrl Pts',(7.24567939772833,3.57485618245337,-4.05647981282269));
#25542=CARTESIAN_POINT('Ctrl Pts',(4.66940260143842,6.59364436450509,-3.89851078590038));
#25543=CARTESIAN_POINT('Ctrl Pts',(0.966517058638944,8.0215529316492,-3.7405417589781));
#25544=CARTESIAN_POINT('Ctrl Pts',(-2.9695646047045,7.51406366211892,-3.5825727320558));
#25545=CARTESIAN_POINT('Ctrl Pts',(-6.18916543686952,5.19362088094133,-3.42460370513352));
#25546=CARTESIAN_POINT('Ctrl Pts',(-7.91547718905155,1.62008874124048,-3.26663467821122));
#25547=CARTESIAN_POINT('Ctrl Pts',(-7.73198449831937,-2.344329835505,-3.10866565128894));
#25548=CARTESIAN_POINT('Ctrl Pts',(-5.68295950994386,-5.74312091708233,
-2.95069662436664));
#25549=CARTESIAN_POINT('Ctrl Pts',(-2.26278012850095,-7.75624217968669,
-2.79272759744436));
#25550=CARTESIAN_POINT('Ctrl Pts',(1.70335086641213,-7.89797837967305,-2.63475857052206));
#25551=CARTESIAN_POINT('Ctrl Pts',(5.25850637939024,-6.13413215685821,-2.47678954359978));
#25552=CARTESIAN_POINT('Ctrl Pts',(7.54491730419073,-2.89027499259379,-2.31882051667748));
#25553=CARTESIAN_POINT('Ctrl Pts',(8.01093051388007,1.05093242488527,-2.1608514897552));
#25554=CARTESIAN_POINT('Ctrl Pts',(6.5441088076344,4.73857642902715,-2.0028824628329));
#25555=CARTESIAN_POINT('Ctrl Pts',(3.49835916347221,7.28292179164652,-1.84491343591062));
#25556=CARTESIAN_POINT('Ctrl Pts',(-0.391456064322818,8.07008232979038,
-1.68694440898833));
#25557=CARTESIAN_POINT('Ctrl Pts',(-4.18682284472876,6.91013611492184,-1.52897538206604));
#25558=CARTESIAN_POINT('Ctrl Pts',(-6.97201516823428,4.08294883066162,-1.37100635514375));
#25559=CARTESIAN_POINT('Ctrl Pts',(-8.07503657186441,0.270649261854018,
-1.21303732822146));
#25560=CARTESIAN_POINT('Ctrl Pts',(-7.22975588917528,-3.60695112842209,
-1.05506830129917));
#25561=CARTESIAN_POINT('Ctrl Pts',(-4.64011796957429,-6.61428544049345,
-0.897099274376876));
#25562=CARTESIAN_POINT('Ctrl Pts',(-0.93093694444881,-8.02575996808715,
-0.739130247454587));
#25563=CARTESIAN_POINT('Ctrl Pts',(3.00285561957928,-7.5008216075208,-0.581161220532296));
#25564=CARTESIAN_POINT('Ctrl Pts',(6.21213507255517,-5.166124708156,-0.423192193610008));
#25565=CARTESIAN_POINT('Ctrl Pts',(7.92258345341839,-1.58497258131202,-0.265223166687717));
#25566=CARTESIAN_POINT('Ctrl Pts',(7.72151282951138,2.378593341364,-0.107254139765427));
#25567=CARTESIAN_POINT('Ctrl Pts',(5.65743645678892,5.76826485152039,0.0507148871568628));
#25568=CARTESIAN_POINT('Ctrl Pts',(2.22836375818162,7.76619994727875,0.208683914079155));
#25569=CARTESIAN_POINT('Ctrl Pts',(-1.73835675421644,7.89034742295674,0.366652941001444));
#25570=CARTESIAN_POINT('Ctrl Pts',(-5.28565574934141,6.11075363268263,0.524621967923734));
#25571=CARTESIAN_POINT('Ctrl Pts',(-7.55765969999705,2.85678954753941,0.682590994846022));
#25572=CARTESIAN_POINT('Ctrl Pts',(-8.00619151772145,-1.08644559985997,
0.840560021768314));
#25573=CARTESIAN_POINT('Ctrl Pts',(-6.52303181942251,-4.76754890302042,
0.998529048690603));
#25574=CARTESIAN_POINT('Ctrl Pts',(-3.46602952737128,-7.29836323947227,
1.15649807561289));
#25575=CARTESIAN_POINT('Ctrl Pts',(0.42723802482138,-8.06826712064225,1.31446710253518));
#25576=CARTESIAN_POINT('Ctrl Pts',(4.21742384757461,-6.89150221285597,1.47243612945747));
#25577=CARTESIAN_POINT('Ctrl Pts',(6.99005196541889,-4.05199212494712,1.63040515637976));
#25578=CARTESIAN_POINT('Ctrl Pts',(8.07615734042419,-0.234838822604965,
1.78837418330205));
#25579=CARTESIAN_POINT('Ctrl Pts',(7.21369021600383,3.6389751479531,1.94634321022434));
#25580=CARTESIAN_POINT('Ctrl Pts',(4.61074209526571,6.63479645436352,2.10431223714663));
#25581=CARTESIAN_POINT('Ctrl Pts',(0.895338524482194,8.0298091874258,2.26228126406892));
#25582=CARTESIAN_POINT('Ctrl Pts',(-3.03608758684171,7.48743205811683,2.42025029099121));
#25583=CARTESIAN_POINT('Ctrl Pts',(-6.23498255393503,5.13852694962435,2.5782193179135));
#25584=CARTESIAN_POINT('Ctrl Pts',(-7.92953392953035,1.54982525476801,2.73618834483579));
#25585=CARTESIAN_POINT('Ctrl Pts',(-7.71088932626506,-2.41281007499168,
2.89415737175808));
#25586=CARTESIAN_POINT('Ctrl Pts',(-5.63180215682195,-5.79329535983672,
3.05212639868037));
#25587=CARTESIAN_POINT('Ctrl Pts',(-2.19390356971854,-7.77600500171303,
3.21009542560265));
#25588=CARTESIAN_POINT('Ctrl Pts',(1.77332845928644,-7.88256131186905,3.36806445252495));
#25589=CARTESIAN_POINT('Ctrl Pts',(5.31270118310939,-6.08725494774761,3.52603347944724));
#25590=CARTESIAN_POINT('Ctrl Pts',(7.57025348334349,-2.82324792708962,3.68400250636953));
#25591=CARTESIAN_POINT('Ctrl Pts',(8.00129508925402,1.12193741116395,3.84197153329182));
#25592=CARTESIAN_POINT('Ctrl Pts',(6.50182656348719,4.79642762879022,3.99994056021411));
#25593=CARTESIAN_POINT('Ctrl Pts',(3.43363173588971,7.31366117359706,4.15790958713639));
#25594=CARTESIAN_POINT('Ctrl Pts',(-0.463011584188287,8.06629325854182,
4.3158786140587));
#25595=CARTESIAN_POINT('Ctrl Pts',(-4.24794191975708,6.87273279753116,4.47384764098098));
#25596=CARTESIAN_POINT('Ctrl Pts',(-7.00795131147991,4.02095574158889,4.63181666790327));
#25597=CARTESIAN_POINT('Ctrl Pts',(-8.07711930087982,0.199023765527639,
4.78978569482556));
#25598=CARTESIAN_POINT('Ctrl Pts',(-7.19748269412656,-3.67092761133184,
4.94775472174785));
#25599=CARTESIAN_POINT('Ctrl Pts',(-4.58127555615453,-6.65517700279045,
5.10572374867013));
#25600=CARTESIAN_POINT('Ctrl Pts',(-0.859722498739969,-8.03370051004207,
5.26369277559244));
#25601=CARTESIAN_POINT('Ctrl Pts',(3.06925985302439,-7.47389527719666,5.42166180251471));
#25602=CARTESIAN_POINT('Ctrl Pts',(6.25770743174028,-5.11082814802378,5.57963082943701));
#25603=CARTESIAN_POINT('Ctrl Pts',(7.93632848071451,-1.51464745273923,5.7375998563593));
#25604=CARTESIAN_POINT('Ctrl Pts',(7.7001141974791,2.44697936355635,5.89556888328158));
#25605=CARTESIAN_POINT('Ctrl Pts',(5.60605711411115,5.81821194983595,6.05353791020388));
#25606=CARTESIAN_POINT('Ctrl Pts',(2.15940024073058,7.78565715018472,6.21150693712617));
#25607=CARTESIAN_POINT('Ctrl Pts',(-1.8082652939448,7.8746201995147,6.36947596404845));
#25608=CARTESIAN_POINT('Ctrl Pts',(-5.33964214887762,6.06363656412707,6.52744499097075));
#25609=CARTESIAN_POINT('Ctrl Pts',(-7.58269840658814,2.78965079080092,6.68541401789304));
#25610=CARTESIAN_POINT('Ctrl Pts',(-7.99624132476026,-1.15740716089275,
6.84338304481532));
#25611=CARTESIAN_POINT('Ctrl Pts',(-6.48049345680476,-4.82521203847034,
7.00135207173762));
#25612=CARTESIAN_POINT('Ctrl Pts',(-3.40116642609152,-7.3288152932056,7.15932109865991));
#25613=CARTESIAN_POINT('Ctrl Pts',(0.498776038978558,-8.0641607823018,7.3172901255822));
#25614=CARTESIAN_POINT('Ctrl Pts',(4.27837646117492,-6.85382823802765,7.47525915250449));
#25615=CARTESIAN_POINT('Ctrl Pts',(7.02571285444676,-3.98984029087707,7.63322817942678));
#25616=CARTESIAN_POINT('Ctrl Pts',(8.07792243431764,-0.163204794890052,
7.79119720634906));
#25617=CARTESIAN_POINT('Ctrl Pts',(7.18113364224099,3.70280789026489,7.94916623327137));
#25618=CARTESIAN_POINT('Ctrl Pts',(4.55171893167374,6.67542668498747,8.10713526019364));
#25619=CARTESIAN_POINT('Ctrl Pts',(0.824089567553389,8.03743385947071,8.26510428711594));
#25620=CARTESIAN_POINT('Ctrl Pts',(-3.10237176580277,7.46021153084213,8.42307331403823));
#25621=CARTESIAN_POINT('Ctrl Pts',(-6.28030925917329,5.08302884821862,8.58104234096052));
#25622=CARTESIAN_POINT('Ctrl Pts',(-7.94296697324716,1.4794398665668,8.73901136788281));
#25623=CARTESIAN_POINT('Ctrl Pts',(-7.68918765526074,-2.48110053440443,
8.89698039480511));
#25624=CARTESIAN_POINT('Ctrl Pts',(-5.5802018344612,-5.84301413302921,9.05494942172739));
#25625=CARTESIAN_POINT('Ctrl Pts',(-2.12485445054169,-7.79515620004759,
9.21291844864968));
#25626=CARTESIAN_POINT('Ctrl Pts',(1.84316657286411,-7.86652424757819,9.37088747557198));
#25627=CARTESIAN_POINT('Ctrl Pts',(5.36647811365167,-6.03989893550398,9.52885650249425));
#25628=CARTESIAN_POINT('Ctrl Pts',(7.59499423129414,-2.75599882019051,9.68682552941656));
#25629=CARTESIAN_POINT('Ctrl Pts',(7.99103031142311,1.19285419210965,9.84479455633884));
#25630=CARTESIAN_POINT('Ctrl Pts',(6.45903294254871,4.85390148732021,10.0027635832611));
#25631=CARTESIAN_POINT('Ctrl Pts',(3.36863419036948,7.34382545322469,10.1607326101834));
#25632=CARTESIAN_POINT('Ctrl Pts',(-0.534530596581897,8.06186943684965,
10.3187016371057));
#25633=CARTESIAN_POINT('Ctrl Pts',(-4.30872704690166,6.8347894829523,10.476670664028));
#25634=CARTESIAN_POINT('Ctrl Pts',(-7.0433359080081,3.958645264208,10.6346396909503));
#25635=CARTESIAN_POINT('Ctrl Pts',(-8.0785673795978,0.127384791276112,10.7926087178726));
#25636=CARTESIAN_POINT('Ctrl Pts',(-7.16464211030434,-3.7346195847746,10.9505777447949));
#25637=CARTESIAN_POINT('Ctrl Pts',(-4.5220752727013,-6.69553689283714,11.1085467717172));
#25638=CARTESIAN_POINT('Ctrl Pts',(-0.788435634721984,-8.04102510874207,
11.2665157986394));
#25639=CARTESIAN_POINT('Ctrl Pts',(3.1354133567725,-7.44635011189922,11.4244848255617));
#25640=CARTESIAN_POINT('Ctrl Pts',(6.30280569228859,-5.05518979784663,11.582453852484));
#25641=CARTESIAN_POINT('Ctrl Pts',(7.94941408401714,-1.4440858958632,11.7404228794063));
#25642=CARTESIAN_POINT('Ctrl Pts',(7.67817863371211,2.51494141425027,11.8983919063286));
#25643=CARTESIAN_POINT('Ctrl Pts',(5.5540996652784,5.86818830563099,12.0563609332509));
#25644=CARTESIAN_POINT('Ctrl Pts',(3.24508066864809,7.15818474870596,12.1616736178657));
#25645=CARTESIAN_POINT('Ctrl Pts',(2.00604344898242,7.49003404122904,12.2143299601732));
#25646=CARTESIAN_POINT('Ctrl Pts',(6.15407444028416,-5.30616721305205,-12.6434914756415));
#25647=CARTESIAN_POINT('Ctrl Pts',(7.03199466088407,-4.28796163047964,-12.5908263193679));
#25648=CARTESIAN_POINT('Ctrl Pts',(8.27181934397364,-1.80868985944361,-12.4855048207869));
#25649=CARTESIAN_POINT('Ctrl Pts',(8.13455990327747,2.3489576238944,-12.3275269798982));
#25650=CARTESIAN_POINT('Ctrl Pts',(6.0349869096692,5.93858006336376,-12.169557952976));
#25651=CARTESIAN_POINT('Ctrl Pts',(2.47915939132291,8.09589243843362,-12.0115889260537));
#25652=CARTESIAN_POINT('Ctrl Pts',(-1.67474285532958,8.29960554832456,-11.8536198991314));
#25653=CARTESIAN_POINT('Ctrl Pts',(-5.42461500560061,6.5009700845693,-11.6956508722091));
#25654=CARTESIAN_POINT('Ctrl Pts',(-7.86564263183886,3.13374479744483,-11.5376818452868));
#25655=CARTESIAN_POINT('Ctrl Pts',(-8.40890102379728,-0.989537724336396,
-11.3797128183645));
#25656=CARTESIAN_POINT('Ctrl Pts',(-6.92329841716338,-4.87408841988581,
-11.2217437914422));
#25657=CARTESIAN_POINT('Ctrl Pts',(-3.76728202977869,-7.58263528234616,
-11.0637747645199));
#25658=CARTESIAN_POINT('Ctrl Pts',(0.297685781609928,-8.46168896560967,
-10.9058057375976));
#25659=CARTESIAN_POINT('Ctrl Pts',(4.29082874280202,-7.29914858111052,-10.7478367106754));
#25660=CARTESIAN_POINT('Ctrl Pts',(7.24870366652204,-4.37550956509642,-10.5898676837531));
#25661=CARTESIAN_POINT('Ctrl Pts',(8.45764952174504,-0.396170086096032,
-10.4318986568308));
#25662=CARTESIAN_POINT('Ctrl Pts',(7.62597857233582,3.67875486810516,-10.2739296299085));
#25663=CARTESIAN_POINT('Ctrl Pts',(4.95435181782442,6.86608949616986,-10.1159606029862));
#25664=CARTESIAN_POINT('Ctrl Pts',(1.08736530694238,8.39681029806963,-9.95799157606393));
#25665=CARTESIAN_POINT('Ctrl Pts',(-3.04197496514258,7.90159319927995,-9.80002254914166));
#25666=CARTESIAN_POINT('Ctrl Pts',(-6.43736360984507,5.49992148880527,-9.64205352221935));
#25667=CARTESIAN_POINT('Ctrl Pts',(-8.27957923694806,1.77125784279299,-9.48408449529707));
#25668=CARTESIAN_POINT('Ctrl Pts',(-8.12414180402343,-2.38476552746483,
-9.32611546837478));
#25669=CARTESIAN_POINT('Ctrl Pts',(-6.0085544353048,-5.96540528948545,-9.16814644145249));
#25670=CARTESIAN_POINT('Ctrl Pts',(-2.44325485262408,-8.10674363732677,
-9.0101774145302));
#25671=CARTESIAN_POINT('Ctrl Pts',(1.71154032950948,-8.29212978502554,-8.85220838760791));
#25672=CARTESIAN_POINT('Ctrl Pts',(5.45338411953825,-6.47683474536908,-8.69423936068563));
#25673=CARTESIAN_POINT('Ctrl Pts',(7.87946425157805,-3.098843297253,-8.53627033376333));
#25674=CARTESIAN_POINT('Ctrl Pts',(8.4044289516939,1.02682066064222,-8.37830130684105));
#25675=CARTESIAN_POINT('Ctrl Pts',(6.90161751539969,4.90473876412536,-8.22033227991874));
#25676=CARTESIAN_POINT('Ctrl Pts',(3.73362033233122,7.59926745726833,-8.06236325299647));
#25677=CARTESIAN_POINT('Ctrl Pts',(-0.335205004060077,8.46028511803427,
-7.90439422607416));
#25678=CARTESIAN_POINT('Ctrl Pts',(-4.32315385116687,7.28004996220959,-7.7464251991519));
#25679=CARTESIAN_POINT('Ctrl Pts',(-7.26803501768335,4.34332288172089,-7.58845617222958));
#25680=CARTESIAN_POINT('Ctrl Pts',(-8.45932316175605,0.35866184369231,-7.43048714530731));
#25681=CARTESIAN_POINT('Ctrl Pts',(-7.60959058496652,-3.71253522573633,
-7.272518118385));
#25682=CARTESIAN_POINT('Ctrl Pts',(-4.92385626616827,-6.88799144477263,
-7.11454909146273));
#25683=CARTESIAN_POINT('Ctrl Pts',(-1.05011996734974,-8.40154954322816,
-6.95658006454043));
#25684=CARTESIAN_POINT('Ctrl Pts',(3.07698371935187,-7.88802623372847,-6.79861103761815));
#25685=CARTESIAN_POINT('Ctrl Pts',(6.46168905941665,-5.47132170252852,-6.64064201069584));
#25686=CARTESIAN_POINT('Ctrl Pts',(8.28735226220217,-1.73452562832534,-6.48267298377357));
#25687=CARTESIAN_POINT('Ctrl Pts',(8.11348697260047,2.42076760937246,-6.32470395685127));
#25688=CARTESIAN_POINT('Ctrl Pts',(5.9820424874916,5.99199085037602,-6.16673492992898));
#25689=CARTESIAN_POINT('Ctrl Pts',(2.40728245141181,8.11749825206445,-6.0087659030067));
#25690=CARTESIAN_POINT('Ctrl Pts',(-1.74829395382065,8.28445863796655,-5.8507968760844));
#25691=CARTESIAN_POINT('Ctrl Pts',(-5.48205124685291,6.45258868982236,-5.69282784916212));
#25692=CARTESIAN_POINT('Ctrl Pts',(-7.89312822921419,3.06387229341016,-5.53485882223982));
#25693=CARTESIAN_POINT('Ctrl Pts',(-8.39979300740726,-1.0640789941808,-5.37688979531754));
#25694=CARTESIAN_POINT('Ctrl Pts',(-6.87980018531119,-4.93529493377415,
-5.21892076839524));
#25695=CARTESIAN_POINT('Ctrl Pts',(-3.69988558636464,-7.61574903216721,
-5.06095174147296));
#25696=CARTESIAN_POINT('Ctrl Pts',(0.372717824936398,-8.45871551100516,
-4.90298271455066));
#25697=CARTESIAN_POINT('Ctrl Pts',(4.35539385207399,-7.26080787973768,-4.74501368762838));
#25698=CARTESIAN_POINT('Ctrl Pts',(7.28722350183364,-4.31105095162049,-4.58704466070608));
#25699=CARTESIAN_POINT('Ctrl Pts',(8.46083043325097,-0.321146466458664,
-4.4290756337838));
#25700=CARTESIAN_POINT('Ctrl Pts',(7.59305297731676,3.74624253843844,-4.2711066068615));
#25701=CARTESIAN_POINT('Ctrl Pts',(4.8932638858212,6.9097579709323,-4.11313757993922));
#25702=CARTESIAN_POINT('Ctrl Pts',(1.0128539819229,8.40612357061492,-3.95516855301692));
#25703=CARTESIAN_POINT('Ctrl Pts',(-3.11193197012765,7.8743041652226,-3.79719952609464));
#25704=CARTESIAN_POINT('Ctrl Pts',(-6.48588744656048,5.44261432619416,-3.63923049917234));
#25705=CARTESIAN_POINT('Ctrl Pts',(-8.29496232693573,1.69775930798845,-3.48126147225005));
#25706=CARTESIAN_POINT('Ctrl Pts',(-8.10267259878177,-2.45672209052951,
-3.32329244532776));
#25707=CARTESIAN_POINT('Ctrl Pts',(-5.95541290999965,-6.01845858543149,
-3.16532341840547));
#25708=CARTESIAN_POINT('Ctrl Pts',(-2.37126271376485,-8.12809324598661,
-3.00735439148318));
#25709=CARTESIAN_POINT('Ctrl Pts',(1.78501319996033,-8.27662458669668,-2.84938536456089));
#25710=CARTESIAN_POINT('Ctrl Pts',(5.5106105761161,-6.42821575178852,-2.6914163376386));
#25711=CARTESIAN_POINT('Ctrl Pts',(7.90663699778871,-3.02884104210559,-2.53344731071631));
#25712=CARTESIAN_POINT('Ctrl Pts',(8.39499189110759,1.10131640384692,-2.37547828379402));
#25713=CARTESIAN_POINT('Ctrl Pts',(6.85784757206785,4.96575405667938,-2.21750925687173));
#25714=CARTESIAN_POINT('Ctrl Pts',(3.66607808651513,7.63208085234415,-2.05954022994944));
#25715=CARTESIAN_POINT('Ctrl Pts',(-0.410223316757149,8.45697957331891,
-1.90157120302715));
#25716=CARTESIAN_POINT('Ctrl Pts',(-4.3875482093001,7.24142302204562,-1.74360217610486));
#25717=CARTESIAN_POINT('Ctrl Pts',(-7.30626869133298,4.2786942497907,-1.58563314918257));
#25718=CARTESIAN_POINT('Ctrl Pts',(-8.46217133249921,0.283624774258379,
-1.42766412226028));
#25719=CARTESIAN_POINT('Ctrl Pts',(-7.57636606124012,-3.77987618570152,
-1.26969509533799));
#25720=CARTESIAN_POINT('Ctrl Pts',(-4.86257528521387,-6.93138862485518,
-1.1117260684157));
#25721=CARTESIAN_POINT('Ctrl Pts',(-0.975568079917719,-8.41053230150091,
-0.953757041493409));
#25722=CARTESIAN_POINT('Ctrl Pts',(3.14681902843333,-7.86042725781713,-0.795788014571121));
#25723=CARTESIAN_POINT('Ctrl Pts',(6.50995829638106,-5.41379992727141,-0.63781898764883));
#25724=CARTESIAN_POINT('Ctrl Pts',(8.30240928102332,-1.66095960321813,-0.479849960726541));
#25725=CARTESIAN_POINT('Ctrl Pts',(8.09169889546763,2.49262826314565,-0.321880933804249));
#25726=CARTESIAN_POINT('Ctrl Pts',(5.92866622634028,6.04480797460074,-0.16391190688196));
#25727=CARTESIAN_POINT('Ctrl Pts',(2.33519634803474,8.13852841054634,-0.00594287995966794));
#25728=CARTESIAN_POINT('Ctrl Pts',(-1.82169734592179,8.2686277853708,0.152026146962621));
#25729=CARTESIAN_POINT('Ctrl Pts',(-5.53906154572492,6.40371641047728,0.309995173884911));
#25730=CARTESIAN_POINT('Ctrl Pts',(-7.91999029167661,2.99375023221594,0.4679642008072));
#25731=CARTESIAN_POINT('Ctrl Pts',(-8.39002569719858,-1.13853215742554,
0.625933227729491));
#25732=CARTESIAN_POINT('Ctrl Pts',(-6.83576010734434,-4.99611553389072,
0.783902254651781));
#25733=CARTESIAN_POINT('Ctrl Pts',(-3.63219849756608,-7.64826259665706,
0.941871281574071));
#25734=CARTESIAN_POINT('Ctrl Pts',(0.447720742020407,-8.4550773391087,1.09984030849636));
#25735=CARTESIAN_POINT('Ctrl Pts',(4.41961629056801,-7.22189577031478,1.25780933541865));
#25736=CARTESIAN_POINT('Ctrl Pts',(7.32517021167997,-4.24625341248742,1.41577836234094));
#25737=CARTESIAN_POINT('Ctrl Pts',(8.46334583313366,-0.246097504911587,
1.57374738926323));
#25738=CARTESIAN_POINT('Ctrl Pts',(7.55953016486508,3.8134355061597,1.73171641618552));
#25739=CARTESIAN_POINT('Ctrl Pts',(4.83179106780148,6.95288298119983,1.88968544310781));
#25740=CARTESIAN_POINT('Ctrl Pts',(0.938262994517446,8.41477564919374,2.0476544700301));
#25741=CARTESIAN_POINT('Ctrl Pts',(-3.18164420825611,7.84639578438501,2.20562349695239));
#25742=CARTESIAN_POINT('Ctrl Pts',(-6.53390113555359,5.38487907236143,2.36359252387468));
#25743=CARTESIAN_POINT('Ctrl Pts',(-8.30969297802931,1.62412723763715,2.52156155079697));
#25744=CARTESIAN_POINT('Ctrl Pts',(-8.08056607844303,-2.52848542116828,
2.67953057771926));
#25745=CARTESIAN_POINT('Ctrl Pts',(-5.90180296245549,-6.07103849975408,
2.83749960464155));
#25746=CARTESIAN_POINT('Ctrl Pts',(-2.29908406342406,-8.14880354054839,
2.99546863156383));
#25747=CARTESIAN_POINT('Ctrl Pts',(1.85834567035452,-8.26046839123662,3.15343765848613));
#25748=CARTESIAN_POINT('Ctrl Pts',(5.56740359622459,-6.3790911476393,3.31140668540842));
#25749=CARTESIAN_POINT('Ctrl Pts',(7.93318784830107,-2.95860055376065,3.46937571233071));
#25750=CARTESIAN_POINT('Ctrl Pts',(8.38489452333455,1.17572552311275,3.627344739253));
#25751=CARTESIAN_POINT('Ctrl Pts',(6.81353822546464,5.02637876838552,3.78531376617529));
#25752=CARTESIAN_POINT('Ctrl Pts',(3.59824748571965,7.66429394691102,3.94328279309757));
#25753=CARTESIAN_POINT('Ctrl Pts',(-0.485209363383541,8.45300884577968,
4.10125182001987));
#25754=CARTESIAN_POINT('Ctrl Pts',(-4.45159746529674,7.20222650852556,4.25922084694216));
#25755=CARTESIAN_POINT('Ctrl Pts',(-7.34392769119849,4.21372907762145,4.41718987386444));
#25756=CARTESIAN_POINT('Ctrl Pts',(-8.46435391205914,0.208565396347819,
4.57515890078674));
#25757=CARTESIAN_POINT('Ctrl Pts',(-7.54254561924968,-3.84691983990853,
4.73312792770903));
#25758=CARTESIAN_POINT('Ctrl Pts',(-4.80091183891932,-6.97424061730516,
4.89109695463132));
#25759=CARTESIAN_POINT('Ctrl Pts',(-0.900939459282501,-8.41885353025294,
5.04906598155361));
#25760=CARTESIAN_POINT('Ctrl Pts',(3.21640682479993,-7.83221002083862,5.2070350084759));
#25761=CARTESIAN_POINT('Ctrl Pts',(6.55771549327035,-5.35585233015872,5.36500403539819));
#25762=CARTESIAN_POINT('Ctrl Pts',(8.31681327472841,-1.58726293551058,5.52297306232048));
#25763=CARTESIAN_POINT('Ctrl Pts',(8.06927436662165,2.56429285950871,5.68094208924277));
#25764=CARTESIAN_POINT('Ctrl Pts',(5.87482364657965,6.0971496450992,5.83891111616505));
#25765=CARTESIAN_POINT('Ctrl Pts',(2.26292657003822,8.15891843394451,5.99688014308736));
#25766=CARTESIAN_POINT('Ctrl Pts',(-1.89495745261251,8.25214656473898,6.15484917000963));
#25767=CARTESIAN_POINT('Ctrl Pts',(-5.5956361703021,6.35434044750129,6.31281819693194));
#25768=CARTESIAN_POINT('Ctrl Pts',(-7.94622940814776,2.92339269791678,6.47078722385421));
#25769=CARTESIAN_POINT('Ctrl Pts',(-8.37959847041395,-1.21289576954504,
6.62875625077651));
#25770=CARTESIAN_POINT('Ctrl Pts',(-6.79118236339584,-5.05654316507279,
6.78672527769879));
#25771=CARTESIAN_POINT('Ctrl Pts',(-3.56422571858213,-7.68017458786904,
6.9446943046211));
#25772=CARTESIAN_POINT('Ctrl Pts',(0.522688443676895,-8.45077413400531,
7.10266333154337));
#25773=CARTESIAN_POINT('Ctrl Pts',(4.48349110461487,-7.18241562345274,7.26063235846567));
#25774=CARTESIAN_POINT('Ctrl Pts',(7.36254076104373,-4.18112188474151,7.41860138538795));
#25775=CARTESIAN_POINT('Ctrl Pts',(8.46519554945526,-0.171029186599225,
7.57657041231025));
#25776=CARTESIAN_POINT('Ctrl Pts',(7.52541275837057,3.88032852853282,7.73453943923254));
#25777=CARTESIAN_POINT('Ctrl Pts',(4.76993820577959,6.99546111316978,7.89250846615483));
#25778=CARTESIAN_POINT('Ctrl Pts',(0.863598208119548,8.4227658645474,8.05047749307711));
#25779=CARTESIAN_POINT('Ctrl Pts',(-3.2511061944664,7.81787024601633,8.20844651999941));
#25780=CARTESIAN_POINT('Ctrl Pts',(-6.58140090131321,5.32672027164962,8.36641554692169));
#25781=CARTESIAN_POINT('Ctrl Pts',(-8.3237700309859,1.55036742132396,8.524384573844));
#25782=CARTESIAN_POINT('Ctrl Pts',(-8.05782398227964,-2.60004987326493,
8.68235360076627));
#25783=CARTESIAN_POINT('Ctrl Pts',(-5.84772880876681,-6.12314089872802,
8.84032262768858));
#25784=CARTESIAN_POINT('Ctrl Pts',(-2.22672457976938,-8.16887288885258,
8.99829165461085));
#25785=CARTESIAN_POINT('Ctrl Pts',(1.9315319745122,-8.24366247531389,9.15626068153316));
#25786=CARTESIAN_POINT('Ctrl Pts',(5.62375870941011,-6.32946478549677,9.31422970845543));
#25787=CARTESIAN_POINT('Ctrl Pts',(7.95911472134858,-2.8881273788749,9.47219873537773));
#25788=CARTESIAN_POINT('Ctrl Pts',(8.37413762979948,1.25004220829073,9.63016776230001));
#25789=CARTESIAN_POINT('Ctrl Pts',(6.76869298555811,5.08660804830173,9.78813678922231));
#25790=CARTESIAN_POINT('Ctrl Pts',(3.53013381694687,7.69590436750279,9.94610581614459));
#25791=CARTESIAN_POINT('Ctrl Pts',(-0.560157152290724,8.44837293648434,
10.1040748430669));
#25792=CARTESIAN_POINT('Ctrl Pts',(-4.51529676322405,7.16246410918141,10.2620438699892));
#25793=CARTESIAN_POINT('Ctrl Pts',(-7.38100870200111,4.14843130086038,10.4200128969115));
#25794=CARTESIAN_POINT('Ctrl Pts',(-8.46587141481043,0.133491894351164,
10.5779819238338));
#25795=CARTESIAN_POINT('Ctrl Pts',(-7.50813058663781,-3.91366534464785,
10.7359509507561));
#25796=CARTESIAN_POINT('Ctrl Pts',(-4.73887336552598,-7.01653544798443,
10.8939199776784));
#25797=CARTESIAN_POINT('Ctrl Pts',(-0.82623494844739,-8.42652928609498,
11.0518890046007));
#25798=CARTESIAN_POINT('Ctrl Pts',(3.28573187094426,-7.80334428059651,11.2098580315229));
#25799=CARTESIAN_POINT('Ctrl Pts',(6.60497586220628,-5.2975465568453,11.3678270584453));
#25800=CARTESIAN_POINT('Ctrl Pts',(8.3305262302241,-1.51331850461435,11.5257960853675));
#25801=CARTESIAN_POINT('Ctrl Pts',(8.04628716436945,2.63551315826054,11.6837651122898));
#25802=CARTESIAN_POINT('Ctrl Pts',(5.82037524500162,6.14952197574412,11.8417341392121));
#25803=CARTESIAN_POINT('Ctrl Pts',(3.4006568715194,7.50136364512427,11.947046823827));
#25804=CARTESIAN_POINT('Ctrl Pts',(2.10221752120281,7.84912251220897,11.9997031661344));
#25805=CARTESIAN_POINT('Ctrl Pts',(2.10208451021619,7.84862588447234,12.));
#25806=CARTESIAN_POINT('Ctrl Pts',(2.2993955749037,7.78116612976009,12.));
#25807=CARTESIAN_POINT('Ctrl Pts',(2.49365425396881,7.70609002735957,12.));
#25808=CARTESIAN_POINT('Ctrl Pts',(2.68449722322631,7.62371149358249,12.));
#25809=CARTESIAN_POINT('Ctrl Pts',(2.87766974768538,7.54032739306849,12.));
#25810=CARTESIAN_POINT('Ctrl Pts',(3.06734326822009,7.44946115104765,12.));
#25811=CARTESIAN_POINT('Ctrl Pts',(3.25311885290036,7.35138992462918,12.));
#25812=CARTESIAN_POINT('Ctrl Pts',(3.43857588515895,7.25348686254041,12.));
#25813=CARTESIAN_POINT('Ctrl Pts',(3.62014888805913,7.1484030613508,12.));
#25814=CARTESIAN_POINT('Ctrl Pts',(3.79741044071271,7.03637241507993,12.));
#25815=CARTESIAN_POINT('Ctrl Pts',(3.97212170910349,6.92595356781374,12.));
#25816=CARTESIAN_POINT('Ctrl Pts',(4.14264513227527,6.80878584951957,12.));
#25817=CARTESIAN_POINT('Ctrl Pts',(4.30853456648212,6.68505947211609,12.));
#25818=CARTESIAN_POINT('Ctrl Pts',(4.45106252434089,6.57875693398944,12.));
#25819=CARTESIAN_POINT('Ctrl Pts',(4.59016935875685,6.46761224470133,12.));
#25820=CARTESIAN_POINT('Ctrl Pts',(4.72554610344008,6.35172956521935,12.));
#25821=CARTESIAN_POINT('Ctrl Pts',(4.74477333824113,6.33527102580781,12.));
#25822=CARTESIAN_POINT('Ctrl Pts',(4.76392528681677,6.31871689013953,12.));
#25823=CARTESIAN_POINT('Ctrl Pts',(4.78300101992008,6.30206743516809,12.));
#25824=CARTESIAN_POINT('Ctrl Pts',(4.80076087393577,6.28656649016472,12.));
#25825=CARTESIAN_POINT('Ctrl Pts',(4.81844738030779,6.27098927657102,12.));
#25826=CARTESIAN_POINT('Ctrl Pts',(4.83605920680848,6.25533688423888,12.));
#25827=CARTESIAN_POINT('Ctrl Pts',(4.98998560005503,6.11853583766523,12.));
#25828=CARTESIAN_POINT('Ctrl Pts',(5.13823022848562,5.97597793333321,12.));
#25829=CARTESIAN_POINT('Ctrl Pts',(5.28041162851553,5.82790909187815,12.));
#25830=CARTESIAN_POINT('Ctrl Pts',(5.32007318404608,5.78660523232639,12.));
#25831=CARTESIAN_POINT('Ctrl Pts',(5.35926272429222,5.74487232374225,12.));
#25832=CARTESIAN_POINT('Ctrl Pts',(5.39797144463401,5.70271520266631,12.));
#25833=CARTESIAN_POINT('Ctrl Pts',(5.537130358362,5.55115919350284,12.));
#25834=CARTESIAN_POINT('Ctrl Pts',(5.67007843940407,5.39412278727632,12.));
#25835=CARTESIAN_POINT('Ctrl Pts',(5.79659171893264,5.23204542006403,12.));
#25836=CARTESIAN_POINT('Ctrl Pts',(5.92308395052344,5.06999501756527,12.));
#25837=CARTESIAN_POINT('Ctrl Pts',(6.04314381607103,4.90290466616952,12.));
#25838=CARTESIAN_POINT('Ctrl Pts',(6.15650094748101,4.73119033909099,12.));
#25839=CARTESIAN_POINT('Ctrl Pts',(6.2685847071828,4.56140492608495,12.));
#25840=CARTESIAN_POINT('Ctrl Pts',(6.37411567049303,4.38709818588679,12.));
#25841=CARTESIAN_POINT('Ctrl Pts',(6.47278349045617,4.20865935363704,12.));
#25842=CARTESIAN_POINT('Ctrl Pts',(6.513215075432,4.13553961903878,12.));
#25843=CARTESIAN_POINT('Ctrl Pts',(6.5524936416175,4.06172594633208,12.));
#25844=CARTESIAN_POINT('Ctrl Pts',(6.59059530005883,3.98724486707222,12.));
#25845=CARTESIAN_POINT('Ctrl Pts',(6.60144172391569,3.9660422898612,12.));
#25846=CARTESIAN_POINT('Ctrl Pts',(6.61219276480136,3.94478562751987,12.));
#25847=CARTESIAN_POINT('Ctrl Pts',(6.62284784887895,3.92347549186304,12.));
#25848=CARTESIAN_POINT('Ctrl Pts',(6.63395017824082,3.90127086700178,12.));
#25849=CARTESIAN_POINT('Ctrl Pts',(6.64494485731741,3.87901508077576,12.));
#25850=CARTESIAN_POINT('Ctrl Pts',(6.65582886903515,3.85671429060614,12.));
#25851=CARTESIAN_POINT('Ctrl Pts',(6.74450049831353,3.6750306017405,12.));
#25852=CARTESIAN_POINT('Ctrl Pts',(6.82588701041696,3.4902491840288,12.));
#25853=CARTESIAN_POINT('Ctrl Pts',(6.89978215802754,3.3027870592376,12.));
#25854=CARTESIAN_POINT('Ctrl Pts',(6.97319794282983,3.11654101389823,12.));
#25855=CARTESIAN_POINT('Ctrl Pts',(7.03921944722408,2.92764827349166,12.));
#25856=CARTESIAN_POINT('Ctrl Pts',(7.09759598956962,2.73650163287192,12.));
#25857=CARTESIAN_POINT('Ctrl Pts',(7.13572390237701,2.6116565811758,12.));
#25858=CARTESIAN_POINT('Ctrl Pts',(7.17058956880297,2.48584973539685,12.));
#25859=CARTESIAN_POINT('Ctrl Pts',(7.20211123195996,2.35918876245082,12.));
#25860=CARTESIAN_POINT('Ctrl Pts',(7.25235994792851,2.15727837396125,12.));
#25861=CARTESIAN_POINT('Ctrl Pts',(7.29411388123278,1.95319690708858,12.));
#25862=CARTESIAN_POINT('Ctrl Pts',(7.32732391013097,1.74748626497986,12.));
#25863=CARTESIAN_POINT('Ctrl Pts',(7.36053393902917,1.54177562287114,12.));
#25864=CARTESIAN_POINT('Ctrl Pts',(7.38520001023308,1.33443494496339,12.));
#25865=CARTESIAN_POINT('Ctrl Pts',(7.40121439147182,1.12601971526756,12.));
#25866=CARTESIAN_POINT('Ctrl Pts',(7.40333855631591,1.09837529383825,12.));
#25867=CARTESIAN_POINT('Ctrl Pts',(7.40531048989455,1.07071006825862,12.));
#25868=CARTESIAN_POINT('Ctrl Pts',(7.40712860673866,1.04304720983276,12.));
#25869=CARTESIAN_POINT('Ctrl Pts',(7.42012496900755,0.845306052184669,12.));
#25870=CARTESIAN_POINT('Ctrl Pts',(7.42528630994362,0.647440157454434,12.));
#25871=CARTESIAN_POINT('Ctrl Pts',(7.42264771266255,0.449916696084704,12.));
#25872=CARTESIAN_POINT('Ctrl Pts',(7.42001587668523,0.252899380964936,12.));
#25873=CARTESIAN_POINT('Ctrl Pts',(7.40962392243267,0.0562220340153437,
12.));
#25874=CARTESIAN_POINT('Ctrl Pts',(7.39145489568746,-0.139648191421885,
12.));
#25875=CARTESIAN_POINT('Ctrl Pts',(7.37321585338488,-0.336273215847537,
12.));
#25876=CARTESIAN_POINT('Ctrl Pts',(7.34713964605262,-0.532085602194281,
12.));
#25877=CARTESIAN_POINT('Ctrl Pts',(7.31315786408237,-0.726598445503667,
12.));
#25878=CARTESIAN_POINT('Ctrl Pts',(7.27917608211211,-0.921111288813166,
12.));
#25879=CARTESIAN_POINT('Ctrl Pts',(7.23728866332716,-1.11432529315272,12.));
#25880=CARTESIAN_POINT('Ctrl Pts',(7.18737683938923,-1.30572860229433,12.));
#25881=CARTESIAN_POINT('Ctrl Pts',(7.16523608896148,-1.39063459378882,12.));
#25882=CARTESIAN_POINT('Ctrl Pts',(7.14151561885176,-1.47518388140826,12.));
#25883=CARTESIAN_POINT('Ctrl Pts',(7.11622968392941,-1.55933456450703,12.));
#25884=CARTESIAN_POINT('Ctrl Pts',(7.10233271500884,-1.60558317786698,12.));
#25885=CARTESIAN_POINT('Ctrl Pts',(7.08796315084845,-1.65171049254164,12.));
#25886=CARTESIAN_POINT('Ctrl Pts',(7.07312223633881,-1.69771223079685,12.));
#25887=CARTESIAN_POINT('Ctrl Pts',(7.06252436973796,-1.73056197769887,12.));
#25888=CARTESIAN_POINT('Ctrl Pts',(7.05168654638728,-1.7633460344081,12.));
#25889=CARTESIAN_POINT('Ctrl Pts',(7.04061734109932,-1.79603977805719,12.));
#25890=CARTESIAN_POINT('Ctrl Pts',(6.97824817218232,-1.98025188426835,12.));
#25891=CARTESIAN_POINT('Ctrl Pts',(6.90848807259781,-2.16175440386442,12.));
#25892=CARTESIAN_POINT('Ctrl Pts',(6.83157468295091,-2.34012772594946,12.));
#25893=CARTESIAN_POINT('Ctrl Pts',(6.75497532969541,-2.51777275202981,12.));
#25894=CARTESIAN_POINT('Ctrl Pts',(6.67128054581601,-2.69231466539617,12.));
#25895=CARTESIAN_POINT('Ctrl Pts',(6.58068264439258,-2.86331016587819,12.));
#25896=CARTESIAN_POINT('Ctrl Pts',(6.51303849241552,-2.9909825008911,12.));
#25897=CARTESIAN_POINT('Ctrl Pts',(6.44154513262403,-3.11667726450743,12.));
#25898=CARTESIAN_POINT('Ctrl Pts',(6.36626922705372,-3.24019647327262,12.));
#25899=CARTESIAN_POINT('Ctrl Pts',(6.35043403973881,-3.26618021658287,12.));
#25900=CARTESIAN_POINT('Ctrl Pts',(6.33443045294555,-3.29206910662706,12.));
#25901=CARTESIAN_POINT('Ctrl Pts',(6.31826810629452,-3.31784702529636,12.));
#25902=CARTESIAN_POINT('Ctrl Pts',(6.21663338793026,-3.47994796029905,12.));
#25903=CARTESIAN_POINT('Ctrl Pts',(6.10865101626227,-3.63778508614921,12.));
#25904=CARTESIAN_POINT('Ctrl Pts',(5.99452112172698,-3.79093554697371,12.));
#25905=CARTESIAN_POINT('Ctrl Pts',(5.88191571077627,-3.94204030921547,12.));
#25906=CARTESIAN_POINT('Ctrl Pts',(5.76332545224429,-4.08858324137673,12.));
#25907=CARTESIAN_POINT('Ctrl Pts',(5.63890846560756,-4.23012100294325,12.));
#25908=CARTESIAN_POINT('Ctrl Pts',(5.58859724884651,-4.2873554465232,12.));
#25909=CARTESIAN_POINT('Ctrl Pts',(5.53733289223766,-4.34377097889626,12.));
#25910=CARTESIAN_POINT('Ctrl Pts',(5.48512449108001,-4.39933625912035,12.));
#25911=CARTESIAN_POINT('Ctrl Pts',(5.4281364310843,-4.45998851915656,12.));
#25912=CARTESIAN_POINT('Ctrl Pts',(5.37002354987676,-4.5196277380235,12.));
#25913=CARTESIAN_POINT('Ctrl Pts',(5.31081700063339,-4.57822770314263,12.));
#25914=CARTESIAN_POINT('Ctrl Pts',(5.31037376991254,-4.57794244025905,-12.));
#25915=CARTESIAN_POINT('Ctrl Pts',(5.44267363655215,-4.44683792433415,-12.));
#25916=CARTESIAN_POINT('Ctrl Pts',(5.56937771169702,-4.31060781960146,-12.));
#25917=CARTESIAN_POINT('Ctrl Pts',(5.6903584571106,-4.16972393460644,-12.));
#25918=CARTESIAN_POINT('Ctrl Pts',(5.8143418732599,-4.02534339469196,-12.));
#25919=CARTESIAN_POINT('Ctrl Pts',(5.93231481872001,-3.87607486581971,-12.));
#25920=CARTESIAN_POINT('Ctrl Pts',(6.04411419453926,-3.72237753023135,-12.));
#25921=CARTESIAN_POINT('Ctrl Pts',(6.15675534768411,-3.56752295265345,-12.));
#25922=CARTESIAN_POINT('Ctrl Pts',(6.26313006821541,-3.40817211459952,-12.));
#25923=CARTESIAN_POINT('Ctrl Pts',(6.36303861860623,-3.24475251660394,-12.));
#25924=CARTESIAN_POINT('Ctrl Pts',(6.45945119635235,-3.08705125244431,-12.));
#25925=CARTESIAN_POINT('Ctrl Pts',(6.54984238090044,-2.92556030592911,-12.));
#25926=CARTESIAN_POINT('Ctrl Pts',(6.63399797028678,-2.76063397584875,-12.));
#25927=CARTESIAN_POINT('Ctrl Pts',(6.67607576497995,-2.67817081080857,-12.));
#25928=CARTESIAN_POINT('Ctrl Pts',(6.71659409382163,-2.59484838741849,-12.));
#25929=CARTESIAN_POINT('Ctrl Pts',(6.7555225444137,-2.51070882516395,-12.));
#25930=CARTESIAN_POINT('Ctrl Pts',(6.77498676970973,-2.46863904403668,-12.));
#25931=CARTESIAN_POINT('Ctrl Pts',(6.79405348565133,-2.42636495809896,-12.));
#25932=CARTESIAN_POINT('Ctrl Pts',(6.81271864440367,-2.38389172142662,-12.));
#25933=CARTESIAN_POINT('Ctrl Pts',(6.82488864469961,-2.35619845025061,-12.));
#25934=CARTESIAN_POINT('Ctrl Pts',(6.83688874062191,-2.32841859568406,-12.));
#25935=CARTESIAN_POINT('Ctrl Pts',(6.84871511036648,-2.30055985767388,-12.));
#25936=CARTESIAN_POINT('Ctrl Pts',(6.85502687237034,-2.28569158212981,-12.));
#25937=CARTESIAN_POINT('Ctrl Pts',(6.86128851596274,-2.27080232980739,-12.));
#25938=CARTESIAN_POINT('Ctrl Pts',(6.86749846779438,-2.25589588159315,-12.));
#25939=CARTESIAN_POINT('Ctrl Pts',(6.9429142099725,-2.0748669644943,-12.));
#25940=CARTESIAN_POINT('Ctrl Pts',(7.01079261617851,-1.8911080179053,-12.));
#25941=CARTESIAN_POINT('Ctrl Pts',(7.07095894577038,-1.70508173509055,-12.));
#25942=CARTESIAN_POINT('Ctrl Pts',(7.08700753589636,-1.65546163052699,-12.));
#25943=CARTESIAN_POINT('Ctrl Pts',(7.10250722151628,-1.60568000149234,-12.));
#25944=CARTESIAN_POINT('Ctrl Pts',(7.11745423244714,-1.55574520184558,-12.));
#25945=CARTESIAN_POINT('Ctrl Pts',(7.17289725401069,-1.37052180257242,-12.));
#25946=CARTESIAN_POINT('Ctrl Pts',(7.22073965069804,-1.18319304603741,-12.));
#25947=CARTESIAN_POINT('Ctrl Pts',(7.26105716846878,-0.994238416058683,
-12.));
#25948=CARTESIAN_POINT('Ctrl Pts',(7.30180998831209,-0.803243671841799,
-12.));
#25949=CARTESIAN_POINT('Ctrl Pts',(7.33487473704459,-0.6105871243123,-12.));
#25950=CARTESIAN_POINT('Ctrl Pts',(7.36028116535095,-0.416741430078175,
-12.));
#25951=CARTESIAN_POINT('Ctrl Pts',(7.38577396141591,-0.222236768045678,
-12.));
#25952=CARTESIAN_POINT('Ctrl Pts',(7.40355641032544,-0.0265341668316033,
-12.));
#25953=CARTESIAN_POINT('Ctrl Pts',(7.41360781144787,0.169901389152281,-12.));
#25954=CARTESIAN_POINT('Ctrl Pts',(7.4166886322644,0.230110184185977,-12.));
#25955=CARTESIAN_POINT('Ctrl Pts',(7.41904278312292,0.29038788552009,-12.));
#25956=CARTESIAN_POINT('Ctrl Pts',(7.42066868798675,0.350721181107772,-12.));
#25957=CARTESIAN_POINT('Ctrl Pts',(7.4216482379621,0.387069850406059,-12.));
#25958=CARTESIAN_POINT('Ctrl Pts',(7.42236347434099,0.423440379102023,-12.));
#25959=CARTESIAN_POINT('Ctrl Pts',(7.42281390769938,0.459825068682672,-12.));
#25960=CARTESIAN_POINT('Ctrl Pts',(7.42316672971766,0.488324999634255,-12.));
#25961=CARTESIAN_POINT('Ctrl Pts',(7.42335696411711,0.51682607170187,-12.));
#25962=CARTESIAN_POINT('Ctrl Pts',(7.4233848049328,0.545317083559071,-12.));
#25963=CARTESIAN_POINT('Ctrl Pts',(7.42357977148935,0.744836901380488,-12.));
#25964=CARTESIAN_POINT('Ctrl Pts',(7.41581674804868,0.944011512545434,-12.));
#25965=CARTESIAN_POINT('Ctrl Pts',(7.40017828941996,1.14234330858621,-12.));
#25966=CARTESIAN_POINT('Ctrl Pts',(7.38439461942376,1.34251672035145,-12.));
#25967=CARTESIAN_POINT('Ctrl Pts',(7.3605887283379,1.54183228746579,-12.));
#25968=CARTESIAN_POINT('Ctrl Pts',(7.32879500122438,1.73979431536829,-12.));
#25969=CARTESIAN_POINT('Ctrl Pts',(7.30959003369515,1.85937307077222,-12.));
#25970=CARTESIAN_POINT('Ctrl Pts',(7.28746951960363,1.97845821396004,-12.));
#25971=CARTESIAN_POINT('Ctrl Pts',(7.2624318954249,2.09694161440503,-12.));
#25972=CARTESIAN_POINT('Ctrl Pts',(7.22127493906698,2.29170514733619,-12.));
#25973=CARTESIAN_POINT('Ctrl Pts',(7.17223845228515,2.48484324886949,-12.));
#25974=CARTESIAN_POINT('Ctrl Pts',(7.11556674531464,2.67596142272514,-12.));
#25975=CARTESIAN_POINT('Ctrl Pts',(7.05858971676105,2.86810925505617,-12.));
#25976=CARTESIAN_POINT('Ctrl Pts',(6.99389478787003,3.05821599278081,-12.));
#25977=CARTESIAN_POINT('Ctrl Pts',(6.92167928825846,3.24586879408122,-12.));
#25978=CARTESIAN_POINT('Ctrl Pts',(6.91269241961899,3.26922127497781,-12.));
#25979=CARTESIAN_POINT('Ctrl Pts',(6.90358902068414,3.29253573016435,-12.));
#25980=CARTESIAN_POINT('Ctrl Pts',(6.89436941920698,3.31581134317188,-12.));
#25981=CARTESIAN_POINT('Ctrl Pts',(6.88279319264489,3.3450364425663,-12.));
#25982=CARTESIAN_POINT('Ctrl Pts',(6.87103714791754,3.37419161400014,-12.));
#25983=CARTESIAN_POINT('Ctrl Pts',(6.85910773788451,3.40326238116243,-12.));
#25984=CARTESIAN_POINT('Ctrl Pts',(6.78106408142094,3.59344688813005,-12.));
#25985=CARTESIAN_POINT('Ctrl Pts',(6.69553789775985,3.78018911471325,-12.));
#25986=CARTESIAN_POINT('Ctrl Pts',(6.60286394971234,3.96308083941159,-12.));
#25987=CARTESIAN_POINT('Ctrl Pts',(6.51036026948687,4.14563654113595,-12.));
#25988=CARTESIAN_POINT('Ctrl Pts',(6.41073477459907,4.3243565276691,-12.));
#25989=CARTESIAN_POINT('Ctrl Pts',(6.3042667134665,4.49882949555396,-12.));
#25990=CARTESIAN_POINT('Ctrl Pts',(6.19750469508528,4.67378418155275,-12.));
#25991=CARTESIAN_POINT('Ctrl Pts',(6.08386202640003,4.84446903588274,-12.));
#25992=CARTESIAN_POINT('Ctrl Pts',(5.96357023683373,5.01045404774627,-12.));
#25993=CARTESIAN_POINT('Ctrl Pts',(5.84327844726742,5.1764390596098,-12.));
#25994=CARTESIAN_POINT('Ctrl Pts',(5.71633726955937,5.33772491039946,-12.));
#25995=CARTESIAN_POINT('Ctrl Pts',(5.58293216084948,5.49385617917443,-12.));
#25996=CARTESIAN_POINT('Ctrl Pts',(5.48072058003189,5.61347996233291,-12.));
#25997=CARTESIAN_POINT('Ctrl Pts',(5.37471348653155,5.730077391454,-12.));
#25998=CARTESIAN_POINT('Ctrl Pts',(5.26507849878159,5.84352819875606,-12.));
#25999=CARTESIAN_POINT('Ctrl Pts',(5.24734949409338,5.86187425721622,-12.));
#26000=CARTESIAN_POINT('Ctrl Pts',(5.22953248942995,5.88013086702314,-12.));
#26001=CARTESIAN_POINT('Ctrl Pts',(5.21162852093184,5.89829754282688,-12.));
#26002=CARTESIAN_POINT('Ctrl Pts',(5.06686638504291,6.04518379274567,-12.));
#26003=CARTESIAN_POINT('Ctrl Pts',(4.91642028337385,6.18619531935667,-12.));
#26004=CARTESIAN_POINT('Ctrl Pts',(4.7607493602725,6.32112569282487,-12.));
#26005=CARTESIAN_POINT('Ctrl Pts',(4.60343491120369,6.45748061988455,-12.));
#26006=CARTESIAN_POINT('Ctrl Pts',(4.44078428868537,6.58762579275016,-12.));
#26007=CARTESIAN_POINT('Ctrl Pts',(4.27322757175171,6.71131806402962,-12.));
#26008=CARTESIAN_POINT('Ctrl Pts',(4.19032886513755,6.77251483068203,-12.));
#26009=CARTESIAN_POINT('Ctrl Pts',(4.10622862770558,6.83213156416253,-12.));
#26010=CARTESIAN_POINT('Ctrl Pts',(4.0209755701235,6.89013557221799,-12.));
#26011=CARTESIAN_POINT('Ctrl Pts',(3.98093099022267,6.91738088401116,-12.));
#26012=CARTESIAN_POINT('Ctrl Pts',(3.94063203236017,6.94427034483953,-12.));
#26013=CARTESIAN_POINT('Ctrl Pts',(3.90008359516906,6.97080038552624,-12.));
#26014=CARTESIAN_POINT('Ctrl Pts',(3.87285102989615,6.98861811451265,-12.));
#26015=CARTESIAN_POINT('Ctrl Pts',(3.84550593396186,7.00627372305823,-12.));
#26016=CARTESIAN_POINT('Ctrl Pts',(3.81804976883042,7.0237660991706,-12.));
#26017=CARTESIAN_POINT('Ctrl Pts',(3.79110003457158,7.04093582719077,-12.));
#26018=CARTESIAN_POINT('Ctrl Pts',(3.76405158817414,7.05794299142264,-12.));
#26019=CARTESIAN_POINT('Ctrl Pts',(3.73690799396172,7.07478559879379,-12.));
#26020=CARTESIAN_POINT('Ctrl Pts',(3.55729426387553,7.18623596570672,-12.));
#26021=CARTESIAN_POINT('Ctrl Pts',(3.37348978795351,7.29050138644909,-12.));
#26022=CARTESIAN_POINT('Ctrl Pts',(3.18594346175011,7.38734226264639,-12.));
#26023=CARTESIAN_POINT('Ctrl Pts',(2.99823564615633,7.4842665250362,-12.));
#26024=CARTESIAN_POINT('Ctrl Pts',(2.80677898323789,7.57375390615019,-12.));
#26025=CARTESIAN_POINT('Ctrl Pts',(2.61198894494858,7.65552549589783,-12.));
#26026=CARTESIAN_POINT('Ctrl Pts',(2.53306554533635,7.68865702516523,-12.));
#26027=CARTESIAN_POINT('Ctrl Pts',(2.45359457631988,7.72052141836669,-12.));
#26028=CARTESIAN_POINT('Ctrl Pts',(2.37360237640535,7.75109805319065,-12.));
#26029=CARTESIAN_POINT('Ctrl Pts',(2.2838343803519,7.78541143921003,-12.));
#26030=CARTESIAN_POINT('Ctrl Pts',(2.19340997675606,7.81810312229487,-12.));
#26031=CARTESIAN_POINT('Ctrl Pts',(2.10237422929003,7.84917075545908,-12.));
#26032=CARTESIAN_POINT('Ctrl Pts',(-2.10221711401193,7.84912099186632,-11.9997040748415));
#26033=CARTESIAN_POINT('Ctrl Pts',(-3.40065621282619,7.50136219214109,-11.9470477325341));
#26034=CARTESIAN_POINT('Ctrl Pts',(-5.82037411761894,6.1495207846071,-11.8417350479192));
#26035=CARTESIAN_POINT('Ctrl Pts',(-8.04628560583682,2.63551264777254,-11.6837660209969));
#26036=CARTESIAN_POINT('Ctrl Pts',(-8.33052461663556,-1.51331821149076,
-11.5257969940746));
#26037=CARTESIAN_POINT('Ctrl Pts',(-6.60497458284972,-5.29754553073239,
-11.3678279671523));
#26038=CARTESIAN_POINT('Ctrl Pts',(-3.28573123451154,-7.80334276912094,
-11.20985894023));
#26039=CARTESIAN_POINT('Ctrl Pts',(0.826234788409155,-8.42652765391102,
-11.0518899133078));
#26040=CARTESIAN_POINT('Ctrl Pts',(4.7388724476258,-7.01653408891042,-10.8939208863855));
#26041=CARTESIAN_POINT('Ctrl Pts',(7.50812913234392,-3.91366458658699,-10.7359518594632));
#26042=CARTESIAN_POINT('Ctrl Pts',(8.46586977500607,0.133491868494349,-10.5779828325409));
#26043=CARTESIAN_POINT('Ctrl Pts',(7.38100727233018,4.14843049732635,-10.4200138056186));
#26044=CARTESIAN_POINT('Ctrl Pts',(4.51529588862971,7.16246272184166,-10.2620447786963));
#26045=CARTESIAN_POINT('Ctrl Pts',(0.560157043790593,8.44837130006937,-10.104075751774));
#26046=CARTESIAN_POINT('Ctrl Pts',(-3.53013313317451,7.69590287683787,-9.94610672485177));
#26047=CARTESIAN_POINT('Ctrl Pts',(-6.76869167449018,5.08660706304677,-9.78813769792948));
#26048=CARTESIAN_POINT('Ctrl Pts',(-8.37413600776358,1.25004196616275,-9.63016867100719));
#26049=CARTESIAN_POINT('Ctrl Pts',(-7.95911317970092,-2.88812681945649,
-9.4721996440849));
#26050=CARTESIAN_POINT('Ctrl Pts',(-5.62375762011129,-6.32946355950556,
-9.31423061716261));
#26051=CARTESIAN_POINT('Ctrl Pts',(-1.93153160038241,-8.2436608785505,-9.15626159024033));
#26052=CARTESIAN_POINT('Ctrl Pts',(2.22672414846207,-8.16887130657559,-8.99829256331803));
#26053=CARTESIAN_POINT('Ctrl Pts',(5.84772767608588,-6.12313971270086,-8.84032353639575));
#26054=CARTESIAN_POINT('Ctrl Pts',(8.05782242151238,-2.60004936964598,-8.68235450947345));
#26055=CARTESIAN_POINT('Ctrl Pts',(8.32376841870599,1.55036712102419,-8.52438548255116));
#26056=CARTESIAN_POINT('Ctrl Pts',(6.581399626523,5.32671923988587,-8.36641645562887));
#26057=CARTESIAN_POINT('Ctrl Pts',(3.25110556474056,7.81786873172712,-8.20844742870658));
#26058=CARTESIAN_POINT('Ctrl Pts',(-0.863598040844137,8.4227642330924,-8.05047840178429));
#26059=CARTESIAN_POINT('Ctrl Pts',(-4.76993728186221,6.99545975817784,-7.89250937486201));
#26060=CARTESIAN_POINT('Ctrl Pts',(-7.52541130072914,3.88032777692923,-7.7345403479397));
#26061=CARTESIAN_POINT('Ctrl Pts',(-8.46519390978181,-0.171029153471515,
-7.57657132101743));
#26062=CARTESIAN_POINT('Ctrl Pts',(-7.36253933495,-4.1811210748754,-7.41860229409512));
#26063=CARTESIAN_POINT('Ctrl Pts',(-4.48349023618117,-7.18241423224846,
-7.26063326717284));
#26064=CARTESIAN_POINT('Ctrl Pts',(-0.52268834243429,-8.45077249712525,
-7.10266424025055));
#26065=CARTESIAN_POINT('Ctrl Pts',(3.56422502820635,-7.68017310025088,-6.94469521332826));
#26066=CARTESIAN_POINT('Ctrl Pts',(6.79118104797183,-5.05654218564124,-6.78672618640598));
#26067=CARTESIAN_POINT('Ctrl Pts',(8.37959684732031,-1.21289553461213,-6.62875715948368));
#26068=CARTESIAN_POINT('Ctrl Pts',(7.94622786899591,2.92339213166767,-6.4707881325614));
#26069=CARTESIAN_POINT('Ctrl Pts',(5.59563508645045,6.35433921669177,-6.3128191056391));
#26070=CARTESIAN_POINT('Ctrl Pts',(1.89495708556707,8.25214496633223,-6.15485007871682));
#26071=CARTESIAN_POINT('Ctrl Pts',(-2.26292613171868,8.15891685359569,-5.99688105179451));
#26072=CARTESIAN_POINT('Ctrl Pts',(-5.87482250865055,6.09714846410646,-5.83891202487224));
#26073=CARTESIAN_POINT('Ctrl Pts',(-8.06927280363647,2.56429236281581,-5.68094299794993));
#26074=CARTESIAN_POINT('Ctrl Pts',(-8.31681166379602,-1.58726262806428,
-5.52297397102766));
#26075=CARTESIAN_POINT('Ctrl Pts',(-6.5577142230679,-5.35585129275224,-5.36500494410535));
#26076=CARTESIAN_POINT('Ctrl Pts',(-3.21640620179515,-7.83220850377189,
-5.20703591718308));
#26077=CARTESIAN_POINT('Ctrl Pts',(0.900939284774293,-8.41885189955573,
-5.04906689026078));
#26078=CARTESIAN_POINT('Ctrl Pts',(4.8009109090025,-6.97423926642352,-4.89109786333849));
#26079=CARTESIAN_POINT('Ctrl Pts',(7.54254415828974,-3.84691909477602,-4.7331288364162));
#26080=CARTESIAN_POINT('Ctrl Pts',(8.46435227254872,0.208565355949563,-4.57515980949391));
#26081=CARTESIAN_POINT('Ctrl Pts',(7.34392626871001,4.21372826143952,-4.41719078257162));
#26082=CARTESIAN_POINT('Ctrl Pts',(4.45159660304068,7.20222511348401,-4.25922175564932));
#26083=CARTESIAN_POINT('Ctrl Pts',(0.485209269400489,8.45300720846675,-4.10125272872704));
#26084=CARTESIAN_POINT('Ctrl Pts',(-3.59824678875397,7.66429246236889,-3.94328370180475));
#26085=CARTESIAN_POINT('Ctrl Pts',(-6.8135369057104,5.02637779479667,-3.78531467488246));
#26086=CARTESIAN_POINT('Ctrl Pts',(-8.3848928992151,1.17572529537953,-3.62734564796017));
#26087=CARTESIAN_POINT('Ctrl Pts',(-7.93318631167529,-2.95859998069199,
-3.46937662103788));
#26088=CARTESIAN_POINT('Ctrl Pts',(-5.56740251784145,-6.37908991203571,
-3.31140759411559));
#26089=CARTESIAN_POINT('Ctrl Pts',(-1.85834531040058,-8.26046679121798,
-3.1534385671933));
#26090=CARTESIAN_POINT('Ctrl Pts',(2.29908361810098,-8.14880196215876,-2.99546954027101));
#26091=CARTESIAN_POINT('Ctrl Pts',(5.90180181930062,-6.07103732381897,-2.83750051334872));
#26092=CARTESIAN_POINT('Ctrl Pts',(8.08056451327072,-2.52848493141107,-2.67953148642643));
#26093=CARTESIAN_POINT('Ctrl Pts',(8.30969136847607,1.62412692305045,-2.52156245950414));
#26094=CARTESIAN_POINT('Ctrl Pts',(6.53389986996386,5.38487802933261,-2.36359343258185));
#26095=CARTESIAN_POINT('Ctrl Pts',(3.1816435919847,7.84639426457055,-2.20562440565956));
#26096=CARTESIAN_POINT('Ctrl Pts',(-0.938262812779821,8.4147740192864,-2.04765537873727));
#26097=CARTESIAN_POINT('Ctrl Pts',(-4.83179013190352,6.95288163445507,-1.88968635181498));
#26098=CARTESIAN_POINT('Ctrl Pts',(-7.55952870061531,3.81343476751294,-1.73171732489269));
#26099=CARTESIAN_POINT('Ctrl Pts',(-8.46334419381849,-0.246097457243576,
-1.5737482979704));
#26100=CARTESIAN_POINT('Ctrl Pts',(-7.32516879282469,-4.24625259000572,
-1.41577927104811));
#26101=CARTESIAN_POINT('Ctrl Pts',(-4.41961543450651,-7.22189437146341,
-1.25781024412582));
#26102=CARTESIAN_POINT('Ctrl Pts',(-0.447720655298665,-8.45507570139511,
-1.09984121720353));
#26103=CARTESIAN_POINT('Ctrl Pts',(3.6321977940243,-7.64826111522011,-0.941872190281239));
#26104=CARTESIAN_POINT('Ctrl Pts',(6.83575878328587,-4.99611456616368,-0.78390316335895));
#26105=CARTESIAN_POINT('Ctrl Pts',(8.39002407208524,-1.1385319368965,-0.625934136436659));
#26106=CARTESIAN_POINT('Ctrl Pts',(7.91998875760714,2.99374965233894,-0.46796510951437));
#26107=CARTESIAN_POINT('Ctrl Pts',(5.53906047283149,6.4037151701039,-0.309996082592078));
#26108=CARTESIAN_POINT('Ctrl Pts',(1.82169699306643,8.26862618377173,-0.152027055669789));
#26109=CARTESIAN_POINT('Ctrl Pts',(-2.33519589571696,8.13852683414694,0.00594197125250266));
#26110=CARTESIAN_POINT('Ctrl Pts',(-5.92866507798216,6.0448068037463,0.163910998174792));
#26111=CARTESIAN_POINT('Ctrl Pts',(-8.09169732813897,2.49262778033376,0.321880025097081));
#26112=CARTESIAN_POINT('Ctrl Pts',(-8.30240767288088,-1.66095928149717,
0.479849052019373));
#26113=CARTESIAN_POINT('Ctrl Pts',(-6.50995703542896,-5.41379887864077,
0.637818078941659));
#26114=CARTESIAN_POINT('Ctrl Pts',(-3.1468184189074,-7.86042573528484,0.795787105863953));
#26115=CARTESIAN_POINT('Ctrl Pts',(0.975567890954294,-8.4105306724155,0.953756132786241));
#26116=CARTESIAN_POINT('Ctrl Pts',(4.86257434335317,-6.93138728227376,1.11172515970853));
#26117=CARTESIAN_POINT('Ctrl Pts',(7.57636459372931,-3.77987545355504,1.26969418663082));
#26118=CARTESIAN_POINT('Ctrl Pts',(8.46216969341154,0.28362471932149,1.42766321355311));
#26119=CARTESIAN_POINT('Ctrl Pts',(7.30626727613884,4.27869342102536,1.5856322404754));
#26120=CARTESIAN_POINT('Ctrl Pts',(4.38754735945002,7.2414216194119,1.74360126739769));
#26121=CARTESIAN_POINT('Ctrl Pts',(0.410223237298467,8.45697793523688,1.90157029431998));
#26122=CARTESIAN_POINT('Ctrl Pts',(-3.66607737641103,7.63207937404152,2.05953932124227));
#26123=CARTESIAN_POINT('Ctrl Pts',(-6.85784624373112,4.96575309483324,2.21750834816456));
#26124=CARTESIAN_POINT('Ctrl Pts',(-8.39499026503231,1.10131619052641,2.37547737508686));
#26125=CARTESIAN_POINT('Ctrl Pts',(-7.90663546630572,-3.02884045543163,
2.53344640200914));
#26126=CARTESIAN_POINT('Ctrl Pts',(-5.51060950873351,-6.42821450666971,
2.69141542893143));
#26127=CARTESIAN_POINT('Ctrl Pts',(-1.78501285421056,-8.27662298354866,
2.84938445585372));
#26128=CARTESIAN_POINT('Ctrl Pts',(2.37126225446112,-8.12809167160846,3.00735348277601));
#26129=CARTESIAN_POINT('Ctrl Pts',(5.9554117564608,-6.01845741968086,3.1653225096983));
#26130=CARTESIAN_POINT('Ctrl Pts',(8.10267102932754,-2.45672161467252,3.32329153662059));
#26131=CARTESIAN_POINT('Ctrl Pts',(8.29496072023576,1.69775897913956,3.48126056354288));
#26132=CARTESIAN_POINT('Ctrl Pts',(6.48588619027077,5.4426132719823,3.63922959046517));
#26133=CARTESIAN_POINT('Ctrl Pts',(3.11193136735919,7.87430264000241,3.79719861738746));
#26134=CARTESIAN_POINT('Ctrl Pts',(-1.01285378573731,8.40612194238345,3.95516764430975));
#26135=CARTESIAN_POINT('Ctrl Pts',(-4.89326293801619,6.9097566325407,4.11313667123204));
#26136=CARTESIAN_POINT('Ctrl Pts',(-7.59305150657372,3.74624181280671,4.27110569815433));
#26137=CARTESIAN_POINT('Ctrl Pts',(-8.46082879442303,-0.321146404253918,
4.42907472507662));
#26138=CARTESIAN_POINT('Ctrl Pts',(-7.2872220903285,-4.31105011658773,4.58704375199891));
#26139=CARTESIAN_POINT('Ctrl Pts',(-4.35539300845213,-7.26080647334918,
4.7450127789212));
#26140=CARTESIAN_POINT('Ctrl Pts',(-0.37271775274243,-8.45871387258687,
4.90298180584349));
#26141=CARTESIAN_POINT('Ctrl Pts',(3.69988486971213,-7.61574755702801,5.06095083276578));
#26142=CARTESIAN_POINT('Ctrl Pts',(6.87979885272231,-4.93529397782784,5.21891985968807));
#26143=CARTESIAN_POINT('Ctrl Pts',(8.39979138040202,-1.06407878807301,5.37688888661037));
#26144=CARTESIAN_POINT('Ctrl Pts',(7.8931267003478,3.06387169995084,5.53485791353265));
#26145=CARTESIAN_POINT('Ctrl Pts',(5.4820501850021,6.45258743998261,5.69282694045494));
#26146=CARTESIAN_POINT('Ctrl Pts',(1.74829361518324,8.28445703330112,5.85079596737723));
#26147=CARTESIAN_POINT('Ctrl Pts',(-2.40728198513118,8.11749667973851,6.00876499429952));
#26148=CARTESIAN_POINT('Ctrl Pts',(-5.98204132879465,5.99198968975211,6.1667340212218));
#26149=CARTESIAN_POINT('Ctrl Pts',(-8.11348540105156,2.42076714047972,6.32470304814411));
#26150=CARTESIAN_POINT('Ctrl Pts',(-8.28735065697621,-1.73452529235496,
6.48267207506639));
#26151=CARTESIAN_POINT('Ctrl Pts',(-6.46168780781411,-5.47132064275613,
6.64064110198868));
#26152=CARTESIAN_POINT('Ctrl Pts',(-3.07698312335276,-7.88802470585037,
6.79861012891098));
#26153=CARTESIAN_POINT('Ctrl Pts',(1.0501197639459,-8.40154791588267,6.95657915583325));
#26154=CARTESIAN_POINT('Ctrl Pts',(4.9238553124377,-6.88799011059706,7.11454818275556));
#26155=CARTESIAN_POINT('Ctrl Pts',(7.60958911102027,-3.71253450663348,7.27251720967785));
#26156=CARTESIAN_POINT('Ctrl Pts',(8.45932152322004,0.358661774221112,7.43048623660013));
#26157=CARTESIAN_POINT('Ctrl Pts',(7.2680336098949,4.34332204043724,7.58845526352242));
#26158=CARTESIAN_POINT('Ctrl Pts',(4.32315301378977,7.28004855209397,7.74642429044472));
#26159=CARTESIAN_POINT('Ctrl Pts',(0.335204939132236,8.46028347931194,7.90439331736699));
#26160=CARTESIAN_POINT('Ctrl Pts',(-3.73361960914439,7.59926598532158,8.0623623442893));
#26161=CARTESIAN_POINT('Ctrl Pts',(-6.9016161785849,4.90473781409765,8.22033137121157));
#26162=CARTESIAN_POINT('Ctrl Pts',(-8.40442732379069,1.02682046175124,8.37830039813387));
#26163=CARTESIAN_POINT('Ctrl Pts',(-7.87946272535832,-3.0988426970199,8.53626942505616));
#26164=CARTESIAN_POINT('Ctrl Pts',(-5.45338306324019,-6.47683349083296,
8.69423845197845));
#26165=CARTESIAN_POINT('Ctrl Pts',(-1.71153999799109,-8.29212817887424,
8.85220747890073));
#26166=CARTESIAN_POINT('Ctrl Pts',(2.44325437937582,-8.10674206708394,9.01017650582304));
#26167=CARTESIAN_POINT('Ctrl Pts',(6.00855327147267,-5.96540413401097,9.16814553274532));
#26168=CARTESIAN_POINT('Ctrl Pts',(8.12414023041075,-2.38476506554547,9.32611455966761));
#26169=CARTESIAN_POINT('Ctrl Pts',(8.2795776332277,1.77125749970778,9.48408358658991));
#26170=CARTESIAN_POINT('Ctrl Pts',(6.43736236295422,5.49992042349329,9.64205261351219));
#26171=CARTESIAN_POINT('Ctrl Pts',(3.04197437592444,7.90159166877402,9.80002164043448));
#26172=CARTESIAN_POINT('Ctrl Pts',(-1.08736509632437,8.39680867164209,9.95799066735678));
#26173=CARTESIAN_POINT('Ctrl Pts',(-4.95435085818707,6.86608816623656,10.1159596942791));
#26174=CARTESIAN_POINT('Ctrl Pts',(-7.62597709521529,3.67875415554537,10.2739287212014));
#26175=CARTESIAN_POINT('Ctrl Pts',(-8.45764788353322,-0.396170009359619,
10.4318977481237));
#26176=CARTESIAN_POINT('Ctrl Pts',(-7.24870226247802,-4.37550871757833,
10.589866775046));
#26177=CARTESIAN_POINT('Ctrl Pts',(-4.29082791168611,-7.29914716729561,
10.7478358019683));
#26178=CARTESIAN_POINT('Ctrl Pts',(-0.297685723949315,-8.46168732661545,
10.9058048288906));
#26179=CARTESIAN_POINT('Ctrl Pts',(3.76728130007181,-7.58263381362094,11.0637738558128));
#26180=CARTESIAN_POINT('Ctrl Pts',(6.92329707614913,-4.87408747579489,11.2217428827352));
#26181=CARTESIAN_POINT('Ctrl Pts',(8.40889939502786,-0.989537532666886,
11.3797119096574));
#26182=CARTESIAN_POINT('Ctrl Pts',(7.86564110829628,3.13374419045154,11.5376809365797));
#26183=CARTESIAN_POINT('Ctrl Pts',(5.42461395487494,6.50096882535833,11.695649963502));
#26184=CARTESIAN_POINT('Ctrl Pts',(1.67474253093863,8.29960394072526,11.8536189904243));
#26185=CARTESIAN_POINT('Ctrl Pts',(-2.4791589111201,8.09589087029261,12.0115880173466));
#26186=CARTESIAN_POINT('Ctrl Pts',(-6.03498574071721,5.93857891308519,12.1695570442689));
#26187=CARTESIAN_POINT('Ctrl Pts',(-8.1345583276468,2.34895716891092,12.3275260711912));
#26188=CARTESIAN_POINT('Ctrl Pts',(-8.27181774175635,-1.80868950910794,
12.4855039120797));
#26189=CARTESIAN_POINT('Ctrl Pts',(-7.03199329881568,-4.28796079991923,
12.5908254106607));
#26190=CARTESIAN_POINT('Ctrl Pts',(-6.15407324826529,-5.30616618526941,
12.6434905669344));
#26191=CARTESIAN_POINT('Ctrl Pts',(-2.00604317752182,7.49003302766729,-12.214330565978));
#26192=CARTESIAN_POINT('Ctrl Pts',(-3.24508022951926,7.15818378005051,-12.1616742236706));
#26193=CARTESIAN_POINT('Ctrl Pts',(-5.55409891368994,5.86818751153965,-12.0563615390557));
#26194=CARTESIAN_POINT('Ctrl Pts',(-7.67817759469036,2.51494107392495,-11.8983925121334));
#26195=CARTESIAN_POINT('Ctrl Pts',(-7.94941300829144,-1.44408570044746,
-11.7404234852111));
#26196=CARTESIAN_POINT('Ctrl Pts',(-6.30280483938424,-5.05518911377136,
-11.5824544582888));
#26197=CARTESIAN_POINT('Ctrl Pts',(-3.13541293248401,-7.44634910424883,
-11.4244854313665));
#26198=CARTESIAN_POINT('Ctrl Pts',(0.78843552802984,-8.04102402061944,-11.2665164044443));
#26199=CARTESIAN_POINT('Ctrl Pts',(4.52207466076785,-6.69553598678779,-11.108547377522));
#26200=CARTESIAN_POINT('Ctrl Pts',(7.16464114077509,-3.73461907940069,-10.9505783505997));
#26201=CARTESIAN_POINT('Ctrl Pts',(8.07856628639489,0.12738477403824,-10.7926093236774));
#26202=CARTESIAN_POINT('Ctrl Pts',(7.04333495489414,3.95864472851865,-10.6346402967551));
#26203=CARTESIAN_POINT('Ctrl Pts',(4.30872646383876,6.83478855805914,-10.4766712698328));
#26204=CARTESIAN_POINT('Ctrl Pts',(0.534530524248469,8.06186834590634,-10.3187022429105));
#26205=CARTESIAN_POINT('Ctrl Pts',(-3.36863373452123,7.34382445944808,-10.1607332159882));
#26206=CARTESIAN_POINT('Ctrl Pts',(-6.45903206850345,4.85390083048357,-10.0027641890659));
#26207=CARTESIAN_POINT('Ctrl Pts',(-7.99102923006582,1.19285403069102,-9.84479516214361));
#26208=CARTESIAN_POINT('Ctrl Pts',(-7.59499320352905,-2.75599844724488,
-9.68682613522134));
#26209=CARTESIAN_POINT('Ctrl Pts',(-5.36647738745246,-6.0398981181765,-9.52885710829904));
#26210=CARTESIAN_POINT('Ctrl Pts',(-1.84316632344425,-7.86652318306926,
-9.37088808137676));
#26211=CARTESIAN_POINT('Ctrl Pts',(2.12485416300348,-7.79515514519626,-9.21291905445446));
#26212=CARTESIAN_POINT('Ctrl Pts',(5.5802010793406,-5.84301334234443,-9.05495002753217));
#26213=CARTESIAN_POINT('Ctrl Pts',(7.68918661474923,-2.48110019865847,-8.89698100060988));
#26214=CARTESIAN_POINT('Ctrl Pts',(7.9429658983939,1.47943966636695,-8.73901197368759));
#26215=CARTESIAN_POINT('Ctrl Pts',(6.28030840931315,5.08302816037614,-8.5810429467653));
#26216=CARTESIAN_POINT('Ctrl Pts',(3.10237134598554,7.46021052131602,-8.42307391984302));
#26217=CARTESIAN_POINT('Ctrl Pts',(-0.824089456036443,8.03743277183402,
-8.26510489292072));
#26218=CARTESIAN_POINT('Ctrl Pts',(-4.55171831572882,6.67542578165953,-8.10713586599843));
#26219=CARTESIAN_POINT('Ctrl Pts',(-7.18113267048003,3.70280738919583,-7.94916683907614));
#26220=CARTESIAN_POINT('Ctrl Pts',(-8.07792134120202,-0.163204772804889,
-7.79119781215386));
#26221=CARTESIAN_POINT('Ctrl Pts',(-7.0257119037176,-3.98983975096633,-7.63322878523156));
#26222=CARTESIAN_POINT('Ctrl Pts',(-4.27837588221913,-6.85382731055814,
-7.47525975830927));
#26223=CARTESIAN_POINT('Ctrl Pts',(-0.498775971483477,-8.06415969104843,
-7.31729073138698));
#26224=CARTESIAN_POINT('Ctrl Pts',(3.401165965841,-7.32881430146016,-7.15932170446469));
#26225=CARTESIAN_POINT('Ctrl Pts',(6.48049257985542,-4.82521138551596,-7.0013526775424));
#26226=CARTESIAN_POINT('Ctrl Pts',(7.99624024269784,-1.15740700427081,-6.84338365062012));
#26227=CARTESIAN_POINT('Ctrl Pts',(7.5826973804869,2.78965041330152,-6.68541462369781));
#26228=CARTESIAN_POINT('Ctrl Pts',(5.33964142630988,6.0636357435874,-6.52744559677554));
#26229=CARTESIAN_POINT('Ctrl Pts',(1.80826504924783,7.8746191339102,-6.36947656985323));
#26230=CARTESIAN_POINT('Ctrl Pts',(-2.15939994851756,7.78565609661882,-6.21150754293096));
#26231=CARTESIAN_POINT('Ctrl Pts',(-5.60605635549174,5.81821116250748,-6.05353851600865));
#26232=CARTESIAN_POINT('Ctrl Pts',(-7.70011315548899,2.44697903242775,-5.89556948908638));
#26233=CARTESIAN_POINT('Ctrl Pts',(-7.93632740675959,-1.51464724777502,
-5.73760046216408));
#26234=CARTESIAN_POINT('Ctrl Pts',(-6.25770658493865,-5.11082745641947,
-5.57963143524179));
#26235=CARTESIAN_POINT('Ctrl Pts',(-3.06925943768785,-7.47389426581884,
-5.4216624083195));
#26236=CARTESIAN_POINT('Ctrl Pts',(0.859722382401179,-8.0336994229106,-5.26369338139721));
#26237=CARTESIAN_POINT('Ctrl Pts',(4.58127493621,-6.65517610220269,-5.10572435447492));
#26238=CARTESIAN_POINT('Ctrl Pts',(7.19748172015326,-3.67092711457684,-4.94775532755263));
#26239=CARTESIAN_POINT('Ctrl Pts',(8.07711820787286,0.199023738595472,-4.78978630063034));
#26240=CARTESIAN_POINT('Ctrl Pts',(7.00795036315426,4.02095519746761,-4.63181727370805));
#26241=CARTESIAN_POINT('Ctrl Pts',(4.24794134491971,6.87273186750345,-4.47384824678576));
#26242=CARTESIAN_POINT('Ctrl Pts',(0.463011521532918,8.06629216699988,-4.31587921986347));
#26243=CARTESIAN_POINT('Ctrl Pts',(-3.43363127124591,7.31366018390231,-4.15791019294118));
#26244=CARTESIAN_POINT('Ctrl Pts',(-6.50182568365104,4.79642697973099,-3.99994116601889));
#26245=CARTESIAN_POINT('Ctrl Pts',(-8.00129400650773,1.12193725934179,-3.8419721390966));
#26246=CARTESIAN_POINT('Ctrl Pts',(-7.57025245892629,-2.82324754504386,
-3.68400311217431));
#26247=CARTESIAN_POINT('Ctrl Pts',(-5.31270046418729,-6.08725412401191,
-3.52603408525202));
#26248=CARTESIAN_POINT('Ctrl Pts',(-1.77332821931713,-7.88256024518995,
-3.36806505832973));
#26249=CARTESIAN_POINT('Ctrl Pts',(2.19390327283648,-7.77600394945329,-3.21009603140744));
#26250=CARTESIAN_POINT('Ctrl Pts',(5.6318013947187,-5.79329457587998,-3.05212700448515));
#26251=CARTESIAN_POINT('Ctrl Pts',(7.71088828281686,-2.41280974848687,-2.89415797756286));
#26252=CARTESIAN_POINT('Ctrl Pts',(7.92953285649486,1.54982504504355,-2.73618895064057));
#26253=CARTESIAN_POINT('Ctrl Pts',(6.23498171020852,5.13852625427182,-2.57821992371828));
#26254=CARTESIAN_POINT('Ctrl Pts',(3.0360871759941,7.48743104490719,-2.42025089679599));
#26255=CARTESIAN_POINT('Ctrl Pts',(-0.895338403323793,8.02980810082093,
-2.2622818698737));
#26256=CARTESIAN_POINT('Ctrl Pts',(-4.61074147133374,6.63479555653366,-2.10431284295141));
#26257=CARTESIAN_POINT('Ctrl Pts',(-7.21368923983733,3.63897465552193,-1.94634381602912));
#26258=CARTESIAN_POINT('Ctrl Pts',(-8.0761562475474,-0.234838790826315,
-1.78837478910683));
#26259=CARTESIAN_POINT('Ctrl Pts',(-6.99005101951537,-4.05199157662599,
-1.63040576218454));
#26260=CARTESIAN_POINT('Ctrl Pts',(-4.21742327686693,-6.8915012802884,-1.47243673526225));
#26261=CARTESIAN_POINT('Ctrl Pts',(-0.42723796700686,-8.06826602883319,
-1.31446770833996));
#26262=CARTESIAN_POINT('Ctrl Pts',(3.46602905834345,-7.29836225184764,-1.15649868141767));
#26263=CARTESIAN_POINT('Ctrl Pts',(6.52303093671688,-4.76754825786905,-0.998529654495381));
#26264=CARTESIAN_POINT('Ctrl Pts',(8.00619043431256,-1.08644545284059,-0.840560627573093));
#26265=CARTESIAN_POINT('Ctrl Pts',(7.55765867728407,2.85678916095475,-0.682591600650801));
#26266=CARTESIAN_POINT('Ctrl Pts',(5.28565503407912,6.11075280576706,-0.524622573728512));
#26267=CARTESIAN_POINT('Ctrl Pts',(1.7383565189795,7.89034635522403,-0.366653546806221));
#26268=CARTESIAN_POINT('Ctrl Pts',(-2.22836345663647,7.76619889634581,-0.20868451988393));
#26269=CARTESIAN_POINT('Ctrl Pts',(-5.65743569121687,5.76826407095074,-0.0507154929616409));
#26270=CARTESIAN_POINT('Ctrl Pts',(-7.7215117846256,2.37859301948939,0.107253533960649));
#26271=CARTESIAN_POINT('Ctrl Pts',(-7.92258238132345,-1.58497236683139,
0.265222560882939));
#26272=CARTESIAN_POINT('Ctrl Pts',(-6.21213423192041,-5.16612400906892,
0.423191587805229));
#26273=CARTESIAN_POINT('Ctrl Pts',(-3.00285521322863,-7.50082059249928,
0.581160614727519));
#26274=CARTESIAN_POINT('Ctrl Pts',(0.930936818473215,-8.0257588820302,0.739129641649809));
#26275=CARTESIAN_POINT('Ctrl Pts',(4.64011734166718,-6.61428454543915,0.897098668572098));
#26276=CARTESIAN_POINT('Ctrl Pts',(7.22975491083474,-3.60695064032443,1.05506769549439));
#26277=CARTESIAN_POINT('Ctrl Pts',(8.0750354791393,0.270649225229449,1.21303672241668));
#26278=CARTESIAN_POINT('Ctrl Pts',(6.97201422477151,4.08294827815141,1.37100574933897));
#26279=CARTESIAN_POINT('Ctrl Pts',(4.18682227816202,6.91013517983273,1.52897477626126));
#26280=CARTESIAN_POINT('Ctrl Pts',(0.391456011350326,8.07008123773568,1.68694380318355));
#26281=CARTESIAN_POINT('Ctrl Pts',(-3.4983586900695,7.28292080611145,1.84491283010584));
#26282=CARTESIAN_POINT('Ctrl Pts',(-6.54410792207659,4.73857578779637,2.00288185702813));
#26283=CARTESIAN_POINT('Ctrl Pts',(-8.01092942982988,1.05093228267159,2.16085088395042));
#26284=CARTESIAN_POINT('Ctrl Pts',(-7.54491628320208,-2.89027460147783,
2.31881991087271));
#26285=CARTESIAN_POINT('Ctrl Pts',(-5.25850566780182,-6.13413132677903,
2.476788937795));
#26286=CARTESIAN_POINT('Ctrl Pts',(-1.70335063591225,-7.89797731090771,
2.63475796471729));
#26287=CARTESIAN_POINT('Ctrl Pts',(2.26277982229849,-7.75624113010126,2.79272699163958));
#26288=CARTESIAN_POINT('Ctrl Pts',(5.68295874091796,-5.74312013991523,2.95069601856187));
#26289=CARTESIAN_POINT('Ctrl Pts',(7.73198345201655,-2.34432951826698,3.10866504548416));
#26290=CARTESIAN_POINT('Ctrl Pts',(7.91547611791824,1.62008852200791,3.26663407240645));
#26291=CARTESIAN_POINT('Ctrl Pts',(6.18916459934302,5.19362017813345,3.42460309932874));
#26292=CARTESIAN_POINT('Ctrl Pts',(2.96956420285885,7.51406264530547,3.58257212625103));
#26293=CARTESIAN_POINT('Ctrl Pts',(-0.966516927848558,8.02155184616155,
3.74054115317332));
#26294=CARTESIAN_POINT('Ctrl Pts',(-4.66940196956842,6.59364347224404,3.89851018009561));
#26295=CARTESIAN_POINT('Ctrl Pts',(-7.24567841723297,3.57485569869889,4.05647920701789));
#26296=CARTESIAN_POINT('Ctrl Pts',(-8.07375592468714,-0.306454337634883,
4.21444823394019));
#26297=CARTESIAN_POINT('Ctrl Pts',(-6.95384033359499,-4.11382469331681,
4.37241726086248));
#26298=CARTESIAN_POINT('Ctrl Pts',(-4.15613895053757,-6.92863319972275,
4.53038628778477));
#26299=CARTESIAN_POINT('Ctrl Pts',(-0.355666358173307,-8.07173775801342,
4.68835531470706));
#26300=CARTESIAN_POINT('Ctrl Pts',(3.53061953069998,-7.26733615033155,4.84632434162935));
#26301=CARTESIAN_POINT('Ctrl Pts',(6.56505622527614,-4.70951013922241,5.00429336855164));
#26302=CARTESIAN_POINT('Ctrl Pts',(8.01551089987296,-1.01539844715936,5.16226239547394));
#26303=CARTESIAN_POINT('Ctrl Pts',(7.53202552724446,2.92370320816144,5.32023142239622));
#26304=CARTESIAN_POINT('Ctrl Pts',(5.23125289921567,6.15738922733681,5.47820044931851));
#26305=CARTESIAN_POINT('Ctrl Pts',(1.66831125846471,7.90545296218727,5.6361694762408));
#26306=CARTESIAN_POINT('Ctrl Pts',(-2.29715169306541,7.74613084652733,5.79413850316309));
#26307=CARTESIAN_POINT('Ctrl Pts',(-5.70837004194135,5.71786327719911,5.95210753008538));
#26308=CARTESIAN_POINT('Ctrl Pts',(-7.74230307907673,2.31001991857098,6.11007655700767));
#26309=CARTESIAN_POINT('Ctrl Pts',(-7.90821420601554,-1.65517282005532,
6.26804558392996));
#26310=CARTESIAN_POINT('Ctrl Pts',(-6.1660732641471,-5.22101422078565,6.42601461085225));
#26311=CARTESIAN_POINT('Ctrl Pts',(-2.93621479951312,-7.52715694293644,
6.58398363777455));
#26312=CARTESIAN_POINT('Ctrl Pts',(1.00207803180911,-8.01718707594133,6.74195266469683));
#26313=CARTESIAN_POINT('Ctrl Pts',(4.69859477918996,-6.5728727428306,6.89992169161912));
#26314=CARTESIAN_POINT('Ctrl Pts',(7.26145944591522,-3.54269046175417,7.05789071854142));
#26315=CARTESIAN_POINT('Ctrl Pts',(8.07231760935175,0.342253423977237,7.2158597454637));
#26316=CARTESIAN_POINT('Ctrl Pts',(6.93552970335405,4.14462021497455,7.373828772386));
#26317=CARTESIAN_POINT('Ctrl Pts',(4.12537389734458,6.94699497621579,7.53179779930828));
#26318=CARTESIAN_POINT('Ctrl Pts',(0.319869711237644,8.07323555709481,7.68976682623056));
#26319=CARTESIAN_POINT('Ctrl Pts',(-3.56281094586469,7.25160859095806,7.84773585315286));
#26320=CARTESIAN_POINT('Ctrl Pts',(-6.58587543438956,4.68035188369609,8.00570488007515));
#26321=CARTESIAN_POINT('Ctrl Pts',(-8.01993475435698,0.979844645020895,
8.16367390699745));
#26322=CARTESIAN_POINT('Ctrl Pts',(-7.51898666288417,-2.9570743236442,8.32164293391973));
#26323=CARTESIAN_POINT('Ctrl Pts',(-5.20389726423089,-6.18052605015402,
8.47961196084203));
#26324=CARTESIAN_POINT('Ctrl Pts',(-1.63323907561256,-7.91277316196025,
8.6375809877643));
#26325=CARTESIAN_POINT('Ctrl Pts',(2.33147839299217,-7.73586824463014,8.79555001468662));
#26326=CARTESIAN_POINT('Ctrl Pts',(5.73366909472596,-5.6924939790616,8.95351904160888));
#26327=CARTESIAN_POINT('Ctrl Pts',(7.75247046264582,-2.27566489581091,9.1114880685312));
#26328=CARTESIAN_POINT('Ctrl Pts',(7.90079678887271,1.69022457254288,9.26945709545346));
#26329=CARTESIAN_POINT('Ctrl Pts',(6.142860679502,5.24830559551758,9.42742612237578));
#26330=CARTESIAN_POINT('Ctrl Pts',(2.90280766070521,7.54010323341772,9.58539514929804));
#26331=CARTESIAN_POINT('Ctrl Pts',(-1.03761943446175,8.01266464649669,9.74336417622037));
#26332=CARTESIAN_POINT('Ctrl Pts',(-4.7276951899361,6.55197278641507,9.90133320314262));
#26333=CARTESIAN_POINT('Ctrl Pts',(-7.27709769929478,3.51045552161269,10.0593022300649));
#26334=CARTESIAN_POINT('Ctrl Pts',(-8.07072053669306,-0.378045701900852,
10.2172712569872));
#26335=CARTESIAN_POINT('Ctrl Pts',(-6.91708274212466,-4.17533438985954,
10.3752402839095));
#26336=CARTESIAN_POINT('Ctrl Pts',(-4.09452763027467,-6.9652198524524,10.5332093108318));
#26337=CARTESIAN_POINT('Ctrl Pts',(-0.284066955593615,-8.0745751800513,
10.6911783377541));
#26338=CARTESIAN_POINT('Ctrl Pts',(3.59493265440695,-7.23573732136131,10.8491473646764));
#26339=CARTESIAN_POINT('Ctrl Pts',(6.60656445663723,-4.65110376197204,11.0071163915987));
#26340=CARTESIAN_POINT('Ctrl Pts',(8.02420223364584,-0.944267365667029,
11.1650854185209));
#26341=CARTESIAN_POINT('Ctrl Pts',(7.50579736838894,2.99037911519842,11.3230544454432));
#26342=CARTESIAN_POINT('Ctrl Pts',(5.17644430840876,6.20355722178662,11.4810234723655));
#26343=CARTESIAN_POINT('Ctrl Pts',(1.59812504897912,7.91990691658437,11.6389924992878));
#26344=CARTESIAN_POINT('Ctrl Pts',(-2.36574033504738,7.72551347720574,11.7969615262101));
#26345=CARTESIAN_POINT('Ctrl Pts',(-5.75889230989227,5.66689598013705,11.9549305531324));
#26346=CARTESIAN_POINT('Ctrl Pts',(-7.76241194430529,2.24149516792393,12.1128995800547));
#26347=CARTESIAN_POINT('Ctrl Pts',(-7.89339190322096,-1.72594411196516,
12.2708774209432));
#26348=CARTESIAN_POINT('Ctrl Pts',(-6.71028795619838,-4.09179168546631,
12.3761989195243));
#26349=CARTESIAN_POINT('Ctrl Pts',(-5.87253170539172,-5.06341538360071,
12.428864075798));
#26350=CARTESIAN_POINT('Ctrl Pts',(-1.90986924103173,7.13094506346825,-12.4289570571144));
#26351=CARTESIAN_POINT('Ctrl Pts',(-3.08950424621235,6.81500536795992,-12.3763007148069));
#26352=CARTESIAN_POINT('Ctrl Pts',(-5.28782370976095,5.58685423847219,-12.2709880301921));
#26353=CARTESIAN_POINT('Ctrl Pts',(-7.31006958354388,2.39436950007738,-12.1130190032698));
#26354=CARTESIAN_POINT('Ctrl Pts',(-7.56830139994735,-1.37485318940416,
-11.9550499763475));
#26355=CARTESIAN_POINT('Ctrl Pts',(-6.00063509591875,-4.81283269681031,
-11.7970809494252));
#26356=CARTESIAN_POINT('Ctrl Pts',(-2.98509463045649,-7.08935543937673,
-11.6391119225029));
#26357=CARTESIAN_POINT('Ctrl Pts',(0.750636267650531,-7.65552038732784,
-11.4811428955806));
#26358=CARTESIAN_POINT('Ctrl Pts',(4.30527687390991,-6.37453788466516,-11.3231738686583));
#26359=CARTESIAN_POINT('Ctrl Pts',(6.82115314920626,-3.55557357221439,-11.1652048417361));
#26360=CARTESIAN_POINT('Ctrl Pts',(7.69126279778371,0.121277679582131,-11.0072358148138));
#26361=CARTESIAN_POINT('Ctrl Pts',(6.70566263745811,3.76885895971093,-10.8492667878915));
#26362=CARTESIAN_POINT('Ctrl Pts',(4.10215703904782,6.50711439427663,-10.6912977609692));
#26363=CARTESIAN_POINT('Ctrl Pts',(0.508904004706356,7.67536539174329,-10.5333287340469));
#26364=CARTESIAN_POINT('Ctrl Pts',(-3.20713433586796,6.9917460420583,-10.3753597071246));
#26365=CARTESIAN_POINT('Ctrl Pts',(-6.14937246251668,4.62119459792037,-10.2173906802023));
#26366=CARTESIAN_POINT('Ctrl Pts',(-7.60792245236808,1.13566609521927,-10.05942165328));
#26367=CARTESIAN_POINT('Ctrl Pts',(-7.23087322735717,-2.62387007503327,
-9.90145262635776));
#26368=CARTESIAN_POINT('Ctrl Pts',(-5.10919715479364,-5.75033267684747,
-9.74348359943547));
#26369=CARTESIAN_POINT('Ctrl Pts',(-1.75480104650608,-7.48938548758801,
-9.58551457251319));
#26370=CARTESIAN_POINT('Ctrl Pts',(2.0229841775449,-7.42143898381695,-9.42754554559091));
#26371=CARTESIAN_POINT('Ctrl Pts',(5.3126744825953,-5.56288697198798,-9.2695765186686));
#26372=CARTESIAN_POINT('Ctrl Pts',(7.32055080798609,-2.36215102767096,-9.11160749174632));
#26373=CARTESIAN_POINT('Ctrl Pts',(7.56216337808177,1.40851221170973,-8.95363846482402));
#26374=CARTESIAN_POINT('Ctrl Pts',(5.97921719210332,4.8393370808664,-8.79566943790175));
#26375=CARTESIAN_POINT('Ctrl Pts',(2.95363712723051,7.10255231090489,-8.63770041097944));
#26376=CARTESIAN_POINT('Ctrl Pts',(-0.784580871228743,7.65210131057567,
-8.47973138405716));
#26377=CARTESIAN_POINT('Ctrl Pts',(-4.33349934959543,6.3553918051412,-8.32176235713486));
#26378=CARTESIAN_POINT('Ctrl Pts',(-6.83685404023092,3.52528700146243,-8.16379333021257));
#26379=CARTESIAN_POINT('Ctrl Pts',(-7.69064877262224,-0.155380392138265,
-8.00582430329029));
#26380=CARTESIAN_POINT('Ctrl Pts',(-6.68888447248521,-3.79855842705726,
-7.84785527636799));
#26381=CARTESIAN_POINT('Ctrl Pts',(-4.0732615282571,-6.52524038886781,-7.68988624944571));
#26382=CARTESIAN_POINT('Ctrl Pts',(-0.474863600532664,-7.67754688497162,
-7.53191722252343));
#26383=CARTESIAN_POINT('Ctrl Pts',(3.23810690347566,-6.97745550266942,-7.37394819560114));
#26384=CARTESIAN_POINT('Ctrl Pts',(6.16980411173903,-4.5938805853907,-7.21597916867884));
#26385=CARTESIAN_POINT('Ctrl Pts',(7.61288363807535,-1.10191847392946,-7.05801014175656));
#26386=CARTESIAN_POINT('Ctrl Pts',(7.21916689197791,2.65590869493537,-6.90004111483424));
#26387=CARTESIAN_POINT('Ctrl Pts',(5.08364776616928,5.77293227048303,-6.74207208791196));
#26388=CARTESIAN_POINT('Ctrl Pts',(1.72157301292862,7.49709330148819,-6.58410306098967));
#26389=CARTESIAN_POINT('Ctrl Pts',(-2.05587376531645,7.41239533964198,-6.42613403406738));
#26390=CARTESIAN_POINT('Ctrl Pts',(-5.33729020233292,5.53927386090847,-6.26816500714509));
#26391=CARTESIAN_POINT('Ctrl Pts',(-7.3309535073415,2.32966570203969,-6.11019598022282));
#26392=CARTESIAN_POINT('Ctrl Pts',(-7.55584314972316,-1.44203186748576,
-5.95222695330051));
#26393=CARTESIAN_POINT('Ctrl Pts',(-5.95769894680941,-4.8658036200867,-5.79425792637823));
#26394=CARTESIAN_POINT('Ctrl Pts',(-2.92211267358056,-7.11558002786579,
-5.63628889945594));
#26395=CARTESIAN_POINT('Ctrl Pts',(0.818505480028056,-7.64854694626547,
-5.47831987253366));
#26396=CARTESIAN_POINT('Ctrl Pts',(4.36163896341749,-6.33611293798186,-5.32035084561134));
#26397=CARTESIAN_POINT('Ctrl Pts',(6.85241928201679,-3.49493513437767,-5.16238181868907));
#26398=CARTESIAN_POINT('Ctrl Pts',(7.689884143197,0.189482121241377,-5.00441279176677));
#26399=CARTESIAN_POINT('Ctrl Pts',(6.67197445759853,3.82818213349571,-4.84644376484448));
#26400=CARTESIAN_POINT('Ctrl Pts',(4.04428608679874,6.5432386215229,-4.68847473792219));
#26401=CARTESIAN_POINT('Ctrl Pts',(0.440813773665348,7.679577125533,-4.5305057109999));
#26402=CARTESIAN_POINT('Ctrl Pts',(-3.26901575373787,6.96302790543571,-4.37253668407762));
#26403=CARTESIAN_POINT('Ctrl Pts',(-6.19011446159165,4.56647616466531,-4.21456765715532));
#26404=CARTESIAN_POINT('Ctrl Pts',(-7.61769511380036,1.06814922330403,-4.05659863023303));
#26405=CARTESIAN_POINT('Ctrl Pts',(-7.20731860617729,-2.68789510939572,
-3.89862960331074));
#26406=CARTESIAN_POINT('Ctrl Pts',(-5.05799841053314,-5.7954183359881,-3.74066057638846));
#26407=CARTESIAN_POINT('Ctrl Pts',(-1.68831112823367,-7.50465369916194,
-3.58269154946616));
#26408=CARTESIAN_POINT('Ctrl Pts',(2.088722927572,-7.4032059367478,-3.42472252254387));
#26409=CARTESIAN_POINT('Ctrl Pts',(5.36180097013677,-5.515551827941,-3.26675349562158));
#26410=CARTESIAN_POINT('Ctrl Pts',(7.34121205236302,-2.29713456556267,-3.10878446869929));
#26411=CARTESIAN_POINT('Ctrl Pts',(7.54937434451365,1.47552316703666,-2.950815441777));
#26412=CARTESIAN_POINT('Ctrl Pts',(5.93606355045319,4.89217447921103,-2.79284641485471));
#26413=CARTESIAN_POINT('Ctrl Pts',(2.89053076000349,7.12846782524383,-2.63487738793242));
#26414=CARTESIAN_POINT('Ctrl Pts',(-0.852413993867771,7.64484218235544,
-2.47690836101013));
#26415=CARTESIAN_POINT('Ctrl Pts',(-4.38969281076395,6.31670947861226,-2.31893933408784));
#26416=CARTESIAN_POINT('Ctrl Pts',(-6.86784977905936,3.46451454353091,-2.16097030716555));
#26417=CARTESIAN_POINT('Ctrl Pts',(-7.6889683012763,-0.223580124409053,
-2.00300128024326));
#26418=CARTESIAN_POINT('Ctrl Pts',(-6.65493324620604,-3.85773056324626,
-1.84503225332097));
#26419=CARTESIAN_POINT('Ctrl Pts',(-4.01523111922735,-6.56110818911341,
-1.68706322639868));
#26420=CARTESIAN_POINT('Ctrl Pts',(-0.406755278715055,-7.68145635627126,
-1.52909419947639));
#26421=CARTESIAN_POINT('Ctrl Pts',(3.2998603226626,-6.94846338847517,-1.3711251725541));
#26422=CARTESIAN_POINT('Ctrl Pts',(6.2103030901479,-4.5389819495744,-1.21315614563181));
#26423=CARTESIAN_POINT('Ctrl Pts',(7.62235679653987,-1.03435896878468,-1.05518711870952));
#26424=CARTESIAN_POINT('Ctrl Pts',(7.195328596961,2.71982866957056,-0.897218091787235));
#26425=CARTESIAN_POINT('Ctrl Pts',(5.03224959532673,5.81779044143021,-0.739249064864944));
#26426=CARTESIAN_POINT('Ctrl Pts',(1.65501604489259,7.51206652667632,-0.581280037942654));
#26427=CARTESIAN_POINT('Ctrl Pts',(-2.12153101755598,7.39387095854469,-0.423311011020362));
#26428=CARTESIAN_POINT('Ctrl Pts',(-5.38620630445157,5.49172133815517,-0.265341984098074));
#26429=CARTESIAN_POINT('Ctrl Pts',(-7.35132624111223,2.26455825864503,-0.107372957175783));
#26430=CARTESIAN_POINT('Ctrl Pts',(-7.54275708976602,-1.50898545216561,
0.0505960697465059));
#26431=CARTESIAN_POINT('Ctrl Pts',(-5.91431142841186,-4.91844913949706,
0.208565096668796));
#26432=CARTESIAN_POINT('Ctrl Pts',(-2.85889200754989,-7.14121544971374,
0.366534123591086));
#26433=CARTESIAN_POINT('Ctrl Pts',(0.88630574599214,-7.6409870916449,0.524503150513376));
#26434=CARTESIAN_POINT('Ctrl Pts',(4.41766033998119,-6.29718180860455,0.682472177435666));
#26435=CARTESIAN_POINT('Ctrl Pts',(6.88314522794016,-3.43402582709381,0.840441204357956));
#26436=CARTESIAN_POINT('Ctrl Pts',(7.68790126486706,0.257673731137408,0.998410231280246));
#26437=CARTESIAN_POINT('Ctrl Pts',(6.63776117340416,3.88720313527745,1.15637925820254));
#26438=CARTESIAN_POINT('Ctrl Pts',(3.98609719687402,6.57884874025357,1.31434828512483));
#26439=CARTESIAN_POINT('Ctrl Pts',(0.372688785402186,7.68318454023448,1.47231731204712));
#26440=CARTESIAN_POINT('Ctrl Pts',(-3.33064000372796,6.93376223818136,1.63028633896941));
#26441=CARTESIAN_POINT('Ctrl Pts',(-6.23036960042207,4.51139848075951,1.7882553658917));
#26442=CARTESIAN_POINT('Ctrl Pts',(-7.62686859462744,1.00054837481676,1.94622439281399));
#26443=CARTESIAN_POINT('Ctrl Pts',(-7.18319710009842,-2.75170874752403,
2.10419341973628));
#26444=CARTESIAN_POINT('Ctrl Pts',(-5.00640182687015,-5.84004814688836,
2.26216244665857));
#26445=CARTESIAN_POINT('Ctrl Pts',(-1.62168841761395,-7.51933163826675,
2.42013147358086));
#26446=CARTESIAN_POINT('Ctrl Pts',(2.15429739013586,-7.38439058859407,2.57810050050315));
#26447=CARTESIAN_POINT('Ctrl Pts',(5.41050572537514,-5.4677828601496,2.73606952742544));
#26448=CARTESIAN_POINT('Ctrl Pts',(7.36129587470557,-2.23193742186146,2.89403855434773));
#26449=CARTESIAN_POINT('Ctrl Pts',(7.53599151560073,1.54241806487627,3.05200758127002));
#26450=CARTESIAN_POINT('Ctrl Pts',(5.89244300841527,4.94462708428458,3.20997660819231));
#26451=CARTESIAN_POINT('Ctrl Pts',(2.8271970383585,7.15382265060854,3.3679456351146));
#26452=CARTESIAN_POINT('Ctrl Pts',(-0.920180069959813,7.63698174993965,
3.52591466203689));
#26453=CARTESIAN_POINT('Ctrl Pts',(-4.44554100112066,6.27753031194737,3.68388368895918));
#26454=CARTESIAN_POINT('Ctrl Pts',(-6.89830532789223,3.40346958459108,3.84185271588147));
#26455=CARTESIAN_POINT('Ctrl Pts',(-7.68668305495123,-0.291762271015844,
3.99982174280376));
#26456=CARTESIAN_POINT('Ctrl Pts',(-6.62045857686149,-3.91659927004588,
4.15779076972605));
#26457=CARTESIAN_POINT('Ctrl Pts',(-3.95688489262299,-6.59645992609632,
4.31575979664834));
#26458=CARTESIAN_POINT('Ctrl Pts',(-0.338614963604182,-7.68476164343996,
4.47372882357063));
#26459=CARTESIAN_POINT('Ctrl Pts',(3.3613541916878,-6.91892474363507,4.63169785049292));
#26460=CARTESIAN_POINT('Ctrl Pts',(6.25031359782997,-4.48372630061699,4.78966687741521));
#26461=CARTESIAN_POINT('Ctrl Pts',(7.63123041934389,-0.966718106245712,
4.94763590433751));
#26462=CARTESIAN_POINT('Ctrl Pts',(7.17092435414114,2.78353471637204,5.10560493125978));
#26463=CARTESIAN_POINT('Ctrl Pts',(4.98045561342925,5.862191014691,5.26357395818209));
#26464=CARTESIAN_POINT('Ctrl Pts',(1.58832890174619,7.52644889107342,5.42154298510437));
#26465=CARTESIAN_POINT('Ctrl Pts',(-2.18702140099965,7.37476501331616,5.57951201202667));
#26466=CARTESIAN_POINT('Ctrl Pts',(-5.43469875508803,5.44373686464613,5.73748103894893));
#26467=CARTESIAN_POINT('Ctrl Pts',(-7.37112075710193,2.19927269666223,5.89545006587125));
#26468=CARTESIAN_POINT('Ctrl Pts',(-7.52907775505485,-1.57582034775569,
6.05341909279352));
#26469=CARTESIAN_POINT('Ctrl Pts',(-5.8704587204801,-4.97070779881518,6.21138811971583));
#26470=CARTESIAN_POINT('Ctrl Pts',(-2.79544647567348,-7.16628918002251,
6.36935714663811));
#26471=CARTESIAN_POINT('Ctrl Pts',(0.954036299672317,-7.63282623599999,
6.5273261735604));
#26472=CARTESIAN_POINT('Ctrl Pts',(4.47333424594222,-6.25775537506413,6.68529520048269));
#26473=CARTESIAN_POINT('Ctrl Pts',(6.91332978081018,-3.37284641687486,6.84326422740498));
#26474=CARTESIAN_POINT('Ctrl Pts',(7.68531369548343,0.325845073733365,7.00123325432727));
#26475=CARTESIAN_POINT('Ctrl Pts',(6.60302579681321,3.94591838951186,7.15920228124957));
#26476=CARTESIAN_POINT('Ctrl Pts',(3.92759478089939,6.61394140033761,7.31717130817185));
#26477=CARTESIAN_POINT('Ctrl Pts',(0.304534483343064,7.68618763487766,7.47514033509413));
#26478=CARTESIAN_POINT('Ctrl Pts',(-3.39200228258501,6.90395119659456,7.63310936201643));
#26479=CARTESIAN_POINT('Ctrl Pts',(-6.27013469019421,4.45596595329453,7.79107838893872));
#26480=CARTESIAN_POINT('Ctrl Pts',(-7.63544218492327,0.932868828290557,
7.94904741586101));
#26481=CARTESIAN_POINT('Ctrl Pts',(-7.15851060041003,-2.81530595026851,
8.10701644278331));
#26482=CARTESIAN_POINT('Ctrl Pts',(-4.9544114652216,-5.88421860947506,8.26498546970558));
#26483=CARTESIAN_POINT('Ctrl Pts',(-1.55493815323402,-7.53341814504625,
8.42295449662788));
#26484=CARTESIAN_POINT('Ctrl Pts',(2.21970240660853,-7.36499442217634,8.58092352355018));
#26485=CARTESIAN_POINT('Ctrl Pts',(5.45878491797924,-5.41958382411224,8.73889255047245));
#26486=CARTESIAN_POINT('Ctrl Pts',(7.38080069488091,-2.16656472607635,8.89686157739476));
#26487=CARTESIAN_POINT('Ctrl Pts',(7.52201594451772,1.60919164537799,9.05483060431704));
#26488=CARTESIAN_POINT('Ctrl Pts',(5.84835899604979,4.99669076754189,9.21279963123934));
#26489=CARTESIAN_POINT('Ctrl Pts',(2.76364094548598,7.1786147980614,9.37076865816163));
#26490=CARTESIAN_POINT('Ctrl Pts',(-0.987873772599122,7.6285206213513,9.52873768508391));
#26491=CARTESIAN_POINT('Ctrl Pts',(-4.50103952168514,6.23785740659357,9.68670671200621));
#26492=CARTESIAN_POINT('Ctrl Pts',(-6.92821830337425,3.34215688767999,9.84467573892849));
#26493=CARTESIAN_POINT('Ctrl Pts',(-7.68379318985292,-0.359921394442083,
10.0026447658508));
#26494=CARTESIAN_POINT('Ctrl Pts',(-6.58546322177129,-3.97516006214074,
10.1606137927731));
#26495=CARTESIAN_POINT('Ctrl Pts',(-3.89822734886324,-6.6312925376092,10.3185828196954));
#26496=CARTESIAN_POINT('Ctrl Pts',(-0.270448187237914,-7.68746303348714,
10.4765518466177));
#26497=CARTESIAN_POINT('Ctrl Pts',(3.42258400874207,-6.88884082910166,10.63452087354));
#26498=CARTESIAN_POINT('Ctrl Pts',(6.28983183712536,-4.4281200481492,10.7924899004623));
#26499=CARTESIAN_POINT('Ctrl Pts',(7.63950507226382,-0.898997198667169,
10.9504589273846));
#26500=CARTESIAN_POINT('Ctrl Pts',(7.14595362848161,2.8470140399453,11.1084279543069));
#26501=CARTESIAN_POINT('Ctrl Pts',(4.92827466194258,5.90614561821491,11.2663969812292));
#26502=CARTESIAN_POINT('Ctrl Pts',(1.52150756701962,7.5402098924435,11.4243660081514));
#26503=CARTESIAN_POINT('Ctrl Pts',(-2.25232175897465,7.35513608411886,11.5823350350737));
#26504=CARTESIAN_POINT('Ctrl Pts',(-5.48279887906735,5.39521304718891,11.740304061996));
#26505=CARTESIAN_POINT('Ctrl Pts',(-7.39026556096377,2.13403316693694,11.8982730889183));
#26506=CARTESIAN_POINT('Ctrl Pts',(-7.51496606468558,-1.64319871482238,
12.0562509298068));
#26507=CARTESIAN_POINT('Ctrl Pts',(-6.38858261358109,-3.89562257101338,
12.1615724283879));
#26508=CARTESIAN_POINT('Ctrl Pts',(-5.59099016251816,-4.82066458193201,
12.2142375846616));
#26509=CARTESIAN_POINT('Ctrl Pts',(-1.81369530454162,6.77185709926922,-12.6435835482508));
#26510=CARTESIAN_POINT('Ctrl Pts',(-2.93392826290543,6.47182695586933,-12.5909272059434));
#26511=CARTESIAN_POINT('Ctrl Pts',(-5.02154850583196,5.30552096540475,-12.4856145213285));
#26512=CARTESIAN_POINT('Ctrl Pts',(-6.94196157239741,2.27379792622978,-12.3276454944063));
#26513=CARTESIAN_POINT('Ctrl Pts',(-7.18718979160325,-1.30562067836087,
-12.169676467484));
#26514=CARTESIAN_POINT('Ctrl Pts',(-5.69846535245324,-4.57047627984927,
-12.0117074405617));
#26515=CARTESIAN_POINT('Ctrl Pts',(-2.83477632842897,-6.73236177450464,
-11.8537384136394));
#26516=CARTESIAN_POINT('Ctrl Pts',(0.712837007271223,-7.27001675403625,
-11.6957693867171));
#26517=CARTESIAN_POINT('Ctrl Pts',(4.08847908705196,-6.05353978254254,-11.5378003597948));
#26518=CARTESIAN_POINT('Ctrl Pts',(6.47766515763744,-3.37652806502808,-11.3798313328725));
#26519=CARTESIAN_POINT('Ctrl Pts',(7.30395930917253,0.11517058512602,-11.2218623059502));
#26520=CARTESIAN_POINT('Ctrl Pts',(6.36799032002208,3.57907319090322,-11.0638932790279));
#26521=CARTESIAN_POINT('Ctrl Pts',(3.89558761425688,6.17944023049411,-10.9059242521056));
#26522=CARTESIAN_POINT('Ctrl Pts',(0.483277485164234,7.28886243758025,-10.7479552251834));
#26523=CARTESIAN_POINT('Ctrl Pts',(-3.04563493721468,6.63966762466852,-10.5899861982611));
#26524=CARTESIAN_POINT('Ctrl Pts',(-5.83971285652995,4.38848836535718,-10.4320171713388));
#26525=CARTESIAN_POINT('Ctrl Pts',(-7.22481567467033,1.07847815974754,-10.2740481444165));
#26526=CARTESIAN_POINT('Ctrl Pts',(-6.86675325118532,-2.49174170282166,
-10.1160791174942));
#26527=CARTESIAN_POINT('Ctrl Pts',(-4.85191692213481,-5.46076723551842,
-9.95811009057192));
#26528=CARTESIAN_POINT('Ctrl Pts',(-1.66643576956793,-7.11224779210676,
-9.80014106364962));
#26529=CARTESIAN_POINT('Ctrl Pts',(1.92111419208633,-7.04772282243761,-9.64217203672734));
#26530=CARTESIAN_POINT('Ctrl Pts',(5.04514788585,-5.28276060163156,-9.48420300980503));
#26531=CARTESIAN_POINT('Ctrl Pts',(6.95191500122294,-2.24320185668345,-9.32623398288276));
#26532=CARTESIAN_POINT('Ctrl Pts',(7.18136085776967,1.3375847570525,-9.16826495596046));
#26533=CARTESIAN_POINT('Ctrl Pts',(5.67812597489346,4.59564600135666,-9.01029592903816));
#26534=CARTESIAN_POINT('Ctrl Pts',(2.8049029084755,6.74489410049379,-8.85232690211588));
#26535=CARTESIAN_POINT('Ctrl Pts',(-0.745072286421055,7.26676984931728,
-8.6943578751936));
#26536=CARTESIAN_POINT('Ctrl Pts',(-4.11528038346203,6.0353578286229,-8.5363888482713));
#26537=CARTESIAN_POINT('Ctrl Pts',(-6.49257540998183,3.34776661372903,-8.37841982134901));
#26538=CARTESIAN_POINT('Ctrl Pts',(-7.30337620404243,-0.147556011471637,
-8.22045079442673));
#26539=CARTESIAN_POINT('Ctrl Pts',(-6.35205704125284,-3.60727710314818,
-8.06248176750443));
#26540=CARTESIAN_POINT('Ctrl Pts',(-3.86814717429505,-6.19665346717748,
-7.90451274058214));
#26541=CARTESIAN_POINT('Ctrl Pts',(-0.450951229581856,-7.29093407889479,
-7.74654371365985));
#26542=CARTESIAN_POINT('Ctrl Pts',(3.07504784111031,-6.62609670387868,-7.58857468673757));
#26543=CARTESIAN_POINT('Ctrl Pts',(5.85911564362261,-4.36254978526543,-7.43060565981527));
#26544=CARTESIAN_POINT('Ctrl Pts',(7.22952703345288,-1.04642994358814,-7.27263663289299));
#26545=CARTESIAN_POINT('Ctrl Pts',(6.85563640346892,2.52216697656922,-7.11466760597068));
#26546=CARTESIAN_POINT('Ctrl Pts',(4.82765410602869,5.48222879737866,-6.9566985790484));
#26547=CARTESIAN_POINT('Ctrl Pts',(1.6348809766094,7.11956746906614,-6.79872955212611));
#26548=CARTESIAN_POINT('Ctrl Pts',(-1.95234758211534,7.03913458266514,-6.64076052520382));
#26549=CARTESIAN_POINT('Ctrl Pts',(-5.06852404917411,5.26033655930947,-6.48279149828154));
#26550=CARTESIAN_POINT('Ctrl Pts',(-6.96179385919399,2.21235237165163,-6.32482247135924));
#26551=CARTESIAN_POINT('Ctrl Pts',(-7.17535889268673,-1.36941648719649,
-6.16685344443695));
#26552=CARTESIAN_POINT('Ctrl Pts',(-5.65769130868016,-4.62077978375393,
-6.00888441751466));
#26553=CARTESIAN_POINT('Ctrl Pts',(-2.77496590947326,-6.75726578991277,
-5.85091539059237));
#26554=CARTESIAN_POINT('Ctrl Pts',(0.777288577654942,-7.26339446962032,
-5.69294636367007));
#26555=CARTESIAN_POINT('Ctrl Pts',(4.14200299062499,-6.01704977376104,-5.53497733674778));
#26556=CARTESIAN_POINT('Ctrl Pts',(6.50735684388032,-3.31894315417848,-5.37700830982551));
#26557=CARTESIAN_POINT('Ctrl Pts',(7.30265007852113,0.17994050388728,-5.2190392829032));
#26558=CARTESIAN_POINT('Ctrl Pts',(6.33599855204277,3.6354090695238,-5.06107025598093));
#26559=CARTESIAN_POINT('Ctrl Pts',(3.84063082867778,6.21374537554234,-4.90310122905862));
#26560=CARTESIAN_POINT('Ctrl Pts',(0.418616025797775,7.29286208406613,-4.74513220213635));
#26561=CARTESIAN_POINT('Ctrl Pts',(-3.10440023622982,6.61239562696912,-4.58716317521405));
#26562=CARTESIAN_POINT('Ctrl Pts',(-5.87840323953228,4.33652534959964,-4.42919414829176));
#26563=CARTESIAN_POINT('Ctrl Pts',(-7.23409622109299,1.01436118726629,-4.27122512136947));
#26564=CARTESIAN_POINT('Ctrl Pts',(-6.84438475342828,-2.55254267374759,
-4.11325609444718));
#26565=CARTESIAN_POINT('Ctrl Pts',(-4.80329635687898,-5.50358254796429,
-3.95528706752489));
#26566=CARTESIAN_POINT('Ctrl Pts',(-1.60329403715022,-7.12674715313392,
-3.7973180406026));
#26567=CARTESIAN_POINT('Ctrl Pts',(1.98354258230751,-7.03040792404231,-3.63934901368031));
#26568=CARTESIAN_POINT('Ctrl Pts',(5.09180054555484,-5.23780908000201,-3.48137998675802));
#26569=CARTESIAN_POINT('Ctrl Pts',(6.97153582190916,-2.18145938263847,-3.32341095983573));
#26570=CARTESIAN_POINT('Ctrl Pts',(7.16921583253244,1.40122128902976,-3.16544193291344));
#26571=CARTESIAN_POINT('Ctrl Pts',(5.63714539069785,4.64582270415024,-3.00747290599115));
#26572=CARTESIAN_POINT('Ctrl Pts',(2.74497434401289,6.76950460558047,-2.84950387906886));
#26573=CARTESIAN_POINT('Ctrl Pts',(-0.809489584411743,7.25987626388997,
-2.69153485214657));
#26574=CARTESIAN_POINT('Ctrl Pts',(-4.16864415019417,5.99862340069084,-2.53356582522428));
#26575=CARTESIAN_POINT('Ctrl Pts',(-6.52201031828139,3.29005443153989,-2.37559679830199));
#26576=CARTESIAN_POINT('Ctrl Pts',(-7.30178035500522,-0.21232145799179,
-2.2176277713797));
#26577=CARTESIAN_POINT('Ctrl Pts',(-6.31981547289671,-3.66346954986654,
-2.05965874445741));
#26578=CARTESIAN_POINT('Ctrl Pts',(-3.81303896158777,-6.23071509793841,
-1.90168971753512));
#26579=CARTESIAN_POINT('Ctrl Pts',(-0.38627259042325,-7.29464668370934,
-1.74372069061283));
#26580=CARTESIAN_POINT('Ctrl Pts',(3.13369158698175,-6.5985645251027,-1.58575166369054));
#26581=CARTESIAN_POINT('Ctrl Pts',(5.89757524357891,-4.31041564127977,-1.42778263676825));
#26582=CARTESIAN_POINT('Ctrl Pts',(7.23852315876718,-0.982272484728769,
-1.26981360984596));
#26583=CARTESIAN_POINT('Ctrl Pts',(6.83299851663794,2.58286817818637,-1.11184458292367));
#26584=CARTESIAN_POINT('Ctrl Pts',(4.77884415657435,5.52482807709338,-0.953875556001376));
#26585=CARTESIAN_POINT('Ctrl Pts',(1.57167557080567,7.13378669812861,-0.795906529079087));
#26586=CARTESIAN_POINT('Ctrl Pts',(-2.0146985784755,7.02154302074358,-0.637937502156794));
#26587=CARTESIAN_POINT('Ctrl Pts',(-5.11497691768626,5.21517860535962,-0.479968475234507));
#26588=CARTESIAN_POINT('Ctrl Pts',(-6.98114069759888,2.15052349780065,-0.321999448312216));
#26589=CARTESIAN_POINT('Ctrl Pts',(-7.16293179820856,-1.43299853749984,
-0.164030421389927));
#26590=CARTESIAN_POINT('Ctrl Pts',(-5.61648862490333,-4.67077426992521,
-0.0060613944676359));
#26591=CARTESIAN_POINT('Ctrl Pts',(-2.71492880187113,-6.7816103069282,0.151907632454654));
#26592=CARTESIAN_POINT('Ctrl Pts',(0.841674673511063,-7.2562153012596,0.309876659376944));
#26593=CARTESIAN_POINT('Ctrl Pts',(4.1952033382952,-5.98007907176994,0.467845686299233));
#26594=CARTESIAN_POINT('Ctrl Pts',(6.53653554504559,-3.2611010138632,0.625814713221524));
#26595=CARTESIAN_POINT('Ctrl Pts',(7.30076705059481,0.244698237045366,0.783783740143812));
#26596=CARTESIAN_POINT('Ctrl Pts',(6.30350812203683,3.69145799240351,0.941752767066107));
#26597=CARTESIAN_POINT('Ctrl Pts',(3.78537211558601,6.24756230067438,1.09972179398839));
#26598=CARTESIAN_POINT('Ctrl Pts',(0.353921559454047,7.2962878427333,1.25769082091068));
#26599=CARTESIAN_POINT('Ctrl Pts',(-3.16292131738643,6.58460367025127,1.41565984783297));
#26600=CARTESIAN_POINT('Ctrl Pts',(-5.91663127876754,4.28422117372264,1.57362887475526));
#26601=CARTESIAN_POINT('Ctrl Pts',(-7.24280775942501,0.950164466961936,
1.73159790167755));
#26602=CARTESIAN_POINT('Ctrl Pts',(-6.82147791699476,-2.61314289357025,
1.88956692859984));
#26603=CARTESIAN_POINT('Ctrl Pts',(-4.75429798593847,-5.54596496699767,
2.04753595552213));
#26604=CARTESIAN_POINT('Ctrl Pts',(-1.54002619931564,-7.1406859656258,2.20550498244442));
#26605=CARTESIAN_POINT('Ctrl Pts',(2.04581495797322,-7.01254004708686,2.36347400936671));
#26606=CARTESIAN_POINT('Ctrl Pts',(5.1380527098323,-5.19244558038397,2.52144303628901));
#26607=CARTESIAN_POINT('Ctrl Pts',(6.99060829739458,-2.11954532545592,2.67941206321129));
#26608=CARTESIAN_POINT('Ctrl Pts',(7.15650691328321,1.46474760774462,2.83738109013358));
#26609=CARTESIAN_POINT('Ctrl Pts',(5.59572141748752,4.69563399043573,2.99535011705587));
#26610=CARTESIAN_POINT('Ctrl Pts',(2.68482987385815,6.79358265591159,3.15331914397817));
#26611=CARTESIAN_POINT('Ctrl Pts',(-0.873843212071065,7.25241165371776,
3.31128817090046));
#26612=CARTESIAN_POINT('Ctrl Pts',(-4.2216800326729,5.96141715165069,3.46925719782274));
#26613=CARTESIAN_POINT('Ctrl Pts',(-6.55093223855147,3.23208347048325,3.62722622474502));
#26614=CARTESIAN_POINT('Ctrl Pts',(-7.29961018521533,-0.277070204396807,
3.78519525166733));
#26615=CARTESIAN_POINT('Ctrl Pts',(-6.28707682012798,-3.71937384677498,
3.94316427858961));
#26616=CARTESIAN_POINT('Ctrl Pts',(-3.75763083470842,-6.26428665246989,
4.10113330551191));
#26617=CARTESIAN_POINT('Ctrl Pts',(-0.321563569035062,-7.29778552886652,
4.2591023324342));
#26618=CARTESIAN_POINT('Ctrl Pts',(3.19208885267565,-6.57051333693858,4.41707135935648));
#26619=CARTESIAN_POINT('Ctrl Pts',(5.93557097038379,-4.25794246201158,4.57504038627877));
#26620=CARTESIAN_POINT('Ctrl Pts',(7.24694993881483,-0.918037765332063,
4.73300941320106));
#26621=CARTESIAN_POINT('Ctrl Pts',(6.80982318103779,2.64336622458265,4.89097844012336));
#26622=CARTESIAN_POINT('Ctrl Pts',(4.72965832764282,5.5669928020452,5.04894746704564));
#26623=CARTESIAN_POINT('Ctrl Pts',(1.50834654502766,7.14744481995958,5.20691649396794));
#26624=CARTESIAN_POINT('Ctrl Pts',(-2.07689110893389,7.00339918010499,5.36488552089023));
#26625=CARTESIAN_POINT('Ctrl Pts',(-5.16102746823473,5.16961045209314,5.52285454781252));
#26626=CARTESIAN_POINT('Ctrl Pts',(-6.99993843512712,2.08852547475349,5.68082357473481));
#26627=CARTESIAN_POINT('Ctrl Pts',(-7.14994130409418,-1.49646787545607,
5.8387926016571));
#26628=CARTESIAN_POINT('Ctrl Pts',(-5.57484417681309,-4.72040137684468,
5.99676162857939));
#26629=CARTESIAN_POINT('Ctrl Pts',(-2.65467815183384,-6.80542141710859,
6.15473065550168));
#26630=CARTESIAN_POINT('Ctrl Pts',(0.905994567535526,-7.24846539605865,
6.31269968242397));
#26631=CARTESIAN_POINT('Ctrl Pts',(4.24807371269448,-5.94263800729767,6.47066870934625));
#26632=CARTESIAN_POINT('Ctrl Pts',(6.56520011570513,-3.20300237199555,6.62863773626855));
#26633=CARTESIAN_POINT('Ctrl Pts',(7.29830978161512,0.309436723489496,6.78660676319084));
#26634=CARTESIAN_POINT('Ctrl Pts',(6.27052189027236,3.74721656404915,6.94457579011314));
#26635=CARTESIAN_POINT('Ctrl Pts',(3.72981566445421,6.28088782445943,7.10254481703542));
#26636=CARTESIAN_POINT('Ctrl Pts',(0.289199255448475,7.2991397126605,7.2605138439577));
#26637=CARTESIAN_POINT('Ctrl Pts',(-3.22119361930532,6.55629380223107,7.41848287088));
#26638=CARTESIAN_POINT('Ctrl Pts',(-5.95439394599886,4.23158002289297,7.5764518978023));
#26639=CARTESIAN_POINT('Ctrl Pts',(-7.25094961548957,0.885893011560218,
7.73442092472457));
#26640=CARTESIAN_POINT('Ctrl Pts',(-6.79803453793589,-2.67353757689281,
7.89238995164688));
#26641=CARTESIAN_POINT('Ctrl Pts',(-4.7049256662123,-5.58791116879611,8.05035897856914));
#26642=CARTESIAN_POINT('Ctrl Pts',(-1.47663723085548,-7.15406312813226,
8.20832800549145));
#26643=CARTESIAN_POINT('Ctrl Pts',(2.10792642022488,-6.99412059972255,8.36629703241375));
#26644=CARTESIAN_POINT('Ctrl Pts',(5.18390074123251,-5.14667366916288,8.52426605933602));
#26645=CARTESIAN_POINT('Ctrl Pts',(7.009130927116,-2.05746455634179,8.68223508625831));
#26646=CARTESIAN_POINT('Ctrl Pts',(7.14323510016273,1.52815871821309,8.84020411318062));
#26647=CARTESIAN_POINT('Ctrl Pts',(5.55385731259759,4.74507593956618,8.9981731401029));
#26648=CARTESIAN_POINT('Ctrl Pts',(2.62447423026674,6.81712636270509,9.15614216702519));
#26649=CARTESIAN_POINT('Ctrl Pts',(-0.938128110736495,7.2443765962059,9.31411119394749));
#26650=CARTESIAN_POINT('Ctrl Pts',(-4.27438385343418,5.92374202677208,9.47208022086977));
#26651=CARTESIAN_POINT('Ctrl Pts',(-6.57933890745375,3.17385825374728,9.63004924779207));
#26652=CARTESIAN_POINT('Ctrl Pts',(-7.29686584301274,-0.34179708698331,
9.78801827471435));
#26653=CARTESIAN_POINT('Ctrl Pts',(-6.25384370141794,-3.77498573442195,
9.94598730163664));
#26654=CARTESIAN_POINT('Ctrl Pts',(-3.7019270674518,-6.297365222766,10.1039563285589));
#26655=CARTESIAN_POINT('Ctrl Pts',(-0.256829418882215,-7.30035088692299,
10.2619253554812));
#26656=CARTESIAN_POINT('Ctrl Pts',(3.25023536307719,-6.54194433684203,10.4198943824035));
#26657=CARTESIAN_POINT('Ctrl Pts',(5.97309921761348,-4.20513633432635,10.5778634093258));
#26658=CARTESIAN_POINT('Ctrl Pts',(7.25480791088178,-0.853727031667314,
10.7358324362481));
#26659=CARTESIAN_POINT('Ctrl Pts',(6.78610988857427,2.70364896469217,10.8938014631704));
#26660=CARTESIAN_POINT('Ctrl Pts',(4.6801050154764,5.6087340146432,11.0517704900927));
#26661=CARTESIAN_POINT('Ctrl Pts',(1.44489008506012,7.16051286830262,11.2097395170149));
#26662=CARTESIAN_POINT('Ctrl Pts',(-2.13890318290192,6.98475869103198,11.3677085439373));
#26663=CARTESIAN_POINT('Ctrl Pts',(-5.20670544824242,5.12353011424077,11.5256775708595));
#26664=CARTESIAN_POINT('Ctrl Pts',(-7.01811917762225,2.02657116594995,11.6836465977818));
#26665=CARTESIAN_POINT('Ctrl Pts',(-7.13654022615019,-1.5604533176796,11.8416244386703));
#26666=CARTESIAN_POINT('Ctrl Pts',(-6.06687727096378,-3.69945345656046,
11.9469459372515));
#26667=CARTESIAN_POINT('Ctrl Pts',(-5.3094486196446,-4.57791378026331,11.9996110935251));
#26668=CARTESIAN_POINT('Ctrl Pts',(-5.31037376991248,-4.57794244025911,
12.));
#26669=CARTESIAN_POINT('Ctrl Pts',(-5.44263380122459,-4.44687739974309,
12.));
#26670=CARTESIAN_POINT('Ctrl Pts',(-5.5693014092247,-4.3106898541843,12.));
#26671=CARTESIAN_POINT('Ctrl Pts',(-5.69024917409142,-4.1698511932344,12.));
#26672=CARTESIAN_POINT('Ctrl Pts',(-5.81418999782626,-4.02552723924421,
12.));
#26673=CARTESIAN_POINT('Ctrl Pts',(-5.93212486388003,-3.876318788248,12.));
#26674=CARTESIAN_POINT('Ctrl Pts',(-6.04389086929985,-3.72268453170137,
12.));
#26675=CARTESIAN_POINT('Ctrl Pts',(-6.15652040037929,-3.56786326733222,
12.));
#26676=CARTESIAN_POINT('Ctrl Pts',(-6.26288583253187,-3.40854703539605,
12.));
#26677=CARTESIAN_POINT('Ctrl Pts',(-6.36278756125166,-3.24516313822355,
12.));
#26678=CARTESIAN_POINT('Ctrl Pts',(-6.46266655647491,-3.08181642046033,
12.));
#26679=CARTESIAN_POINT('Ctrl Pts',(-6.55608521685512,-2.914403315385,12.));
#26680=CARTESIAN_POINT('Ctrl Pts',(-6.64280476241556,-2.74331712888927,
12.));
#26681=CARTESIAN_POINT('Ctrl Pts',(-6.71416600011118,-2.60253085121616,
12.));
#26682=CARTESIAN_POINT('Ctrl Pts',(-6.78099027006545,-2.45925655037198,
12.));
#26683=CARTESIAN_POINT('Ctrl Pts',(-6.84312140434658,-2.31370042357453,
12.));
#26684=CARTESIAN_POINT('Ctrl Pts',(-6.85476347855885,-2.28642625177913,
12.));
#26685=CARTESIAN_POINT('Ctrl Pts',(-6.86623701980134,-2.25908044570938,
12.));
#26686=CARTESIAN_POINT('Ctrl Pts',(-6.87753655261754,-2.23167620907008,
12.));
#26687=CARTESIAN_POINT('Ctrl Pts',(-6.95229594262949,-2.05036570285519,
12.));
#26688=CARTESIAN_POINT('Ctrl Pts',(-7.01950773615009,-1.86634543828863,
12.));
#26689=CARTESIAN_POINT('Ctrl Pts',(-7.07899546236369,-1.68007671471902,
12.));
#26690=CARTESIAN_POINT('Ctrl Pts',(-7.0921962818188,-1.63874214124503,12.));
#26691=CARTESIAN_POINT('Ctrl Pts',(-7.1050165991878,-1.59729670185842,12.));
#26692=CARTESIAN_POINT('Ctrl Pts',(-7.11745423244715,-1.55574520184557,
12.));
#26693=CARTESIAN_POINT('Ctrl Pts',(-7.17295666561696,-1.37032332097173,
12.));
#26694=CARTESIAN_POINT('Ctrl Pts',(-7.22084218410379,-1.18279157288797,
12.));
#26695=CARTESIAN_POINT('Ctrl Pts',(-7.26118675281216,-0.993630970717798,
12.));
#26696=CARTESIAN_POINT('Ctrl Pts',(-7.30190404530392,-0.80272280604871,
12.));
#26697=CARTESIAN_POINT('Ctrl Pts',(-7.33494057259123,-0.610154914422011,
12.));
#26698=CARTESIAN_POINT('Ctrl Pts',(-7.36032600263038,-0.416399269132085,
12.));
#26699=CARTESIAN_POINT('Ctrl Pts',(-7.38580045309683,-0.22196417069481,
12.));
#26700=CARTESIAN_POINT('Ctrl Pts',(-7.40357018172954,-0.0263322814024089,
12.));
#26701=CARTESIAN_POINT('Ctrl Pts',(-7.41361448974918,0.170031926235426,
12.));
#26702=CARTESIAN_POINT('Ctrl Pts',(-7.41789307147214,0.2536773409518,12.));
#26703=CARTESIAN_POINT('Ctrl Pts',(-7.42076922976018,0.337455728705427,
12.));
#26704=CARTESIAN_POINT('Ctrl Pts',(-7.42223849461264,0.421331393594551,
12.));
#26705=CARTESIAN_POINT('Ctrl Pts',(-7.42278385315547,0.452464181060878,
12.));
#26706=CARTESIAN_POINT('Ctrl Pts',(-7.42313532094487,0.483614843921272,
12.));
#26707=CARTESIAN_POINT('Ctrl Pts',(-7.42329265508154,0.514752665167828,
12.));
#26708=CARTESIAN_POINT('Ctrl Pts',(-7.42430042249123,0.714198774723802,
12.));
#26709=CARTESIAN_POINT('Ctrl Pts',(-7.41735325724622,0.913326000511656,
12.));
#26710=CARTESIAN_POINT('Ctrl Pts',(-7.40253605861267,1.11163646571176,12.));
#26711=CARTESIAN_POINT('Ctrl Pts',(-7.3875739546921,1.31188631470432,12.));
#26712=CARTESIAN_POINT('Ctrl Pts',(-7.36458728597274,1.51130404209091,12.));
#26713=CARTESIAN_POINT('Ctrl Pts',(-7.33361305290546,1.70939347351054,12.));
#26714=CARTESIAN_POINT('Ctrl Pts',(-7.31331709001647,1.83919219169224,12.));
#26715=CARTESIAN_POINT('Ctrl Pts',(-7.28959057761779,1.96842091312578,12.));
#26716=CARTESIAN_POINT('Ctrl Pts',(-7.26243189542493,2.09694161440494,12.));
#26717=CARTESIAN_POINT('Ctrl Pts',(-7.22127493916038,2.29170514689428,12.));
#26718=CARTESIAN_POINT('Ctrl Pts',(-7.17223845250762,2.48484324799321,12.));
#26719=CARTESIAN_POINT('Ctrl Pts',(-7.11556674570035,2.67596142142443,12.));
#26720=CARTESIAN_POINT('Ctrl Pts',(-7.05858971833812,2.86810924986448,12.));
#26721=CARTESIAN_POINT('Ctrl Pts',(-6.99389479095136,3.05821598378138,12.0000000000001));
#26722=CARTESIAN_POINT('Ctrl Pts',(-6.92167929314466,3.24586878138439,12.));
#26723=CARTESIAN_POINT('Ctrl Pts',(-6.91269242292701,3.26922126650541,12.));
#26724=CARTESIAN_POINT('Ctrl Pts',(-6.90358902237198,3.29253572590266,12.));
#26725=CARTESIAN_POINT('Ctrl Pts',(-6.89436941923266,3.31581134310704,12.));
#26726=CARTESIAN_POINT('Ctrl Pts',(-6.88573306865334,3.33761449310057,12.));
#26727=CARTESIAN_POINT('Ctrl Pts',(-6.87699606722048,3.35938015973985,12.));
#26728=CARTESIAN_POINT('Ctrl Pts',(-6.86816257821046,3.38109857716582,12.));
#26729=CARTESIAN_POINT('Ctrl Pts',(-6.7899490171883,3.57339799189585,12.));
#26730=CARTESIAN_POINT('Ctrl Pts',(-6.70409267881087,3.76220414798894,12.));
#26731=CARTESIAN_POINT('Ctrl Pts',(-6.61094013320699,3.94709682805149,12.));
#26732=CARTESIAN_POINT('Ctrl Pts',(-6.5188674146208,4.12984622678978,12.));
#26733=CARTESIAN_POINT('Ctrl Pts',(-6.41966627981606,4.30877300552798,12.));
#26734=CARTESIAN_POINT('Ctrl Pts',(-6.3136173503513,4.48346635617926,12.));
#26735=CARTESIAN_POINT('Ctrl Pts',(-6.20570281127415,4.66123290705839,12.));
#26736=CARTESIAN_POINT('Ctrl Pts',(-6.09069729335284,4.8346165151789,12.));
#26737=CARTESIAN_POINT('Ctrl Pts',(-5.96884373944417,5.00316848119551,12.));
#26738=CARTESIAN_POINT('Ctrl Pts',(-5.84699018553566,5.17172044721195,12.));
#26739=CARTESIAN_POINT('Ctrl Pts',(-5.71828830820229,5.33544150355174,12.));
#26740=CARTESIAN_POINT('Ctrl Pts',(-5.58293216084951,5.49385617917438,12.));
#26741=CARTESIAN_POINT('Ctrl Pts',(-5.48072057973372,5.61347996268186,12.));
#26742=CARTESIAN_POINT('Ctrl Pts',(-5.37471348591305,5.73007739213431,12.));
#26743=CARTESIAN_POINT('Ctrl Pts',(-5.265078497822,5.84352819974904,12.));
#26744=CARTESIAN_POINT('Ctrl Pts',(-5.24734949338018,5.86187425794772,12.));
#26745=CARTESIAN_POINT('Ctrl Pts',(-5.22953248896639,5.88013086749493,12.));
#26746=CARTESIAN_POINT('Ctrl Pts',(-5.21162852071991,5.89829754304194,12.));
#26747=CARTESIAN_POINT('Ctrl Pts',(-5.06686638441565,6.04518379337078,12.));
#26748=CARTESIAN_POINT('Ctrl Pts',(-4.91642028229973,6.18619532035819,12.));
#26749=CARTESIAN_POINT('Ctrl Pts',(-4.76074935872281,6.32112569416813,12.));
#26750=CARTESIAN_POINT('Ctrl Pts',(-4.60343491033637,6.45748062056515,12.));
#26751=CARTESIAN_POINT('Ctrl Pts',(-4.44078428855073,6.58762579282384,12.));
#26752=CARTESIAN_POINT('Ctrl Pts',(-4.27322757239386,6.7113180635556,12.));
#26753=CARTESIAN_POINT('Ctrl Pts',(-4.1903288657841,6.77251483021751,12.));
#26754=CARTESIAN_POINT('Ctrl Pts',(-4.10622862835614,6.83213156370766,12.));
#26755=CARTESIAN_POINT('Ctrl Pts',(-4.02097557077802,6.89013557177268,12.));
#26756=CARTESIAN_POINT('Ctrl Pts',(-3.95347972739972,6.93605802376314,12.));
#26757=CARTESIAN_POINT('Ctrl Pts',(-3.88526124287464,6.98096956683595,12.));
#26758=CARTESIAN_POINT('Ctrl Pts',(-3.81634342773284,7.02485291118474,12.));
#26759=CARTESIAN_POINT('Ctrl Pts',(-3.79116897753097,7.04088271515818,12.));
#26760=CARTESIAN_POINT('Ctrl Pts',(-3.76590910034549,7.05677028659542,12.));
#26761=CARTESIAN_POINT('Ctrl Pts',(-3.74056584986644,7.0725145443284,12.));
#26762=CARTESIAN_POINT('Ctrl Pts',(-3.56101544976198,7.18405855395118,12.));
#26763=CARTESIAN_POINT('Ctrl Pts',(-3.37727141976454,7.28841963306843,12.));
#26764=CARTESIAN_POINT('Ctrl Pts',(-3.18978287088803,7.38535844839708,12.));
#26765=CARTESIAN_POINT('Ctrl Pts',(-3.00212282400591,7.48238593481309,12.));
#26766=CARTESIAN_POINT('Ctrl Pts',(-2.8107108547889,7.57197802781875,12.));
#26767=CARTESIAN_POINT('Ctrl Pts',(-2.61596266530345,7.65385608862354,12.));
#26768=CARTESIAN_POINT('Ctrl Pts',(-2.53573323788768,7.68758697954293,12.));
#26769=CARTESIAN_POINT('Ctrl Pts',(-2.45493724389214,7.72000819012581,12.));
#26770=CARTESIAN_POINT('Ctrl Pts',(-2.37360237640543,7.75109805319064,12.));
#26771=CARTESIAN_POINT('Ctrl Pts',(-2.28382628244401,7.78541453459649,12.));
#26772=CARTESIAN_POINT('Ctrl Pts',(-2.19339366251994,7.81810902050074,12.));
#26773=CARTESIAN_POINT('Ctrl Pts',(-2.10234959246262,7.84917916318753,12.));
#26774=CARTESIAN_POINT('',(-5.31059994331846,-4.57805082698748,-12.0001612281326));
#26775=CARTESIAN_POINT('Ctrl Pts',(-5.31041659161217,-4.57789276698681,
-12.0001612281326));
#26776=CARTESIAN_POINT('Ctrl Pts',(-5.30898519516614,-4.57955320593178,
-12.0001074854218));
#26777=CARTESIAN_POINT('Ctrl Pts',(-5.30755301995135,-4.58121297353208,
-12.0000537427109));
#26778=CARTESIAN_POINT('Ctrl Pts',(-5.30612006659788,-4.5828720690575,-12.));
#26779=CARTESIAN_POINT('Ctrl Pts',(-2.10208451021625,7.84862588447231,-12.));
#26780=CARTESIAN_POINT('Ctrl Pts',(-2.29939557502752,7.78116612971775,-12.));
#26781=CARTESIAN_POINT('Ctrl Pts',(-2.4936542542127,7.70609002726533,-12.));
#26782=CARTESIAN_POINT('Ctrl Pts',(-2.68449722358562,7.62371149342739,-12.));
#26783=CARTESIAN_POINT('Ctrl Pts',(-2.87766974795956,7.54032739293898,-12.));
#26784=CARTESIAN_POINT('Ctrl Pts',(-3.06734326841189,7.44946115095014,-12.));
#26785=CARTESIAN_POINT('Ctrl Pts',(-3.25311885301286,7.35138992456979,-12.));
#26786=CARTESIAN_POINT('Ctrl Pts',(-3.43857588505528,7.2534868625914,-12.));
#26787=CARTESIAN_POINT('Ctrl Pts',(-3.62014888774859,7.14840306152861,-12.));
#26788=CARTESIAN_POINT('Ctrl Pts',(-3.79741044020532,7.03637241540061,-12.));
#26789=CARTESIAN_POINT('Ctrl Pts',(-3.97212170749682,6.92595356884738,-12.));
#26790=CARTESIAN_POINT('Ctrl Pts',(-4.14264512962284,6.80878585135145,-12.));
#26791=CARTESIAN_POINT('Ctrl Pts',(-4.30853456284606,6.68505947482801,-12.));
#26792=CARTESIAN_POINT('Ctrl Pts',(-4.45106252196752,6.5787569358854,-12.));
#26793=CARTESIAN_POINT('Ctrl Pts',(-4.59016935759093,6.46761224569854,-12.));
#26794=CARTESIAN_POINT('Ctrl Pts',(-4.72554610341853,6.35172956523783,-12.));
#26795=CARTESIAN_POINT('Ctrl Pts',(-4.74477333857637,6.335271025521,-12.));
#26796=CARTESIAN_POINT('Ctrl Pts',(-4.76392528750574,6.31871688954409,-12.));
#26797=CARTESIAN_POINT('Ctrl Pts',(-4.78300102096013,6.30206743426034,-12.));
#26798=CARTESIAN_POINT('Ctrl Pts',(-4.80076087470544,6.28656648948747,-12.));
#26799=CARTESIAN_POINT('Ctrl Pts',(-4.81844738080901,6.27098927612685,-12.));
#26800=CARTESIAN_POINT('Ctrl Pts',(-4.83605920704347,6.25533688403005,-12.));
#26801=CARTESIAN_POINT('Ctrl Pts',(-4.98998560019154,6.11853583753291,-12.));
#26802=CARTESIAN_POINT('Ctrl Pts',(-5.13823022853012,5.97597793328466,-12.));
#26803=CARTESIAN_POINT('Ctrl Pts',(-5.28041162847577,5.82790909191958,-12.));
#26804=CARTESIAN_POINT('Ctrl Pts',(-5.3200731840196,5.78660523235457,-12.));
#26805=CARTESIAN_POINT('Ctrl Pts',(-5.35926272427924,5.7448723237564,-12.));
#26806=CARTESIAN_POINT('Ctrl Pts',(-5.39797144463395,5.70271520266639,-12.));
#26807=CARTESIAN_POINT('Ctrl Pts',(-5.53713035840687,5.55115919345398,-12.));
#26808=CARTESIAN_POINT('Ctrl Pts',(-5.67007843949,5.39412278717484,-12.));
#26809=CARTESIAN_POINT('Ctrl Pts',(-5.79659171905523,5.23204541990698,-12.));
#26810=CARTESIAN_POINT('Ctrl Pts',(-5.92308395045967,5.06999501763838,-12.));
#26811=CARTESIAN_POINT('Ctrl Pts',(-6.04314381583919,4.90290466648765,-12.));
#26812=CARTESIAN_POINT('Ctrl Pts',(-6.156500947101,4.73119033966662,-12.));
#26813=CARTESIAN_POINT('Ctrl Pts',(-6.26858470722818,4.56140492604889,-12.));
#26814=CARTESIAN_POINT('Ctrl Pts',(-6.37411567091608,4.38709818520557,-12.));
#26815=CARTESIAN_POINT('Ctrl Pts',(-6.47278349120591,4.2086593522812,-12.));
#26816=CARTESIAN_POINT('Ctrl Pts',(-6.51321507587661,4.13553961820042,-12.));
#26817=CARTESIAN_POINT('Ctrl Pts',(-6.55249364177314,4.06172594602181,-12.));
#26818=CARTESIAN_POINT('Ctrl Pts',(-6.59059529994264,3.98724486729933,-12.));
#26819=CARTESIAN_POINT('Ctrl Pts',(-6.60144172394684,3.96604228980204,-12.));
#26820=CARTESIAN_POINT('Ctrl Pts',(-6.61219276497738,3.94478562717274,-12.));
#26821=CARTESIAN_POINT('Ctrl Pts',(-6.6228478491971,3.92347549122676,-12.));
#26822=CARTESIAN_POINT('Ctrl Pts',(-6.63395017846395,3.90127086655045,-12.));
#26823=CARTESIAN_POINT('Ctrl Pts',(-6.64494485744702,3.87901508051083,-12.));
#26824=CARTESIAN_POINT('Ctrl Pts',(-6.65582886907332,3.85671429052793,-12.));
#26825=CARTESIAN_POINT('Ctrl Pts',(-6.74450049838414,3.67503060159064,-12.));
#26826=CARTESIAN_POINT('Ctrl Pts',(-6.82588701051427,3.49024918380503,-12.));
#26827=CARTESIAN_POINT('Ctrl Pts',(-6.89978215814578,3.30278705893769,-12.));
#26828=CARTESIAN_POINT('Ctrl Pts',(-6.97319794291742,3.11654101365302,-12.));
#26829=CARTESIAN_POINT('Ctrl Pts',(-7.03921944728565,2.92764827330257,-12.));
#26830=CARTESIAN_POINT('Ctrl Pts',(-7.09759598960971,2.73650163274067,-12.));
#26831=CARTESIAN_POINT('Ctrl Pts',(-7.13572390240132,2.61165658108795,-12.));
#26832=CARTESIAN_POINT('Ctrl Pts',(-7.17058956881407,2.48584973535233,-12.));
#26833=CARTESIAN_POINT('Ctrl Pts',(-7.20211123196002,2.35918876245064,-12.));
#26834=CARTESIAN_POINT('Ctrl Pts',(-7.25068389468356,2.16401312439806,-12.));
#26835=CARTESIAN_POINT('Ctrl Pts',(-7.29131871208896,1.96680886809969,-12.));
#26836=CARTESIAN_POINT('Ctrl Pts',(-7.32397220360618,1.76806533469225,-12.));
#26837=CARTESIAN_POINT('Ctrl Pts',(-7.34491006029522,1.64062831564753,-12.));
#26838=CARTESIAN_POINT('Ctrl Pts',(-7.36256531297852,1.51255845860445,-12.));
#26839=CARTESIAN_POINT('Ctrl Pts',(-7.37691540720549,1.38398700277358,-12.));
#26840=CARTESIAN_POINT('Ctrl Pts',(-7.38319357342979,1.32773699084752,-12.));
#26841=CARTESIAN_POINT('Ctrl Pts',(-7.38883900049354,1.27139100187669,-12.));
#26842=CARTESIAN_POINT('Ctrl Pts',(-7.3938492823474,1.21496020175245,-12.));
#26843=CARTESIAN_POINT('Ctrl Pts',(-7.3971413694576,1.17788142751856,-12.));
#26844=CARTESIAN_POINT('Ctrl Pts',(-7.40015928907374,1.14076530742901,-12.));
#26845=CARTESIAN_POINT('Ctrl Pts',(-7.40290212229044,1.10361724454502,-12.));
#26846=CARTESIAN_POINT('Ctrl Pts',(-7.4050102017394,1.07506608530655,-12.));
#26847=CARTESIAN_POINT('Ctrl Pts',(-7.40695526086128,1.04650256796338,-12.));
#26848=CARTESIAN_POINT('Ctrl Pts',(-7.40873654184619,1.01794082405229,-12.));
#26849=CARTESIAN_POINT('Ctrl Pts',(-7.42105643069599,0.820398991336265,
-12.));
#26850=CARTESIAN_POINT('Ctrl Pts',(-7.42556039755354,0.622752454170974,
-12.));
#26851=CARTESIAN_POINT('Ctrl Pts',(-7.42228121331595,0.425466835953437,
-12.));
#26852=CARTESIAN_POINT('Ctrl Pts',(-7.41900759948271,0.228516350068992,
-12.));
#26853=CARTESIAN_POINT('Ctrl Pts',(-7.40797716007023,0.0319248474341827,
-12.));
#26854=CARTESIAN_POINT('Ctrl Pts',(-7.38917084323832,-0.163840412592323,
-12.));
#26855=CARTESIAN_POINT('Ctrl Pts',(-7.37064698047464,-0.356665453403957,
-12.));
#26856=CARTESIAN_POINT('Ctrl Pts',(-7.34457887203224,-0.548689509627672,
-12.));
#26857=CARTESIAN_POINT('Ctrl Pts',(-7.31090041837079,-0.739452309249457,
-12.));
#26858=CARTESIAN_POINT('Ctrl Pts',(-7.27732639532349,-0.929623588948032,
-12.));
#26859=CARTESIAN_POINT('Ctrl Pts',(-7.23618907077922,-1.11854204252748,
-12.));
#26860=CARTESIAN_POINT('Ctrl Pts',(-7.18737683938924,-1.30572860229432,
-12.));
#26861=CARTESIAN_POINT('Ctrl Pts',(-7.16523608895308,-1.39063459382108,
-12.));
#26862=CARTESIAN_POINT('Ctrl Pts',(-7.1415156188337,-1.4751838814727,-12.));
#26863=CARTESIAN_POINT('Ctrl Pts',(-7.11622968390057,-1.55933456460308,
-12.));
#26864=CARTESIAN_POINT('Ctrl Pts',(-7.10233271497777,-1.60558317796809,
-12.));
#26865=CARTESIAN_POINT('Ctrl Pts',(-7.0879631508151,-1.65171049264756,-12.));
#26866=CARTESIAN_POINT('Ctrl Pts',(-7.07312223630299,-1.69771223090791,
-12.));
#26867=CARTESIAN_POINT('Ctrl Pts',(-7.06252436985534,-1.73056197733326,
-12.));
#26868=CARTESIAN_POINT('Ctrl Pts',(-7.05168654666488,-1.76334603356747,
-12.));
#26869=CARTESIAN_POINT('Ctrl Pts',(-7.04061734154373,-1.79603977674457,
-12.));
#26870=CARTESIAN_POINT('Ctrl Pts',(-6.97824817291142,-1.98025188223161,
-12.));
#26871=CARTESIAN_POINT('Ctrl Pts',(-6.9084880736702,-2.16175440112574,-12.));
#26872=CARTESIAN_POINT('Ctrl Pts',(-6.8315746844225,-2.34012772253663,-12.));
#26873=CARTESIAN_POINT('Ctrl Pts',(-6.75497533051359,-2.51777275038292,
-12.));
#26874=CARTESIAN_POINT('Ctrl Pts',(-6.6712805458415,-2.692314665458,-12.));
#26875=CARTESIAN_POINT('Ctrl Pts',(-6.58068264349192,-2.86331016757811,
-12.));
#26876=CARTESIAN_POINT('Ctrl Pts',(-6.51303849165583,-2.99098250224288,
-12.));
#26877=CARTESIAN_POINT('Ctrl Pts',(-6.44154513202555,-3.11667726552047,
-12.));
#26878=CARTESIAN_POINT('Ctrl Pts',(-6.36626922663613,-3.24019647395781,
-12.));
#26879=CARTESIAN_POINT('Ctrl Pts',(-6.35043403970592,-3.26618021663031,
-12.));
#26880=CARTESIAN_POINT('Ctrl Pts',(-6.33443045330557,-3.29206910604144,
-12.));
#26881=CARTESIAN_POINT('Ctrl Pts',(-6.31826810705525,-3.31784702408304,
-12.));
#26882=CARTESIAN_POINT('Ctrl Pts',(-6.21663338877916,-3.47994795901695,
-12.));
#26883=CARTESIAN_POINT('Ctrl Pts',(-6.1086510172057,-3.63778508480432,-12.));
#26884=CARTESIAN_POINT('Ctrl Pts',(-5.99452112277152,-3.79093554557209,
-12.));
#26885=CARTESIAN_POINT('Ctrl Pts',(-5.88191571230597,-3.94204030724072,
-12.));
#26886=CARTESIAN_POINT('Ctrl Pts',(-5.76332545430664,-4.08858323886591,
-12.));
#26887=CARTESIAN_POINT('Ctrl Pts',(-5.63890846824723,-4.23012099994035,
-12.));
#26888=CARTESIAN_POINT('Ctrl Pts',(-5.58859725063955,-4.28735544455003,
-12.));
#26889=CARTESIAN_POINT('Ctrl Pts',(-5.53733289315066,-4.34377097792458,
-12.));
#26890=CARTESIAN_POINT('Ctrl Pts',(-5.48512449108,-4.39933625912037,-12.));
#26891=CARTESIAN_POINT('Ctrl Pts',(-5.42813643108429,-4.45998851915659,
-12.));
#26892=CARTESIAN_POINT('Ctrl Pts',(-5.37002354987675,-4.51962773802353,
-12.));
#26893=CARTESIAN_POINT('Ctrl Pts',(-5.31081700063333,-4.57822770314271,
-12.));
#26894=CARTESIAN_POINT('Origin',(2.22044604925031E-15,-4.16333634234434E-16,
12.));
#26895=CARTESIAN_POINT('',(15.1652636634099,-5.0941581860707,12.));
#26896=CARTESIAN_POINT('',(15.8449177974003,-2.20777027769627,12.));
#26897=CARTESIAN_POINT('Origin',(0.,0.,12.));
#26898=CARTESIAN_POINT('',(15.3516930915734,-2.13904623492406,11.9999999854331));
#26899=CARTESIAN_POINT('',(15.8449177974003,-2.20777027769627,12.));
#26900=CARTESIAN_POINT('',(15.4951571010802,0.387435137602754,11.9999999854331));
#26901=CARTESIAN_POINT('Origin',(2.22044604925031E-15,-4.16333634234434E-16,
12.));
#26902=CARTESIAN_POINT('',(15.9929910697025,0.399882795164268,12.));
#26903=CARTESIAN_POINT('',(15.4951570863814,0.387435139568728,12.));
#26904=CARTESIAN_POINT('',(15.6444542379842,3.34465561770867,12.));
#26905=CARTESIAN_POINT('Origin',(0.,0.,12.));
#26906=CARTESIAN_POINT('',(15.1574696145705,3.24054230899359,11.9999999854331));
#26907=CARTESIAN_POINT('',(15.6444542379842,3.34465561770867,12.));
#26908=CARTESIAN_POINT('',(14.4281741645111,5.66372579240368,11.9999999854331));
#26909=CARTESIAN_POINT('Origin',(2.22044604925031E-15,-4.16333634234434E-16,
12.));
#26910=CARTESIAN_POINT('',(14.8917277215788,5.8456920096609,12.));
#26911=CARTESIAN_POINT('',(14.4281741500264,5.66372578922383,12.));
#26912=CARTESIAN_POINT('',(13.5570386099129,8.4936666837582,12.));
#26913=CARTESIAN_POINT('Origin',(0.,0.,12.));
#26914=CARTESIAN_POINT('',(13.1350316016236,8.22927362513566,11.9999999854331));
#26915=CARTESIAN_POINT('',(13.5570386099129,8.4936666837582,12.));
#26916=CARTESIAN_POINT('',(11.6209404865298,10.2568875289503,11.9999999854331));
#26917=CARTESIAN_POINT('Origin',(2.22044604925031E-15,-4.16333634234434E-16,
12.));
#26918=CARTESIAN_POINT('',(11.9943022317386,10.5864244945667,12.));
#26919=CARTESIAN_POINT('',(11.6209404740062,10.2568875210082,12.));
#26920=CARTESIAN_POINT('',(9.83444404490535,12.6182161945767,12.));
#26921=CARTESIAN_POINT('Origin',(0.,0.,12.));
#26922=CARTESIAN_POINT('',(9.52831492510037,12.2254330909426,11.9999999854331));
#26923=CARTESIAN_POINT('',(9.83444404490536,12.6182161945767,12.));
#26924=CARTESIAN_POINT('',(7.41204987905737,13.6129172539676,11.9999999854331));
#26925=CARTESIAN_POINT('Origin',(2.22044604925031E-15,-4.16333634234434E-16,
12.));
#26926=CARTESIAN_POINT('',(7.65018687570268,14.0502779464422,12.));
#26927=CARTESIAN_POINT('',(7.41204987000543,13.6129172422212,12.));
#26928=CARTESIAN_POINT('',(4.92567038714607,15.2208226072918,12.));
#26929=CARTESIAN_POINT('Origin',(0.,0.,12.));
#26930=CARTESIAN_POINT('',(4.77234284565852,14.7470248978055,11.9999999854331));
#26931=CARTESIAN_POINT('',(4.92567038714608,15.2208226072918,12.));
#26932=CARTESIAN_POINT('',(2.30915666596483,15.3270282528948,11.9999999854331));
#26933=CARTESIAN_POINT('Origin',(2.22044604925031E-15,-4.16333634234434E-16,
12.));
#26934=CARTESIAN_POINT('',(2.38334607772337,15.8194605179587,12.));
#26935=CARTESIAN_POINT('',(2.30915666147631,15.3270282387607,12.));
#26936=CARTESIAN_POINT('',(-0.577211814455682,15.9875731781501,12.));
#26937=CARTESIAN_POINT('Origin',(0.,0.,12.));
#26938=CARTESIAN_POINT('',(-0.559244213248937,15.4899078590853,11.9999999854331));
#26939=CARTESIAN_POINT('',(-0.577211814455683,15.9875731781501,12.));
#26940=CARTESIAN_POINT('',(-3.0722549205659,15.1924734416771,11.9999999854331));
#26941=CARTESIAN_POINT('Origin',(2.22044604925031E-15,-4.16333634234434E-16,
12.));
#26942=CARTESIAN_POINT('',(-3.17096143167129,15.6805826806374,12.));
#26943=CARTESIAN_POINT('',(-3.07225491994961,15.1924734268603,12.));
#26944=CARTESIAN_POINT('',(-6.01047375249498,14.825986472273,12.));
#26945=CARTESIAN_POINT('Origin',(0.,0.,12.));
#26946=CARTESIAN_POINT('',(-5.823378166473,14.3644793258666,11.9999999854331));
#26947=CARTESIAN_POINT('',(-6.01047375249498,14.825986472273,12.));
#26948=CARTESIAN_POINT('',(-8.08310722202279,13.2254821163649,11.9999999854331));
#26949=CARTESIAN_POINT('Origin',(2.22044604925031E-15,-4.16333634234434E-16,
12.));
#26950=CARTESIAN_POINT('',(-8.34280419399984,13.6503951512779,12.));
#26951=CARTESIAN_POINT('',(-8.08310721637601,13.2254821026524,12.));
#26952=CARTESIAN_POINT('',(-10.7187838508382,11.8761669895831,12.));
#26953=CARTESIAN_POINT('Origin',(0.,0.,12.));
#26954=CARTESIAN_POINT('',(-10.3851267689119,11.5064825888119,11.9999999854331));
#26955=CARTESIAN_POINT('',(-10.7187838508382,11.8761669895831,12.));
#26956=CARTESIAN_POINT('',(-12.1190174985463,9.6633024604911,11.9999999854331));
#26957=CARTESIAN_POINT('Origin',(2.22044604925031E-15,-4.16333634234434E-16,
12.));
#26958=CARTESIAN_POINT('',(-12.5083816438555,9.97376850829778,12.));
#26959=CARTESIAN_POINT('',(-12.1190174885501,9.66330244953692,12.));
#26960=CARTESIAN_POINT('',(-14.1342504243686,7.49390649439194,12.));
#26961=CARTESIAN_POINT('Origin',(0.,0.,12.));
#26962=CARTESIAN_POINT('',(-13.6942758148726,7.26063423394962,11.9999999854331));
#26963=CARTESIAN_POINT('',(-14.1342504243686,7.49390649439194,12.));
#26964=CARTESIAN_POINT('',(-14.6931954070957,4.93558591272671,11.9999999854331));
#26965=CARTESIAN_POINT('Origin',(2.22044604925031E-15,-4.16333634234434E-16,
12.));
#26966=CARTESIAN_POINT('',(-15.1652636634099,5.09415818607069,12.));
#26967=CARTESIAN_POINT('',(-14.6931953939558,4.93558590585204,12.));
#26968=CARTESIAN_POINT('',(-15.8449177974003,2.20777027769626,12.));
#26969=CARTESIAN_POINT('Origin',(0.,0.,12.));
#26970=CARTESIAN_POINT('',(-15.3516930915734,2.13904623492405,11.9999999854331));
#26971=CARTESIAN_POINT('',(-15.8449177974003,2.20777027769626,12.));
#26972=CARTESIAN_POINT('',(-15.4951571010802,-0.387435137602753,11.9999999854331));
#26973=CARTESIAN_POINT('Origin',(2.22044604925031E-15,-4.16333634234434E-16,
12.));
#26974=CARTESIAN_POINT('',(-15.9929910697025,-0.399882795164266,12.));
#26975=CARTESIAN_POINT('',(-15.4951570863814,-0.387435139568727,12.));
#26976=CARTESIAN_POINT('',(-15.6444542379842,-3.34465561770867,12.));
#26977=CARTESIAN_POINT('Origin',(0.,0.,12.));
#26978=CARTESIAN_POINT('',(-15.1574696145705,-3.24054230899359,11.9999999854331));
#26979=CARTESIAN_POINT('',(-15.6444542379842,-3.34465561770867,12.));
#26980=CARTESIAN_POINT('',(-14.4281741645111,-5.66372579240368,11.9999999854331));
#26981=CARTESIAN_POINT('Origin',(2.22044604925031E-15,-4.16333634234434E-16,
12.));
#26982=CARTESIAN_POINT('',(-14.8917277215788,-5.8456920096609,12.));
#26983=CARTESIAN_POINT('',(-14.4281741500264,-5.66372578922383,12.));
#26984=CARTESIAN_POINT('',(-13.5570386099129,-8.4936666837582,12.));
#26985=CARTESIAN_POINT('Origin',(0.,0.,12.));
#26986=CARTESIAN_POINT('',(-13.1350316016236,-8.22927362513566,11.9999999854331));
#26987=CARTESIAN_POINT('',(-13.5570386099129,-8.4936666837582,12.));
#26988=CARTESIAN_POINT('',(-11.6209404865298,-10.2568875289503,11.9999999854331));
#26989=CARTESIAN_POINT('Origin',(2.22044604925031E-15,-4.16333634234434E-16,
12.));
#26990=CARTESIAN_POINT('',(-11.9943022317386,-10.5864244945667,12.));
#26991=CARTESIAN_POINT('',(-11.6209404740062,-10.2568875210082,12.));
#26992=CARTESIAN_POINT('',(-9.83444404490535,-12.6182161945767,12.));
#26993=CARTESIAN_POINT('Origin',(0.,0.,12.));
#26994=CARTESIAN_POINT('',(-9.52831492510037,-12.2254330909426,11.9999999854331));
#26995=CARTESIAN_POINT('',(-9.83444404490535,-12.6182161945767,12.));
#26996=CARTESIAN_POINT('',(-7.41204987905737,-13.6129172539676,11.9999999854331));
#26997=CARTESIAN_POINT('Origin',(2.22044604925031E-15,-4.16333634234434E-16,
12.));
#26998=CARTESIAN_POINT('',(-7.65018687570268,-14.0502779464422,12.));
#26999=CARTESIAN_POINT('',(-7.41204987000543,-13.6129172422212,12.));
#27000=CARTESIAN_POINT('',(-4.92567038714607,-15.2208226072918,12.));
#27001=CARTESIAN_POINT('Origin',(0.,0.,12.));
#27002=CARTESIAN_POINT('',(-4.77234284565852,-14.7470248978055,11.9999999854331));
#27003=CARTESIAN_POINT('',(-4.92567038714608,-15.2208226072918,12.));
#27004=CARTESIAN_POINT('',(-2.30915666596483,-15.3270282528948,11.9999999854331));
#27005=CARTESIAN_POINT('Origin',(2.22044604925031E-15,-4.16333634234434E-16,
12.));
#27006=CARTESIAN_POINT('',(-2.38334607772337,-15.8194605179587,12.));
#27007=CARTESIAN_POINT('',(-2.30915666147631,-15.3270282387607,12.));
#27008=CARTESIAN_POINT('',(0.577211814455688,-15.9875731781501,12.));
#27009=CARTESIAN_POINT('Origin',(0.,0.,12.));
#27010=CARTESIAN_POINT('',(0.559244213248943,-15.4899078590853,11.9999999854331));
#27011=CARTESIAN_POINT('',(0.577211814455689,-15.9875731781501,12.));
#27012=CARTESIAN_POINT('',(3.0722549205659,-15.1924734416771,11.9999999854331));
#27013=CARTESIAN_POINT('Origin',(2.22044604925031E-15,-4.16333634234434E-16,
12.));
#27014=CARTESIAN_POINT('',(3.1709614316713,-15.6805826806374,12.));
#27015=CARTESIAN_POINT('',(3.07225491994961,-15.1924734268603,12.));
#27016=CARTESIAN_POINT('',(6.01047375249498,-14.825986472273,12.));
#27017=CARTESIAN_POINT('Origin',(0.,0.,12.));
#27018=CARTESIAN_POINT('',(5.823378166473,-14.3644793258666,11.9999999854331));
#27019=CARTESIAN_POINT('',(6.01047375249497,-14.825986472273,12.));
#27020=CARTESIAN_POINT('',(8.0831072220228,-13.2254821163649,11.9999999854331));
#27021=CARTESIAN_POINT('Origin',(2.22044604925031E-15,-4.16333634234434E-16,
12.));
#27022=CARTESIAN_POINT('',(8.34280419399985,-13.6503951512779,12.));
#27023=CARTESIAN_POINT('',(8.08310721637602,-13.2254821026524,12.));
#27024=CARTESIAN_POINT('',(10.7187838508382,-11.8761669895831,12.));
#27025=CARTESIAN_POINT('Origin',(0.,0.,12.));
#27026=CARTESIAN_POINT('',(10.385126768912,-11.506482588812,11.9999999854331));
#27027=CARTESIAN_POINT('',(10.7187838508382,-11.8761669895831,12.));
#27028=CARTESIAN_POINT('',(12.1190174985463,-9.6633024604911,11.9999999854331));
#27029=CARTESIAN_POINT('Origin',(2.22044604925031E-15,-4.16333634234434E-16,
12.));
#27030=CARTESIAN_POINT('',(12.5083816438555,-9.97376850829778,12.));
#27031=CARTESIAN_POINT('',(12.1190174885501,-9.66330244953692,12.));
#27032=CARTESIAN_POINT('',(14.1342504243686,-7.49390649439194,12.));
#27033=CARTESIAN_POINT('Origin',(0.,0.,12.));
#27034=CARTESIAN_POINT('',(13.6942758148726,-7.26063423394962,11.9999999854331));
#27035=CARTESIAN_POINT('',(14.1342504243686,-7.49390649439194,12.));
#27036=CARTESIAN_POINT('',(14.6931954070957,-4.93558591272672,11.9999999854331));
#27037=CARTESIAN_POINT('Origin',(2.22044604925031E-15,-4.16333634234434E-16,
12.));
#27038=CARTESIAN_POINT('',(14.6931953939558,-4.93558590585205,12.));
#27039=CARTESIAN_POINT('Origin',(0.,-23.1141426487074,8.));
#27040=CARTESIAN_POINT('',(16.9018270974371,-10.6886774987574,8.00000000095189));
#27041=CARTESIAN_POINT('',(16.9029194185226,-10.6907051200357,8.00000000000001));
#27042=CARTESIAN_POINT('',(16.901826662391,-10.6886766938315,8.00000000000001));
#27043=CARTESIAN_POINT('',(15.9309316922789,-12.0882174594936,8.00000000066043));
#27044=CARTESIAN_POINT('Origin',(0.,0.,8.));
#27045=CARTESIAN_POINT('',(15.9332134908661,-12.0885304601968,8.00000000000001));
#27046=CARTESIAN_POINT('',(15.9332134908661,-12.0885304601968,8.00000000000001));
#27047=CARTESIAN_POINT('Origin',(-0.00247907756725008,0.00171979730317018,
8.));
#27048=CARTESIAN_POINT('Origin',(0.,-23.1141426487074,8.));
#27049=CARTESIAN_POINT('',(12.22677921905,-15.8248366763907,8.00000000093426));
#27050=CARTESIAN_POINT('',(12.2271131583396,-15.8271170588848,8.00000001165519));
#27051=CARTESIAN_POINT('',(12.2267790880642,-15.8248357882219,7.99999999999988));
#27052=CARTESIAN_POINT('',(10.8357650986362,-16.8079082773193,8.00000000066548));
#27053=CARTESIAN_POINT('Origin',(0.,0.,8.));
#27054=CARTESIAN_POINT('',(10.8378022221802,-16.8089828313771,8.));
#27055=CARTESIAN_POINT('',(10.8378022221802,-16.8089828313771,8.));
#27056=CARTESIAN_POINT('Origin',(-0.00174136557906213,0.00246397530291764,
8.));
#27057=CARTESIAN_POINT('Origin',(0.,-23.1141426487074,8.));
#27058=CARTESIAN_POINT('',(6.07700129997158,-19.0522870308522,8.00000000093426));
#27059=CARTESIAN_POINT('',(6.07653516349412,-19.0545441034233,8.00000001165519));
#27060=CARTESIAN_POINT('',(6.07700148065507,-19.0522861514548,7.99999999999989));
#27061=CARTESIAN_POINT('',(4.43364529035575,-19.5003173146329,8.00000000066041));
#27062=CARTESIAN_POINT('Origin',(0.,0.,8.));
#27063=CARTESIAN_POINT('',(4.43519205657354,-19.5020237989274,8.00000000000001));
#27064=CARTESIAN_POINT('',(4.43519205657354,-19.5020237989274,8.00000000000001));
#27065=CARTESIAN_POINT('Origin',(-0.000793619201507889,0.00291096152692738,
8.));
#27066=CARTESIAN_POINT('Origin',(0.,-23.1141426487074,8.));
#27067=CARTESIAN_POINT('',(-0.805752662867996,-19.9817503875941,8.00000000093425));
#27068=CARTESIAN_POINT('',(-0.806962652176574,-19.9837119139682,8.00000001165519));
#27069=CARTESIAN_POINT('',(-0.80575219231358,-19.981749623035,7.99999999999988));
#27070=CARTESIAN_POINT('',(-2.50323756031562,-19.8407002812071,8.00000000066041));
#27071=CARTESIAN_POINT('Origin',(0.,0.,8.));
#27072=CARTESIAN_POINT('',(-2.50236772751931,-19.8428328771094,8.));
#27073=CARTESIAN_POINT('',(-2.50236772751931,-19.8428328771094,8.));
#27074=CARTESIAN_POINT('Origin',(0.00024984937073258,0.00300684281118402,
8.00000000000001));
#27075=CARTESIAN_POINT('Origin',(0.,-23.1141426487074,8.));
#27076=CARTESIAN_POINT('',(-7.59132096296416,-18.5011197483583,8.00000000093426));
#27077=CARTESIAN_POINT('',(-7.59312886249445,-18.5025491395115,8.00000001165519));
#27078=CARTESIAN_POINT('',(-7.5913202592824,-18.5011191908384,7.99999999999989));
#27079=CARTESIAN_POINT('',(-9.13819300331897,-17.7880019835195,8.00000000066548));
#27080=CARTESIAN_POINT('Origin',(0.,0.,8.));
#27081=CARTESIAN_POINT('',(-9.13810503265895,-17.790303461288,8.));
#27082=CARTESIAN_POINT('',(-9.13810503265895,-17.790303461288,8.));
#27083=CARTESIAN_POINT('Origin',(0.00126318242769763,0.0027400545031897,
8.));
#27084=CARTESIAN_POINT('Origin',(0.,-23.1141426487074,8.));
#27085=CARTESIAN_POINT('',(-13.4612639189362,-14.7889810200223,8.00000000093431));
#27086=CARTESIAN_POINT('',(-13.4634504416559,-14.7897046298329,8.));
#27087=CARTESIAN_POINT('',(-13.461263067007,-14.7889807367977,8.));
#27088=CARTESIAN_POINT('',(-14.6709475311075,-13.5898081101815,8.00000000066043));
#27089=CARTESIAN_POINT('Origin',(0.,0.,8.));
#27090=CARTESIAN_POINT('',(-14.671652006793,-13.5920008911193,8.00000000000001));
#27091=CARTESIAN_POINT('',(-14.671652006793,-13.5920008911193,8.00000000000001));
#27092=CARTESIAN_POINT('Origin',(0.0021241570201247,0.00214277514138717,
8.));
#27093=CARTESIAN_POINT('Origin',(0.,-23.1141426487074,8.));
#27094=CARTESIAN_POINT('',(-17.7075797791827,-9.29307291856211,8.00000000093427));
#27095=CARTESIAN_POINT('',(-17.7098835054945,-9.29300580029393,8.00000001165519));
#27096=CARTESIAN_POINT('',(-17.7075788817646,-9.293072943795,7.99999999999989));
#27097=CARTESIAN_POINT('',(-18.4341692464304,-7.75248283619897,8.00000000066548));
#27098=CARTESIAN_POINT('Origin',(0.,0.,8.));
#27099=CARTESIAN_POINT('',(-18.4355812183855,-7.75430241691263,8.00000000000001));
#27100=CARTESIAN_POINT('',(-18.4355812183855,-7.75430241691263,8.00000000000001));
#27101=CARTESIAN_POINT('Origin',(0.00272892695798221,0.00128704551039749,
8.));
#27102=CARTESIAN_POINT('Origin',(0.,-23.1141426487074,8.));
#27103=CARTESIAN_POINT('',(-19.8181001820145,-2.67628307199986,8.00000000093425));
#27104=CARTESIAN_POINT('',(-19.8202420208341,-2.67543208062671,8.00000001165519));
#27105=CARTESIAN_POINT('',(-19.8180993473604,-2.67628340264097,7.99999999999988));
#27106=CARTESIAN_POINT('',(-19.9739581027431,-0.980093690383901,8.00000000066039));
#27107=CARTESIAN_POINT('Origin',(0.,0.,8.));
#27108=CARTESIAN_POINT('',(-19.9759072548391,-0.981320629910932,8.));
#27109=CARTESIAN_POINT('',(-19.9759072548391,-0.981320629910932,8.));
#27110=CARTESIAN_POINT('Origin',(0.0030045479955132,0.000276079177594091,
8.));
#27111=CARTESIAN_POINT('Origin',(0.,-23.1141426487074,8.));
#27112=CARTESIAN_POINT('',(-19.5382652188964,4.26330601082053,8.00000000093426));
#27113=CARTESIAN_POINT('',(-19.5399868328426,4.2648382331363,8.00000001165519));
#27114=CARTESIAN_POINT('',(-19.5382645476573,4.26330541464507,7.99999999999988));
#27115=CARTESIAN_POINT('',(-19.1045928215184,5.91050920446365,8.00000000066042));
#27116=CARTESIAN_POINT('Origin',(0.,0.,8.));
#27117=CARTESIAN_POINT('',(-19.1068440633666,5.91002290780806,8.00000000000001));
#27118=CARTESIAN_POINT('',(-19.1068440633666,5.91002290780806,8.00000000000001));
#27119=CARTESIAN_POINT('Origin',(0.00291777623414591,-0.000768186374036639,
8.00000000000001));
#27120=CARTESIAN_POINT('Origin',(0.,-23.1141426487074,8.));
#27121=CARTESIAN_POINT('',(-16.9018271162855,10.6886774690337,8.00000000093431));
#27122=CARTESIAN_POINT('',(-16.9029194185225,10.6907051200357,8.));
#27123=CARTESIAN_POINT('',(-16.9018266894279,10.6886766792289,8.));
#27124=CARTESIAN_POINT('',(-15.9309316922789,12.0882174594936,8.00000000066042));
#27125=CARTESIAN_POINT('Origin',(0.,0.,8.));
#27126=CARTESIAN_POINT('',(-15.9332134908661,12.0885304601968,7.99999999999999));
#27127=CARTESIAN_POINT('',(-15.9332134908661,12.0885304601968,7.99999999999999));
#27128=CARTESIAN_POINT('Origin',(0.00247907756889099,-0.00171979730426486,
8.));
#27129=CARTESIAN_POINT('Origin',(0.,-23.1141426487074,8.));
#27130=CARTESIAN_POINT('',(-12.22677921905,15.8248366763907,8.00000000093427));
#27131=CARTESIAN_POINT('',(-12.2271131583396,15.8271170588848,8.00000001165519));
#27132=CARTESIAN_POINT('',(-12.2267790880642,15.8248357882219,7.99999999999989));
#27133=CARTESIAN_POINT('',(-10.8357650986362,16.8079082773193,8.00000000066548));
#27134=CARTESIAN_POINT('Origin',(0.,0.,8.));
#27135=CARTESIAN_POINT('',(-10.8378022221802,16.8089828313771,8.00000000000001));
#27136=CARTESIAN_POINT('',(-10.8378022221802,16.8089828313771,8.00000000000001));
#27137=CARTESIAN_POINT('Origin',(0.00174136557906213,-0.00246397530291764,
8.00000000000001));
#27138=CARTESIAN_POINT('Origin',(0.,-23.1141426487074,8.));
#27139=CARTESIAN_POINT('',(-6.07700129997157,19.0522870308522,8.00000000093426));
#27140=CARTESIAN_POINT('',(-6.07653516349413,19.0545441034233,8.00000001165519));
#27141=CARTESIAN_POINT('',(-6.07700148065505,19.0522861514548,7.99999999999989));
#27142=CARTESIAN_POINT('',(-4.43364529035575,19.5003173146329,8.00000000066041));
#27143=CARTESIAN_POINT('Origin',(0.,0.,8.));
#27144=CARTESIAN_POINT('',(-4.43519205657354,19.5020237989274,8.00000000000001));
#27145=CARTESIAN_POINT('',(-4.43519205657354,19.5020237989274,8.00000000000001));
#27146=CARTESIAN_POINT('Origin',(0.000793619202019702,-0.00291096152836845,
8.00000000000001));
#27147=CARTESIAN_POINT('Origin',(0.,-23.1141426487074,8.));
#27148=CARTESIAN_POINT('',(0.805752662868007,19.9817503875941,8.00000000093425));
#27149=CARTESIAN_POINT('',(0.806962652176586,19.9837119139682,8.00000001165519));
#27150=CARTESIAN_POINT('',(0.805752192313582,19.981749623035,7.99999999999988));
#27151=CARTESIAN_POINT('',(2.50323756031564,19.8407002812071,8.00000000066041));
#27152=CARTESIAN_POINT('Origin',(0.,0.,8.));
#27153=CARTESIAN_POINT('',(2.50236772751932,19.8428328771094,8.00000000000001));
#27154=CARTESIAN_POINT('',(2.50236772751932,19.8428328771094,8.00000000000001));
#27155=CARTESIAN_POINT('Origin',(-0.00024984937056341,-0.00300684281156149,
8.00000000000001));
#27156=CARTESIAN_POINT('Origin',(0.,-23.1141426487074,8.));
#27157=CARTESIAN_POINT('',(7.59132096296184,18.5011197483593,8.00000000093431));
#27158=CARTESIAN_POINT('',(7.59312813310105,18.5025475539703,8.));
#27159=CARTESIAN_POINT('',(7.59132025928104,18.5011191908401,8.));
#27160=CARTESIAN_POINT('',(9.13819300331897,17.7880019835195,8.00000000066548));
#27161=CARTESIAN_POINT('Origin',(0.,0.,8.));
#27162=CARTESIAN_POINT('',(9.13810503265895,17.790303461288,8.));
#27163=CARTESIAN_POINT('',(9.13810503265895,17.790303461288,8.));
#27164=CARTESIAN_POINT('Origin',(-0.00126318241234658,-0.00274005446868619,
8.));
#27165=CARTESIAN_POINT('Origin',(0.,-23.1141426487074,8.));
#27166=CARTESIAN_POINT('',(13.461263918938,14.7889810200206,8.00000000093427));
#27167=CARTESIAN_POINT('',(13.4634516693485,14.789705870287,8.00000001165519));
#27168=CARTESIAN_POINT('',(13.4612630670076,14.7889807367957,7.99999999999988));
#27169=CARTESIAN_POINT('',(14.6709475311075,13.5898081101815,8.00000000066043));
#27170=CARTESIAN_POINT('Origin',(0.,0.,8.));
#27171=CARTESIAN_POINT('',(14.6716520067931,13.5920008911193,8.00000000000001));
#27172=CARTESIAN_POINT('',(14.6716520067931,13.5920008911193,8.00000000000001));
#27173=CARTESIAN_POINT('Origin',(-0.00212415699918145,-0.00214277512075034,
8.));
#27174=CARTESIAN_POINT('Origin',(0.,-23.1141426487074,8.));
#27175=CARTESIAN_POINT('',(17.7075797791828,9.2930729185621,8.00000000093426));
#27176=CARTESIAN_POINT('',(17.7098835054945,9.29300580029393,8.00000001165519));
#27177=CARTESIAN_POINT('',(17.7075788817646,9.29307294379499,7.99999999999988));
#27178=CARTESIAN_POINT('',(18.4341692464304,7.75248283619896,8.00000000066548));
#27179=CARTESIAN_POINT('Origin',(0.,0.,8.));
#27180=CARTESIAN_POINT('',(18.4355812183855,7.75430241691263,8.00000000000001));
#27181=CARTESIAN_POINT('',(18.4355812183855,7.75430241691263,8.00000000000001));
#27182=CARTESIAN_POINT('Origin',(-0.00272892695798221,-0.00128704551039749,
8.));
#27183=CARTESIAN_POINT('Origin',(0.,-23.1141426487074,8.));
#27184=CARTESIAN_POINT('',(19.8181001866742,2.67628303717104,8.00000000095184));
#27185=CARTESIAN_POINT('',(19.8202402830185,2.67543191952935,8.));
#27186=CARTESIAN_POINT('',(19.8180993360536,2.6762833741219,8.));
#27187=CARTESIAN_POINT('',(19.9739581027431,0.9800936903839,8.00000000066039));
#27188=CARTESIAN_POINT('Origin',(0.,0.,8.));
#27189=CARTESIAN_POINT('',(19.9759072548391,0.981320629910934,8.));
#27190=CARTESIAN_POINT('',(19.9759072548391,0.981320629910934,8.));
#27191=CARTESIAN_POINT('Origin',(-0.00300454799559757,-0.000276079177270461,
8.));
#27192=CARTESIAN_POINT('Origin',(0.,-23.1141426487074,8.));
#27193=CARTESIAN_POINT('',(19.5382652113567,-4.26330604517097,8.00000000095186));
#27194=CARTESIAN_POINT('',(19.5399851447315,-4.26483779015038,8.00000000000001));
#27195=CARTESIAN_POINT('',(19.5382645272615,-4.26330543759598,8.00000000000001));
#27196=CARTESIAN_POINT('',(19.1045928261591,-5.91050918942428,8.00000000066548));
#27197=CARTESIAN_POINT('Origin',(0.,0.,8.));
#27198=CARTESIAN_POINT('',(19.1068440633666,-5.91002290780807,8.00000000000001));
#27199=CARTESIAN_POINT('',(19.1068440633666,-5.91002290780807,8.00000000000001));
#27200=CARTESIAN_POINT('Origin',(-0.0029177762343191,0.000768186373893975,
8.));
#27201=CARTESIAN_POINT('Origin',(0.,0.,10.));
#27202=CARTESIAN_POINT('',(14.8535887419165,9.11368652088976,10.5713323675468));
#27203=CARTESIAN_POINT('Origin',(84.1567763450378,-127.862145793829,15.4574255506428));
#27204=CARTESIAN_POINT('',(16.2804344971325,6.21577136145369,10.5713324655957));
#27205=CARTESIAN_POINT('Origin',(59.1130480768744,-141.197517255051,15.4574255505854));
#27206=CARTESIAN_POINT('',(16.2815542228302,6.21606770943294,10.5701811473657));
#27207=CARTESIAN_POINT('',(16.2815542228691,6.21606770944323,10.5701811473257));
#27208=CARTESIAN_POINT('Ctrl Pts',(18.4341692463042,7.75248283719143,8.0000000013502));
#27209=CARTESIAN_POINT('Ctrl Pts',(18.0976291578699,7.40188904813054,8.44613531208677));
#27210=CARTESIAN_POINT('Ctrl Pts',(17.5769004256285,6.91371871607935,9.11066173754706));
#27211=CARTESIAN_POINT('Ctrl Pts',(16.8162268218363,6.45382336227621,9.98587039279228));
#27212=CARTESIAN_POINT('Ctrl Pts',(16.6537681950271,6.36537822880674,10.169193466808));
#27213=CARTESIAN_POINT('Ctrl Pts',(16.3647226969178,6.23920570500999,10.4842294831125));
#27214=CARTESIAN_POINT('Ctrl Pts',(16.2893139084681,6.2181207143498,10.5621995723545));
#27215=CARTESIAN_POINT('Ctrl Pts',(16.2815542228302,6.21606770943295,10.5701811473657));
#27216=CARTESIAN_POINT('',(14.8546432677704,9.11416913747482,10.5701811473657));
#27217=CARTESIAN_POINT('Ctrl Pts',(14.8546432677704,9.11416913747483,10.5701811473657));
#27218=CARTESIAN_POINT('Ctrl Pts',(14.8597660838235,9.11651393900879,10.5645884462914));
#27219=CARTESIAN_POINT('Ctrl Pts',(14.9084174072453,9.13819358907152,10.5117975421207));
#27220=CARTESIAN_POINT('Ctrl Pts',(15.1198127387954,9.20461324531954,10.2967812590607));
#27221=CARTESIAN_POINT('Ctrl Pts',(15.2446732178268,9.23447867692749,10.1745830867788));
#27222=CARTESIAN_POINT('Ctrl Pts',(15.660664811749,9.3162344169338,9.77607160548408));
#27223=CARTESIAN_POINT('Ctrl Pts',(16.0628737176647,9.3664847623405,9.40557671670551));
#27224=CARTESIAN_POINT('Ctrl Pts',(16.9608851316969,9.36432155355651,8.62456347338103));
#27225=CARTESIAN_POINT('Ctrl Pts',(17.3352154811581,9.33918367920404,8.30828898496766));
#27226=CARTESIAN_POINT('Ctrl Pts',(17.7075797799539,9.2930729176553,8.00000000200136));
#27227=CARTESIAN_POINT('',(14.8535890570749,9.11368666787079,10.5713320220547));
#27228=CARTESIAN_POINT('Origin',(0.,0.,10.));
#27229=CARTESIAN_POINT('',(10.8407433628677,13.644290522247,10.5713323675468));
#27230=CARTESIAN_POINT('Origin',(122.81293115029,-91.3678021723692,15.4574255506302));
#27231=CARTESIAN_POINT('',(13.1726851506206,11.4091510222243,10.5713324600808));
#27232=CARTESIAN_POINT('Origin',(103.840490158678,-112.464411861885,15.4574255506843));
#27233=CARTESIAN_POINT('',(13.1736359892169,11.4098124657167,10.5701811473657));
#27234=CARTESIAN_POINT('',(13.1736359892499,11.4098124657397,10.5701811473257));
#27235=CARTESIAN_POINT('Ctrl Pts',(14.6709475306549,13.5898081110632,8.00000000133987));
#27236=CARTESIAN_POINT('Ctrl Pts',(14.3604369828165,12.8867251148482,8.70558327641035));
#27237=CARTESIAN_POINT('Ctrl Pts',(14.0026935284487,12.3256974886778,9.34347607836948));
#27238=CARTESIAN_POINT('Ctrl Pts',(13.5537520758817,11.7645428250857,10.0506526867367));
#27239=CARTESIAN_POINT('Ctrl Pts',(13.4343328006559,11.6419837068836,10.2211211362091));
#27240=CARTESIAN_POINT('Ctrl Pts',(13.2466269841097,11.4634026012673,10.4799221943139));
#27241=CARTESIAN_POINT('Ctrl Pts',(13.1815445130367,11.415313000214,10.560601969236));
#27242=CARTESIAN_POINT('Ctrl Pts',(13.1736359892169,11.4098124657167,10.5701811473657));
#27243=CARTESIAN_POINT('',(10.8415692284374,13.6451047025743,10.5701811473657));
#27244=CARTESIAN_POINT('Ctrl Pts',(10.8415692284374,13.6451047025743,10.5701811473657));
#27245=CARTESIAN_POINT('Ctrl Pts',(10.8455842606271,13.6490632866647,10.5645840842365));
#27246=CARTESIAN_POINT('Ctrl Pts',(10.883887975225,13.6860750821818,10.5117924805975));
#27247=CARTESIAN_POINT('Ctrl Pts',(11.0598138704061,13.8207873220949,10.29678118048));
#27248=CARTESIAN_POINT('Ctrl Pts',(11.1669292473831,13.8915559581339,10.1745837097664));
#27249=CARTESIAN_POINT('Ctrl Pts',(11.5298621847818,14.110652648375,9.77608272381361));
#27250=CARTESIAN_POINT('Ctrl Pts',(11.8906295678059,14.2954387244256,9.40558508351274));
#27251=CARTESIAN_POINT('Ctrl Pts',(12.7352323400834,14.6005479099196,8.62456348537514));
#27252=CARTESIAN_POINT('Ctrl Pts',(13.0955850513573,14.7049548519353,8.30828904986755));
#27253=CARTESIAN_POINT('Ctrl Pts',(13.4612639199729,14.7889810194323,8.00000000200137));
#27254=CARTESIAN_POINT('',(10.8407436087492,13.6442907681545,10.5713320220547));
#27255=CARTESIAN_POINT('Origin',(0.,0.,10.));
#27256=CARTESIAN_POINT('',(5.52034434192461,16.5291917183393,10.5713323675469));
#27257=CARTESIAN_POINT('Origin',(146.656033934188,-43.8531531648588,15.4574255506454));
#27258=CARTESIAN_POINT('',(8.47611556230388,15.2264186862092,10.5713324655952));
#27259=CARTESIAN_POINT('Origin',(136.043236604389,-70.1664386002706,15.4574255506333));
#27260=CARTESIAN_POINT('',(8.47678283314335,15.2273654477372,10.5701811473657));
#27261=CARTESIAN_POINT('',(8.47678283315298,15.2273654477509,10.5701811473491));
#27262=CARTESIAN_POINT('Ctrl Pts',(9.13819300258433,17.7880019841986,8.0000000013502));
#27263=CARTESIAN_POINT('Ctrl Pts',(9.1057333419349,17.3029234088212,8.44630493034894));
#27264=CARTESIAN_POINT('Ctrl Pts',(9.02059000744949,16.5943080601136,9.11078948273925));
#27265=CARTESIAN_POINT('Ctrl Pts',(8.73353860606274,15.7531796317961,9.98586915522852));
#27266=CARTESIAN_POINT('Ctrl Pts',(8.66593979429594,15.5809995444073,10.1691927873516));
#27267=CARTESIAN_POINT('Ctrl Pts',(8.52562343281535,15.2985565384195,10.4842223372029));
#27268=CARTESIAN_POINT('Ctrl Pts',(8.48141008850886,15.2339297120029,10.5621950204523));
#27269=CARTESIAN_POINT('Ctrl Pts',(8.47678283314336,15.2273654477372,10.5701811473657));
#27270=CARTESIAN_POINT('',(5.52084193563401,16.5302392602455,10.5701811473657));
#27271=CARTESIAN_POINT('Ctrl Pts',(5.52084193563401,16.5302392602455,10.5701811473657));
#27272=CARTESIAN_POINT('Ctrl Pts',(5.52567641619241,16.540418080074,10.5589950747589));
#27273=CARTESIAN_POINT('Ctrl Pts',(5.5781171184741,16.6458555011213,10.4424799720176));
#27274=CARTESIAN_POINT('Ctrl Pts',(5.81421816143414,16.9698353195168,10.0598387239416));
#27275=CARTESIAN_POINT('Ctrl Pts',(5.98506360658063,17.1780723224927,9.80772177835393));
#27276=CARTESIAN_POINT('Ctrl Pts',(6.56710234337044,17.7566384813563,9.06700837109431));
#27277=CARTESIAN_POINT('Ctrl Pts',(7.02051088852432,18.1312684084711,8.55884949994453));
#27278=CARTESIAN_POINT('Ctrl Pts',(7.59132096413546,18.5011197481603,8.00000000200138));
#27279=CARTESIAN_POINT('',(5.52034448887238,16.5291920335133,10.5713320220547));
#27280=CARTESIAN_POINT('Origin',(0.,0.,10.));
#27281=CARTESIAN_POINT('',(-0.465889678260082,17.4204284483111,10.5713323675468));
#27282=CARTESIAN_POINT('Origin',(152.810254612387,8.95083331849518,15.457425550625));
#27283=CARTESIAN_POINT('',(2.757201345432,17.2071555398934,10.571332465597));
#27284=CARTESIAN_POINT('Origin',(151.837160932365,-19.4053572977299,15.4574255506596));
#27285=CARTESIAN_POINT('',(2.75750456340205,17.2082734247813,10.5701811473657));
#27286=CARTESIAN_POINT('',(2.75750456341259,17.2082734248201,10.5701811473257));
#27287=CARTESIAN_POINT('Ctrl Pts',(2.50323755940219,19.8407002815916,8.00000000133983));
#27288=CARTESIAN_POINT('Ctrl Pts',(2.71730857582917,19.1025054196079,8.70559254922064));
#27289=CARTESIAN_POINT('Ctrl Pts',(2.80390036182858,18.4427875325087,9.34347542918631));
#27290=CARTESIAN_POINT('Ctrl Pts',(2.82069736000104,17.7243294684306,10.0506659154585));
#27291=CARTESIAN_POINT('Ctrl Pts',(2.80799094009269,17.5536854982717,10.2211322370019));
#27292=CARTESIAN_POINT('Ctrl Pts',(2.77898047459641,17.2962388867833,10.479925433458));
#27293=CARTESIAN_POINT('Ctrl Pts',(2.76002529911824,17.2175636893543,10.5606090686878));
#27294=CARTESIAN_POINT('Ctrl Pts',(2.75750456340205,17.2082734247813,10.5701811473657));
#27295=CARTESIAN_POINT('',(-0.465780373556083,17.4215830027821,10.5701811473657));
#27296=CARTESIAN_POINT('Ctrl Pts',(-0.465780373556084,17.4215830027821,
10.5701811473657));
#27297=CARTESIAN_POINT('Ctrl Pts',(-0.465251399100026,17.4271731252073,
10.5646071593077));
#27298=CARTESIAN_POINT('Ctrl Pts',(-0.459705523523858,17.4801431215775,
10.5118192507908));
#27299=CARTESIAN_POINT('Ctrl Pts',(-0.411525259581317,17.6964481226821,
10.2967816258166));
#27300=CARTESIAN_POINT('Ctrl Pts',(-0.374958897313839,17.8195161996499,
10.1745804540546));
#27301=CARTESIAN_POINT('Ctrl Pts',(-0.237752210713215,18.2206987157159,
9.77602389544655));
#27302=CARTESIAN_POINT('Ctrl Pts',(-0.0801626929279727,18.5941348378397,
9.40554077366254));
#27303=CARTESIAN_POINT('Ctrl Pts',(0.370700233274875,19.3707182726362,8.62456342312436));
#27304=CARTESIAN_POINT('Ctrl Pts',(0.579637618643333,19.6823290959358,8.30828870776132));
#27305=CARTESIAN_POINT('Ctrl Pts',(0.805752664038896,19.9817503878085,8.00000000200133));
#27306=CARTESIAN_POINT('',(-0.465889647970186,17.4204287947368,10.5713320220547));
#27307=CARTESIAN_POINT('Origin',(0.,0.,10.));
#27308=CARTESIAN_POINT('',(-6.39593052744725,16.2105044092744,10.5713323675468));
#27309=CARTESIAN_POINT('Origin',(140.533303344984,60.6752172033596,15.4574255506187));
#27310=CARTESIAN_POINT('',(-3.29427204554907,17.1124554876038,10.571332460081));
#27311=CARTESIAN_POINT('Origin',(149.317282773282,33.6962964878064,15.4574255506284));
#27312=CARTESIAN_POINT('',(-3.29436945311861,17.1136096597291,10.5701811473657));
#27313=CARTESIAN_POINT('',(-3.29436945312001,17.1136096597458,10.5701811473491));
#27314=CARTESIAN_POINT('Ctrl Pts',(-4.4336452913456,19.5003173146818,8.00000000133982));
#27315=CARTESIAN_POINT('Ctrl Pts',(-3.98000666779979,18.8798574375332,8.70559279101266));
#27316=CARTESIAN_POINT('Ctrl Pts',(-3.67299983374732,18.289541876818,9.34347541242857));
#27317=CARTESIAN_POINT('Ctrl Pts',(-3.41148864538283,17.6201571111346,10.0506658403939));
#27318=CARTESIAN_POINT('Ctrl Pts',(-3.36506521136807,17.4554584510177,10.2211320704509));
#27319=CARTESIAN_POINT('Ctrl Pts',(-3.30427440668142,17.2036153133682,10.4799255162373));
#27320=CARTESIAN_POINT('Ctrl Pts',(-3.29517817846106,17.1232016110272,10.5606092524601));
#27321=CARTESIAN_POINT('Ctrl Pts',(-3.29436945311862,17.1136096597291,10.5701811473657));
#27322=CARTESIAN_POINT('',(-6.39622269550912,16.2116267200016,10.5701811473657));
#27323=CARTESIAN_POINT('Ctrl Pts',(-6.39622269550912,16.2116267200016,10.5701811473657));
#27324=CARTESIAN_POINT('Ctrl Pts',(-6.39764036742581,16.2170714320148,10.5645960857331));
#27325=CARTESIAN_POINT('Ctrl Pts',(-6.41054379697014,16.2687464183021,10.5118064054396));
#27326=CARTESIAN_POINT('Ctrl Pts',(-6.43924755267471,16.4884725819013,10.2967814029678));
#27327=CARTESIAN_POINT('Ctrl Pts',(-6.44697775603165,16.6166234337939,10.1745820042309));
#27328=CARTESIAN_POINT('Ctrl Pts',(-6.45525643928604,17.0405111803984,9.7760521316184));
#27329=CARTESIAN_POINT('Ctrl Pts',(-6.43489762059455,17.4453312682621,9.40556205383272));
#27330=CARTESIAN_POINT('Ctrl Pts',(-6.27683044794119,18.3293083104535,8.62456345283506));
#27331=CARTESIAN_POINT('Ctrl Pts',(-6.18707187916466,18.6935869635504,8.30828887166431));
#27332=CARTESIAN_POINT('Ctrl Pts',(-6.07700129894464,19.0522870314542,8.00000000200134));
#27333=CARTESIAN_POINT('',(-6.39593061746862,16.2105047451678,10.5713320220547));
#27334=CARTESIAN_POINT('Origin',(0.,0.,10.));
#27335=CARTESIAN_POINT('',(-11.554527761143,13.045354296914,10.5713323675469));
#27336=CARTESIAN_POINT('Origin',(111.305961646472,105.081274424751,15.4574255506739));
#27337=CARTESIAN_POINT('',(-8.94840760976408,14.9537407454735,10.5713324655966));
#27338=CARTESIAN_POINT('Origin',(128.787536624443,82.7336796129508,15.4574255506023));
#27339=CARTESIAN_POINT('',(-8.94889389387817,14.9547919997346,10.5701811473657));
#27340=CARTESIAN_POINT('',(-8.94889389389506,14.9547919997711,10.5701811473257));
#27341=CARTESIAN_POINT('Ctrl Pts',(-10.8357650995917,16.8079082770226,8.00000000135021));
#27342=CARTESIAN_POINT('Ctrl Pts',(-10.4319083043907,16.5372606075049,8.44630079324293));
#27343=CARTESIAN_POINT('Ctrl Pts',(-9.86079935971527,16.1092165464162,9.11078637104974));
#27344=CARTESIAN_POINT('Ctrl Pts',(-9.2758843950842,15.4400561032042,9.98586919170886));
#27345=CARTESIAN_POINT('Ctrl Pts',(-9.16057149290411,15.2954237764487,10.1691928081977));
#27346=CARTESIAN_POINT('Ctrl Pts',(-8.98612677762985,15.0326846060299,10.4842225127632));
#27347=CARTESIAN_POINT('Ctrl Pts',(-8.952265038833,14.9620813509935,10.5621951317299));
#27348=CARTESIAN_POINT('Ctrl Pts',(-8.94889389387818,14.9547919997346,10.5701811473657));
#27349=CARTESIAN_POINT('',(-11.5551861621905,13.0463089966602,10.5701811473657));
#27350=CARTESIAN_POINT('Ctrl Pts',(-11.5551861621905,13.0463089966602,10.5701811473657));
#27351=CARTESIAN_POINT('Ctrl Pts',(-11.558387142026,13.0509500533379,10.5645845413472));
#27352=CARTESIAN_POINT('Ctrl Pts',(-11.5881853135902,13.0950987474776,10.5117930110297));
#27353=CARTESIAN_POINT('Ctrl Pts',(-11.6903020291204,13.2917449279464,10.2967811885933));
#27354=CARTESIAN_POINT('Ctrl Pts',(-11.7413951816398,13.4095218883709,10.1745836443185));
#27355=CARTESIAN_POINT('Ctrl Pts',(-11.8941411179178,13.8049878581245,9.77608155874724));
#27356=CARTESIAN_POINT('Ctrl Pts',(-12.0134730293053,14.1923619596404,9.40558420693438));
#27357=CARTESIAN_POINT('Ctrl Pts',(-12.1672829307558,15.0771140530975,8.62456348411121));
#27358=CARTESIAN_POINT('Ctrl Pts',(-12.2075290668195,15.450122309667,8.30828904306058));
#27359=CARTESIAN_POINT('Ctrl Pts',(-12.2267792182909,15.8248366773076,8.00000000200137));
#27360=CARTESIAN_POINT('',(-11.5545279606177,13.0453545817615,10.5713320220547));
#27361=CARTESIAN_POINT('Origin',(0.,0.,10.));
#27362=CARTESIAN_POINT('',(-15.3194784201766,8.30674192742137,10.5713323675468));
#27363=CARTESIAN_POINT('Origin',(68.6534782678162,136.81297911302,15.4574255506294));
#27364=CARTESIAN_POINT('',(-13.5232331517002,10.991384178438,10.5713324655949));
#27365=CARTESIAN_POINT('Origin',(92.7241128561788,121.792159957727,15.4574255506777));
#27366=CARTESIAN_POINT('',(-13.5240496594282,10.9922057153483,10.5701811473657));
#27367=CARTESIAN_POINT('',(-13.5240496594565,10.9922057153769,10.5701811473257));
#27368=CARTESIAN_POINT('Ctrl Pts',(-15.9309316930687,12.0882174588948,8.00000000133986));
#27369=CARTESIAN_POINT('Ctrl Pts',(-15.1846105254595,11.9045133471794,8.70558326806036));
#27370=CARTESIAN_POINT('Ctrl Pts',(-14.5699846733765,11.6496262306723,9.3434760766814));
#27371=CARTESIAN_POINT('Ctrl Pts',(-13.9393973439685,11.3049486899113,10.0506526873813));
#27372=CARTESIAN_POINT('Ctrl Pts',(-13.7979632304026,11.2086258296407,10.2211211399706));
#27373=CARTESIAN_POINT('Ctrl Pts',(-13.5895004003257,11.0547819798244,10.4799221915463));
#27374=CARTESIAN_POINT('Ctrl Pts',(-13.5308399330947,10.9990389370527,10.5606019637361));
#27375=CARTESIAN_POINT('Ctrl Pts',(-13.5240496594282,10.9922057153483,10.5701811473657));
#27376=CARTESIAN_POINT('',(-15.3204236413265,8.30741386530727,10.5701811473657));
#27377=CARTESIAN_POINT('Ctrl Pts',(-15.3204236413265,8.30741386530727,10.5701811473657));
#27378=CARTESIAN_POINT('Ctrl Pts',(-15.3296093183982,8.31394314010386,10.5589938627884));
#27379=CARTESIAN_POINT('Ctrl Pts',(-15.4243397912466,8.38389819046196,10.4424768097922));
#27380=CARTESIAN_POINT('Ctrl Pts',(-15.7023973354593,8.67266944970296,10.059837781778));
#27381=CARTESIAN_POINT('Ctrl Pts',(-15.877803352698,8.87707981846489,9.80772094036177));
#27382=CARTESIAN_POINT('Ctrl Pts',(-16.3465096379412,9.55074263810651,9.06700787399611));
#27383=CARTESIAN_POINT('Ctrl Pts',(-16.6367153184879,10.0623165531715,8.5588483583004));
#27384=CARTESIAN_POINT('Ctrl Pts',(-16.9018271158858,10.688677470155,8.00000000200139));
#27385=CARTESIAN_POINT('',(-15.3194787050451,8.30674212686605,10.5713320220547));
#27386=CARTESIAN_POINT('Origin',(0.,0.,10.));
#27387=CARTESIAN_POINT('',(-17.2366738903149,2.56621388702747,10.5713323675469));
#27388=CARTESIAN_POINT('Origin',(17.7203721943182,152.043019376197,15.4574255505794));
#27389=CARTESIAN_POINT('',(-16.46695719617,5.70330446537958,10.571332460081));
#27390=CARTESIAN_POINT('Origin',(45.476792614545,146.160708349105,15.4574255506031));
#27391=CARTESIAN_POINT('',(-16.4680054423355,5.70379719401241,10.5701811473657));
#27392=CARTESIAN_POINT('',(-16.4680054423506,5.70379719401952,10.5701811473491));
#27393=CARTESIAN_POINT('Ctrl Pts',(-19.1045928220558,5.91050920363085,8.00000000133985));
#27394=CARTESIAN_POINT('Ctrl Pts',(-18.3404453742124,5.99314117727813,8.70558736914872));
#27395=CARTESIAN_POINT('Ctrl Pts',(-17.6757112795656,5.96384825561592,9.34347579792883));
#27396=CARTESIAN_POINT('Ctrl Pts',(-16.965266952437,5.85563210275787,10.0506513818862));
#27397=CARTESIAN_POINT('Ctrl Pts',(-16.7994199777579,5.81349051075214,10.2211182925806));
#27398=CARTESIAN_POINT('Ctrl Pts',(-16.5509086476868,5.74021758827718,10.4799236386272));
#27399=CARTESIAN_POINT('Ctrl Pts',(-16.4767204468357,5.70789456465678,10.5606051118207));
#27400=CARTESIAN_POINT('Ctrl Pts',(-16.4680054423355,5.7037971940124,10.5701811473657));
#27401=CARTESIAN_POINT('',(-17.2377919239465,2.56652201742732,10.5701811473657));
#27402=CARTESIAN_POINT('Ctrl Pts',(-17.2377919239465,2.56652201742732,10.5701811473657));
#27403=CARTESIAN_POINT('Ctrl Pts',(-17.2432165977388,2.56801679306029,10.5645954896389));
#27404=CARTESIAN_POINT('Ctrl Pts',(-17.2944202352089,2.58267975187223,10.5118057138876));
#27405=CARTESIAN_POINT('Ctrl Pts',(-17.499059900203,2.66768441718779,10.2967813913972));
#27406=CARTESIAN_POINT('Ctrl Pts',(-17.6139068024539,2.7250652631623,10.1745820882336));
#27407=CARTESIAN_POINT('Ctrl Pts',(-17.9851423528615,2.92983891430192,9.77605365105219));
#27408=CARTESIAN_POINT('Ctrl Pts',(-18.3255478232859,3.14988018146411,9.40556319816633));
#27409=CARTESIAN_POINT('Ctrl Pts',(-19.0120618406687,3.7287595937826,8.62456345423171));
#27410=CARTESIAN_POINT('Ctrl Pts',(-19.2826571305709,3.98863205185952,8.30828888039902));
#27411=CARTESIAN_POINT('Ctrl Pts',(-19.5382652189043,4.26330601201086,8.00000000200134));
#27412=CARTESIAN_POINT('',(-17.2366742262179,2.5662139770134,10.5713320220547));
#27413=CARTESIAN_POINT('Origin',(0.,0.,10.));
#27414=CARTESIAN_POINT('',(-17.0748721030675,-3.48383742142528,10.5713323675469));
#27415=CARTESIAN_POINT('Origin',(-35.3500722902058,148.93442758746,15.4574255506556));
#27416=CARTESIAN_POINT('',(-17.4245231720677,-0.272677940736843,10.5713324655957));
#27417=CARTESIAN_POINT('Origin',(-7.25569998124663,152.900118213319,15.4574255506581));
#27418=CARTESIAN_POINT('',(-17.4256767270215,-0.272573448002652,10.5701811473657));
#27419=CARTESIAN_POINT('',(-17.4256767270616,-0.272573447999024,10.5701811473257));
#27420=CARTESIAN_POINT('Ctrl Pts',(-19.9739581029631,-0.980093691350214,
8.00000000133979));
#27421=CARTESIAN_POINT('Ctrl Pts',(-19.2841435286873,-0.641084932274938,
8.70560031770914));
#27422=CARTESIAN_POINT('Ctrl Pts',(-18.6494933378834,-0.441236392474984,
9.34347484440447));
#27423=CARTESIAN_POINT('Ctrl Pts',(-17.9448526543321,-0.299930716980267,
10.0506796721615));
#27424=CARTESIAN_POINT('Ctrl Pts',(-17.774596174239,-0.282817401607676,
10.2211444100579));
#27425=CARTESIAN_POINT('Ctrl Pts',(-17.5160325453378,-0.266691128994518,
10.4799280527013));
#27426=CARTESIAN_POINT('Ctrl Pts',(-17.4352576748299,-0.271704780182462,
10.5606149575372));
#27427=CARTESIAN_POINT('Ctrl Pts',(-17.4256767270215,-0.272573448002655,
10.5701811473657));
#27428=CARTESIAN_POINT('',(-17.0760280978245,-3.48393026358523,10.5701811473657));
#27429=CARTESIAN_POINT('Ctrl Pts',(-17.0760280978245,-3.48393026358523,
10.5701811473657));
#27430=CARTESIAN_POINT('Ctrl Pts',(-17.0816242548471,-3.48437996814373,
10.5646080499549));
#27431=CARTESIAN_POINT('Ctrl Pts',(-17.134752365133,-3.48811668217437,10.5118202838587));
#27432=CARTESIAN_POINT('Ctrl Pts',(-17.3561386567893,-3.47822935651112,
10.2967816445881));
#27433=CARTESIAN_POINT('Ctrl Pts',(-17.483686879022,-3.46358907535537,10.1745803305061));
#27434=CARTESIAN_POINT('Ctrl Pts',(-17.9026024617299,-3.39813122398345,
9.77602162422452));
#27435=CARTESIAN_POINT('Ctrl Pts',(-18.2977298390231,-3.3077820989418,9.40553906114762));
#27436=CARTESIAN_POINT('Ctrl Pts',(-19.1408049443345,-2.99862155763995,
8.62456342110259));
#27437=CARTESIAN_POINT('Ctrl Pts',(-19.483963321225,-2.84696895217793,8.30828869477175));
#27438=CARTESIAN_POINT('Ctrl Pts',(-19.818100182429,-2.676283070884,8.00000000200132));
#27439=CARTESIAN_POINT('',(-17.07487244949,-3.48383745175174,10.5713320220547));
#27440=CARTESIAN_POINT('Origin',(0.,0.,10.));
#27441=CARTESIAN_POINT('',(-14.8535887419165,-9.11368652088975,10.5713323675468));
#27442=CARTESIAN_POINT('Origin',(-84.1567763447132,127.862145793152,15.4574255506348));
#27443=CARTESIAN_POINT('',(-16.2804344971332,-6.21577136145381,10.5713324655964));
#27444=CARTESIAN_POINT('Origin',(-59.1130480768611,141.19751725499,15.4574255506146));
#27445=CARTESIAN_POINT('',(-16.2815542228302,-6.21606770943294,10.5701811473657));
#27446=CARTESIAN_POINT('',(-16.2815542228464,-6.21606770943721,10.5701811473491));
#27447=CARTESIAN_POINT('Ctrl Pts',(-18.4341692463042,-7.75248283719144,
8.0000000013502));
#27448=CARTESIAN_POINT('Ctrl Pts',(-18.0976291590699,-7.40188904938079,
8.44613531049589));
#27449=CARTESIAN_POINT('Ctrl Pts',(-17.5769004278482,-6.91371871795296,
9.11066173479789));
#27450=CARTESIAN_POINT('Ctrl Pts',(-16.8162268240735,-6.45382336350305,
9.9858703902644));
#27451=CARTESIAN_POINT('Ctrl Pts',(-16.6537681965835,-6.36537822955351,
10.1691934650876));
#27452=CARTESIAN_POINT('Ctrl Pts',(-16.3647226973184,-6.23920570512901,
10.4842294826958));
#27453=CARTESIAN_POINT('Ctrl Pts',(-16.2893139085124,-6.2181207143615,10.562199572309));
#27454=CARTESIAN_POINT('Ctrl Pts',(-16.2815542228302,-6.21606770943295,
10.5701811473657));
#27455=CARTESIAN_POINT('',(-14.8546432677704,-9.11416913747482,10.5701811473657));
#27456=CARTESIAN_POINT('Ctrl Pts',(-14.8546432677704,-9.11416913747483,
10.5701811473657));
#27457=CARTESIAN_POINT('Ctrl Pts',(-14.8597660838178,-9.11651393900607,
10.5645884462977));
#27458=CARTESIAN_POINT('Ctrl Pts',(-14.9084174072385,-9.13819358906896,
10.5117975421278));
#27459=CARTESIAN_POINT('Ctrl Pts',(-15.1198127387867,-9.20461324531697,
10.2967812590694));
#27460=CARTESIAN_POINT('Ctrl Pts',(-15.2446732178137,-9.23447867692434,
10.1745830867917));
#27461=CARTESIAN_POINT('Ctrl Pts',(-15.6606648117142,-9.31623441692814,
9.77607160551689));
#27462=CARTESIAN_POINT('Ctrl Pts',(-16.0628737176155,-9.36648476233705,
9.40557671674966));
#27463=CARTESIAN_POINT('Ctrl Pts',(-16.9608851316586,-9.36432155355913,
8.62456347341339));
#27464=CARTESIAN_POINT('Ctrl Pts',(-17.3352154811392,-9.33918367920639,
8.30828898498332));
#27465=CARTESIAN_POINT('Ctrl Pts',(-17.7075797799539,-9.2930729176553,8.00000000200136));
#27466=CARTESIAN_POINT('',(-14.8535890570749,-9.11368666787078,10.5713320220547));
#27467=CARTESIAN_POINT('Origin',(0.,0.,10.));
#27468=CARTESIAN_POINT('',(-10.8407433628676,-13.644290522247,10.5713323675469));
#27469=CARTESIAN_POINT('Origin',(-122.812931151392,91.367802173297,15.4574255507475));
#27470=CARTESIAN_POINT('',(-13.1726851506205,-11.4091510222241,10.5713324600806));
#27471=CARTESIAN_POINT('Origin',(-103.840490158285,112.464411861506,15.4574255506242));
#27472=CARTESIAN_POINT('',(-13.1736359892169,-11.4098124657167,10.5701811473657));
#27473=CARTESIAN_POINT('',(-13.1736359892306,-11.4098124657263,10.5701811473491));
#27474=CARTESIAN_POINT('Ctrl Pts',(-14.6709475306549,-13.5898081110632,
8.00000000133986));
#27475=CARTESIAN_POINT('Ctrl Pts',(-14.3604369835261,-12.8867251164551,
8.70558327479781));
#27476=CARTESIAN_POINT('Ctrl Pts',(-14.0026935300856,-12.3256974912484,
9.34347607544347));
#27477=CARTESIAN_POINT('Ctrl Pts',(-13.5537520773979,-11.7645428267245,
10.0506526845183));
#27478=CARTESIAN_POINT('Ctrl Pts',(-13.4343328018142,-11.6419837080455,
10.2211211345728));
#27479=CARTESIAN_POINT('Ctrl Pts',(-13.24662698436,-11.4634026014367,10.4799221940139));
#27480=CARTESIAN_POINT('Ctrl Pts',(-13.18154451303,-11.4153130002093,10.5606019692441));
#27481=CARTESIAN_POINT('Ctrl Pts',(-13.1736359892169,-11.4098124657167,
10.5701811473657));
#27482=CARTESIAN_POINT('',(-10.8415692284374,-13.6451047025743,10.5701811473657));
#27483=CARTESIAN_POINT('Ctrl Pts',(-10.8415692284374,-13.6451047025743,
10.5701811473657));
#27484=CARTESIAN_POINT('Ctrl Pts',(-10.8495944627031,-13.6530171085486,
10.5589937544163));
#27485=CARTESIAN_POINT('Ctrl Pts',(-10.9349367082249,-13.7341609123916,
10.442476527063));
#27486=CARTESIAN_POINT('Ctrl Pts',(-11.2676049195369,-13.9578493996888,
10.0598376976806));
#27487=CARTESIAN_POINT('Ctrl Pts',(-11.4993688063476,-14.0950950751287,
9.8077208654343));
#27488=CARTESIAN_POINT('Ctrl Pts',(-12.2441871286723,-14.4397003276068,
9.06700782909466));
#27489=CARTESIAN_POINT('Ctrl Pts',(-12.7983827738291,-14.6366633254469,
8.55884825596709));
#27490=CARTESIAN_POINT('Ctrl Pts',(-13.461263919971,-14.788981019434,8.00000000200138));
#27491=CARTESIAN_POINT('',(-10.8407436087492,-13.6442907681545,10.5713320220547));
#27492=CARTESIAN_POINT('Origin',(0.,0.,10.));
#27493=CARTESIAN_POINT('',(-5.52034434192461,-16.5291917183394,10.5713323675469));
#27494=CARTESIAN_POINT('Origin',(-146.656033933765,43.8531531647029,15.4574255506582));
#27495=CARTESIAN_POINT('',(-8.47611556230396,-15.2264186862093,10.5713324655953));
#27496=CARTESIAN_POINT('Origin',(-136.043236604895,70.1664386006067,15.4574255506575));
#27497=CARTESIAN_POINT('',(-8.47678283314336,-15.2273654477372,10.5701811473657));
#27498=CARTESIAN_POINT('',(-8.47678283316653,-15.2273654477701,10.5701811473257));
#27499=CARTESIAN_POINT('Ctrl Pts',(-9.13819300258432,-17.7880019841986,
8.0000000013502));
#27500=CARTESIAN_POINT('Ctrl Pts',(-9.10573334157513,-17.3029234034518,
8.44630493528937));
#27501=CARTESIAN_POINT('Ctrl Pts',(-9.02059000590332,-16.5943080511345,
9.11078949135942));
#27502=CARTESIAN_POINT('Ctrl Pts',(-8.73353860313941,-15.7531796242835,
9.98586916321519));
#27503=CARTESIAN_POINT('Ctrl Pts',(-8.66593979204522,-15.5809995394391,
10.1691927927873));
#27504=CARTESIAN_POINT('Ctrl Pts',(-8.52562343208767,-15.2985565373186,
10.4842223385187));
#27505=CARTESIAN_POINT('Ctrl Pts',(-8.48141008842605,-15.2339297118854,
10.5621950205953));
#27506=CARTESIAN_POINT('Ctrl Pts',(-8.47678283314335,-15.2273654477372,
10.5701811473657));
#27507=CARTESIAN_POINT('',(-5.52084193563401,-16.5302392602455,10.5701811473657));
#27508=CARTESIAN_POINT('Ctrl Pts',(-5.52084193563401,-16.5302392602455,
10.5701811473657));
#27509=CARTESIAN_POINT('Ctrl Pts',(-5.5232591818717,-16.535328682705,10.5645880972756));
#27510=CARTESIAN_POINT('Ctrl Pts',(-5.54659294916294,-16.5832087508318,
10.5117971371651));
#27511=CARTESIAN_POINT('Ctrl Pts',(-5.66583723437205,-16.7699711064541,
10.2967812527268));
#27512=CARTESIAN_POINT('Ctrl Pts',(-5.74228875577475,-16.8731080724369,
10.1745831365675));
#27513=CARTESIAN_POINT('Ctrl Pts',(-6.00840470366951,-17.2031301364064,
9.77607249529175));
#27514=CARTESIAN_POINT('Ctrl Pts',(-6.28421432461988,-17.5001592694047,
9.40557738653905));
#27515=CARTESIAN_POINT('Ctrl Pts',(-6.97352197177043,-18.075733287063,8.62456347451042));
#27516=CARTESIAN_POINT('Ctrl Pts',(-7.27643393079308,-18.2970914797066,
8.30828899024054));
#27517=CARTESIAN_POINT('Ctrl Pts',(-7.59132096413778,-18.5011197481594,
8.00000000200135));
#27518=CARTESIAN_POINT('',(-5.52034448887238,-16.5291920335133,10.5713320220547));
#27519=CARTESIAN_POINT('Origin',(0.,0.,10.));
#27520=CARTESIAN_POINT('',(0.465889678260092,-17.4204284483111,10.5713323675468));
#27521=CARTESIAN_POINT('Origin',(-152.810254612452,-8.95083331846698,15.4574255505984));
#27522=CARTESIAN_POINT('',(-2.7572013454317,-17.207155539892,10.5713324655956));
#27523=CARTESIAN_POINT('Origin',(-151.837160932647,19.4053572978174,15.4574255506476));
#27524=CARTESIAN_POINT('',(-2.75750456340204,-17.2082734247813,10.5701811473657));
#27525=CARTESIAN_POINT('',(-2.75750456341258,-17.2082734248201,10.5701811473257));
#27526=CARTESIAN_POINT('Ctrl Pts',(-2.50323755940218,-19.8407002815916,
8.00000000133983));
#27527=CARTESIAN_POINT('Ctrl Pts',(-2.71730857598249,-19.1025054190797,
8.70559254972556));
#27528=CARTESIAN_POINT('Ctrl Pts',(-2.80390036195331,-18.4427875315623,
9.34347543010285));
#27529=CARTESIAN_POINT('Ctrl Pts',(-2.82069735996715,-17.7243294677321,
10.0506659161534));
#27530=CARTESIAN_POINT('Ctrl Pts',(-2.80799094004872,-17.5536854977597,
10.2211322375144));
#27531=CARTESIAN_POINT('Ctrl Pts',(-2.77898047457061,-17.2962388866928,
10.4799254335514));
#27532=CARTESIAN_POINT('Ctrl Pts',(-2.76002529911911,-17.2175636893571,
10.5606090686849));
#27533=CARTESIAN_POINT('Ctrl Pts',(-2.75750456340204,-17.2082734247813,
10.5701811473657));
#27534=CARTESIAN_POINT('',(0.46578037355609,-17.4215830027821,10.5701811473657));
#27535=CARTESIAN_POINT('Ctrl Pts',(0.465780373556093,-17.4215830027821,
10.5701811473657));
#27536=CARTESIAN_POINT('Ctrl Pts',(0.46525139910022,-17.4271731252052,10.5646071593099));
#27537=CARTESIAN_POINT('Ctrl Pts',(0.459705523525212,-17.4801431215649,
10.5118192508034));
#27538=CARTESIAN_POINT('Ctrl Pts',(0.41152525959577,-17.6964481226244,10.2967816258739));
#27539=CARTESIAN_POINT('Ctrl Pts',(0.374958897339234,-17.8195161995657,
10.1745804541382));
#27540=CARTESIAN_POINT('Ctrl Pts',(0.237752210792364,-18.2206987155065,
9.77602389565469));
#27541=CARTESIAN_POINT('Ctrl Pts',(0.0801626930635958,-18.5941348375598,
9.40554077394135));
#27542=CARTESIAN_POINT('Ctrl Pts',(-0.370700233139312,-19.370718272434,
8.6245634233295));
#27543=CARTESIAN_POINT('Ctrl Pts',(-0.579637618570482,-19.6823290958393,
8.30828870786065));
#27544=CARTESIAN_POINT('Ctrl Pts',(-0.805752664038882,-19.9817503878085,
8.00000000200133));
#27545=CARTESIAN_POINT('',(0.46588964797019,-17.4204287947368,10.5713320220547));
#27546=CARTESIAN_POINT('Origin',(0.,0.,10.));
#27547=CARTESIAN_POINT('',(6.39593052744725,-16.2105044092744,10.5713323675468));
#27548=CARTESIAN_POINT('Origin',(-140.533303345581,-60.6752172035179,15.4574255506022));
#27549=CARTESIAN_POINT('',(3.29427204554917,-17.1124554876035,10.5713324600807));
#27550=CARTESIAN_POINT('Origin',(-149.317282773139,-33.6962964878742,15.4574255506621));
#27551=CARTESIAN_POINT('',(3.29436945311861,-17.1136096597291,10.5701811473657));
#27552=CARTESIAN_POINT('',(3.29436945312199,-17.1136096597692,10.5701811473257));
#27553=CARTESIAN_POINT('Ctrl Pts',(4.43364529134561,-19.5003173146818,8.00000000133983));
#27554=CARTESIAN_POINT('Ctrl Pts',(3.98000666786252,-18.8798574376189,8.70559279091519));
#27555=CARTESIAN_POINT('Ctrl Pts',(3.67299983383264,-18.2895418769823,9.34347541225073));
#27556=CARTESIAN_POINT('Ctrl Pts',(3.41148864542289,-17.6201571112643,10.0506658402589));
#27557=CARTESIAN_POINT('Ctrl Pts',(3.36506521139396,-17.4554584511142,10.2211320703513));
#27558=CARTESIAN_POINT('Ctrl Pts',(3.30427440668273,-17.2036153133869,10.4799255162188));
#27559=CARTESIAN_POINT('Ctrl Pts',(3.29517817846112,-17.1232016110275,10.5606092524598));
#27560=CARTESIAN_POINT('Ctrl Pts',(3.29436945311862,-17.1136096597291,10.5701811473657));
#27561=CARTESIAN_POINT('',(6.39622269550912,-16.2116267200016,10.5701811473657));
#27562=CARTESIAN_POINT('Ctrl Pts',(6.39622269550912,-16.2116267200016,10.5701811473657));
#27563=CARTESIAN_POINT('Ctrl Pts',(6.39764036742772,-16.2170714320218,10.5645960857259));
#27564=CARTESIAN_POINT('Ctrl Pts',(6.41054379697892,-16.2687464183396,10.5118064054016));
#27565=CARTESIAN_POINT('Ctrl Pts',(6.43924755269189,-16.4884725820687,10.2967814028056));
#27566=CARTESIAN_POINT('Ctrl Pts',(6.44697775604531,-16.6166234340433,10.1745820039935));
#27567=CARTESIAN_POINT('Ctrl Pts',(6.45525643927773,-17.0405111810353,9.77605213102646));
#27568=CARTESIAN_POINT('Ctrl Pts',(6.43489762050362,-17.4453312691443,9.40556205303796));
#27569=CARTESIAN_POINT('Ctrl Pts',(6.27683044777478,-18.3293083111279,8.6245634522497));
#27570=CARTESIAN_POINT('Ctrl Pts',(6.18707187906349,-18.6935869638801,8.30828887138087));
#27571=CARTESIAN_POINT('Ctrl Pts',(6.07700129894464,-19.0522870314542,8.00000000200134));
#27572=CARTESIAN_POINT('',(6.39593061746862,-16.2105047451678,10.5713320220547));
#27573=CARTESIAN_POINT('Origin',(0.,0.,10.));
#27574=CARTESIAN_POINT('',(11.554527761143,-13.045354296914,10.5713323675468));
#27575=CARTESIAN_POINT('Origin',(-111.305961644556,-105.081274423327,15.4574255506698));
#27576=CARTESIAN_POINT('',(8.94840760976382,-14.953740745473,10.571332465596));
#27577=CARTESIAN_POINT('Origin',(-128.787536624077,-82.7336796127344,15.4574255505594));
#27578=CARTESIAN_POINT('',(8.94889389387819,-14.9547919997346,10.5701811473657));
#27579=CARTESIAN_POINT('',(8.94889389389507,-14.9547919997711,10.5701811473257));
#27580=CARTESIAN_POINT('Ctrl Pts',(10.8357650995917,-16.8079082770226,8.00000000135021));
#27581=CARTESIAN_POINT('Ctrl Pts',(10.4319083085344,-16.5372606102823,8.44630078866327));
#27582=CARTESIAN_POINT('Ctrl Pts',(9.86079936621396,-16.1092165518233,9.11078636305187));
#27583=CARTESIAN_POINT('Ctrl Pts',(9.27588439976794,-15.4400561090421,9.98586918429367));
#27584=CARTESIAN_POINT('Ctrl Pts',(9.16057149585408,-15.2954237805644,10.1691928031512));
#27585=CARTESIAN_POINT('Ctrl Pts',(8.98612677817748,-15.0326846071263,10.4842225115412));
#27586=CARTESIAN_POINT('Ctrl Pts',(8.95226503888915,-14.962081351115,10.5621951315968));
#27587=CARTESIAN_POINT('Ctrl Pts',(8.94889389387818,-14.9547919997346,10.5701811473657));
#27588=CARTESIAN_POINT('',(11.5551861621905,-13.0463089966602,10.5701811473657));
#27589=CARTESIAN_POINT('Ctrl Pts',(11.5551861621905,-13.0463089966602,10.5701811473657));
#27590=CARTESIAN_POINT('Ctrl Pts',(11.5583871420256,-13.0509500533373,10.564584541348));
#27591=CARTESIAN_POINT('Ctrl Pts',(11.5881853135926,-13.0950987474807,10.5117930110258));
#27592=CARTESIAN_POINT('Ctrl Pts',(11.6903020291314,-13.2917449279689,10.2967811885692));
#27593=CARTESIAN_POINT('Ctrl Pts',(11.7413951816546,-13.4095218884055,10.1745836442827));
#27594=CARTESIAN_POINT('Ctrl Pts',(11.8941411179495,-13.8049878582153,9.77608155865787));
#27595=CARTESIAN_POINT('Ctrl Pts',(12.0134730293381,-14.1923619597709,9.40558420681378));
#27596=CARTESIAN_POINT('Ctrl Pts',(12.1672829307671,-15.0771140532029,8.62456348402197));
#27597=CARTESIAN_POINT('Ctrl Pts',(12.2075290668222,-15.4501223097195,8.30828904301733));
#27598=CARTESIAN_POINT('Ctrl Pts',(12.2267792182909,-15.8248366773076,8.00000000200136));
#27599=CARTESIAN_POINT('',(11.5545279606177,-13.0453545817615,10.5713320220547));
#27600=CARTESIAN_POINT('Origin',(0.,0.,10.));
#27601=CARTESIAN_POINT('',(15.3194784201766,-8.30674192742138,10.5713323675468));
#27602=CARTESIAN_POINT('Origin',(-68.6534782675676,-136.812979112652,15.4574255506315));
#27603=CARTESIAN_POINT('',(13.5232331517007,-10.9913841784383,10.5713324655954));
#27604=CARTESIAN_POINT('Origin',(-92.7241128554327,-121.792159957011,15.4574255506737));
#27605=CARTESIAN_POINT('',(13.5240496594282,-10.9922057153483,10.5701811473657));
#27606=CARTESIAN_POINT('',(13.52404965944,-10.9922057153602,10.5701811473491));
#27607=CARTESIAN_POINT('Ctrl Pts',(15.9309316930687,-12.0882174588948,8.00000000133986));
#27608=CARTESIAN_POINT('Ctrl Pts',(15.1846105255028,-11.90451334719,8.70558326801943));
#27609=CARTESIAN_POINT('Ctrl Pts',(14.5699846734489,-11.6496262307027,9.34347607660589));
#27610=CARTESIAN_POINT('Ctrl Pts',(13.9393973440172,-11.304948689943,10.0506526873236));
#27611=CARTESIAN_POINT('Ctrl Pts',(13.7979632304376,-11.2086258296654,10.2211211399278));
#27612=CARTESIAN_POINT('Ctrl Pts',(13.5895004003317,-11.0547819798306,10.4799221915377));
#27613=CARTESIAN_POINT('Ctrl Pts',(13.5308399330952,-10.9990389370533,10.5606019637353));
#27614=CARTESIAN_POINT('Ctrl Pts',(13.5240496594282,-10.9922057153483,10.5701811473657));
#27615=CARTESIAN_POINT('',(15.3204236413265,-8.30741386530727,10.5701811473657));
#27616=CARTESIAN_POINT('Ctrl Pts',(15.3204236413265,-8.30741386530728,10.5701811473657));
#27617=CARTESIAN_POINT('Ctrl Pts',(15.3259880972987,-8.31136913848444,10.5634041670742));
#27618=CARTESIAN_POINT('Ctrl Pts',(15.3542103341916,-8.33285296379557,10.5283572769709));
#27619=CARTESIAN_POINT('Ctrl Pts',(15.4571749141827,-8.42277175408883,10.3949486774381));
#27620=CARTESIAN_POINT('Ctrl Pts',(15.5156233515662,-8.47953131429124,10.3164605964467));
#27621=CARTESIAN_POINT('Ctrl Pts',(15.7507362195951,-8.7230165051001,9.9932461136542));
#27622=CARTESIAN_POINT('Ctrl Pts',(15.9183553520326,-8.93678627005409,9.74293971143246));
#27623=CARTESIAN_POINT('Ctrl Pts',(16.3885040715423,-9.61540679748373,8.99849349761917));
#27624=CARTESIAN_POINT('Ctrl Pts',(16.6709049544784,-10.1431184734786,8.48676446374045));
#27625=CARTESIAN_POINT('Ctrl Pts',(16.9018270970315,-10.6886774998989,8.00000000203882));
#27626=CARTESIAN_POINT('',(15.3194787050451,-8.30674212686605,10.5713320220547));
#27627=CARTESIAN_POINT('Origin',(0.,0.,10.));
#27628=CARTESIAN_POINT('',(17.0748721030675,3.48383742142528,10.5713323675469));
#27629=CARTESIAN_POINT('Origin',(35.3500722903246,-148.93442758794,15.4574255506851));
#27630=CARTESIAN_POINT('',(17.4245231720676,0.272677940736963,10.5713324655955));
#27631=CARTESIAN_POINT('Origin',(7.25569998132668,-152.900118213192,15.4574255506867));
#27632=CARTESIAN_POINT('',(17.4256767270215,0.272573448002653,10.5701811473657));
#27633=CARTESIAN_POINT('',(17.4256767270616,0.272573447999023,10.5701811473257));
#27634=CARTESIAN_POINT('Ctrl Pts',(19.9739581029631,0.980093691350215,8.00000000133979));
#27635=CARTESIAN_POINT('Ctrl Pts',(19.2841435288454,0.641084932352634,8.70560031754744));
#27636=CARTESIAN_POINT('Ctrl Pts',(18.6494933381746,0.441236392566893,9.34347484411127));
#27637=CARTESIAN_POINT('Ctrl Pts',(17.9448526545539,0.299930717008343,10.0506796719394));
#27638=CARTESIAN_POINT('Ctrl Pts',(17.7745961744026,0.282817401622175,10.221144409894));
#27639=CARTESIAN_POINT('Ctrl Pts',(17.5160325453688,0.266691128991328,10.4799280526703));
#27640=CARTESIAN_POINT('Ctrl Pts',(17.4352576748297,0.271704780182212,10.5606149575373));
#27641=CARTESIAN_POINT('Ctrl Pts',(17.4256767270215,0.272573448002658,10.5701811473657));
#27642=CARTESIAN_POINT('',(17.0760280978245,3.48393026358524,10.5701811473657));
#27643=CARTESIAN_POINT('Ctrl Pts',(17.0760280978245,3.48393026358523,10.5701811473657));
#27644=CARTESIAN_POINT('Ctrl Pts',(17.082832989171,3.48447710146804,10.5634042963604));
#27645=CARTESIAN_POINT('Ctrl Pts',(17.118266172143,3.48616508036893,10.5283524025663));
#27646=CARTESIAN_POINT('Ctrl Pts',(17.2549505214738,3.48347943228899,10.3949314562896));
#27647=CARTESIAN_POINT('Ctrl Pts',(17.3362095820895,3.47757286967626,10.3164420312485));
#27648=CARTESIAN_POINT('Ctrl Pts',(17.6728162805958,3.44219121402148,9.99323475872722));
#27649=CARTESIAN_POINT('Ctrl Pts',(17.9386285191952,3.38617468577126,9.74292915184891));
#27650=CARTESIAN_POINT('Ctrl Pts',(18.734981412195,3.16851614964894,8.99849596508342));
#27651=CARTESIAN_POINT('Ctrl Pts',(19.2905272574431,2.94577048137857,8.48676235755947));
#27652=CARTESIAN_POINT('Ctrl Pts',(19.8181001870972,2.67628303603597,8.00000000203872));
#27653=CARTESIAN_POINT('',(17.07487244949,3.48383745175174,10.5713320220547));
#27654=CARTESIAN_POINT('Origin',(0.,0.,10.));
#27655=CARTESIAN_POINT('',(17.2366738903149,-2.5662138870275,10.5713323675469));
#27656=CARTESIAN_POINT('Origin',(-17.7203721942858,-152.043019376379,15.4574255506204));
#27657=CARTESIAN_POINT('',(16.4669571961699,-5.70330446537945,10.5713324600809));
#27658=CARTESIAN_POINT('Origin',(-45.4767926147669,-146.160708349767,15.4574255506576));
#27659=CARTESIAN_POINT('',(16.4680054423355,-5.70379719401242,10.5701811473657));
#27660=CARTESIAN_POINT('',(16.4680054423719,-5.70379719402953,10.5701811473257));
#27661=CARTESIAN_POINT('Ctrl Pts',(19.1045928267004,-5.91050918858286,8.0000000013502));
#27662=CARTESIAN_POINT('Ctrl Pts',(18.6214219412756,-5.96275677323712,8.44614350899531));
#27663=CARTESIAN_POINT('Ctrl Pts',(17.9087334712743,-6.00199692466679,9.11066791005939));
#27664=CARTESIAN_POINT('Ctrl Pts',(17.0304148875782,-5.86534666547789,9.98587033076591));
#27665=CARTESIAN_POINT('Ctrl Pts',(16.8491128872892,-5.82867319603526,10.1691934324495));
#27666=CARTESIAN_POINT('Ctrl Pts',(16.5465893477924,-5.7395321967925,10.4842291374935));
#27667=CARTESIAN_POINT('Ctrl Pts',(16.4752695527236,-5.70721242491232,10.5621993523733));
#27668=CARTESIAN_POINT('Ctrl Pts',(16.4680054423355,-5.70379719401242,10.5701811473657));
#27669=CARTESIAN_POINT('',(17.2377919239465,-2.56652201742733,10.5701811473657));
#27670=CARTESIAN_POINT('Ctrl Pts',(17.2377919239465,-2.56652201742733,10.5701811473657));
#27671=CARTESIAN_POINT('Ctrl Pts',(17.244373526362,-2.56833558618609,10.5634042277214));
#27672=CARTESIAN_POINT('Ctrl Pts',(17.2782442385717,-2.57886982391587,10.5283549849369));
#27673=CARTESIAN_POINT('Ctrl Pts',(17.4057597403456,-2.62814633108562,10.394940581853));
#27674=CARTESIAN_POINT('Ctrl Pts',(17.4800971046558,-2.66149073253721,10.3164518741183));
#27675=CARTESIAN_POINT('Ctrl Pts',(17.7843053281657,-2.80987217796775,9.99324083646631));
#27676=CARTESIAN_POINT('Ctrl Pts',(18.0149289146885,-2.95342222781332,9.74293477054091));
#27677=CARTESIAN_POINT('Ctrl Pts',(18.6888196107373,-3.4303196438136,8.99849465091812));
#27678=CARTESIAN_POINT('Ctrl Pts',(19.1346780195212,-3.8296291338376,8.48676348247822));
#27679=CARTESIAN_POINT('Ctrl Pts',(19.538265211366,-4.26330604638229,8.00000000203877));
#27680=CARTESIAN_POINT('',(17.2366742262179,-2.56621397701342,10.5713320220547));
#27681=CARTESIAN_POINT('Origin',(0.,0.,-10.));
#27682=CARTESIAN_POINT('',(15.8586462619277,-2.10689542799376,-12.));
#27683=CARTESIAN_POINT('',(17.2955741454208,-2.13341885727951,-10.5713324653939));
#27684=CARTESIAN_POINT('Origin',(23.5558393036297,151.248847158071,-15.457425550669));
#27685=CARTESIAN_POINT('',(15.9750644581313,0.856145527351446,-12.));
#27686=CARTESIAN_POINT('Origin',(0.,0.,-12.));
#27687=CARTESIAN_POINT('',(17.3922038024245,1.0952750368686,-10.5713323676496));
#27688=CARTESIAN_POINT('Origin',(-4.76307193196004,152.99805383595,-15.4574255506925));
#27689=CARTESIAN_POINT('',(17.3933450474474,1.09546964341861,-10.5701811473657));
#27690=CARTESIAN_POINT('',(17.3933450474559,1.09546964342005,-10.5701811473572));
#27691=CARTESIAN_POINT('',(19.9892823205607,0.590066302194425,-8.0000000006604));
#27692=CARTESIAN_POINT('Ctrl Pts',(19.9892823208559,0.590066301248343,-8.00000000133981));
#27693=CARTESIAN_POINT('Ctrl Pts',(19.2749998010589,0.873906210786177,-8.70559645872247));
#27694=CARTESIAN_POINT('Ctrl Pts',(18.6266223644309,1.02333760517501,-9.34347512881039));
#27695=CARTESIAN_POINT('Ctrl Pts',(17.9130663535317,1.10892131617197,-10.0506808566673));
#27696=CARTESIAN_POINT('Ctrl Pts',(17.7419904686334,1.11262517441619,-10.2211470622343));
#27697=CARTESIAN_POINT('Ctrl Pts',(17.4829623350634,1.10841935625201,-10.4799267635866));
#27698=CARTESIAN_POINT('Ctrl Pts',(17.4028311940924,1.09708783867808,-10.5606120436833));
#27699=CARTESIAN_POINT('Ctrl Pts',(17.3933450474474,1.09546964341861,-10.5701811473657));
#27700=CARTESIAN_POINT('',(19.966986344762,-1.11312273006808,-8.00000000095182));
#27701=CARTESIAN_POINT('Origin',(0.,0.,-8.));
#27702=CARTESIAN_POINT('',(17.2967344200949,-2.13342074610697,-10.5701811473657));
#27703=CARTESIAN_POINT('Ctrl Pts',(17.2967344200949,-2.13342074610697,-10.5701811473657));
#27704=CARTESIAN_POINT('Ctrl Pts',(17.3035611999971,-2.13343199258597,-10.5634043347187));
#27705=CARTESIAN_POINT('Ctrl Pts',(17.3390189242949,-2.13233598307216,-10.5283509622276));
#27706=CARTESIAN_POINT('Ctrl Pts',(17.4750744944769,-2.11893772957618,-10.3949263636951));
#27707=CARTESIAN_POINT('Ctrl Pts',(17.5556199162956,-2.10667499553378,-10.3164365320466));
#27708=CARTESIAN_POINT('Ctrl Pts',(17.8884105141753,-2.04499610289594,-9.99323129759905));
#27709=CARTESIAN_POINT('Ctrl Pts',(18.1490082042499,-1.96829604022225,-9.74292598155898));
#27710=CARTESIAN_POINT('Ctrl Pts',(18.925825438827,-1.68882439134058,-8.998496694386));
#27711=CARTESIAN_POINT('Ctrl Pts',(19.462184152493,-1.42317193372476,-8.48676171610473));
#27712=CARTESIAN_POINT('Ctrl Pts',(19.9669863450947,-1.11312272890333,-8.00000000203869));
#27713=CARTESIAN_POINT('',(17.2955750463447,-2.1334188914951,-10.5713320279724));
#27714=CARTESIAN_POINT('Origin',(0.,0.,-10.));
#27715=CARTESIAN_POINT('',(15.6228535442421,3.44414238100227,-12.));
#27716=CARTESIAN_POINT('',(16.9821956200472,3.91067679088529,-10.5713324653932));
#27717=CARTESIAN_POINT('Origin',(-29.594904012793,150.183997111332,-15.4574255505978));
#27718=CARTESIAN_POINT('',(14.7188311719128,6.26830746997787,-12.));
#27719=CARTESIAN_POINT('Origin',(0.,0.,-12.));
#27720=CARTESIAN_POINT('',(15.9687194472522,6.97770590713078,-10.5713323676496));
#27721=CARTESIAN_POINT('Origin',(-56.8042398485925,142.14207563998,-15.4574255506378));
#27722=CARTESIAN_POINT('',(15.9697253074185,6.97827910625622,-10.5701811473657));
#27723=CARTESIAN_POINT('',(15.969725307426,6.97827910626046,-10.5701811473572));
#27724=CARTESIAN_POINT('',(18.5819665360208,7.39121813950882,-8.00000000066548));
#27725=CARTESIAN_POINT('Ctrl Pts',(18.5819665366264,7.39121813871246,-8.0000000013502));
#27726=CARTESIAN_POINT('Ctrl Pts',(18.115084008858,7.40484396995126,-8.42878730500133));
#27727=CARTESIAN_POINT('Ctrl Pts',(17.6409432928525,7.38300231236836,-8.87475273362061));
#27728=CARTESIAN_POINT('Ctrl Pts',(16.796836385882,7.26187969081736,-9.69886565230376));
#27729=CARTESIAN_POINT('Ctrl Pts',(16.5173942721915,7.18523112291558,-9.98545215664171));
#27730=CARTESIAN_POINT('Ctrl Pts',(16.2441712341572,7.09655132569949,-10.2713413261852));
#27731=CARTESIAN_POINT('Ctrl Pts',(16.157205635271,7.0645803511292,-10.3638298171814));
#27732=CARTESIAN_POINT('Ctrl Pts',(16.0106083799487,7.00085283491759,-10.5236792308836));
#27733=CARTESIAN_POINT('Ctrl Pts',(15.9750505957941,6.98131421081911,-10.5640861067932));
#27734=CARTESIAN_POINT('Ctrl Pts',(15.9697253074185,6.97827910625623,-10.5701811473657));
#27735=CARTESIAN_POINT('',(19.1435401333719,5.78311828236397,-8.00000000093431));
#27736=CARTESIAN_POINT('Origin',(0.,0.,-8.));
#27737=CARTESIAN_POINT('',(16.9832865676143,3.91107185327861,-10.5701811473657));
#27738=CARTESIAN_POINT('Ctrl Pts',(16.9832865676143,3.91107185327861,-10.5701811473657));
#27739=CARTESIAN_POINT('Ctrl Pts',(16.9938807774509,3.91490807712278,-10.5589962499751));
#27740=CARTESIAN_POINT('Ctrl Pts',(17.1038574353568,3.95700002189838,-10.4424830400739));
#27741=CARTESIAN_POINT('Ctrl Pts',(17.4489770135646,4.16096284457778,-10.0598396416896));
#27742=CARTESIAN_POINT('Ctrl Pts',(17.6726303951008,4.31106257269274,-9.80772259382915));
#27743=CARTESIAN_POINT('Ctrl Pts',(18.3043191739733,4.83496893723644,-9.06700885143705));
#27744=CARTESIAN_POINT('Ctrl Pts',(18.7206809583787,5.25038372694467,-8.55885060615725));
#27745=CARTESIAN_POINT('Ctrl Pts',(19.1435401332864,5.78311828355128,-8.00000000200138));
#27746=CARTESIAN_POINT('',(16.9821964783418,3.91067706686746,-10.5713320279724));
#27747=CARTESIAN_POINT('Origin',(0.,0.,-10.));
#27748=CARTESIAN_POINT('',(13.5027141203588,8.57976578872144,-12.));
#27749=CARTESIAN_POINT('',(14.6205136742489,9.48308710459935,-10.5713324598778));
#27750=CARTESIAN_POINT('Origin',(-79.1760651305894,131.004740533131,-15.4574255506352));
#27751=CARTESIAN_POINT('',(11.6872896195489,10.9244190213593,-12.));
#27752=CARTESIAN_POINT('Origin',(0.,0.,-12.));
#27753=CARTESIAN_POINT('',(12.6191718535419,12.0185224650217,-10.5713323676496));
#27754=CARTESIAN_POINT('Origin',(-101.9939780973,114.141665326891,-15.4574255506697));
#27755=CARTESIAN_POINT('',(12.6199210072709,12.0194051204483,-10.5701811473657));
#27756=CARTESIAN_POINT('',(12.6199210072764,12.0194051204548,-10.5701811473572));
#27757=CARTESIAN_POINT('',(14.9333913461676,13.3008800022332,-8.00000000066548));
#27758=CARTESIAN_POINT('Ctrl Pts',(14.9333913470091,13.300880001692,-8.00000000135021));
#27759=CARTESIAN_POINT('Ctrl Pts',(14.4900047007427,13.1540007731545,-8.42878756921447));
#27760=CARTESIAN_POINT('Ctrl Pts',(14.05192955011,12.9713101258595,-8.87475254749765));
#27761=CARTESIAN_POINT('Ctrl Pts',(13.3001554516508,12.5687901368235,-9.69886534036099));
#27762=CARTESIAN_POINT('Ctrl Pts',(13.0637795260502,12.4011888222765,-9.9854532705251));
#27763=CARTESIAN_POINT('Ctrl Pts',(12.8373640975609,12.2244096937772,-10.2713421856512));
#27764=CARTESIAN_POINT('Ctrl Pts',(12.7665785152972,12.164623380239,-10.3638298315781));
#27765=CARTESIAN_POINT('Ctrl Pts',(12.6506190175245,12.0546010170489,-10.523677911962));
#27766=CARTESIAN_POINT('Ctrl Pts',(12.6238878102618,12.0240794086141,-10.564084976174));
#27767=CARTESIAN_POINT('Ctrl Pts',(12.6199210072709,12.0194051204483,-10.5701811473657));
#27768=CARTESIAN_POINT('',(16.0111004341151,11.9818299434094,-8.00000000095188));
#27769=CARTESIAN_POINT('Origin',(0.,0.,-8.));
#27770=CARTESIAN_POINT('',(14.6214037084642,9.48383146588572,-10.5701811473657));
#27771=CARTESIAN_POINT('Ctrl Pts',(14.6214037084642,9.48383146588573,-10.5701811473657));
#27772=CARTESIAN_POINT('Ctrl Pts',(14.6266406861662,9.48821113033898,-10.563404164166));
#27773=CARTESIAN_POINT('Ctrl Pts',(14.6530901817765,9.51184302828194,-10.5283573867385));
#27774=CARTESIAN_POINT('Ctrl Pts',(14.7486820596608,9.60956316447749,-10.3949490649912));
#27775=CARTESIAN_POINT('Ctrl Pts',(14.8024969463754,9.67073361738553,-10.3164610136522));
#27776=CARTESIAN_POINT('Ctrl Pts',(15.0177813930359,9.93191529884655,-9.99324636281345));
#27777=CARTESIAN_POINT('Ctrl Pts',(15.1681116736084,10.1581772795485,-9.74293994559928));
#27778=CARTESIAN_POINT('Ctrl Pts',(15.5835674700258,10.8715932850833,-8.99849344133071));
#27779=CARTESIAN_POINT('Ctrl Pts',(15.8236941965497,11.4198346996499,-8.48676450976364));
#27780=CARTESIAN_POINT('Ctrl Pts',(16.0111004336212,11.9818299445155,-8.00000000203881));
#27781=CARTESIAN_POINT('',(14.6205143845238,9.48308765551917,-10.5713320279724));
#27782=CARTESIAN_POINT('Origin',(0.,0.,-10.));
#27783=CARTESIAN_POINT('',(9.75394809472371,12.6805428184636,-12.));
#27784=CARTESIAN_POINT('',(10.4953820000271,13.9116971543318,-10.5713324653938));
#27785=CARTESIAN_POINT('Origin',(-119.207424280339,96.024378823486,-15.4574255505985));
#27786=CARTESIAN_POINT('',(7.24608845304286,14.2628844115113,-12.));
#27787=CARTESIAN_POINT('Origin',(0.,0.,-12.));
#27788=CARTESIAN_POINT('',(7.74756589515309,15.6097278391302,-10.5713323676496));
#27789=CARTESIAN_POINT('Origin',(-134.881737317318,72.3740856247486,-15.4574255506614));
#27790=CARTESIAN_POINT('',(7.74796798344852,15.610813489587,-10.5701811473657));
#27791=CARTESIAN_POINT('',(7.74796798345149,15.610813489595,-10.5701811473572));
#27792=CARTESIAN_POINT('',(9.48362876657315,17.6062594366159,-8.00000000066547));
#27793=CARTESIAN_POINT('Ctrl Pts',(9.48362876754896,17.6062594363951,-8.0000000013502));
#27794=CARTESIAN_POINT('Ctrl Pts',(9.10230391485961,17.3048011250946,-8.44623968757263));
#27795=CARTESIAN_POINT('Ctrl Pts',(8.56651432227087,16.8332645253691,-9.1107403480541));
#27796=CARTESIAN_POINT('Ctrl Pts',(8.0358763831978,16.1202369320469,-9.98586963003723));
#27797=CARTESIAN_POINT('Ctrl Pts',(7.93226696459376,15.9670031889161,-10.1691930478072));
#27798=CARTESIAN_POINT('Ctrl Pts',(7.77897326462272,15.6913850801188,-10.4842250863003));
#27799=CARTESIAN_POINT('Ctrl Pts',(7.75075624770121,15.6183433206485,-10.5621967716335));
#27800=CARTESIAN_POINT('Ctrl Pts',(7.74796798344853,15.610813489587,-10.5701811473657));
#27801=CARTESIAN_POINT('',(10.9474857635323,16.7353560273778,-8.00000000093431));
#27802=CARTESIAN_POINT('Origin',(0.,0.,-8.));
#27803=CARTESIAN_POINT('',(10.4959637731368,13.9127010372614,-10.5701811473657));
#27804=CARTESIAN_POINT('Ctrl Pts',(10.4959637731368,13.9127010372614,-10.5701811473657));
#27805=CARTESIAN_POINT('Ctrl Pts',(10.5016144966778,13.9224512473345,-10.5589943393125));
#27806=CARTESIAN_POINT('Ctrl Pts',(10.5588056026778,14.0253908150085,-10.4424780527323));
#27807=CARTESIAN_POINT('Ctrl Pts',(10.6920761194039,14.4034708467085,-10.0598381515106));
#27808=CARTESIAN_POINT('Ctrl Pts',(10.7669214225258,14.6622159512276,-9.80772126903106));
#27809=CARTESIAN_POINT('Ctrl Pts',(10.9140625720399,15.4695925301061,-9.06700806847332));
#27810=CARTESIAN_POINT('Ctrl Pts',(10.9659919501974,16.0554512351927,-8.55884880660357));
#27811=CARTESIAN_POINT('Ctrl Pts',(10.9474857627036,16.7353560282324,-8.0000000020014));
#27812=CARTESIAN_POINT('',(10.4953824801207,13.9116979174471,-10.5713320279724));
#27813=CARTESIAN_POINT('Origin',(0.,0.,-10.));
#27814=CARTESIAN_POINT('',(4.82871197592245,15.2518592394185,-12.));
#27815=CARTESIAN_POINT('',(5.10435236312686,16.6623512144409,-10.5713324653938));
#27816=CARTESIAN_POINT('Origin',(-144.86060874693,49.4620598581121,-15.4574255506524));
#27817=CARTESIAN_POINT('',(1.93090207822382,15.8810354438797,-12.));
#27818=CARTESIAN_POINT('Origin',(0.,0.,-12.));
#27819=CARTESIAN_POINT('',(1.94148914791391,17.3181696607923,-10.5713323676496));
#27820=CARTESIAN_POINT('Origin',(-151.50076837451,21.8771230683502,-15.4574255506003));
#27821=CARTESIAN_POINT('',(1.94149567299321,17.3193273608118,-10.5701811473657));
#27822=CARTESIAN_POINT('',(1.94149567299326,17.3193273608203,-10.5701811473572));
#27823=CARTESIAN_POINT('',(2.89000059425646,19.7880641422247,-8.00000000066547));
#27824=CARTESIAN_POINT('Ctrl Pts',(2.89000059524891,19.788064142351,-8.00000000135018));
#27825=CARTESIAN_POINT('Ctrl Pts',(2.64475964931276,19.39054597626,-8.42878617646645));
#27826=CARTESIAN_POINT('Ctrl Pts',(2.42659969707148,18.9690059600901,-8.87475353017283));
#27827=CARTESIAN_POINT('Ctrl Pts',(2.10944806509491,18.1774498969438,-9.69884249196947));
#27828=CARTESIAN_POINT('Ctrl Pts',(2.03610698480492,17.8971303337412,-9.98542034745814));
#27829=CARTESIAN_POINT('Ctrl Pts',(1.97628997602387,17.6161445060139,-10.2713376725187));
#27830=CARTESIAN_POINT('Ctrl Pts',(1.96049432139808,17.5248410224956,-10.3638297783296));
#27831=CARTESIAN_POINT('Ctrl Pts',(1.94238591343305,17.3660145389221,-10.5236848708594));
#27832=CARTESIAN_POINT('Ctrl Pts',(1.94152981246431,17.3254518932292,-10.5640909344681));
#27833=CARTESIAN_POINT('Ctrl Pts',(1.94149567299321,17.3193273608118,-10.5701811473657));
#27834=CARTESIAN_POINT('',(4.56344268684126,19.4703512230268,-8.00000000095185));
#27835=CARTESIAN_POINT('Origin',(0.,0.,-8.));
#27836=CARTESIAN_POINT('',(5.10455570284158,16.6634935339443,-10.5701811473657));
#27837=CARTESIAN_POINT('Ctrl Pts',(5.10455570284159,16.6634935339443,-10.5701811473657));
#27838=CARTESIAN_POINT('Ctrl Pts',(5.10575225003943,16.670214723682,-10.5634042571891));
#27839=CARTESIAN_POINT('Ctrl Pts',(5.11082706385406,16.7053218793388,-10.5283538728356));
#27840=CARTESIAN_POINT('Ctrl Pts',(5.12125055225597,16.8416316419825,-10.3949366521605));
#27841=CARTESIAN_POINT('Ctrl Pts',(5.1231583356211,16.923082645346,-10.3164476362452));
#27842=CARTESIAN_POINT('Ctrl Pts',(5.12019877873412,17.2615339859569,-9.99323823168558));
#27843=CARTESIAN_POINT('Ctrl Pts',(5.08991797344972,17.5314913857707,-9.74293234996718));
#27844=CARTESIAN_POINT('Ctrl Pts',(4.94959210998568,18.3450426232497,-8.99849520740764));
#27845=CARTESIAN_POINT('Ctrl Pts',(4.78112411324725,18.9193771867733,-8.48676299740456));
#27846=CARTESIAN_POINT('Ctrl Pts',(4.56344268575195,19.4703512235566,-8.00000000203874));
#27847=CARTESIAN_POINT('',(5.10435255326647,16.6623520957364,-10.5713320279724));
#27848=CARTESIAN_POINT('Origin',(0.,0.,-10.));
#27849=CARTESIAN_POINT('',(-0.678938071373979,15.9835763426303,-12.));
#27850=CARTESIAN_POINT('',(-0.902337501759209,17.4032798105771,-10.5713324598781));
#27851=CARTESIAN_POINT('Origin',(-153.041465883393,-3.06611350821765,-15.4574255506746));
#27852=CARTESIAN_POINT('',(-3.61717958430867,15.5836992225952,-12.));
#27853=CARTESIAN_POINT('Origin',(0.,0.,-12.));
#27854=CARTESIAN_POINT('',(-4.09875984389179,16.9377846323997,-10.5713323676496));
#27855=CARTESIAN_POINT('Origin',(-149.846570852488,-31.2585434020205,-15.4574255506772));
#27856=CARTESIAN_POINT('',(-4.09914966904954,16.9388747462736,-10.5701811473657));
#27857=CARTESIAN_POINT('',(-4.09914966905242,16.9388747462817,-10.5701811473572));
#27858=CARTESIAN_POINT('',(-4.05220430155577,19.5831362715489,-8.00000000066547));
#27859=CARTESIAN_POINT('Ctrl Pts',(-4.05220430066634,19.583136272007,-8.0000000013502));
#27860=CARTESIAN_POINT('Ctrl Pts',(-4.14669632796146,19.125713331242,-8.42878684330689));
#27861=CARTESIAN_POINT('Ctrl Pts',(-4.20752191859742,18.6549819182125,-8.87475305913646));
#27862=CARTESIAN_POINT('Ctrl Pts',(-4.23481731144313,17.80269093116,-9.69884177101634));
#27863=CARTESIAN_POINT('Ctrl Pts',(-4.2078615995899,17.5141886502129,-9.98542319365981));
#27864=CARTESIAN_POINT('Ctrl Pts',(-4.16796931937234,17.2296902080373,-10.2713398280482));
#27865=CARTESIAN_POINT('Ctrl Pts',(-4.15158517621766,17.1384926619022,-10.3638297967784));
#27866=CARTESIAN_POINT('Ctrl Pts',(-4.11428113814177,16.9830542376031,-10.5236815368733));
#27867=CARTESIAN_POINT('Ctrl Pts',(-4.10121326794226,16.9446443015203,-10.5640880820797));
#27868=CARTESIAN_POINT('Ctrl Pts',(-4.09914966904954,16.9388747462736,-10.5701811473657));
#27869=CARTESIAN_POINT('',(-2.37101889769494,19.8569346902003,-8.00000000095185));
#27870=CARTESIAN_POINT('Origin',(0.,0.,-8.));
#27871=CARTESIAN_POINT('',(-0.902537120435117,17.4044227834609,-10.5701811473657));
#27872=CARTESIAN_POINT('Ctrl Pts',(-0.902537120435117,17.4044227834609,
-10.5701811473657));
#27873=CARTESIAN_POINT('Ctrl Pts',(-0.903711515722634,17.4111478767131,
-10.5634042595987));
#27874=CARTESIAN_POINT('Ctrl Pts',(-0.910950040701272,17.445873597137,-10.5283537819086));
#27875=CARTESIAN_POINT('Ctrl Pts',(-0.947775684927258,17.5775281579718,
-10.3949363308107));
#27876=CARTESIAN_POINT('Ctrl Pts',(-0.973840771994048,17.65471959454,-10.3164472895697));
#27877=CARTESIAN_POINT('Ctrl Pts',(-1.0923787754393,17.9717474770875,-9.99323801735438));
#27878=CARTESIAN_POINT('Ctrl Pts',(-1.21316434486273,18.215067793567,-9.74293215129558));
#27879=CARTESIAN_POINT('Ctrl Pts',(-1.62327857933575,18.9315613697452,-8.99849525274451));
#27880=CARTESIAN_POINT('Ctrl Pts',(-1.97802108022651,19.4136399232311,-8.48676295744821));
#27881=CARTESIAN_POINT('Ctrl Pts',(-2.37101889889979,19.8569346903256,-8.00000000203875));
#27882=CARTESIAN_POINT('',(-0.902337623732298,17.403280701153,-10.5713320279724));
#27883=CARTESIAN_POINT('Origin',(0.,0.,-10.));
#27884=CARTESIAN_POINT('',(-6.10469816720394,14.7874382464574,-12.));
#27885=CARTESIAN_POINT('',(-6.80019214539383,16.045116011612,-10.5713324653945));
#27886=CARTESIAN_POINT('Origin',(-142.763263583003,-55.2244683342239,-15.4574255506132));
#27887=CARTESIAN_POINT('',(-8.72897600508841,13.4067388841599,-12.));
#27888=CARTESIAN_POINT('Origin',(0.,0.,-12.));
#27889=CARTESIAN_POINT('',(-9.64463790727134,14.5144528022616,-10.5713323676496));
#27890=CARTESIAN_POINT('Origin',(-130.118665385434,-80.6239682110755,-15.4574255506424));
#27891=CARTESIAN_POINT('',(-9.64537706399891,14.5153438461684,-10.5701811473657));
#27892=CARTESIAN_POINT('',(-9.64537706400437,14.515343846175,-10.5701811473572));
#27893=CARTESIAN_POINT('',(-10.5056535544358,17.0161931502252,-8.00000000066548));
#27894=CARTESIAN_POINT('Ctrl Pts',(-10.5056535537567,17.0161931509599,-8.0000000013502));
#27895=CARTESIAN_POINT('Ctrl Pts',(-10.4379990384668,16.5540372634017,-8.42878754157539));
#27896=CARTESIAN_POINT('Ctrl Pts',(-10.3341548985703,16.090893457156,-8.87475256715481));
#27897=CARTESIAN_POINT('Ctrl Pts',(-10.0682943444031,15.280643580727,-9.69886537601137));
#27898=CARTESIAN_POINT('Ctrl Pts',(-9.94428552962841,15.0187552442567,-9.98545315751203));
#27899=CARTESIAN_POINT('Ctrl Pts',(-9.80950865920445,14.7650822007685,-10.2713420955023));
#27900=CARTESIAN_POINT('Ctrl Pts',(-9.7629223749456,14.6849901507037,-10.3638298300135));
#27901=CARTESIAN_POINT('Ctrl Pts',(-9.6747075515577,14.5516870556448,-10.5236780502563));
#27902=CARTESIAN_POINT('Ctrl Pts',(-9.64929143497656,14.5200619743597,-10.5640850947464));
#27903=CARTESIAN_POINT('Ctrl Pts',(-9.64537706399891,14.5153438461684,-10.5701811473657));
#27904=CARTESIAN_POINT('',(-9.01950057931991,17.8484787924764,-8.00000000093431));
#27905=CARTESIAN_POINT('Origin',(0.,0.,-8.));
#27906=CARTESIAN_POINT('',(-6.80077064695807,16.0461217833684,-10.5701811473657));
#27907=CARTESIAN_POINT('Ctrl Pts',(-6.80077064695807,16.0461217833684,-10.5701811473657));
#27908=CARTESIAN_POINT('Ctrl Pts',(-6.80638919125232,16.055890517594,-10.5589943862035));
#27909=CARTESIAN_POINT('Ctrl Pts',(-6.86694184573586,16.156889202588,-10.4424781739493));
#27910=CARTESIAN_POINT('Ctrl Pts',(-7.12773354662917,16.4613449449585,-10.0598381867424));
#27911=CARTESIAN_POINT('Ctrl Pts',(-7.31439070989755,16.6555354459819,-9.80772129864558));
#27912=CARTESIAN_POINT('Ctrl Pts',(-7.9400287825512,17.1866517200601,-9.06700808049053));
#27913=CARTESIAN_POINT('Ctrl Pts',(-8.42143262084641,17.5245532010067,-8.55884884664401));
#27914=CARTESIAN_POINT('Ctrl Pts',(-9.01950058047432,17.848478792186,-8.00000000200139));
#27915=CARTESIAN_POINT('',(-6.80019256622393,16.0451168089422,-10.5713320279724));
#27916=CARTESIAN_POINT('Origin',(0.,0.,-10.));
#27917=CARTESIAN_POINT('',(-10.7941415683196,11.8077168584163,-12.));
#27918=CARTESIAN_POINT('',(-11.8778432569209,12.7516744235555,-10.5713324653938));
#27919=CARTESIAN_POINT('Origin',(-115.265704733187,-100.721937252455,-15.4574255506293));
#27920=CARTESIAN_POINT('',(-12.787929093689,9.61272797390185,-12.));
#27921=CARTESIAN_POINT('Origin',(0.,0.,-12.));
#27922=CARTESIAN_POINT('',(-14.0272302993381,10.3404637536615,-10.5713323676496));
#27923=CARTESIAN_POINT('Origin',(-94.6965285267638,-120.264952571911,-15.4574255506283));
#27924=CARTESIAN_POINT('',(-14.0282296344253,10.3410482545556,-10.5701811473657));
#27925=CARTESIAN_POINT('',(-14.0282296344327,10.3410482545599,-10.5701811473572));
#27926=CARTESIAN_POINT('',(-15.6919659417353,12.3968460027146,-8.00000000066548));
#27927=CARTESIAN_POINT('Ctrl Pts',(-15.6919659413484,12.3968460036373,-8.0000000013502));
#27928=CARTESIAN_POINT('Ctrl Pts',(-15.4612482665808,11.9688635895045,-8.44634716807826));
#27929=CARTESIAN_POINT('Ctrl Pts',(-15.0899124083607,11.3593769508001,-9.11082129036562));
#27930=CARTESIAN_POINT('Ctrl Pts',(-14.4799190402401,10.7130444208772,-9.98586884763384));
#27931=CARTESIAN_POINT('Ctrl Pts',(-14.347004802687,10.5843997718203,-10.1691926186395));
#27932=CARTESIAN_POINT('Ctrl Pts',(-14.1021964490745,10.3855767651888,-10.4842205569699));
#27933=CARTESIAN_POINT('Ctrl Pts',(-14.0351633980038,10.3451031649441,-10.5621938865181));
#27934=CARTESIAN_POINT('Ctrl Pts',(-14.0282296344253,10.3410482545556,-10.5701811473657));
#27935=CARTESIAN_POINT('',(-14.5800974363697,13.6872329069855,-8.00000000095188));
#27936=CARTESIAN_POINT('Origin',(0.,0.,-8.));
#27937=CARTESIAN_POINT('',(-11.8787308647727,12.7524216806657,-10.5701811473657));
#27938=CARTESIAN_POINT('Ctrl Pts',(-11.8787308647727,12.7524216806657,-10.5701811473657));
#27939=CARTESIAN_POINT('Ctrl Pts',(-11.8839533839592,12.7568185761942,-10.5634041641101));
#27940=CARTESIAN_POINT('Ctrl Pts',(-11.9118191664806,12.7787626049671,-10.5283573896283));
#27941=CARTESIAN_POINT('Ctrl Pts',(-12.0246540683064,12.8559332948898,-10.3949490753317));
#27942=CARTESIAN_POINT('Ctrl Pts',(-12.0942400622391,12.8983084727834,-10.3164610250703));
#27943=CARTESIAN_POINT('Ctrl Pts',(-12.3888375656887,13.0649685394825,-9.99324637132914));
#27944=CARTESIAN_POINT('Ctrl Pts',(-12.6377666955721,13.1737249856624,-9.74293995479456));
#27945=CARTESIAN_POINT('Ctrl Pts',(-13.4124874524261,13.4589856947628,-8.99849344275429));
#27946=CARTESIAN_POINT('Ctrl Pts',(-13.9940974085794,13.6002632407478,-8.4867645122222));
#27947=CARTESIAN_POINT('Ctrl Pts',(-14.5800974373733,13.687232906307,-8.00000000203881));
#27948=CARTESIAN_POINT('',(-11.8778439250753,12.7516750288689,-10.5713320279724));
#27949=CARTESIAN_POINT('Origin',(0.,0.,-10.));
#27950=CARTESIAN_POINT('',(-14.1816521917328,7.40381055390888,-12.));
#27951=CARTESIAN_POINT('',(-15.5228511760091,7.92019270597809,-10.571332459879));
#27952=CARTESIAN_POINT('Origin',(-73.8654007526338,-134.070854041611,-15.4574255505795));
#27953=CARTESIAN_POINT('',(-15.3044692038576,4.65928020123584,-12.));
#27954=CARTESIAN_POINT('Origin',(0.,0.,-12.));
#27955=CARTESIAN_POINT('',(-16.7179316974337,4.91926216737799,-10.5713323676496));
#27956=CARTESIAN_POINT('Origin',(-47.8525927545976,-145.400208728616,-15.4574255506014));
#27957=CARTESIAN_POINT('',(-16.7190706763204,4.91946962582534,-10.5701811473657));
#27958=CARTESIAN_POINT('',(-16.7190706763288,4.91946962582688,-10.5701811473572));
#27959=CARTESIAN_POINT('',(-18.9855956477114,6.28225626930338,-8.00000000066547));
#27960=CARTESIAN_POINT('Ctrl Pts',(-18.9855956476635,6.2822562703027,-8.00000000135019));
#27961=CARTESIAN_POINT('Ctrl Pts',(-18.6367017450793,5.97171227824352,-8.42878687911838));
#27962=CARTESIAN_POINT('Ctrl Pts',(-18.2594491909432,5.68367023000594,-8.87475303340393));
#27963=CARTESIAN_POINT('Ctrl Pts',(-17.5349912283894,5.23388632148025,-9.69884173367996));
#27964=CARTESIAN_POINT('Ctrl Pts',(-17.2716629153967,5.11297935279029,-9.98542334889029));
#27965=CARTESIAN_POINT('Ctrl Pts',(-17.0053339464139,5.00527782996971,-10.2713399444911));
#27966=CARTESIAN_POINT('Ctrl Pts',(-16.9181625924622,4.97386817752492,-10.363829798057));
#27967=CARTESIAN_POINT('Ctrl Pts',(-16.7648971338693,4.92845522395886,-10.5236813571024));
#27968=CARTESIAN_POINT('Ctrl Pts',(-16.7250992094526,4.92056730211027,-10.5640879281721));
#27969=CARTESIAN_POINT('Ctrl Pts',(-16.7190706763204,4.91946962582535,-10.5701811473657));
#27970=CARTESIAN_POINT('',(-18.3821193318641,7.87510474680894,-8.00000000095187));
#27971=CARTESIAN_POINT('Origin',(0.,0.,-8.));
#27972=CARTESIAN_POINT('',(-15.5239408288994,7.92059131757518,-10.5701811473657));
#27973=CARTESIAN_POINT('Ctrl Pts',(-15.5239408288994,7.92059131757521,-10.5701811473657));
#27974=CARTESIAN_POINT('Ctrl Pts',(-15.5303521795289,7.92293682684727,-10.563404205282));
#27975=CARTESIAN_POINT('Ctrl Pts',(-15.5640436349665,7.93402859460558,-10.5283558304942));
#27976=CARTESIAN_POINT('Ctrl Pts',(-15.6964698353132,7.96795801108948,-10.3949435685778));
#27977=CARTESIAN_POINT('Ctrl Pts',(-15.7763523057977,7.98397907252595,-10.3164550925782));
#27978=CARTESIAN_POINT('Ctrl Pts',(-16.1101805969897,8.03983262596674,-9.99324279225774));
#27979=CARTESIAN_POINT('Ctrl Pts',(-16.3812946407727,8.05689058530697,-9.74293659276605));
#27980=CARTESIAN_POINT('Ctrl Pts',(-17.2068565502871,8.05997362328367,-8.99849421884513));
#27981=CARTESIAN_POINT('Ctrl Pts',(-17.8017148435408,7.99380365638828,-8.48676384407007));
#27982=CARTESIAN_POINT('Ctrl Pts',(-18.382119332575,7.87510474582817,-8.00000000203878));
#27983=CARTESIAN_POINT('',(-15.5228520082561,7.92019304563385,-10.5713320279724));
#27984=CARTESIAN_POINT('Origin',(0.,0.,-10.));
#27985=CARTESIAN_POINT('',(-15.8586462619277,2.10689542799376,-12.));
#27986=CARTESIAN_POINT('',(-17.2955741454207,2.1334188572795,-10.5713324653938));
#27987=CARTESIAN_POINT('Origin',(-23.5558393036639,-151.248847157487,-15.4574255507057));
#27988=CARTESIAN_POINT('',(-15.9750644581313,-0.856145527351444,-12.));
#27989=CARTESIAN_POINT('Origin',(0.,0.,-12.));
#27990=CARTESIAN_POINT('',(-17.3922038024244,-1.09527503686864,-10.5713323676496));
#27991=CARTESIAN_POINT('Origin',(4.76307193199126,-152.998053835939,-15.4574255506736));
#27992=CARTESIAN_POINT('',(-17.3933450474474,-1.09546964341861,-10.5701811473657));
#27993=CARTESIAN_POINT('',(-17.3933450474559,-1.09546964342005,-10.5701811473572));
#27994=CARTESIAN_POINT('',(-19.9892823210147,-0.590066286421281,-8.00000000066547));
#27995=CARTESIAN_POINT('Ctrl Pts',(-19.9892823213114,-0.590066285465836,
-8.00000000135018));
#27996=CARTESIAN_POINT('Ctrl Pts',(-19.5552177612373,-0.762553143854976,
-8.42878612191519));
#27997=CARTESIAN_POINT('Ctrl Pts',(-19.1021987068298,-0.904199324209642,
-8.87475356581035));
#27998=CARTESIAN_POINT('Ctrl Pts',(-18.2675953127712,-1.07908057562433,
-9.69884256067525));
#27999=CARTESIAN_POINT('Ctrl Pts',(-17.9787991830665,-1.10263031045676,
-9.9854201300736));
#28000=CARTESIAN_POINT('Ctrl Pts',(-17.6916950067099,-1.11274582052662,
-10.2713374991643));
#28001=CARTESIAN_POINT('Ctrl Pts',(-17.5990355696582,-1.112446815737,-10.363829776856));
#28002=CARTESIAN_POINT('Ctrl Pts',(-17.4394772602174,-1.10270011330808,
-10.5236851384871));
#28003=CARTESIAN_POINT('Ctrl Pts',(-17.3993822358286,-1.09649949779314,
-10.5640911633362));
#28004=CARTESIAN_POINT('Ctrl Pts',(-17.3933450474474,-1.09546964341861,
-10.5701811473657));
#28005=CARTESIAN_POINT('',(-19.966986344762,1.11312273006808,-8.00000000095182));
#28006=CARTESIAN_POINT('Origin',(0.,0.,-8.));
#28007=CARTESIAN_POINT('',(-17.2967344200949,2.13342074610697,-10.5701811473657));
#28008=CARTESIAN_POINT('Ctrl Pts',(-17.2967344200949,2.13342074610697,-10.5701811473657));
#28009=CARTESIAN_POINT('Ctrl Pts',(-17.3035611999969,2.13343199258578,-10.563404334719));
#28010=CARTESIAN_POINT('Ctrl Pts',(-17.3390189242868,2.13233598307222,-10.5283509622356));
#28011=CARTESIAN_POINT('Ctrl Pts',(-17.4750744944391,2.11893772958056,-10.394926363732));
#28012=CARTESIAN_POINT('Ctrl Pts',(-17.5556199162392,2.10667499554252,-10.3164365321016));
#28013=CARTESIAN_POINT('Ctrl Pts',(-17.8884105140494,2.04499610292459,-9.99323129772077));
#28014=CARTESIAN_POINT('Ctrl Pts',(-18.1490082040659,1.96829604027826,-9.74292598173563));
#28015=CARTESIAN_POINT('Ctrl Pts',(-18.9258254386725,1.68882439141746,-8.99849669453326));
#28016=CARTESIAN_POINT('Ctrl Pts',(-19.4621841524218,1.42317193376853,-8.48676171617345));
#28017=CARTESIAN_POINT('Ctrl Pts',(-19.9669863450947,1.11312272890334,-8.00000000203869));
#28018=CARTESIAN_POINT('',(-17.2955750463446,2.1334188914951,-10.5713320279724));
#28019=CARTESIAN_POINT('Origin',(0.,0.,-10.));
#28020=CARTESIAN_POINT('',(-15.6228535442421,-3.44414238100227,-12.));
#28021=CARTESIAN_POINT('',(-16.9821956200471,-3.91067679088527,-10.5713324653932));
#28022=CARTESIAN_POINT('Origin',(29.5949040129132,-150.183997111823,-15.457425550639));
#28023=CARTESIAN_POINT('',(-14.7188311719128,-6.26830746997787,-12.));
#28024=CARTESIAN_POINT('Origin',(0.,0.,-12.));
#28025=CARTESIAN_POINT('',(-15.9687194472521,-6.9777059071309,-10.5713323676496));
#28026=CARTESIAN_POINT('Origin',(56.8042398484162,-142.14207563962,-15.4574255506568));
#28027=CARTESIAN_POINT('',(-15.9697253074185,-6.97827910625622,-10.5701811473657));
#28028=CARTESIAN_POINT('',(-15.969725307426,-6.97827910626046,-10.5701811473572));
#28029=CARTESIAN_POINT('',(-18.5819665360208,-7.39121813950882,-8.00000000066548));
#28030=CARTESIAN_POINT('Ctrl Pts',(-18.5819665366264,-7.39121813871246,
-8.0000000013502));
#28031=CARTESIAN_POINT('Ctrl Pts',(-18.1150840094864,-7.40484396993293,
-8.42878730442417));
#28032=CARTESIAN_POINT('Ctrl Pts',(-17.6409432941562,-7.3830023124265,-8.87475273239537));
#28033=CARTESIAN_POINT('Ctrl Pts',(-16.7968363871264,-7.26187969111102,
-9.69886565104633));
#28034=CARTESIAN_POINT('Ctrl Pts',(-16.5173942730729,-7.18523112316875,
-9.98545215573256));
#28035=CARTESIAN_POINT('Ctrl Pts',(-16.2441712345817,-7.09655132585296,
-10.2713413257348));
#28036=CARTESIAN_POINT('Ctrl Pts',(-16.157205635565,-7.06458035124848,-10.3638298168642));
#28037=CARTESIAN_POINT('Ctrl Pts',(-16.0106083799904,-7.00085283494231,
-10.5236792308355));
#28038=CARTESIAN_POINT('Ctrl Pts',(-15.9750505957893,-6.98131421081621,
-10.5640861067988));
#28039=CARTESIAN_POINT('Ctrl Pts',(-15.9697253074185,-6.97827910625622,
-10.5701811473657));
#28040=CARTESIAN_POINT('',(-19.1435401333719,-5.78311828236397,-8.00000000093431));
#28041=CARTESIAN_POINT('Origin',(0.,0.,-8.));
#28042=CARTESIAN_POINT('',(-16.9832865676143,-3.91107185327861,-10.5701811473657));
#28043=CARTESIAN_POINT('Ctrl Pts',(-16.9832865676143,-3.9110718532786,-10.5701811473657));
#28044=CARTESIAN_POINT('Ctrl Pts',(-16.9938807775104,-3.91490807714427,
-10.5589962499124));
#28045=CARTESIAN_POINT('Ctrl Pts',(-17.1038574351457,-3.95700002184885,
-10.4424830402896));
#28046=CARTESIAN_POINT('Ctrl Pts',(-17.4489770132551,-4.16096284432762,
-10.0598396420491));
#28047=CARTESIAN_POINT('Ctrl Pts',(-17.6726303942686,-4.31106257224221,
-9.8077225947347));
#28048=CARTESIAN_POINT('Ctrl Pts',(-18.304319171989,-4.83496893525044,-9.06700885386361));
#28049=CARTESIAN_POINT('Ctrl Pts',(-18.7206809573621,-5.25038372566414,
-8.55885060750064));
#28050=CARTESIAN_POINT('Ctrl Pts',(-19.1435401332864,-5.78311828355127,
-8.00000000200138));
#28051=CARTESIAN_POINT('',(-16.9821964783418,-3.91067706686746,-10.5713320279724));
#28052=CARTESIAN_POINT('Origin',(0.,0.,-10.));
#28053=CARTESIAN_POINT('',(-13.5027141203588,-8.57976578872145,-12.));
#28054=CARTESIAN_POINT('',(-14.6205136742495,-9.48308710459978,-10.5713324598787));
#28055=CARTESIAN_POINT('Origin',(79.1760651301776,-131.0047405326,-15.4574255506641));
#28056=CARTESIAN_POINT('',(-11.6872896195489,-10.9244190213593,-12.));
#28057=CARTESIAN_POINT('Origin',(0.,0.,-12.));
#28058=CARTESIAN_POINT('',(-12.6191718535418,-12.0185224650217,-10.5713323676496));
#28059=CARTESIAN_POINT('Origin',(101.993978097991,-114.141665327459,-15.4574255506783));
#28060=CARTESIAN_POINT('',(-12.6199210072709,-12.0194051204483,-10.5701811473657));
#28061=CARTESIAN_POINT('',(-12.6199210072764,-12.0194051204548,-10.5701811473572));
#28062=CARTESIAN_POINT('',(-14.9333913461659,-13.3008800022351,-8.00000000066548));
#28063=CARTESIAN_POINT('Ctrl Pts',(-14.9333913470074,-13.3008800016939,
-8.0000000013502));
#28064=CARTESIAN_POINT('Ctrl Pts',(-14.4718373134409,-13.1479825233628,
-8.44635677144831));
#28065=CARTESIAN_POINT('Ctrl Pts',(-13.8071322456388,-12.8881234815153,
-9.11082852198501));
#28066=CARTESIAN_POINT('Ctrl Pts',(-13.0647008722188,-12.3996358745634,
-9.9858687774913));
#28067=CARTESIAN_POINT('Ctrl Pts',(-12.914930261871,-12.2910798159437,-10.1691925801447));
#28068=CARTESIAN_POINT('Ctrl Pts',(-12.6766175616922,-12.0845161595089,
-10.4842201521152));
#28069=CARTESIAN_POINT('Ctrl Pts',(-12.6251185176542,-12.0255296144883,
-10.5621936286663));
#28070=CARTESIAN_POINT('Ctrl Pts',(-12.6199210072709,-12.0194051204483,
-10.5701811473657));
#28071=CARTESIAN_POINT('',(-16.0111004341151,-11.9818299434094,-8.00000000095188));
#28072=CARTESIAN_POINT('Origin',(0.,0.,-8.));
#28073=CARTESIAN_POINT('',(-14.6214037084642,-9.48383146588572,-10.5701811473657));
#28074=CARTESIAN_POINT('Ctrl Pts',(-14.6214037084642,-9.48383146588574,
-10.5701811473657));
#28075=CARTESIAN_POINT('Ctrl Pts',(-14.6266406861523,-9.48821113032728,
-10.5634041641841));
#28076=CARTESIAN_POINT('Ctrl Pts',(-14.6530901816378,-9.51184302815803,
-10.5283573869222));
#28077=CARTESIAN_POINT('Ctrl Pts',(-14.7486820590948,-9.60956316387482,
-10.3949490657943));
#28078=CARTESIAN_POINT('Ctrl Pts',(-14.802496945566,-9.67073361645766,-10.3164610148372));
#28079=CARTESIAN_POINT('Ctrl Pts',(-15.0177813913654,-9.93191529664271,
-9.99324636542056));
#28080=CARTESIAN_POINT('Ctrl Pts',(-15.1681116713633,-10.1581772761004,
-9.74293994937975));
#28081=CARTESIAN_POINT('Ctrl Pts',(-15.5835674685494,-10.8715932816978,
-8.9984934444827));
#28082=CARTESIAN_POINT('Ctrl Pts',(-15.8236941959833,-11.4198346979515,
-8.48676451123472));
#28083=CARTESIAN_POINT('Ctrl Pts',(-16.0111004336212,-11.9818299445155,
-8.00000000203882));
#28084=CARTESIAN_POINT('',(-14.6205143845238,-9.48308765551918,-10.5713320279724));
#28085=CARTESIAN_POINT('Origin',(0.,0.,-10.));
#28086=CARTESIAN_POINT('',(-9.75394809472372,-12.6805428184636,-12.));
#28087=CARTESIAN_POINT('',(-10.4953820000267,-13.9116971543312,-10.571332465393));
#28088=CARTESIAN_POINT('Origin',(119.207424280112,-96.0243788233682,-15.4574255506602));
#28089=CARTESIAN_POINT('',(-7.24608845304286,-14.2628844115113,-12.));
#28090=CARTESIAN_POINT('Origin',(0.,0.,-12.));
#28091=CARTESIAN_POINT('',(-7.7475658951531,-15.6097278391302,-10.5713323676496));
#28092=CARTESIAN_POINT('Origin',(134.881737317284,-72.3740856247587,-15.4574255506782));
#28093=CARTESIAN_POINT('',(-7.74796798344852,-15.610813489587,-10.5701811473657));
#28094=CARTESIAN_POINT('',(-7.74796798345149,-15.610813489595,-10.5701811473572));
#28095=CARTESIAN_POINT('',(-9.4836287665753,-17.6062594366147,-8.00000000066547));
#28096=CARTESIAN_POINT('Ctrl Pts',(-9.4836287675511,-17.606259436394,-8.0000000013502));
#28097=CARTESIAN_POINT('Ctrl Pts',(-9.117217467711,-17.3165911098976,-8.42878732671352));
#28098=CARTESIAN_POINT('Ctrl Pts',(-8.76804424999057,-16.9950876418137,
-8.87475271998277));
#28099=CARTESIAN_POINT('Ctrl Pts',(-8.19927701868966,-16.3597208566847,
-9.69886562696287));
#28100=CARTESIAN_POINT('Ctrl Pts',(-8.03448058174276,-16.1213826471877,
-9.9854522442967));
#28101=CARTESIAN_POINT('Ctrl Pts',(-7.88218185215363,-15.8778256257657,
-10.2713413953036));
#28102=CARTESIAN_POINT('Ctrl Pts',(-7.83611291692439,-15.7974340885403,
-10.363829818583));
#28103=CARTESIAN_POINT('Ctrl Pts',(-7.76477618887298,-15.6543851854117,
-10.5236791254642));
#28104=CARTESIAN_POINT('Ctrl Pts',(-7.75009649497616,-15.6165616292045,
-10.5640860164002));
#28105=CARTESIAN_POINT('Ctrl Pts',(-7.74796798344854,-15.610813489587,-10.5701811473657));
#28106=CARTESIAN_POINT('',(-10.9474857635323,-16.7353560273778,-8.00000000093432));
#28107=CARTESIAN_POINT('Origin',(0.,0.,-8.));
#28108=CARTESIAN_POINT('',(-10.4959637731368,-13.9127010372614,-10.5701811473657));
#28109=CARTESIAN_POINT('Ctrl Pts',(-10.4959637731368,-13.9127010372614,
-10.5701811473657));
#28110=CARTESIAN_POINT('Ctrl Pts',(-10.5016144965552,-13.9224512471231,
-10.5589943395551));
#28111=CARTESIAN_POINT('Ctrl Pts',(-10.5588056031706,-14.0253908156642,
-10.4424780519163));
#28112=CARTESIAN_POINT('Ctrl Pts',(-10.6920761196939,-14.403470848196,-10.0598381501417));
#28113=CARTESIAN_POINT('Ctrl Pts',(-10.7669214238514,-14.6622159545809,
-9.80772126558064));
#28114=CARTESIAN_POINT('Ctrl Pts',(-10.9140625729676,-15.4695925407666,
-9.06700805922446));
#28115=CARTESIAN_POINT('Ctrl Pts',(-10.9659919500273,-16.0554512414216,
-8.558848801484));
#28116=CARTESIAN_POINT('Ctrl Pts',(-10.9474857627035,-16.7353560282324,
-8.00000000200139));
#28117=CARTESIAN_POINT('',(-10.4953824801207,-13.9116979174471,-10.5713320279724));
#28118=CARTESIAN_POINT('Origin',(0.,0.,-10.));
#28119=CARTESIAN_POINT('',(-4.82871197592244,-15.2518592394185,-12.));
#28120=CARTESIAN_POINT('',(-5.10435236312695,-16.6623512144413,-10.5713324653942));
#28121=CARTESIAN_POINT('Origin',(144.860608746725,-49.4620598580445,-15.4574255505872));
#28122=CARTESIAN_POINT('',(-1.93090207822381,-15.8810354438797,-12.));
#28123=CARTESIAN_POINT('Origin',(0.,0.,-12.));
#28124=CARTESIAN_POINT('',(-1.94148914791405,-17.3181696607923,-10.5713323676496));
#28125=CARTESIAN_POINT('Origin',(151.500768374491,-21.8771230684231,-15.4574255506288));
#28126=CARTESIAN_POINT('',(-1.94149567299321,-17.3193273608118,-10.5701811473657));
#28127=CARTESIAN_POINT('',(-1.94149567299325,-17.3193273608203,-10.5701811473572));
#28128=CARTESIAN_POINT('',(-2.89000059425648,-19.7880641422247,-8.00000000066547));
#28129=CARTESIAN_POINT('Ctrl Pts',(-2.89000059524895,-19.788064142351,-8.00000000135019));
#28130=CARTESIAN_POINT('Ctrl Pts',(-2.64475964944046,-19.390545976467,-8.42878617624322));
#28131=CARTESIAN_POINT('Ctrl Pts',(-2.42659969730428,-18.969005960538,-8.87475352969895));
#28132=CARTESIAN_POINT('Ctrl Pts',(-2.10944806523733,-18.1774498974171,
-9.69884249148341));
#28133=CARTESIAN_POINT('Ctrl Pts',(-2.03610698489061,-17.897130334085,-9.98542034710692));
#28134=CARTESIAN_POINT('Ctrl Pts',(-1.97628997605455,-17.6161445061853,
-10.2713376723449));
#28135=CARTESIAN_POINT('Ctrl Pts',(-1.96049432141494,-17.5248410226167,
-10.3638297782074));
#28136=CARTESIAN_POINT('Ctrl Pts',(-1.94238591343281,-17.3660145389405,
-10.5236848708411));
#28137=CARTESIAN_POINT('Ctrl Pts',(-1.94152981246431,-17.3254518932265,
-10.5640909344707));
#28138=CARTESIAN_POINT('Ctrl Pts',(-1.9414956729932,-17.3193273608118,-10.5701811473657));
#28139=CARTESIAN_POINT('',(-4.56344268684126,-19.4703512230268,-8.00000000095185));
#28140=CARTESIAN_POINT('Origin',(0.,0.,-8.));
#28141=CARTESIAN_POINT('',(-5.10455570284158,-16.6634935339443,-10.5701811473657));
#28142=CARTESIAN_POINT('Ctrl Pts',(-5.10455570284158,-16.6634935339443,
-10.5701811473657));
#28143=CARTESIAN_POINT('Ctrl Pts',(-5.10575225004077,-16.6702147236891,
-10.5634042571818));
#28144=CARTESIAN_POINT('Ctrl Pts',(-5.11082706386516,-16.7053218794149,
-10.5283538727596));
#28145=CARTESIAN_POINT('Ctrl Pts',(-5.12125055227524,-16.841631642325,-10.3949366518273));
#28146=CARTESIAN_POINT('Ctrl Pts',(-5.123158335631,-16.9230826458571,-10.3164476357533));
#28147=CARTESIAN_POINT('Ctrl Pts',(-5.12019877867727,-17.2615339871035,
-9.99323823060328));
#28148=CARTESIAN_POINT('Ctrl Pts',(-5.08991797324345,-17.5314913874667,
-9.74293234839749));
#28149=CARTESIAN_POINT('Ctrl Pts',(-4.94959210955161,-18.3450426247206,
-8.99849520609888));
#28150=CARTESIAN_POINT('Ctrl Pts',(-4.7811241129742,-18.9193771874646,-8.48676299679378));
#28151=CARTESIAN_POINT('Ctrl Pts',(-4.56344268575194,-19.4703512235566,
-8.00000000203874));
#28152=CARTESIAN_POINT('',(-5.10435255326646,-16.6623520957364,-10.5713320279724));
#28153=CARTESIAN_POINT('Origin',(0.,0.,-10.));
#28154=CARTESIAN_POINT('',(0.678938071373981,-15.9835763426303,-12.));
#28155=CARTESIAN_POINT('',(0.902337501759208,-17.403279810577,-10.571332459878));
#28156=CARTESIAN_POINT('Origin',(153.041465883414,3.06611350829458,-15.4574255506013));
#28157=CARTESIAN_POINT('',(3.61717958430867,-15.5836992225952,-12.));
#28158=CARTESIAN_POINT('Origin',(0.,0.,-12.));
#28159=CARTESIAN_POINT('',(4.09875984389177,-16.9377846323997,-10.5713323676496));
#28160=CARTESIAN_POINT('Origin',(149.846570852324,31.2585434019396,-15.4574255506915));
#28161=CARTESIAN_POINT('',(4.09914966904954,-16.9388747462736,-10.5701811473657));
#28162=CARTESIAN_POINT('',(4.09914966905241,-16.9388747462817,-10.5701811473572));
#28163=CARTESIAN_POINT('',(4.05220430155578,-19.5831362715489,-8.00000000066547));
#28164=CARTESIAN_POINT('Ctrl Pts',(4.05220430066636,-19.583136272007,-8.00000000135019));
#28165=CARTESIAN_POINT('Ctrl Pts',(4.14669632797403,-19.1257133311813,-8.42878684336377));
#28166=CARTESIAN_POINT('Ctrl Pts',(4.20752191861409,-18.654981918085,-8.8747530592572));
#28167=CARTESIAN_POINT('Ctrl Pts',(4.23481731143593,-17.8026909310343,-9.6988417711401));
#28168=CARTESIAN_POINT('Ctrl Pts',(4.20786159958046,-17.5141886501232,-9.98542319374921));
#28169=CARTESIAN_POINT('Ctrl Pts',(4.16796931936474,-17.2296902079935,-10.2713398280925));
#28170=CARTESIAN_POINT('Ctrl Pts',(4.15158517621114,-17.1384926618717,-10.3638297968096));
#28171=CARTESIAN_POINT('Ctrl Pts',(4.11428113814045,-16.9830542376001,-10.5236815368766));
#28172=CARTESIAN_POINT('Ctrl Pts',(4.10121326794294,-16.9446443015219,-10.5640880820779));
#28173=CARTESIAN_POINT('Ctrl Pts',(4.09914966904953,-16.9388747462736,-10.5701811473657));
#28174=CARTESIAN_POINT('',(2.37101889769492,-19.8569346902003,-8.00000000095185));
#28175=CARTESIAN_POINT('Origin',(0.,0.,-8.));
#28176=CARTESIAN_POINT('',(0.902537120435117,-17.4044227834609,-10.5701811473657));
#28177=CARTESIAN_POINT('Ctrl Pts',(0.902537120435115,-17.4044227834609,
-10.5701811473657));
#28178=CARTESIAN_POINT('Ctrl Pts',(0.903711515723591,-17.4111478767184,
-10.5634042595934));
#28179=CARTESIAN_POINT('Ctrl Pts',(0.910950040711359,-17.4458735971854,
-10.5283537818598));
#28180=CARTESIAN_POINT('Ctrl Pts',(0.947775684990051,-17.5775281581801,
-10.3949363305994));
#28181=CARTESIAN_POINT('Ctrl Pts',(0.973840772098866,-17.6547195948464,
-10.316447289258));
#28182=CARTESIAN_POINT('Ctrl Pts',(1.09237877572117,-17.9717474777571,-9.99323801666938));
#28183=CARTESIAN_POINT('Ctrl Pts',(1.21316434535198,-18.2150677945305,-9.7429321503027));
#28184=CARTESIAN_POINT('Ctrl Pts',(1.62327857991182,-18.9315613705256,-8.99849525191663));
#28185=CARTESIAN_POINT('Ctrl Pts',(1.97802108053847,-19.413639923583,-8.48676295706184));
#28186=CARTESIAN_POINT('Ctrl Pts',(2.37101889889975,-19.8569346903256,-8.00000000203875));
#28187=CARTESIAN_POINT('',(0.902337623732299,-17.403280701153,-10.5713320279724));
#28188=CARTESIAN_POINT('Origin',(0.,0.,-10.));
#28189=CARTESIAN_POINT('',(6.10469816720395,-14.7874382464574,-12.));
#28190=CARTESIAN_POINT('',(6.80019214539348,-16.0451160116112,-10.5713324653937));
#28191=CARTESIAN_POINT('Origin',(142.763263582719,55.2244683340621,-15.4574255506391));
#28192=CARTESIAN_POINT('',(8.72897600508842,-13.4067388841598,-12.));
#28193=CARTESIAN_POINT('Origin',(0.,0.,-12.));
#28194=CARTESIAN_POINT('',(9.64463790727137,-14.5144528022616,-10.5713323676496));
#28195=CARTESIAN_POINT('Origin',(130.118665385375,80.6239682110759,-15.4574255506054));
#28196=CARTESIAN_POINT('',(9.64537706399892,-14.5153438461684,-10.5701811473657));
#28197=CARTESIAN_POINT('',(9.64537706400438,-14.515343846175,-10.5701811473572));
#28198=CARTESIAN_POINT('',(10.5056535544358,-17.0161931502252,-8.00000000066548));
#28199=CARTESIAN_POINT('Ctrl Pts',(10.5056535537567,-17.0161931509599,-8.0000000013502));
#28200=CARTESIAN_POINT('Ctrl Pts',(10.4379990385103,-16.5540372636988,-8.42878754129977));
#28201=CARTESIAN_POINT('Ctrl Pts',(10.3341548987057,-16.0908934577644,-8.87475256656962));
#28202=CARTESIAN_POINT('Ctrl Pts',(10.0682943446443,-15.2806435812879,-9.69886537541095));
#28203=CARTESIAN_POINT('Ctrl Pts',(9.9442855298204,-15.0187552446499,-9.9854531570782));
#28204=CARTESIAN_POINT('Ctrl Pts',(9.80950865931173,-14.7650822009551,-10.2713420952875));
#28205=CARTESIAN_POINT('Ctrl Pts',(9.76292237502594,-14.6849901508317,-10.3638298298625));
#28206=CARTESIAN_POINT('Ctrl Pts',(9.67470755157361,-14.5516870556634,-10.523678050232));
#28207=CARTESIAN_POINT('Ctrl Pts',(9.64929143497573,-14.5200619743586,-10.5640850947478));
#28208=CARTESIAN_POINT('Ctrl Pts',(9.64537706399891,-14.5153438461684,-10.5701811473657));
#28209=CARTESIAN_POINT('',(9.01950057931991,-17.8484787924764,-8.00000000093431));
#28210=CARTESIAN_POINT('Origin',(0.,0.,-8.));
#28211=CARTESIAN_POINT('',(6.80077064695808,-16.0461217833684,-10.5701811473657));
#28212=CARTESIAN_POINT('Ctrl Pts',(6.80077064695807,-16.0461217833684,-10.5701811473657));
#28213=CARTESIAN_POINT('Ctrl Pts',(6.80638919136614,-16.055890517792,-10.5589943859768));
#28214=CARTESIAN_POINT('Ctrl Pts',(6.86694184542916,-16.1568892018711,-10.4424781747251));
#28215=CARTESIAN_POINT('Ctrl Pts',(7.12773354554721,-16.4613449440162,-10.0598381880387));
#28216=CARTESIAN_POINT('Ctrl Pts',(7.31439070777692,-16.6555354433093,-9.80772130191037));
#28217=CARTESIAN_POINT('Ctrl Pts',(7.940028774259,-17.1866517142592,-9.06700808923736));
#28218=CARTESIAN_POINT('Ctrl Pts',(8.42143261566513,-17.524553198201,-8.55884885148502));
#28219=CARTESIAN_POINT('Ctrl Pts',(9.01950058047433,-17.848478792186,-8.00000000200139));
#28220=CARTESIAN_POINT('',(6.80019256622394,-16.0451168089422,-10.5713320279724));
#28221=CARTESIAN_POINT('Origin',(0.,0.,-10.));
#28222=CARTESIAN_POINT('',(10.7941415683196,-11.8077168584163,-12.));
#28223=CARTESIAN_POINT('',(11.8778432569201,-12.7516744235547,-10.5713324653927));
#28224=CARTESIAN_POINT('Origin',(115.265704733382,100.721937252619,-15.4574255506547));
#28225=CARTESIAN_POINT('',(12.787929093689,-9.61272797390185,-12.));
#28226=CARTESIAN_POINT('Origin',(0.,0.,-12.));
#28227=CARTESIAN_POINT('',(14.0272302993381,-10.3404637536614,-10.5713323676496));
#28228=CARTESIAN_POINT('Origin',(94.696528526693,120.26495257181,-15.45742555065));
#28229=CARTESIAN_POINT('',(14.0282296344253,-10.3410482545556,-10.5701811473657));
#28230=CARTESIAN_POINT('',(14.0282296344327,-10.3410482545599,-10.5701811473572));
#28231=CARTESIAN_POINT('',(15.6919659514913,-12.3968459903841,-8.00000000066043));
#28232=CARTESIAN_POINT('Ctrl Pts',(15.6919659511093,-12.3968459912986,-8.00000000133986));
#28233=CARTESIAN_POINT('Ctrl Pts',(15.3272491998243,-11.7202924653894,-8.70558356387746));
#28234=CARTESIAN_POINT('Ctrl Pts',(14.9265913761347,-11.1890623070545,-9.34347605757007));
#28235=CARTESIAN_POINT('Ctrl Pts',(14.435006267903,-10.664861021749,-10.0506525934817));
#28236=CARTESIAN_POINT('Ctrl Pts',(14.306339263984,-10.5520493954836,-10.2211209350345));
#28237=CARTESIAN_POINT('Ctrl Pts',(14.1052003455229,-10.3887460880048,-10.479922296626));
#28238=CARTESIAN_POINT('Ctrl Pts',(14.0365451533539,-10.3459112245296,-10.5606021910004));
#28239=CARTESIAN_POINT('Ctrl Pts',(14.0282296344253,-10.3410482545556,-10.5701811473657));
#28240=CARTESIAN_POINT('',(14.5800974363697,-13.6872329069855,-8.00000000095188));
#28241=CARTESIAN_POINT('Origin',(0.,0.,-8.));
#28242=CARTESIAN_POINT('',(11.8787308647727,-12.7524216806657,-10.5701811473657));
#28243=CARTESIAN_POINT('Ctrl Pts',(11.8787308647727,-12.7524216806657,-10.5701811473657));
#28244=CARTESIAN_POINT('Ctrl Pts',(11.8839533839603,-12.7568185761951,-10.5634041641087));
#28245=CARTESIAN_POINT('Ctrl Pts',(11.9118191664865,-12.7787626049719,-10.5283573896208));
#28246=CARTESIAN_POINT('Ctrl Pts',(12.0246540683316,-12.8559332949065,-10.3949490753023));
#28247=CARTESIAN_POINT('Ctrl Pts',(12.0942400622771,-12.8983084728067,-10.3164610250273));
#28248=CARTESIAN_POINT('Ctrl Pts',(12.3888375657762,-13.0649685395278,-9.99324637123619));
#28249=CARTESIAN_POINT('Ctrl Pts',(12.637766695706,-13.1737249857198,-9.74293995466056));
#28250=CARTESIAN_POINT('Ctrl Pts',(13.412487452553,-13.4589856947937,-8.99849344264267));
#28251=CARTESIAN_POINT('Ctrl Pts',(13.9940974086421,-13.6002632407572,-8.48676451217013));
#28252=CARTESIAN_POINT('Ctrl Pts',(14.5800974373733,-13.687232906307,-8.00000000203881));
#28253=CARTESIAN_POINT('',(11.8778439250753,-12.7516750288689,-10.5713320279724));
#28254=CARTESIAN_POINT('Origin',(0.,0.,-10.));
#28255=CARTESIAN_POINT('',(14.1816521917328,-7.40381055390889,-12.));
#28256=CARTESIAN_POINT('',(15.5228511760086,-7.92019270597788,-10.5713324598785));
#28257=CARTESIAN_POINT('Origin',(73.8654007527194,134.070854041584,-15.4574255507092));
#28258=CARTESIAN_POINT('',(15.3044692038576,-4.65928020123585,-12.));
#28259=CARTESIAN_POINT('Origin',(0.,0.,-12.));
#28260=CARTESIAN_POINT('',(16.7179316974337,-4.91926216737799,-10.5713323676496));
#28261=CARTESIAN_POINT('Origin',(47.8525927546613,145.400208728593,-15.4574255506749));
#28262=CARTESIAN_POINT('',(16.7190706763204,-4.91946962582535,-10.5701811473657));
#28263=CARTESIAN_POINT('',(16.7190706763288,-4.91946962582688,-10.5701811473572));
#28264=CARTESIAN_POINT('',(18.9855956526705,-6.28225625435353,-8.00000000066041));
#28265=CARTESIAN_POINT('Ctrl Pts',(18.9855956526243,-6.28225625534351,-8.00000000133983));
#28266=CARTESIAN_POINT('Ctrl Pts',(18.411474177151,-5.77123997637943,-8.70558959925413));
#28267=CARTESIAN_POINT('Ctrl Pts',(17.8532967549382,-5.40907168025849,-9.34347563383209));
#28268=CARTESIAN_POINT('Ctrl Pts',(17.2120575414615,-5.08460724071215,-10.0506668368878));
#28269=CARTESIAN_POINT('Ctrl Pts',(17.0525658199616,-5.02261030481196,-10.2211342731052));
#28270=CARTESIAN_POINT('Ctrl Pts',(16.807712775309,-4.93795899302286,-10.4799244165698));
#28271=CARTESIAN_POINT('Ctrl Pts',(16.728543360769,-4.92119441373731,-10.5606068211688));
#28272=CARTESIAN_POINT('Ctrl Pts',(16.7190706763204,-4.91946962582536,-10.5701811473657));
#28273=CARTESIAN_POINT('',(18.3821193180501,-7.87510477916341,-8.00000000093431));
#28274=CARTESIAN_POINT('Origin',(0.,0.,-8.));
#28275=CARTESIAN_POINT('',(15.5239408288994,-7.92059131757519,-10.5701811473657));
#28276=CARTESIAN_POINT('Ctrl Pts',(15.5239408288994,-7.92059131757522,-10.5701811473657));
#28277=CARTESIAN_POINT('Ctrl Pts',(15.5345224289455,-7.92446245837779,-10.5589961576797));
#28278=CARTESIAN_POINT('Ctrl Pts',(15.6458257921794,-7.96290977382766,-10.442482799353));
#28279=CARTESIAN_POINT('Ctrl Pts',(16.0413073392502,-8.02850372400974,-10.0598395697742));
#28280=CARTESIAN_POINT('Ctrl Pts',(16.3091180269029,-8.05728223823699,-9.80772253039812));
#28281=CARTESIAN_POINT('Ctrl Pts',(17.1297801903807,-8.06198840490791,-9.06700881562152));
#28282=CARTESIAN_POINT('Ctrl Pts',(17.7157553277321,-8.01139446553857,-8.55885052036936));
#28283=CARTESIAN_POINT('Ctrl Pts',(18.3821193187478,-7.87510477819889,-8.00000000200138));
#28284=CARTESIAN_POINT('',(15.5228520082561,-7.92019304563387,-10.5713320279724));
#28285=CARTESIAN_POINT('Origin',(0.,-19.9979895488606,-8.));
#28286=CARTESIAN_POINT('',(19.9690530659844,-1.11210632608748,-8.));
#28287=CARTESIAN_POINT('',(19.9669855232122,-1.11312313271343,-8.));
#28288=CARTESIAN_POINT('',(19.9913217286364,0.58899607364984,-8.));
#28289=CARTESIAN_POINT('',(19.9913217286364,0.58899607364984,-8.));
#28290=CARTESIAN_POINT('Origin',(-0.00301694686781318,3.94939979918296E-5,
-8.));
#28291=CARTESIAN_POINT('Origin',(0.,-19.9979895488606,-8.));
#28292=CARTESIAN_POINT('',(19.1451345752296,5.78478028355213,-8.));
#28293=CARTESIAN_POINT('',(19.1435395109765,5.78311763536045,-8.));
#28294=CARTESIAN_POINT('',(18.5842506056703,7.39091063456494,-8.00000000377262));
#28295=CARTESIAN_POINT('',(18.5842489954763,7.39090998578283,-8.));
#28296=CARTESIAN_POINT('Origin',(-0.00284851047704926,-0.000994744391011881,
-8.));
#28297=CARTESIAN_POINT('Origin',(0.,-19.9979895488606,-8.));
#28298=CARTESIAN_POINT('',(16.0120303026084,11.983937016731,-8.));
#28299=CARTESIAN_POINT('',(16.0111000635635,11.9818291068306,-8.));
#28300=CARTESIAN_POINT('',(14.9356428424434,13.3013722399403,-8.00000000377261));
#28301=CARTESIAN_POINT('',(14.9356415512525,13.3013710795657,-8.));
#28302=CARTESIAN_POINT('Origin',(-0.00233650163240506,-0.00190900190652155,
-8.));
#28303=CARTESIAN_POINT('Origin',(0.,-19.9979895488606,-8.));
#28304=CARTESIAN_POINT('',(10.9476388630933,16.7376540816183,-8.));
#28305=CARTESIAN_POINT('',(10.9474857026353,16.7353551316722,-8.));
#28306=CARTESIAN_POINT('',(9.48557530180814,17.6074905090519,-8.));
#28307=CARTESIAN_POINT('',(9.48557530180814,17.6074905090519,-8.));
#28308=CARTESIAN_POINT('Origin',(-0.00154267626085947,-0.00259300566760157,
-8.));
#28309=CARTESIAN_POINT('Origin',(0.,-19.9979895488606,-8.));
#28310=CARTESIAN_POINT('',(4.56280060674729,19.4725630427967,-8.));
#28311=CARTESIAN_POINT('',(4.56344294071614,19.4703503440143,-8.));
#28312=CARTESIAN_POINT('',(2.89140893620136,19.7898884520894,-8.00000000377262));
#28313=CARTESIAN_POINT('',(2.89140869296617,19.7898867332294,-8.));
#28314=CARTESIAN_POINT('Origin',(-0.000562781322250294,-0.0029642546098918,
-8.));
#28315=CARTESIAN_POINT('Origin',(0.,-19.9979895488606,-8.));
#28316=CARTESIAN_POINT('',(-2.37237874253754,19.8587935165906,-8.));
#28317=CARTESIAN_POINT('',(-2.37101835849106,19.8569339510296,-8.));
#28318=CARTESIAN_POINT('',(-4.05150484375975,19.5853322433773,-8.00000000377262));
#28319=CARTESIAN_POINT('',(-4.05150448444132,19.5853305449859,-8.));
#28320=CARTESIAN_POINT('Origin',(0.000484993332277583,-0.00297797073663508,
-8.));
#28321=CARTESIAN_POINT('Origin',(0.,-19.9979895488606,-8.));
#28322=CARTESIAN_POINT('',(-9.02141420289104,17.8497604077057,-8.));
#28323=CARTESIAN_POINT('',(-9.01949983406462,17.8484782918853,-8.));
#28324=CARTESIAN_POINT('',(-10.5057473457201,17.0184959173946,-8.00000000377262));
#28325=CARTESIAN_POINT('',(-10.5057464271872,17.018494444323,-8.));
#28326=CARTESIAN_POINT('Origin',(0.00147427065201211,-0.00263249966895751,
-8.));
#28327=CARTESIAN_POINT('Origin',(0.,-19.9979895488606,-8.));
#28328=CARTESIAN_POINT('',(-14.5823339684823,13.6877827592445,-8.));
#28329=CARTESIAN_POINT('',(-14.5800965481548,13.6872326873338,-8.));
#28330=CARTESIAN_POINT('',(-15.6928402991217,12.3989767391864,-8.));
#28331=CARTESIAN_POINT('',(-15.6928402991217,12.3989767391864,-8.));
#28332=CARTESIAN_POINT('Origin',(0.00228572915365266,-0.00196951024334036,
-8.));
#28333=CARTESIAN_POINT('Origin',(0.,-19.9979895488606,-8.));
#28334=CARTESIAN_POINT('',(-18.3844090451459,7.87485649985959,-8.));
#28335=CARTESIAN_POINT('',(-18.3821184221034,7.8751048441898,-8.));
#28336=CARTESIAN_POINT('',(-18.9871476862031,6.28396000343702,-8.00000000377262));
#28337=CARTESIAN_POINT('',(-18.9871460356938,6.28395946542021,-8.));
#28338=CARTESIAN_POINT('Origin',(0.00282149497524475,-0.00106896882248741,
-8.));
#28339=CARTESIAN_POINT('Origin',(0.,-19.9979895488606,-8.));
#28340=CARTESIAN_POINT('',(-19.9690530659844,1.11210632608748,-8.));
#28341=CARTESIAN_POINT('',(-19.9669855232122,1.11312313271343,-8.));
#28342=CARTESIAN_POINT('',(-19.9913234715256,-0.588996128437261,-8.00000000377262));
#28343=CARTESIAN_POINT('',(-19.9913217365416,-0.588996069500264,-8.));
#28344=CARTESIAN_POINT('Origin',(0.00301694686786202,-3.94939976390563E-5,
-8.));
#28345=CARTESIAN_POINT('Origin',(0.,-19.9979895488606,-8.));
#28346=CARTESIAN_POINT('',(-19.1451345752296,-5.78478028355213,-8.));
#28347=CARTESIAN_POINT('',(-19.1435395109765,-5.78311763536045,-8.));
#28348=CARTESIAN_POINT('',(-18.5842506056703,-7.39091063456494,-8.00000000377262));
#28349=CARTESIAN_POINT('',(-18.5842489954764,-7.39090998578282,-8.));
#28350=CARTESIAN_POINT('Origin',(0.00284851047831713,0.000994744391827895,
-8.));
#28351=CARTESIAN_POINT('Origin',(0.,-19.9979895488606,-8.));
#28352=CARTESIAN_POINT('',(-16.0120303026084,-11.983937016731,-8.));
#28353=CARTESIAN_POINT('',(-16.0111000635635,-11.9818291068306,-8.));
#28354=CARTESIAN_POINT('',(-14.9356415425294,-13.3013710776631,-8.));
#28355=CARTESIAN_POINT('',(-14.9356415425294,-13.3013710776631,-8.));
#28356=CARTESIAN_POINT('Origin',(0.0023365016822785,0.00190900194720678,
-8.));
#28357=CARTESIAN_POINT('Origin',(0.,-19.9979895488606,-8.));
#28358=CARTESIAN_POINT('',(-10.9476388630933,-16.7376540816183,-8.));
#28359=CARTESIAN_POINT('',(-10.9474857026353,-16.7353551316722,-8.));
#28360=CARTESIAN_POINT('',(-9.48557612580544,-17.6074920458319,-8.00000000377262));
#28361=CARTESIAN_POINT('',(-9.4855753093544,-17.6074905138232,-8.));
#28362=CARTESIAN_POINT('Origin',(0.00154267626200966,0.00259300566851861,
-8.));
#28363=CARTESIAN_POINT('Origin',(0.,-19.9979895488606,-8.));
#28364=CARTESIAN_POINT('',(-4.56280060674728,-19.4725630427967,-8.));
#28365=CARTESIAN_POINT('',(-4.56344294071613,-19.4703503440143,-8.));
#28366=CARTESIAN_POINT('',(-2.89140893620135,-19.7898884520893,-8.00000000377262));
#28367=CARTESIAN_POINT('',(-2.89140869296616,-19.7898867332294,-8.));
#28368=CARTESIAN_POINT('Origin',(0.000562781322135386,0.00296425461041583,
-8.));
#28369=CARTESIAN_POINT('Origin',(0.,-19.9979895488606,-8.));
#28370=CARTESIAN_POINT('',(2.37237874253754,-19.8587935165906,-8.));
#28371=CARTESIAN_POINT('',(2.37101835849106,-19.8569339510296,-8.));
#28372=CARTESIAN_POINT('',(4.05150484375973,-19.5853322433773,-8.00000000377262));
#28373=CARTESIAN_POINT('',(4.05150448444132,-19.585330544986,-8.));
#28374=CARTESIAN_POINT('Origin',(-0.000484993332055816,0.00297797073728345,
-8.));
#28375=CARTESIAN_POINT('Origin',(0.,-19.9979895488606,-8.));
#28376=CARTESIAN_POINT('',(9.02141420289106,-17.8497604077057,-8.));
#28377=CARTESIAN_POINT('',(9.01949983406462,-17.8484782918853,-8.));
#28378=CARTESIAN_POINT('',(10.5057473457202,-17.0184959173946,-8.00000000377261));
#28379=CARTESIAN_POINT('',(10.5057464271872,-17.018494444323,-8.));
#28380=CARTESIAN_POINT('Origin',(-0.00147427065151251,0.00263249966817813,
-8.));
#28381=CARTESIAN_POINT('Origin',(0.,-19.9979895488606,-8.));
#28382=CARTESIAN_POINT('',(14.5823339684823,-13.6877827592445,-8.));
#28383=CARTESIAN_POINT('',(14.5800965481548,-13.6872326873338,-8.));
#28384=CARTESIAN_POINT('',(15.6928402991217,-12.3989767391864,-8.));
#28385=CARTESIAN_POINT('',(15.6928402991217,-12.3989767391864,-8.));
#28386=CARTESIAN_POINT('Origin',(-0.00228572915365266,0.00196951024334036,
-8.));
#28387=CARTESIAN_POINT('Origin',(0.,-19.9979895488606,-8.));
#28388=CARTESIAN_POINT('',(18.3844090451459,-7.8748564998596,-8.));
#28389=CARTESIAN_POINT('',(18.3821184253814,-7.8751048747288,-8.));
#28390=CARTESIAN_POINT('',(18.9871460296846,-6.28395945881716,-8.));
#28391=CARTESIAN_POINT('',(18.9871460296846,-6.28395945881716,-8.));
#28392=CARTESIAN_POINT('Origin',(-0.00282149497482953,0.00106896882247964,
-8.));
#28393=CARTESIAN_POINT('Origin',(0.,24.1327223341711,-4.));
#28394=CARTESIAN_POINT('',(19.9913181983012,-0.588996262810959,-4.00000000280937));
#28395=CARTESIAN_POINT('',(19.9039912377183,-0.634233661918812,-3.99999999974498));
#28396=CARTESIAN_POINT('Origin',(19.1722717191265,1.97134495680374,-4.));
#28397=CARTESIAN_POINT('',(19.9690495720087,1.11210570270611,-3.99999999517897));
#28398=CARTESIAN_POINT('Origin',(-0.00301694691578147,-3.94939979864173E-5,
-4.));
#28399=CARTESIAN_POINT('',(19.8805681942686,1.15504449566104,-3.99999999942637));
#28400=CARTESIAN_POINT('Ctrl Pts',(19.8805681939836,1.15504449506584,-4.));
#28401=CARTESIAN_POINT('Ctrl Pts',(19.8953407698874,1.14797303633899,-4.));
#28402=CARTESIAN_POINT('Ctrl Pts',(19.9100944560528,1.14086163112927,-4.));
#28403=CARTESIAN_POINT('Ctrl Pts',(19.9395859598404,1.12654859964875,-4.));
#28404=CARTESIAN_POINT('Ctrl Pts',(19.9543240817709,1.11934667292683,-4.));
#28405=CARTESIAN_POINT('Ctrl Pts',(19.9690425803289,1.11210530225922,-4.));
#28406=CARTESIAN_POINT('Origin',(0.,0.,-4.));
#28407=CARTESIAN_POINT('Origin',(0.,24.1327223341711,-4.));
#28408=CARTESIAN_POINT('',(18.9871427769515,6.28395807361808,-4.00000000280937));
#28409=CARTESIAN_POINT('',(18.9205613829861,6.21155990717689,-3.99999999972963));
#28410=CARTESIAN_POINT('Origin',(17.7623944925155,8.36511986266225,-4.));
#28411=CARTESIAN_POINT('',(18.3844059803083,7.87485471676291,-3.99999999499105));
#28412=CARTESIAN_POINT('Origin',(-0.00282149497308426,-0.00106896882069996,
-4.));
#28413=CARTESIAN_POINT('',(18.2865666864733,7.88496026217301,-3.99999999944014));
#28414=CARTESIAN_POINT('Origin',(18.8467331574664,5.50254089697986,-4.00000000000001));
#28415=CARTESIAN_POINT('Origin',(0.,0.,-4.));
#28416=CARTESIAN_POINT('Origin',(0.,24.1327223341711,-4.));
#28417=CARTESIAN_POINT('',(15.6928377163185,12.3989743250248,-4.00000000280937));
#28418=CARTESIAN_POINT('',(15.6550192930803,12.3081879438969,-3.99999999974396));
#28419=CARTESIAN_POINT('Origin',(13.4170351668742,13.8335250454269,-4.));
#28420=CARTESIAN_POINT('',(14.582331698332,13.6877800354455,-3.99999999499104));
#28421=CARTESIAN_POINT('Origin',(-0.00228572913896219,-0.0019695102302042,
-4.));
#28422=CARTESIAN_POINT('',(14.4869365435604,13.6638131243706,-3.99999999943991));
#28423=CARTESIAN_POINT('Origin',(15.8280793362557,11.6165408927719,-4.00000000000001));
#28424=CARTESIAN_POINT('Origin',(0.,0.,-4.));
#28425=CARTESIAN_POINT('Origin',(0.,24.1327223341711,-4.));
#28426=CARTESIAN_POINT('',(10.505744825479,17.0184912834615,-4.00000000280937));
#28427=CARTESIAN_POINT('',(10.5012771500662,16.9202333832982,-3.99999999972948));
#28428=CARTESIAN_POINT('Origin',(8.22962456417494,17.8253797968202,-3.99999999999978));
#28429=CARTESIAN_POINT('',(9.02141299576732,17.8497570701434,-3.99999999517897));
#28430=CARTESIAN_POINT('Origin',(-0.00147427062574423,-0.0026324996252014,
-4.));
#28431=CARTESIAN_POINT('',(8.93996803521359,17.7946084824593,-3.99999999943877));
#28432=CARTESIAN_POINT('Ctrl Pts',(8.93996803557834,17.7946084819266,-4.));
#28433=CARTESIAN_POINT('Ctrl Pts',(8.95347996181212,17.803859942227,-4.));
#28434=CARTESIAN_POINT('Ctrl Pts',(8.96701623560628,17.8130763372781,-4.));
#28435=CARTESIAN_POINT('Ctrl Pts',(8.9941634619296,17.8314571197425,-4.));
#28436=CARTESIAN_POINT('Ctrl Pts',(9.00777496072053,17.8406216686514,-4.));
#28437=CARTESIAN_POINT('Ctrl Pts',(9.02140984672463,17.8497508149477,-4.));
#28438=CARTESIAN_POINT('Origin',(0.,0.,-4.));
#28439=CARTESIAN_POINT('Origin',(0.,24.1327223341711,-4.));
#28440=CARTESIAN_POINT('',(4.05150406040619,19.5853270269313,-4.00000000280937));
#28441=CARTESIAN_POINT('',(4.080889940232,19.4914713868594,-3.99999999974451));
#28442=CARTESIAN_POINT('Origin',(1.38702113800135,19.2224444775015,-4.));
#28443=CARTESIAN_POINT('',(2.37237875432575,19.858789970815,-3.99999999499105));
#28444=CARTESIAN_POINT('Origin',(-0.000484993334474715,-0.00297797075199169,
-4.));
#28445=CARTESIAN_POINT('',(2.31470740046591,19.7791114351774,-3.99999999944106));
#28446=CARTESIAN_POINT('Origin',(4.65787767890032,19.0736433944222,-4.00000000001511));
#28447=CARTESIAN_POINT('Origin',(0.,0.,-4.));
#28448=CARTESIAN_POINT('Origin',(0.,24.1327223341711,-4.));
#28449=CARTESIAN_POINT('',(-2.89140788818329,19.7898832823108,-4.00000000280937));
#28450=CARTESIAN_POINT('',(-2.83169367133746,19.7117383931695,-3.99999999974453));
#28451=CARTESIAN_POINT('Origin',(-5.27109455453329,18.5376028456143,-4.));
#28452=CARTESIAN_POINT('',(-4.56279938294332,19.4725597148893,-3.99999999499105));
#28453=CARTESIAN_POINT('Origin',(0.000562781319235484,-0.00296425459876293,
-4.));
#28454=CARTESIAN_POINT('',(-4.58974103670107,19.3779616247666,-3.99999999944051));
#28455=CARTESIAN_POINT('Origin',(-2.14638779193655,19.5161339587139,-4.));
#28456=CARTESIAN_POINT('Origin',(0.,0.,-4.));
#28457=CARTESIAN_POINT('Origin',(0.,24.1327223341711,-4.));
#28458=CARTESIAN_POINT('',(-9.4855733728222,17.6074875462724,-4.00000000280937));
#28459=CARTESIAN_POINT('',(-9.40271337253749,17.5544894759627,-3.99999999972949));
#28460=CARTESIAN_POINT('Origin',(-11.3224289626212,16.0397515114471,-4.));
#28461=CARTESIAN_POINT('',(-10.9476365748824,16.7376513729739,-3.99999999499105));
#28462=CARTESIAN_POINT('Origin',(0.00154267624008497,-0.00259300563156151,
-4.));
#28463=CARTESIAN_POINT('',(-10.9405989708154,16.6395436738711,-3.99999999943994));
#28464=CARTESIAN_POINT('Origin',(-8.69154686798984,17.6048190481095,-4.));
#28465=CARTESIAN_POINT('Origin',(0.,0.,-4.));
#28466=CARTESIAN_POINT('Origin',(0.,24.1327223341711,-4.));
#28467=CARTESIAN_POINT('',(-14.9356387165454,13.3013689533132,-4.00000000280937));
#28468=CARTESIAN_POINT('',(-14.8396644843238,13.2798899664757,-3.99999999974395));
#28469=CARTESIAN_POINT('Origin',(-15.9531968912017,10.8110539794297,-4.));
#28470=CARTESIAN_POINT('',(-16.0120272253659,11.9839352483846,-3.99999999517897));
#28471=CARTESIAN_POINT('Origin',(0.00233650163479426,-0.0019090019073964,
-4.));
#28472=CARTESIAN_POINT('',(-15.9718592319238,11.8941511756936,-3.99999999943859));
#28473=CARTESIAN_POINT('Ctrl Pts',(-15.9718592313356,11.8941511759604,-4.));
#28474=CARTESIAN_POINT('Ctrl Pts',(-15.9786238224323,11.9090643240662,-4.));
#28475=CARTESIAN_POINT('Ctrl Pts',(-15.9853496524799,11.9239953610795,-4.));
#28476=CARTESIAN_POINT('Ctrl Pts',(-15.9987371250949,11.9539219468768,-4.));
#28477=CARTESIAN_POINT('Ctrl Pts',(-16.0053988318356,11.9689180616204,-4.));
#28478=CARTESIAN_POINT('Ctrl Pts',(-16.0120216120262,11.9839310609795,-4.));
#28479=CARTESIAN_POINT('Origin',(0.,0.,-4.));
#28480=CARTESIAN_POINT('Origin',(0.,24.1327223341711,-4.));
#28481=CARTESIAN_POINT('',(-18.5842456045018,7.39090895728596,-4.00000000280937));
#28482=CARTESIAN_POINT('',(-18.4867130617665,7.40355047939383,-3.9999999997442));
#28483=CARTESIAN_POINT('Origin',(-18.6890790787513,4.70324601679737,-4.00000000001672));
#28484=CARTESIAN_POINT('',(-19.1451310812753,5.78477967944377,-3.99999999499105));
#28485=CARTESIAN_POINT('Origin',(0.00284851048307999,-0.000994744392314173,
-4.));
#28486=CARTESIAN_POINT('',(-19.0766775585171,5.71414847928127,-3.99999999944049));
#28487=CARTESIAN_POINT('Origin',(-17.9746451113272,7.899234737925,-4.00000000001512));
#28488=CARTESIAN_POINT('Origin',(0.,0.,-4.));
#28489=CARTESIAN_POINT('Origin',(0.,24.1327223341711,-4.));
#28490=CARTESIAN_POINT('',(-19.9913181983012,0.588996262810962,-4.00000000280937));
#28491=CARTESIAN_POINT('',(-19.9039912377183,0.634233661918836,-3.99999999974498));
#28492=CARTESIAN_POINT('Origin',(-19.1722692499955,-1.97135300847255,-4.));
#28493=CARTESIAN_POINT('',(-19.9690495761241,-1.11210569876088,-3.99999999499105));
#28494=CARTESIAN_POINT('Origin',(0.00301694687294463,3.94939983909548E-5,
-4.));
#28495=CARTESIAN_POINT('',(-19.8805670108458,-1.15506486493628,-3.99999999944111));
#28496=CARTESIAN_POINT('Origin',(-19.5927310596763,1.27500392343756,-4.00000000000001));
#28497=CARTESIAN_POINT('Origin',(0.,0.,-4.));
#28498=CARTESIAN_POINT('Origin',(0.,24.1327223341711,-4.));
#28499=CARTESIAN_POINT('',(-18.9871427769515,-6.28395807361808,-4.00000000280937));
#28500=CARTESIAN_POINT('',(-18.9205613829861,-6.21155990717691,-3.99999999972963));
#28501=CARTESIAN_POINT('Origin',(-17.7623922349505,-8.3651238873378,-3.9999999999849));
#28502=CARTESIAN_POINT('',(-18.3844059803083,-7.87485471676291,-3.99999999499105));
#28503=CARTESIAN_POINT('Origin',(0.00282149497308426,0.00106896882069996,
-3.99999999999969));
#28504=CARTESIAN_POINT('',(-18.2865666864733,-7.88496026217301,-3.99999999944013));
#28505=CARTESIAN_POINT('Origin',(-18.8467341402544,-5.50253621564204,-4.00000000000001));
#28506=CARTESIAN_POINT('Origin',(0.,0.,-4.));
#28507=CARTESIAN_POINT('Origin',(0.,24.1327223341711,-4.));
#28508=CARTESIAN_POINT('',(-15.6928377163185,-12.3989743250248,-4.00000000280937));
#28509=CARTESIAN_POINT('',(-15.6550192930802,-12.3081879438969,-3.99999999974395));
#28510=CARTESIAN_POINT('Origin',(-13.4170409317638,-13.8335212840106,-4.));
#28511=CARTESIAN_POINT('',(-14.5823316926435,-13.6877800358225,-3.99999999517897));
#28512=CARTESIAN_POINT('Origin',(0.00228572913896219,0.0019695102302042,
-4.));
#28513=CARTESIAN_POINT('',(-14.4869365434846,-13.6638131244428,-3.99999999943857));
#28514=CARTESIAN_POINT('Ctrl Pts',(-14.4869365436452,-13.6638131238172,
-4.));
#28515=CARTESIAN_POINT('Ctrl Pts',(-14.5027977864062,-13.6678853048282,
-4.));
#28516=CARTESIAN_POINT('Ctrl Pts',(-14.5186699155297,-13.6719162072235,
-4.));
#28517=CARTESIAN_POINT('Ctrl Pts',(-14.5504665592734,-13.6799035971688,
-4.));
#28518=CARTESIAN_POINT('Ctrl Pts',(-14.5663916423942,-13.6838600496388,
-4.));
#28519=CARTESIAN_POINT('Ctrl Pts',(-14.5823265941083,-13.6877752348972,
-4.));
#28520=CARTESIAN_POINT('Origin',(0.,0.,-4.));
#28521=CARTESIAN_POINT('Origin',(0.,24.1327223341711,-4.));
#28522=CARTESIAN_POINT('',(-10.505744825479,-17.0184912834615,-4.00000000280937));
#28523=CARTESIAN_POINT('',(-10.5012771500661,-16.9202333832982,-3.99999999972949));
#28524=CARTESIAN_POINT('Origin',(-8.22961578723204,-17.8253832975409,-4.));
#28525=CARTESIAN_POINT('',(-9.02141300124166,-17.8497570717348,-3.99999999499105));
#28526=CARTESIAN_POINT('Origin',(0.00147427062565764,0.00263249962513257,
-4.));
#28527=CARTESIAN_POINT('',(-8.93996803530948,-17.7946084824175,-3.99999999944011));
#28528=CARTESIAN_POINT('Origin',(-10.9004721713661,-16.3296227715457,-4.));
#28529=CARTESIAN_POINT('Origin',(0.,0.,-4.));
#28530=CARTESIAN_POINT('Origin',(0.,24.1327223341711,-4.));
#28531=CARTESIAN_POINT('',(-4.05150406040619,-19.5853270269313,-4.00000000280937));
#28532=CARTESIAN_POINT('',(-4.08088994023202,-19.4914713868594,-3.99999999974451));
#28533=CARTESIAN_POINT('Origin',(-1.38701078444917,-19.2224432491099,-4.00000000001672));
#28534=CARTESIAN_POINT('',(-2.37237875432574,-19.858789970815,-3.99999999499105));
#28535=CARTESIAN_POINT('Origin',(0.00048499333459795,0.0029779707527644,
-4.));
#28536=CARTESIAN_POINT('',(-2.31470740046595,-19.7791114351774,-3.99999999944107));
#28537=CARTESIAN_POINT('Origin',(-4.65788263325231,-19.073641819594,-3.99999999999017));
#28538=CARTESIAN_POINT('Origin',(0.,0.,-4.));
#28539=CARTESIAN_POINT('Origin',(0.,24.1327223341711,-4.));
#28540=CARTESIAN_POINT('',(2.89140788818329,-19.7898832823108,-4.00000000280937));
#28541=CARTESIAN_POINT('',(2.83169367133745,-19.7117383931695,-3.99999999974453));
#28542=CARTESIAN_POINT('Origin',(5.27108671270436,-18.5376067961811,-4.));
#28543=CARTESIAN_POINT('',(4.5627993829433,-19.4725597148893,-3.99999999499105));
#28544=CARTESIAN_POINT('Origin',(-0.000562781329067619,0.00296425464298977,
-4.));
#28545=CARTESIAN_POINT('',(4.58974103670108,-19.3779616247666,-3.99999999944051));
#28546=CARTESIAN_POINT('Origin',(2.14638847124274,-19.5161339346574,-4.00000000000001));
#28547=CARTESIAN_POINT('Origin',(0.,0.,-4.));
#28548=CARTESIAN_POINT('Origin',(0.,24.1327223341711,-4.));
#28549=CARTESIAN_POINT('',(9.48557337282221,-17.6074875462724,-4.00000000280937));
#28550=CARTESIAN_POINT('',(9.40271337253742,-17.5544894759628,-3.99999999972949));
#28551=CARTESIAN_POINT('Origin',(11.3224256916247,-16.0397541074757,-4.));
#28552=CARTESIAN_POINT('',(10.9476365748824,-16.7376513729739,-3.99999999499105));
#28553=CARTESIAN_POINT('Origin',(-0.00154267623871274,0.00259300562955644,
-4.));
#28554=CARTESIAN_POINT('',(10.9405989708155,-16.639543673871,-3.99999999943993));
#28555=CARTESIAN_POINT('Origin',(8.69154190830326,-17.6048210232288,-3.9999999999849));
#28556=CARTESIAN_POINT('Origin',(0.,0.,-4.));
#28557=CARTESIAN_POINT('Origin',(0.,24.1327223341711,-4.));
#28558=CARTESIAN_POINT('',(14.9356387165454,-13.3013689533132,-4.00000000280937));
#28559=CARTESIAN_POINT('',(14.8396644843238,-13.2798899664757,-3.99999999974396));
#28560=CARTESIAN_POINT('Origin',(15.9531974199694,-10.8110527965528,-4.));
#28561=CARTESIAN_POINT('',(16.0120272253659,-11.9839352483846,-3.99999999517897));
#28562=CARTESIAN_POINT('Origin',(-0.00233650165790245,0.00190900192542198,
-4.));
#28563=CARTESIAN_POINT('',(15.9718469875142,-11.8941676178388,-3.99999999942454));
#28564=CARTESIAN_POINT('Ctrl Pts',(15.9718469869114,-11.8941676181125,-4.));
#28565=CARTESIAN_POINT('Ctrl Pts',(15.978618029634,-11.9090802746427,-4.));
#28566=CARTESIAN_POINT('Ctrl Pts',(15.985348914733,-11.9240113943218,-4.));
#28567=CARTESIAN_POINT('Ctrl Pts',(15.9987405096734,-11.953932543778,-4.));
#28568=CARTESIAN_POINT('Ctrl Pts',(16.0054012593359,-11.9689229988458,-4.));
#28569=CARTESIAN_POINT('Ctrl Pts',(16.0120216120262,-11.9839310609795,-4.));
#28570=CARTESIAN_POINT('Origin',(0.,0.,-4.));
#28571=CARTESIAN_POINT('Origin',(0.,24.1327223341711,-4.));
#28572=CARTESIAN_POINT('',(18.5842456045018,-7.39090895728597,-4.00000000280937));
#28573=CARTESIAN_POINT('',(18.4867046535595,-7.40357147462304,-3.99999999972962));
#28574=CARTESIAN_POINT('Origin',(18.9837728420122,-5.00938144430632,-4.));
#28575=CARTESIAN_POINT('',(19.1451310787574,-5.78477967432897,-3.99999999517897));
#28576=CARTESIAN_POINT('Origin',(-0.0028485105206455,0.0009947444054903,
-4.));
#28577=CARTESIAN_POINT('',(19.0766716890448,-5.71416807437949,-3.9999999994254));
#28578=CARTESIAN_POINT('Ctrl Pts',(19.0766716885727,-5.71416807484213,-4.));
#28579=CARTESIAN_POINT('Ctrl Pts',(19.0881348030286,-5.72586557189522,-4.));
#28580=CARTESIAN_POINT('Ctrl Pts',(19.0995665001737,-5.73759414976848,-4.));
#28581=CARTESIAN_POINT('Ctrl Pts',(19.1223841117608,-5.76113066141302,-4.));
#28582=CARTESIAN_POINT('Ctrl Pts',(19.1337702092287,-5.77293898138808,-4.));
#28583=CARTESIAN_POINT('Ctrl Pts',(19.1451243717667,-5.78477765933064,-4.));
#28584=CARTESIAN_POINT('Origin',(0.,0.,-4.));
#28585=CARTESIAN_POINT('Origin',(0.,19.9140934904867,4.));
#28586=CARTESIAN_POINT('',(19.9099067849541,0.408327476897224,3.99999999942692));
#28587=CARTESIAN_POINT('',(19.9947464642997,0.458076119992405,3.99999999517722));
#28588=CARTESIAN_POINT('Ctrl Pts',(19.9099067846237,0.408327477467692,4.));
#28589=CARTESIAN_POINT('Ctrl Pts',(19.9240789959544,0.416536192806554,4.));
#28590=CARTESIAN_POINT('Ctrl Pts',(19.9382292433099,0.424783246564917,4.));
#28591=CARTESIAN_POINT('Ctrl Pts',(19.9665068467169,0.441366048207167,4.));
#28592=CARTESIAN_POINT('Ctrl Pts',(19.9806344826889,0.449702119578792,4.));
#28593=CARTESIAN_POINT('Ctrl Pts',(19.9947394627542,0.458075970644694,4.));
#28594=CARTESIAN_POINT('',(19.7928724810088,2.19392763772769,3.99999999974475));
#28595=CARTESIAN_POINT('Origin',(0.,0.,4.));
#28596=CARTESIAN_POINT('',(19.8834795218938,2.15568133214589,4.00000000280589));
#28597=CARTESIAN_POINT('Origin',(19.2673652038706,-0.46139871247229,4.));
#28598=CARTESIAN_POINT('Origin',(-0.00301074532259138,-0.000197334674881602,
4.));
#28599=CARTESIAN_POINT('Origin',(0.,19.9140934904867,4.));
#28600=CARTESIAN_POINT('',(18.5695436020587,7.19327254633851,3.99999999943895));
#28601=CARTESIAN_POINT('',(18.6322444467737,7.26905680119529,3.99999999517722));
#28602=CARTESIAN_POINT('Ctrl Pts',(18.5695436015635,7.19327254675251,4.));
#28603=CARTESIAN_POINT('Ctrl Pts',(18.5800475284678,7.20583555504045,4.));
#28604=CARTESIAN_POINT('Ctrl Pts',(18.5905188856696,7.21842615925354,4.));
#28605=CARTESIAN_POINT('Ctrl Pts',(18.6114169918593,7.24368668807207,4.));
#28606=CARTESIAN_POINT('Ctrl Pts',(18.6218439539793,7.25635714098723,4.));
#28607=CARTESIAN_POINT('Ctrl Pts',(18.632237918553,7.26905426618477,4.));
#28608=CARTESIAN_POINT('',(17.8488387931384,8.83119885770583,3.99999999972955));
#28609=CARTESIAN_POINT('Origin',(0.,0.,4.));
#28610=CARTESIAN_POINT('',(17.947072548527,8.82622835625882,4.00000000299381));
#28611=CARTESIAN_POINT('Origin',(18.5321522754301,6.48331038043728,4.));
#28612=CARTESIAN_POINT('Origin',(-0.00276168272250299,-0.00121516948046296,
4.));
#28613=CARTESIAN_POINT('Origin',(0.,19.9140934904867,4.));
#28614=CARTESIAN_POINT('',(14.9894054755396,13.1106385429418,3.99999999942451));
#28615=CARTESIAN_POINT('',(15.0224187663253,13.2032819523213,3.99999999517722));
#28616=CARTESIAN_POINT('Ctrl Pts',(14.9894054749172,13.1106385431674,4.));
#28617=CARTESIAN_POINT('Ctrl Pts',(14.9949856121388,13.1260364783791,4.));
#28618=CARTESIAN_POINT('Ctrl Pts',(15.0005242666941,13.1414496691744,4.));
#28619=CARTESIAN_POINT('Ctrl Pts',(15.0115269942644,13.1723292732651,4.));
#28620=CARTESIAN_POINT('Ctrl Pts',(15.0169910736063,13.1877961136521,4.));
#28621=CARTESIAN_POINT('Ctrl Pts',(15.0224134988291,13.2032773374076,4.));
#28622=CARTESIAN_POINT('',(13.7519742127091,14.4032747936281,3.99999999972944));
#28623=CARTESIAN_POINT('Origin',(0.,0.,4.));
#28624=CARTESIAN_POINT('',(13.8459837511274,14.4322019810711,4.00000000299381));
#28625=CARTESIAN_POINT('Origin',(15.1970464502794,12.4305473706751,4.));
#28626=CARTESIAN_POINT('Origin',(-0.00217952044569536,-0.0020864369252549,
4.));
#28627=CARTESIAN_POINT('Origin',(0.,19.9140934904867,4.));
#28628=CARTESIAN_POINT('',(9.60134920853995,17.4466390141573,3.99999999943866));
#28629=CARTESIAN_POINT('',(9.60066767536943,17.5449964403088,3.99999999517722));
#28630=CARTESIAN_POINT('Ctrl Pts',(9.60134920789419,17.4466390141562,4.));
#28631=CARTESIAN_POINT('Ctrl Pts',(9.60132034098192,17.4630146314442,4.));
#28632=CARTESIAN_POINT('Ctrl Pts',(9.60124878486742,17.4793904530073,4.));
#28633=CARTESIAN_POINT('Ctrl Pts',(9.60102051245635,17.5121741820761,4.));
#28634=CARTESIAN_POINT('Ctrl Pts',(9.6008636198518,17.5285826312153,4.));
#28635=CARTESIAN_POINT('Ctrl Pts',(9.6006643039356,17.5449903021187,4.));
#28636=CARTESIAN_POINT('',(7.99641856994512,18.2381032342188,3.99999999972954));
#28637=CARTESIAN_POINT('Origin',(0.,0.,4.));
#28638=CARTESIAN_POINT('',(8.07486496484469,18.2974390476607,4.00000000280589));
#28639=CARTESIAN_POINT('Origin',(10.0290598294463,16.8787298443224,3.99999999999999));
#28640=CARTESIAN_POINT('Origin',(-0.00133447584031332,-0.00270604931077445,
4.));
#28641=CARTESIAN_POINT('Origin',(0.,19.9140934904867,4.));
#28642=CARTESIAN_POINT('',(3.05519487166812,19.6783359004266,3.99999999942581));
#28643=CARTESIAN_POINT('',(3.02093437199968,19.7705254210252,3.99999999517722));
#28644=CARTESIAN_POINT('Ctrl Pts',(3.05519487104775,19.6783359001999,4.));
#28645=CARTESIAN_POINT('Ctrl Pts',(3.0495718701275,19.6937182385374,4.));
#28646=CARTESIAN_POINT('Ctrl Pts',(3.04390729298132,19.7090856016079,4.));
#28647=CARTESIAN_POINT('Ctrl Pts',(3.03248680703719,19.739813173271,4.));
#28648=CARTESIAN_POINT('Ctrl Pts',(3.02673062840326,19.755173713429,4.));
#28649=CARTESIAN_POINT('Ctrl Pts',(3.02093330327285,19.770518499915,4.));
#28650=CARTESIAN_POINT('',(1.27637679137333,19.873147254883,3.99999999973));
#28651=CARTESIAN_POINT('Origin',(0.,0.,4.));
#28652=CARTESIAN_POINT('',(1.32979829814077,19.9557349287161,4.0000000029938));
#28653=CARTESIAN_POINT('Origin',(3.6511832014166,19.2915843141947,4.));
#28654=CARTESIAN_POINT('Origin',(-0.000328473722452371,-0.00299927214920226,
4.));
#28655=CARTESIAN_POINT('Origin',(0.,19.9140934904867,4.));
#28656=CARTESIAN_POINT('',(-3.85944318620814,19.5365252234455,3.99999999942585));
#28657=CARTESIAN_POINT('',(-3.92316820087621,19.6114372540864,3.99999999517722));
#28658=CARTESIAN_POINT('Ctrl Pts',(-3.8594431867135,19.5365252230202,4.));
#28659=CARTESIAN_POINT('Ctrl Pts',(-3.86998814946638,19.5490567127974,4.));
#28660=CARTESIAN_POINT('Ctrl Pts',(-3.88056705909194,19.5615599106554,4.));
#28661=CARTESIAN_POINT('Ctrl Pts',(-3.90180825488829,19.5865283465661,4.));
#28662=CARTESIAN_POINT('Ctrl Pts',(-3.91247090803087,19.5989938039058,4.));
#28663=CARTESIAN_POINT('Ctrl Pts',(-3.92316683799181,19.611430384844,4.));
#28664=CARTESIAN_POINT('',(-5.59761479267543,19.1111964084047,3.99999999972973));
#28665=CARTESIAN_POINT('Origin',(0.,0.,4.));
#28666=CARTESIAN_POINT('',(-5.57566167259198,19.2070746593985,4.00000000299381));
#28667=CARTESIAN_POINT('Origin',(-3.16690114173538,19.3766326568612,4.));
#28668=CARTESIAN_POINT('Origin',(0.000717147159679521,-0.00293073854793047,
4.));
#28669=CARTESIAN_POINT('Origin',(0.,19.9140934904867,4.));
#28670=CARTESIAN_POINT('',(-10.3085579923323,17.0383318324703,3.99999999943867));
#28671=CARTESIAN_POINT('',(-10.3940787889303,17.0869203203164,3.99999999517722));
#28672=CARTESIAN_POINT('Ctrl Pts',(-10.3085579926542,17.0383318319105,4.));
#28673=CARTESIAN_POINT('Ctrl Pts',(-10.3227541267253,17.0464946409769,4.));
#28674=CARTESIAN_POINT('Ctrl Pts',(-10.3369717822929,17.0546205822697,4.));
#28675=CARTESIAN_POINT('Ctrl Pts',(-10.3654774608083,17.0708147570336,4.));
#28676=CARTESIAN_POINT('Ctrl Pts',(-10.379766040979,17.0788831086342,4.));
#28677=CARTESIAN_POINT('Ctrl Pts',(-10.3940751588187,17.086914331474,4.));
#28678=CARTESIAN_POINT('',(-11.7964514251346,16.0441532435407,3.99999999972946));
#28679=CARTESIAN_POINT('Origin',(0.,0.,4.));
#28680=CARTESIAN_POINT('',(-11.8086145576078,16.1417577199254,4.00000000299381));
#28681=CARTESIAN_POINT('Origin',(-9.60276988745231,17.1247213783635,4.));
#28682=CARTESIAN_POINT('Origin',(0.00167626948831101,-0.00250871457599722,
4.));
#28683=CARTESIAN_POINT('Origin',(0.,19.9140934904867,4.));
#28684=CARTESIAN_POINT('',(-15.5143414292227,12.4850442342554,3.9999999994245));
#28685=CARTESIAN_POINT('',(-15.611310074774,12.5014686198299,3.99999999517722));
#28686=CARTESIAN_POINT('Ctrl Pts',(-15.5143414293368,12.4850442336032,4.));
#28687=CARTESIAN_POINT('Ctrl Pts',(-15.5304744159661,12.4878657726368,4.));
#28688=CARTESIAN_POINT('Ctrl Pts',(-15.546615223024,12.4906438101088,4.));
#28689=CARTESIAN_POINT('Ctrl Pts',(-15.5789363001155,12.4961171945695,4.));
#28690=CARTESIAN_POINT('Ctrl Pts',(-15.5951169918514,12.4988124736256,4.));
#28691=CARTESIAN_POINT('Ctrl Pts',(-15.6113046152802,12.5014642337302,4.));
#28692=CARTESIAN_POINT('',(-16.5724619474212,11.0419484027528,3.99999999972945));
#28693=CARTESIAN_POINT('Origin',(0.,0.,4.));
#28694=CARTESIAN_POINT('',(-16.6172742483527,11.1295065685037,4.00000000280589));
#28695=CARTESIAN_POINT('Origin',(-14.8806548824468,12.8076250541992,4.));
#28696=CARTESIAN_POINT('Origin',(0.00243320901777366,-0.00178410266734153,
4.));
#28697=CARTESIAN_POINT('Origin',(0.,19.9140934904867,4.));
#28698=CARTESIAN_POINT('',(-18.8488487596698,6.42588670526778,3.99999999942508));
#28699=CARTESIAN_POINT('',(-18.9455869672014,6.40815530176509,3.99999999517722));
#28700=CARTESIAN_POINT('Ctrl Pts',(-18.8488487595541,6.42588670461663,4.));
#28701=CARTESIAN_POINT('Ctrl Pts',(-18.864973830457,6.42302026310499,4.));
#28702=CARTESIAN_POINT('Ctrl Pts',(-18.8810913724055,6.42011027220655,4.));
#28703=CARTESIAN_POINT('Ctrl Pts',(-18.913335263081,6.41419909595026,4.));
#28704=CARTESIAN_POINT('Ctrl Pts',(-18.9294619849968,6.41119770248451,4.));
#28705=CARTESIAN_POINT('Ctrl Pts',(-18.9455803368209,6.40815304743644,4.));
#28706=CARTESIAN_POINT('',(-19.3495889823633,4.70792159465315,3.99999999972972));
#28707=CARTESIAN_POINT('Origin',(0.,0.,4.));
#28708=CARTESIAN_POINT('',(-19.4216454237194,4.77487267832733,4.00000000299381));
#28709=CARTESIAN_POINT('Origin',(-18.3640870092082,6.94570038752625,4.));
#28710=CARTESIAN_POINT('Origin',(0.00289666758562568,-0.000844301606275355,
4.));
#28711=CARTESIAN_POINT('Origin',(0.,19.9140934904867,4.));
#28712=CARTESIAN_POINT('',(-19.9099067849541,-0.408327476897221,3.99999999942691));
#28713=CARTESIAN_POINT('',(-19.9947464642997,-0.458076119992403,3.99999999517722));
#28714=CARTESIAN_POINT('Ctrl Pts',(-19.9099067846237,-0.408327477467691,
4.));
#28715=CARTESIAN_POINT('Ctrl Pts',(-19.9240789959545,-0.416536192806615,
4.));
#28716=CARTESIAN_POINT('Ctrl Pts',(-19.9382292433101,-0.424783246565044,
4.));
#28717=CARTESIAN_POINT('Ctrl Pts',(-19.9665068467166,-0.441366048206973,
4.));
#28718=CARTESIAN_POINT('Ctrl Pts',(-19.9806344826885,-0.449702119578518,
4.));
#28719=CARTESIAN_POINT('Ctrl Pts',(-19.9947394627542,-0.458075970644692,
4.));
#28720=CARTESIAN_POINT('',(-19.7928699969466,-2.19395004769781,3.99999999973002));
#28721=CARTESIAN_POINT('Origin',(0.,0.,4.));
#28722=CARTESIAN_POINT('',(-19.8834795259929,-2.15568133042439,4.0000000029938));
#28723=CARTESIAN_POINT('Origin',(-19.6325516134049,0.245736990623587,4.));
#28724=CARTESIAN_POINT('Origin',(0.00301074532257362,0.000197334674880076,
4.));
#28725=CARTESIAN_POINT('Origin',(0.,19.9140934904867,4.));
#28726=CARTESIAN_POINT('',(-18.5695436020587,-7.19327254633852,3.99999999943895));
#28727=CARTESIAN_POINT('',(-18.6322444467737,-7.26905680119529,3.99999999517722));
#28728=CARTESIAN_POINT('Ctrl Pts',(-18.5695436015635,-7.19327254675251,
4.));
#28729=CARTESIAN_POINT('Ctrl Pts',(-18.5800475284678,-7.20583555504053,
4.));
#28730=CARTESIAN_POINT('Ctrl Pts',(-18.5905188856698,-7.2184261592537,4.));
#28731=CARTESIAN_POINT('Ctrl Pts',(-18.6114169918594,-7.24368668807219,
4.));
#28732=CARTESIAN_POINT('Ctrl Pts',(-18.6218439539793,-7.25635714098729,
4.));
#28733=CARTESIAN_POINT('Ctrl Pts',(-18.632237918553,-7.26905426618477,4.));
#28734=CARTESIAN_POINT('',(-17.8488387931384,-8.83119885770584,3.99999999972955));
#28735=CARTESIAN_POINT('Origin',(0.,0.,4.));
#28736=CARTESIAN_POINT('',(-17.947072548527,-8.82622835625882,4.00000000299381));
#28737=CARTESIAN_POINT('Origin',(-18.5321530186718,-6.48330768932856,4.0000000000151));
#28738=CARTESIAN_POINT('Origin',(0.00276168272122623,0.0012151694794782,
4.));
#28739=CARTESIAN_POINT('Origin',(0.,19.9140934904867,4.));
#28740=CARTESIAN_POINT('',(-14.9894054755396,-13.1106385429418,3.9999999994245));
#28741=CARTESIAN_POINT('',(-15.0224187663253,-13.2032819523213,3.99999999517722));
#28742=CARTESIAN_POINT('Ctrl Pts',(-14.9894054749172,-13.1106385431674,
4.));
#28743=CARTESIAN_POINT('Ctrl Pts',(-14.9949856121388,-13.1260364783793,
4.));
#28744=CARTESIAN_POINT('Ctrl Pts',(-15.0005242666942,-13.1414496691749,
4.));
#28745=CARTESIAN_POINT('Ctrl Pts',(-15.0115269942646,-13.1723292732657,
4.));
#28746=CARTESIAN_POINT('Ctrl Pts',(-15.0169910736066,-13.1877961136528,
4.));
#28747=CARTESIAN_POINT('Ctrl Pts',(-15.0224134988291,-13.2032773374076,
4.));
#28748=CARTESIAN_POINT('',(-13.751974212639,-14.403274793695,3.99999999972944));
#28749=CARTESIAN_POINT('Origin',(0.,0.,4.));
#28750=CARTESIAN_POINT('',(-13.8459837468808,-14.4322019797551,4.00000000280589));
#28751=CARTESIAN_POINT('Origin',(-15.1970434703156,-12.4305516593735,4.));
#28752=CARTESIAN_POINT('Origin',(0.00217952044569536,0.0020864369252549,
4.));
#28753=CARTESIAN_POINT('Origin',(0.,19.9140934904867,4.));
#28754=CARTESIAN_POINT('',(-9.60134920853987,-17.4466390141574,3.99999999943866));
#28755=CARTESIAN_POINT('',(-9.60066767536943,-17.5449964403088,3.99999999517722));
#28756=CARTESIAN_POINT('Ctrl Pts',(-9.60134920789411,-17.4466390141562,
4.));
#28757=CARTESIAN_POINT('Ctrl Pts',(-9.60132034098186,-17.4630146314438,
4.));
#28758=CARTESIAN_POINT('Ctrl Pts',(-9.60124878486737,-17.4793904530065,
4.));
#28759=CARTESIAN_POINT('Ctrl Pts',(-9.60102051245632,-17.5121741820764,
4.));
#28760=CARTESIAN_POINT('Ctrl Pts',(-9.60086361985177,-17.5285826312158,
4.));
#28761=CARTESIAN_POINT('Ctrl Pts',(-9.6006643039356,-17.5449903021187,4.));
#28762=CARTESIAN_POINT('',(-7.99641857003384,-18.2381032341799,3.99999999972955));
#28763=CARTESIAN_POINT('Origin',(0.,0.,4.));
#28764=CARTESIAN_POINT('',(-8.07486496838508,-18.2974390503498,4.0000000029938));
#28765=CARTESIAN_POINT('Origin',(-10.0290617346374,-16.8787286365668,4.00000000001511));
#28766=CARTESIAN_POINT('Origin',(0.00133447584018453,0.00270604930997509,
4.));
#28767=CARTESIAN_POINT('Origin',(0.,19.9140934904867,4.));
#28768=CARTESIAN_POINT('',(-3.05519487166813,-19.6783359004266,3.99999999942581));
#28769=CARTESIAN_POINT('',(-3.02093437199967,-19.7705254210252,3.99999999517722));
#28770=CARTESIAN_POINT('Ctrl Pts',(-3.05519487104776,-19.6783359001999,
4.));
#28771=CARTESIAN_POINT('Ctrl Pts',(-3.04957187012752,-19.6937182385374,
4.));
#28772=CARTESIAN_POINT('Ctrl Pts',(-3.04390729298135,-19.7090856016078,
4.));
#28773=CARTESIAN_POINT('Ctrl Pts',(-3.03248680703726,-19.7398131732708,
4.));
#28774=CARTESIAN_POINT('Ctrl Pts',(-3.02673062840331,-19.7551737134288,
4.));
#28775=CARTESIAN_POINT('Ctrl Pts',(-3.02093330327284,-19.770518499915,4.));
#28776=CARTESIAN_POINT('',(-1.27637679137335,-19.873147254883,3.99999999973));
#28777=CARTESIAN_POINT('Origin',(0.,0.,4.));
#28778=CARTESIAN_POINT('',(-1.32979829814076,-19.9557349287161,4.0000000029938));
#28779=CARTESIAN_POINT('Origin',(-3.65116939301718,-19.2915880101181,3.9999999999849));
#28780=CARTESIAN_POINT('Origin',(0.000328473722462364,0.00299927214920226,
4.));
#28781=CARTESIAN_POINT('Origin',(0.,19.9140934904867,4.));
#28782=CARTESIAN_POINT('',(3.85944318620815,-19.5365252234455,3.99999999942585));
#28783=CARTESIAN_POINT('',(3.92316820087621,-19.6114372540864,3.99999999517722));
#28784=CARTESIAN_POINT('Ctrl Pts',(3.85944318671351,-19.5365252230202,4.));
#28785=CARTESIAN_POINT('Ctrl Pts',(3.86998814946643,-19.5490567127974,4.));
#28786=CARTESIAN_POINT('Ctrl Pts',(3.88056705909203,-19.5615599106555,4.));
#28787=CARTESIAN_POINT('Ctrl Pts',(3.9018082548882,-19.5865283465659,4.));
#28788=CARTESIAN_POINT('Ctrl Pts',(3.91247090803083,-19.5989938039058,4.));
#28789=CARTESIAN_POINT('Ctrl Pts',(3.92316683799182,-19.6114303848441,4.));
#28790=CARTESIAN_POINT('',(5.59761479267544,-19.1111964084047,3.99999999972974));
#28791=CARTESIAN_POINT('Origin',(0.,0.,4.));
#28792=CARTESIAN_POINT('',(5.57566167259198,-19.2070746593985,4.00000000299381));
#28793=CARTESIAN_POINT('Origin',(3.16689861973229,-19.3766328787332,4.00000000000001));
#28794=CARTESIAN_POINT('Origin',(-0.000717147160155251,0.00293073854892079,
4.));
#28795=CARTESIAN_POINT('Origin',(0.,19.9140934904867,4.));
#28796=CARTESIAN_POINT('',(10.3085579923322,-17.0383318324703,3.99999999943867));
#28797=CARTESIAN_POINT('',(10.3940787889303,-17.0869203203164,3.99999999517722));
#28798=CARTESIAN_POINT('Ctrl Pts',(10.3085579926541,-17.0383318319105,4.));
#28799=CARTESIAN_POINT('Ctrl Pts',(10.3227541267254,-17.046494640977,4.));
#28800=CARTESIAN_POINT('Ctrl Pts',(10.336971782293,-17.0546205822698,4.));
#28801=CARTESIAN_POINT('Ctrl Pts',(10.3654774608076,-17.0708147570333,4.));
#28802=CARTESIAN_POINT('Ctrl Pts',(10.3797660409782,-17.0788831086338,4.));
#28803=CARTESIAN_POINT('Ctrl Pts',(10.3940751588187,-17.086914331474,4.));
#28804=CARTESIAN_POINT('',(11.7964514251347,-16.0441532435407,3.99999999972945));
#28805=CARTESIAN_POINT('Origin',(0.,0.,4.));
#28806=CARTESIAN_POINT('',(11.8086145576078,-16.1417577199254,4.0000000029938));
#28807=CARTESIAN_POINT('Origin',(9.60277970218749,-17.1247167460198,3.9999999999849));
#28808=CARTESIAN_POINT('Origin',(-0.00167626950157151,0.00250871459651858,
4.));
#28809=CARTESIAN_POINT('Origin',(0.,19.9140934904867,4.));
#28810=CARTESIAN_POINT('',(15.5143414292227,-12.4850442342554,3.9999999994245));
#28811=CARTESIAN_POINT('',(15.611310074774,-12.5014686198299,3.99999999517722));
#28812=CARTESIAN_POINT('Ctrl Pts',(15.5143414293368,-12.4850442336032,4.));
#28813=CARTESIAN_POINT('Ctrl Pts',(15.5304744159665,-12.4878657726369,4.));
#28814=CARTESIAN_POINT('Ctrl Pts',(15.5466152230249,-12.4906438101089,4.));
#28815=CARTESIAN_POINT('Ctrl Pts',(15.5789363001168,-12.4961171945697,4.));
#28816=CARTESIAN_POINT('Ctrl Pts',(15.5951169918525,-12.4988124736257,4.));
#28817=CARTESIAN_POINT('Ctrl Pts',(15.6113046152802,-12.5014642337302,4.));
#28818=CARTESIAN_POINT('',(16.5724493912922,-11.0419672478261,3.99999999974397));
#28819=CARTESIAN_POINT('Origin',(0.,0.,4.));
#28820=CARTESIAN_POINT('',(16.6172742483527,-11.1295065685037,4.00000000280589));
#28821=CARTESIAN_POINT('Origin',(14.4611068945492,-12.7381772024518,4.));
#28822=CARTESIAN_POINT('Origin',(-0.00243320901777366,0.00178410266734153,
4.));
#28823=CARTESIAN_POINT('Origin',(0.,19.9140934904867,4.));
#28824=CARTESIAN_POINT('',(18.8488421537318,-6.42590608228654,3.99999999943894));
#28825=CARTESIAN_POINT('',(18.9455869672014,-6.4081553017651,3.99999999517722));
#28826=CARTESIAN_POINT('Ctrl Pts',(18.8488421536186,-6.42590608165111,4.));
#28827=CARTESIAN_POINT('Ctrl Pts',(18.8649639745842,-6.42303405323124,4.));
#28828=CARTESIAN_POINT('Ctrl Pts',(18.881078584019,-6.4201199496557,4.));
#28829=CARTESIAN_POINT('Ctrl Pts',(18.9133246169989,-6.41420230587836,4.));
#28830=CARTESIAN_POINT('Ctrl Pts',(18.929456543401,-6.41119849796776,4.));
#28831=CARTESIAN_POINT('Ctrl Pts',(18.9455803368209,-6.40815304743646,4.));
#28832=CARTESIAN_POINT('',(19.3495836396352,-4.70794355337793,3.99999999974434));
#28833=CARTESIAN_POINT('Origin',(0.,0.,4.));
#28834=CARTESIAN_POINT('',(19.4216454204563,-4.77487267530771,4.00000000280589));
#28835=CARTESIAN_POINT('Origin',(17.9465883718404,-7.02371079670489,3.99999999998329));
#28836=CARTESIAN_POINT('Origin',(-0.00289666758440221,0.000844301606205411,
4.));
#28837=CARTESIAN_POINT('Origin',(0.,0.,-1.52655665885959E-15));
#28838=CARTESIAN_POINT('Ctrl Pts',(19.9039912380639,-0.634233661349708,
-3.99999999959214));
#28839=CARTESIAN_POINT('Ctrl Pts',(19.6812984735891,-0.667619141633003,
-3.37209215899804));
#28840=CARTESIAN_POINT('Ctrl Pts',(19.5117100620297,-0.663422606908006,
-2.72442970848406));
#28841=CARTESIAN_POINT('Ctrl Pts',(19.3267092023989,-0.612554982700328,
-1.65557386075461));
#28842=CARTESIAN_POINT('Ctrl Pts',(19.2773785775181,-0.58222314238337,-1.2405673563286));
#28843=CARTESIAN_POINT('Ctrl Pts',(19.2307632060366,-0.514706825018647,
-0.535449716754467));
#28844=CARTESIAN_POINT('Ctrl Pts',(19.2222233880155,-0.482364065768703,
-0.245612043957726));
#28845=CARTESIAN_POINT('Ctrl Pts',(19.2260726306592,-0.407801406965312,
0.339574192499094));
#28846=CARTESIAN_POINT('Ctrl Pts',(19.2389599748712,-0.365366877207829,
0.634888638796465));
#28847=CARTESIAN_POINT('Ctrl Pts',(19.2983007127951,-0.246059610097558,
1.3754102996081));
#28848=CARTESIAN_POINT('Ctrl Pts',(19.3587572800291,-0.16286451845944,1.81818944950897));
#28849=CARTESIAN_POINT('Ctrl Pts',(19.5571030357013,0.0653676913969697,
2.85334850598286));
#28850=CARTESIAN_POINT('Ctrl Pts',(19.7151513706548,0.22131331524976,3.43719532452554));
#28851=CARTESIAN_POINT('Ctrl Pts',(19.9099067854224,0.408327477794068,3.99999999896687));
#28852=CARTESIAN_POINT('Ctrl Pts',(19.7928724813984,2.19392763718696,3.99999999959177));
#28853=CARTESIAN_POINT('Ctrl Pts',(19.568248154273,2.20973759437162,3.37209584227646));
#28854=CARTESIAN_POINT('Ctrl Pts',(19.3995124415109,2.19224756440723,2.72443686861351));
#28855=CARTESIAN_POINT('Ctrl Pts',(19.2190722839147,2.12702120186606,1.65558298745174));
#28856=CARTESIAN_POINT('Ctrl Pts',(19.1722730539926,2.09291204321717,1.24057456625547));
#28857=CARTESIAN_POINT('Ctrl Pts',(19.1310981391587,2.02194588750386,0.535453312298503));
#28858=CARTESIAN_POINT('Ctrl Pts',(19.1251221278395,1.98903256836499,0.245613912296371));
#28859=CARTESIAN_POINT('Ctrl Pts',(19.1348096591669,1.91500135462234,-0.339575749237676));
#28860=CARTESIAN_POINT('Ctrl Pts',(19.1509867906522,1.87370858720253,-0.634891908540389));
#28861=CARTESIAN_POINT('Ctrl Pts',(19.2195059168057,1.75942465784691,-1.37541694661038));
#28862=CARTESIAN_POINT('Ctrl Pts',(19.2863040300092,1.68122936510914,-1.81819780767567));
#28863=CARTESIAN_POINT('Ctrl Pts',(19.5019456671156,1.46926376538599,-2.85335500863366));
#28864=CARTESIAN_POINT('Ctrl Pts',(19.6717414173474,1.32620060584982,-3.4371986138663));
#28865=CARTESIAN_POINT('Ctrl Pts',(19.8805681948062,1.15504449480289,-3.99999999896589));
#28866=CARTESIAN_POINT('Origin',(0.,0.,-1.52655665885959E-15));
#28867=CARTESIAN_POINT('Ctrl Pts',(18.9205613831265,6.21155990787279,-3.9999999995661));
#28868=CARTESIAN_POINT('Ctrl Pts',(18.722324530204,6.10368372785984,-3.37073547207111));
#28869=CARTESIAN_POINT('Ctrl Pts',(18.5614565921267,6.04926209466265,-2.72191645121725));
#28870=CARTESIAN_POINT('Ctrl Pts',(18.3705057444971,6.03370239487818,-1.65243153944395));
#28871=CARTESIAN_POINT('Ctrl Pts',(18.3139896008122,6.04528699644631,-1.23816612795984));
#28872=CARTESIAN_POINT('Ctrl Pts',(18.247326598681,6.09268509358316,-0.534322227019105));
#28873=CARTESIAN_POINT('Ctrl Pts',(18.2282992017452,6.12010477942619,-0.245020449800811));
#28874=CARTESIAN_POINT('Ctrl Pts',(18.2064590003793,6.19136501242513,0.339092780639954));
#28875=CARTESIAN_POINT('Ctrl Pts',(18.2040399950647,6.23557815835783,0.633871337552541));
#28876=CARTESIAN_POINT('Ctrl Pts',(18.2188652552579,6.36780451907379,1.37316141097512));
#28877=CARTESIAN_POINT('Ctrl Pts',(18.2470631112819,6.46654273341169,1.81522672164396));
#28878=CARTESIAN_POINT('Ctrl Pts',(18.3550861881491,6.74910453149341,2.85098957620195));
#28879=CARTESIAN_POINT('Ctrl Pts',(18.4502683407472,6.9503037778164,3.43595659389031));
#28880=CARTESIAN_POINT('Ctrl Pts',(18.5695436021889,7.1932725473206,3.99999999898836));
#28881=CARTESIAN_POINT('Ctrl Pts',(17.8488387937264,8.83119885730777,3.99999999956597));
#28882=CARTESIAN_POINT('Ctrl Pts',(17.6318350798684,8.76919556450322,3.37073606763092));
#28883=CARTESIAN_POINT('Ctrl Pts',(17.4789514598686,8.69525791381623,2.72191758661121));
#28884=CARTESIAN_POINT('Ctrl Pts',(17.3318496791326,8.57251654264658,1.65243297598597));
#28885=CARTESIAN_POINT('Ctrl Pts',(17.299659216222,8.52464104899507,1.23816724736839));
#28886=CARTESIAN_POINT('Ctrl Pts',(17.2853335211168,8.44410950932137,0.534322772007183));
#28887=CARTESIAN_POINT('Ctrl Pts',(17.290980930954,8.41121588890205,0.245020734146467));
#28888=CARTESIAN_POINT('Ctrl Pts',(17.3253503814398,8.34508143893279,-0.339093015441015));
#28889=CARTESIAN_POINT('Ctrl Pts',(17.3546144576286,8.31185087091933,-0.633871831961161));
#28890=CARTESIAN_POINT('Ctrl Pts',(17.4578673627717,8.22793150916394,-1.37316245063156));
#28891=CARTESIAN_POINT('Ctrl Pts',(17.5471861070962,8.17727058957665,-1.81522805453279));
#28892=CARTESIAN_POINT('Ctrl Pts',(17.8222838092634,8.05144781005231,-2.85099062303143));
#28893=CARTESIAN_POINT('Ctrl Pts',(18.0311947505155,7.97465658921816,-3.43595713130924));
#28894=CARTESIAN_POINT('Ctrl Pts',(18.2865666872494,7.88496026156532,-3.9999999989921));
#28895=CARTESIAN_POINT('Origin',(0.,0.,-1.52655665885959E-15));
#28896=CARTESIAN_POINT('Ctrl Pts',(15.6550192929788,12.3081879445576,-3.9999999995905));
#28897=CARTESIAN_POINT('Ctrl Pts',(15.5058897133034,12.1394742461233,-3.37210842589158));
#28898=CARTESIAN_POINT('Ctrl Pts',(15.3732799472876,12.0336838212003,-2.72446133399751));
#28899=CARTESIAN_POINT('Ctrl Pts',(15.1988603399475,11.9537342169491,-1.65561417383655));
#28900=CARTESIAN_POINT('Ctrl Pts',(15.1415712421423,11.9452603559541,-1.24059920501932));
#28901=CARTESIAN_POINT('Ctrl Pts',(15.0624597690905,11.9670172783189,-0.535465601249687));
#28902=CARTESIAN_POINT('Ctrl Pts',(15.0351273125387,11.9863044050078,-0.245620297792711));
#28903=CARTESIAN_POINT('Ctrl Pts',(14.9901468786545,12.0458983790383,0.339581070069207));
#28904=CARTESIAN_POINT('Ctrl Pts',(14.9727426549031,12.086689935466,0.634903084117227));
#28905=CARTESIAN_POINT('Ctrl Pts',(14.9415120504097,12.2162307198855,1.3754396605205));
#28906=CARTESIAN_POINT('Ctrl Pts',(14.9343491772112,12.318824241377,1.81822636537783));
#28907=CARTESIAN_POINT('Ctrl Pts',(14.9395904852342,12.6211525532081,2.85337722509545));
#28908=CARTESIAN_POINT('Ctrl Pts',(14.9604246816766,12.8421986625435,3.43720985077337));
#28909=CARTESIAN_POINT('Ctrl Pts',(14.9894054753209,13.110638543934,3.99999999896253));
#28910=CARTESIAN_POINT('Ctrl Pts',(13.7519742133981,14.4032747934551,3.99999999956581));
#28911=CARTESIAN_POINT('Ctrl Pts',(13.5692640754011,14.2707912447614,3.3707368720194));
#28912=CARTESIAN_POINT('Ctrl Pts',(13.4508888400675,14.1490232672934,2.72191911983545));
#28913=CARTESIAN_POINT('Ctrl Pts',(13.3546383747822,13.9833721569018,1.65243491602215));
#28914=CARTESIAN_POINT('Ctrl Pts',(13.3407635890821,13.9273739927272,1.23816875923414));
#28915=CARTESIAN_POINT('Ctrl Pts',(13.3548452424663,13.8467992629272,0.534323508198989));
#28916=CARTESIAN_POINT('Ctrl Pts',(13.3714023670614,13.8178208485285,0.245021118273289));
#28917=CARTESIAN_POINT('Ctrl Pts',(13.426318460135,13.7674297777744,-0.339093332539267));
#28918=CARTESIAN_POINT('Ctrl Pts',(13.4651832658699,13.7462121517018,-0.633872499721225));
#28919=CARTESIAN_POINT('Ctrl Pts',(13.5909115042562,13.7026683504298,-1.37316385456509));
#28920=CARTESIAN_POINT('Ctrl Pts',(13.6921708194976,13.6856115280933,-1.81522985428248));
#28921=CARTESIAN_POINT('Ctrl Pts',(13.9937119595891,13.6614659735749,-2.850992036466));
#28922=CARTESIAN_POINT('Ctrl Pts',(14.2162878528165,13.6607577213958,-3.43595785705526));
#28923=CARTESIAN_POINT('Ctrl Pts',(14.4869365444979,13.6638131240649,-3.99999999899171));
#28924=CARTESIAN_POINT('Origin',(0.,0.,-1.52655665885959E-15));
#28925=CARTESIAN_POINT('Ctrl Pts',(10.5012771497263,16.9202333839218,-3.99999999956587));
#28926=CARTESIAN_POINT('Ctrl Pts',(10.4187604568623,16.7101716410052,-3.37073654282549));
#28927=CARTESIAN_POINT('Ctrl Pts',(10.3305099036439,16.5650785907123,-2.72191849209908));
#28928=CARTESIAN_POINT('Ctrl Pts',(10.1942344309634,16.4304182339908,-1.652434121808));
#28929=CARTESIAN_POINT('Ctrl Pts',(10.143493957598,16.4029645969779,-1.23816814035234));
#28930=CARTESIAN_POINT('Ctrl Pts',(10.0619600213757,16.396423433878,-0.534323206889723));
#28931=CARTESIAN_POINT('Ctrl Pts',(10.0297590861831,16.4051975588644,-0.245020961051929));
#28932=CARTESIAN_POINT('Ctrl Pts',(9.96722322846384,16.4457475107094,0.339093202773109));
#28933=CARTESIAN_POINT('Ctrl Pts',(9.93695047231674,16.4780618942998,0.633872226446596));
#28934=CARTESIAN_POINT('Ctrl Pts',(9.86331380879727,16.5888828385059,1.37316327986747));
#28935=CARTESIAN_POINT('Ctrl Pts',(9.82144696476986,16.6826460743351,1.81522911749121));
#28936=CARTESIAN_POINT('Ctrl Pts',(9.72257053472987,16.968536856076,2.85099145780179));
#28937=CARTESIAN_POINT('Ctrl Pts',(9.66615620033031,17.1838459623933,3.43595756003759));
#28938=CARTESIAN_POINT('Ctrl Pts',(9.60134920800818,17.4466390149938,3.99999999898783));
#28939=CARTESIAN_POINT('Ctrl Pts',(7.9964185706515,18.2381032342919,3.99999999956596));
#28940=CARTESIAN_POINT('Ctrl Pts',(7.87003904657797,18.0511186748182,3.37073613064603));
#28941=CARTESIAN_POINT('Ctrl Pts',(7.80044962132109,17.8962074545261,2.72191770646729));
#28942=CARTESIAN_POINT('Ctrl Pts',(7.76665975518057,17.7076268932318,1.65243312773053));
#28943=CARTESIAN_POINT('Ctrl Pts',(7.77277420554943,17.6502604963407,1.23816736568045));
#28944=CARTESIAN_POINT('Ctrl Pts',(7.81356476628747,17.5793613666168,0.534322829701268));
#28945=CARTESIAN_POINT('Ctrl Pts',(7.83903454727416,17.5577934732534,0.245020764278644));
#28946=CARTESIAN_POINT('Ctrl Pts',(7.90787348487,17.5292237994333,-0.339093040194778));
#28947=CARTESIAN_POINT('Ctrl Pts',(7.95165126879749,17.5225782935396,-0.633871884162621));
#28948=CARTESIAN_POINT('Ctrl Pts',(8.08468991779793,17.5246620267298,-1.37316256028439));
#28949=CARTESIAN_POINT('Ctrl Pts',(8.18567626219244,17.5432664999848,-1.81522819503422));
#28950=CARTESIAN_POINT('Ctrl Pts',(8.47729064067002,17.6237100684105,-2.85099073335041));
#28951=CARTESIAN_POINT('Ctrl Pts',(8.68668612406968,17.699169946924,-3.43595718806009));
#28952=CARTESIAN_POINT('Ctrl Pts',(8.93996803620397,17.7946084824949,-3.99999999898803));
#28953=CARTESIAN_POINT('Origin',(0.,0.,-1.52655665885959E-15));
#28954=CARTESIAN_POINT('Ctrl Pts',(4.08088993973065,19.4914713872994,-3.99999999959139));
#28955=CARTESIAN_POINT('Ctrl Pts',(4.07509761685323,19.2663672599298,-3.37209958171796));
#28956=CARTESIAN_POINT('Ctrl Pts',(4.0415148849561,19.1000854490341,-2.72444413839122));
#28957=CARTESIAN_POINT('Ctrl Pts',(3.95929377670302,18.9267270968025,-1.65559225411347));
#28958=CARTESIAN_POINT('Ctrl Pts',(3.92085570624596,18.8834120879112,-1.24058188703958));
#28959=CARTESIAN_POINT('Ctrl Pts',(3.84626919931116,18.8492280764774,-0.535456963378757));
#28960=CARTESIAN_POINT('Ctrl Pts',(3.81293438334342,18.8464340988294,-0.245615809484055));
#28961=CARTESIAN_POINT('Ctrl Pts',(3.74017208754659,18.8631726846676,0.339577330001301));
#28962=CARTESIAN_POINT('Ctrl Pts',(3.70061976633521,18.8832332349204,0.634895228749923));
#28963=CARTESIAN_POINT('Ctrl Pts',(3.59342903056888,18.9623911496099,1.37542369557564));
#28964=CARTESIAN_POINT('Ctrl Pts',(3.52199606603956,19.0363769342805,1.81820629356909));
#28965=CARTESIAN_POINT('Ctrl Pts',(3.33167571846254,19.2713421302727,2.85336161046155));
#28966=CARTESIAN_POINT('Ctrl Pts',(3.20554674527637,19.4540672990726,3.4372019532105));
#28967=CARTESIAN_POINT('Ctrl Pts',(3.05519487086468,19.6783359010447,3.99999999896489));
#28968=CARTESIAN_POINT('Ctrl Pts',(1.27637679201105,19.8731472551927,3.99999999956669));
#28969=CARTESIAN_POINT('Ctrl Pts',(1.22157081634607,19.6542137025969,3.37073263858838));
#28970=CARTESIAN_POINT('Ctrl Pts',(1.20916011335533,19.4848433224629,2.72191105135517));
#28971=CARTESIAN_POINT('Ctrl Pts',(1.24190597611347,19.2960794163503,1.65242470708135));
#28972=CARTESIAN_POINT('Ctrl Pts',(1.26727187692808,19.2442644111506,1.23816080392278));
#28973=CARTESIAN_POINT('Ctrl Pts',(1.32985096795065,19.1915927623126,0.534319634829282));
#28974=CARTESIAN_POINT('Ctrl Pts',(1.36116119974462,19.180036875869,0.245019097176994));
#28975=CARTESIAN_POINT('Ctrl Pts',(1.4356196770548,19.176734501299,-0.339091664301467));
#28976=CARTESIAN_POINT('Ctrl Pts',(1.47903005465291,19.1854625584862,-0.633868986560752));
#28977=CARTESIAN_POINT('Ctrl Pts',(1.60333245432168,19.2329220526458,-1.37315646709438));
#28978=CARTESIAN_POINT('Ctrl Pts',(1.69186532339448,19.2849434365886,-1.81522038318764));
#28979=CARTESIAN_POINT('Ctrl Pts',(1.93838073553048,19.4602730828479,-2.85098459800567));
#28980=CARTESIAN_POINT('Ctrl Pts',(2.10934078988013,19.6028000727414,-3.43595403740795));
#28981=CARTESIAN_POINT('Ctrl Pts',(2.31470740137874,19.7791114355451,-3.99999999899377));
#28982=CARTESIAN_POINT('Origin',(0.,0.,-1.52655665885959E-15));
#28983=CARTESIAN_POINT('Ctrl Pts',(-2.83169367195905,19.7117383934115,-3.99999999959142));
#28984=CARTESIAN_POINT('Ctrl Pts',(-2.76014648784994,19.498228538721,-3.37209935132288));
#28985=CARTESIAN_POINT('Ctrl Pts',(-2.73483215303947,19.3304887480367,-2.72444369047209));
#28986=CARTESIAN_POINT('Ctrl Pts',(-2.7528026499327,19.1394639546639,-1.65559168315368));
#28987=CARTESIAN_POINT('Ctrl Pts',(-2.77410799980422,19.0856146013948,-1.24058143596684));
#28988=CARTESIAN_POINT('Ctrl Pts',(-2.83250474306813,19.0279820902425,-0.535456738414391));
#28989=CARTESIAN_POINT('Ctrl Pts',(-2.86287361435436,19.0139554414172,-0.245615692594552));
#28990=CARTESIAN_POINT('Ctrl Pts',(-2.93697271462192,19.0047984005021,0.339577232578708));
#28991=CARTESIAN_POINT('Ctrl Pts',(-2.98100083826584,19.0101214553002,0.634895024141513));
#28992=CARTESIAN_POINT('Ctrl Pts',(-3.10880075779996,19.0478441421203,1.37542327969907));
#28993=CARTESIAN_POINT('Ctrl Pts',(-3.201230406372,19.0929364953574,1.81820577067646));
#28994=CARTESIAN_POINT('Ctrl Pts',(-3.46043591760429,19.2486381220978,2.85336120366925));
#28995=CARTESIAN_POINT('Ctrl Pts',(-3.64145416795512,19.3772049873777,3.4372017474516));
#28996=CARTESIAN_POINT('Ctrl Pts',(-3.85944318717446,19.5365252237514,3.99999999896495));
#28997=CARTESIAN_POINT('Ctrl Pts',(-5.59761479218164,19.1111964089144,3.99999999956627));
#28998=CARTESIAN_POINT('Ctrl Pts',(-5.57423581313916,18.8867221808592,3.37073466341711));
#28999=CARTESIAN_POINT('Ctrl Pts',(-5.52796963846162,18.7233217839671,2.72191491022201));
#29000=CARTESIAN_POINT('Ctrl Pts',(-5.43263718388652,18.5571411928451,1.65242958953604));
#29001=CARTESIAN_POINT('Ctrl Pts',(-5.39107901246423,18.5171264390623,1.23816460840836));
#29002=CARTESIAN_POINT('Ctrl Pts',(-5.31425879573908,18.4890343760598,0.534321487023973));
#29003=CARTESIAN_POINT('Ctrl Pts',(-5.28088432901033,18.4888840935175,0.245020063602722));
#29004=CARTESIAN_POINT('Ctrl Pts',(-5.20978656133472,18.5112472302162,-0.339092462175414));
#29005=CARTESIAN_POINT('Ctrl Pts',(-5.17197924185572,18.5342962315364,-0.633870666713147));
#29006=CARTESIAN_POINT('Ctrl Pts',(-5.07140519543395,18.6214078210159,-1.37316000039744));
#29007=CARTESIAN_POINT('Ctrl Pts',(-5.00600388404419,18.7005722398839,-1.81522491330522));
#29008=CARTESIAN_POINT('Ctrl Pts',(-4.83432201949194,18.9496415943053,-2.85098815599153));
#29009=CARTESIAN_POINT('Ctrl Pts',(-4.72241993176988,19.142044415309,-3.43595586451284));
#29010=CARTESIAN_POINT('Ctrl Pts',(-4.58974103596834,19.377961625425,-3.99999999899278));
#29011=CARTESIAN_POINT('Origin',(0.,0.,-1.52655665885959E-15));
#29012=CARTESIAN_POINT('Ctrl Pts',(-9.40271337324756,17.5544894759802,-3.99999999956588));
#29013=CARTESIAN_POINT('Ctrl Pts',(-9.26205290644085,17.3779970458197,-3.37073651667098));
#29014=CARTESIAN_POINT('Ctrl Pts',(-9.18052390874618,17.2290232989812,-2.72191844225021));
#29015=CARTESIAN_POINT('Ctrl Pts',(-9.13204235463609,17.0436751051816,-1.65243405873456));
#29016=CARTESIAN_POINT('Ctrl Pts',(-9.13363704400476,16.9860057520412,-1.23816809120242));
#29017=CARTESIAN_POINT('Ctrl Pts',(-9.16873919747736,16.9121247155117,-0.53432318297038));
#29018=CARTESIAN_POINT('Ctrl Pts',(-9.19243827931884,16.8886249515421,-0.245020948588286));
#29019=CARTESIAN_POINT('Ctrl Pts',(-9.25882349418853,16.8547422874071,0.339093192415483));
#29020=CARTESIAN_POINT('Ctrl Pts',(-9.30194494783863,16.8446825032542,0.633872204674519));
#29021=CARTESIAN_POINT('Ctrl Pts',(-9.43473702863313,16.8363217519894,1.37316323412291));
#29022=CARTESIAN_POINT('Ctrl Pts',(-9.53687179234548,16.8469456166805,1.81522905885359));
#29023=CARTESIAN_POINT('Ctrl Pts',(-9.83389869109708,16.9042615007379,2.85099141175238));
#29024=CARTESIAN_POINT('Ctrl Pts',(-10.0485690253374,16.9630598055312,3.43595753639452));
#29025=CARTESIAN_POINT('Ctrl Pts',(-10.3085579933226,17.038331832428,3.99999999898785));
#29026=CARTESIAN_POINT('Ctrl Pts',(-11.7964514248447,16.0441532441892,3.99999999956582));
#29027=CARTESIAN_POINT('Ctrl Pts',(-11.6977078731037,15.841213326112,3.37073678762359));
#29028=CARTESIAN_POINT('Ctrl Pts',(-11.5983454761381,15.7034916683205,2.72191895896554));
#29029=CARTESIAN_POINT('Ctrl Pts',(-11.451924714039,15.5799384566389,1.65243471246575));
#29030=CARTESIAN_POINT('Ctrl Pts',(-11.3991866319024,15.5565504862445,1.23816860059909));
#29031=CARTESIAN_POINT('Ctrl Pts',(-11.3173907762762,15.5564265561475,0.534323430942822));
#29032=CARTESIAN_POINT('Ctrl Pts',(-11.2859775000167,15.5677000913793,0.245021077953252));
#29033=CARTESIAN_POINT('Ctrl Pts',(-11.2268159107147,15.6130315628994,-0.339093299295225));
#29034=CARTESIAN_POINT('Ctrl Pts',(-11.1991718272373,15.6476215182721,-0.633872429691263));
#29035=CARTESIAN_POINT('Ctrl Pts',(-11.1344570739679,15.7638783461568,-1.37316370731725));
#29036=CARTESIAN_POINT('Ctrl Pts',(-11.1000758830394,15.8606374078146,-1.81522966552197));
#29037=CARTESIAN_POINT('Ctrl Pts',(-11.0239350595913,16.1534046315372,-2.85099188822321));
#29038=CARTESIAN_POINT('Ctrl Pts',(-10.9845876486582,16.3724761407069,-3.43595778093828));
#29039=CARTESIAN_POINT('Ctrl Pts',(-10.9405989703516,16.6395436747412,-3.99999999899175));
#29040=CARTESIAN_POINT('Origin',(0.,0.,-1.52655665885959E-15));
#29041=CARTESIAN_POINT('Ctrl Pts',(-14.8396644849569,13.2798899662611,-3.9999999995905));
#29042=CARTESIAN_POINT('Ctrl Pts',(-14.6476178493579,13.1623228272291,-3.37210843277778));
#29043=CARTESIAN_POINT('Ctrl Pts',(-14.5204071762167,13.0500980157328,-2.72446134739535));
#29044=CARTESIAN_POINT('Ctrl Pts',(-14.4113845387682,12.8922113357405,-1.65561419092038));
#29045=CARTESIAN_POINT('Ctrl Pts',(-14.3930912670057,12.8372640574723,-1.24059921852505));
#29046=CARTESIAN_POINT('Ctrl Pts',(-14.4007800895362,12.7555764141237,-0.535465608026784));
#29047=CARTESIAN_POINT('Ctrl Pts',(-14.4150279702577,12.7253100241341,-0.245620301364524));
#29048=CARTESIAN_POINT('Ctrl Pts',(-14.4659058080358,12.6706645585323,0.339581072840045));
#29049=CARTESIAN_POINT('Ctrl Pts',(-14.503055437724,12.6464413644899,0.634903090053654));
#29050=CARTESIAN_POINT('Ctrl Pts',(-14.6252050701333,12.5931907021228,1.37543967266357));
#29051=CARTESIAN_POINT('Ctrl Pts',(-14.7249961464028,12.5683214715082,1.81822638064967));
#29052=CARTESIAN_POINT('Ctrl Pts',(-15.0236415549683,12.5209843938598,2.85337723697866));
#29053=CARTESIAN_POINT('Ctrl Pts',(-15.2449472948761,12.5031178193119,3.43720985678689));
#29054=CARTESIAN_POINT('Ctrl Pts',(-15.5143414301618,12.4850442338677,3.99999999896252));
#29055=CARTESIAN_POINT('Ctrl Pts',(-16.5724619473705,11.0419484034613,3.99999999956582));
#29056=CARTESIAN_POINT('Ctrl Pts',(-16.4102638255241,10.8850195504957,3.37073680996054));
#29057=CARTESIAN_POINT('Ctrl Pts',(-16.2697901329922,10.7895874722902,2.72191900128754));
#29058=CARTESIAN_POINT('Ctrl Pts',(-16.0899419309864,10.7235642814288,1.65243476610461));
#29059=CARTESIAN_POINT('Ctrl Pts',(-16.0323851836635,10.7196242645906,1.23816864245814));
#29060=CARTESIAN_POINT('Ctrl Pts',(-15.9554798306858,10.7474836393633,0.534323451403115));
#29061=CARTESIAN_POINT('Ctrl Pts',(-15.9298167816178,10.7688212711311,0.245021088648856));
#29062=CARTESIAN_POINT('Ctrl Pts',(-15.8897273477402,10.8316533775811,-0.339093308039497));
#29063=CARTESIAN_POINT('Ctrl Pts',(-15.875580867942,10.8736121380598,-0.633872448158881));
#29064=CARTESIAN_POINT('Ctrl Pts',(-15.8545310703183,11.0049915738749,-1.37316374602659));
#29065=CARTESIAN_POINT('Ctrl Pts',(-15.855316869219,11.1076744121152,-1.81522971507324));
#29066=CARTESIAN_POINT('Ctrl Pts',(-15.8839001931801,11.4088273039884,-2.85099192711218));
#29067=CARTESIAN_POINT('Ctrl Pts',(-15.9218525929265,11.6281447821453,-3.43595780101046));
#29068=CARTESIAN_POINT('Ctrl Pts',(-15.9718592317868,11.8941511766754,-3.9999999989877));
#29069=CARTESIAN_POINT('Origin',(0.,0.,-1.52655665885959E-15));
#29070=CARTESIAN_POINT('Ctrl Pts',(-18.4867130622875,7.40355047897599,-3.9999999995909));
#29071=CARTESIAN_POINT('Ctrl Pts',(-18.2660364568889,7.35875728365076,-3.37210452431144));
#29072=CARTESIAN_POINT('Ctrl Pts',(-18.1081135146886,7.29680957511262,-2.72445374790304));
#29073=CARTESIAN_POINT('Ctrl Pts',(-17.9516658028163,7.18573329947562,-1.65560450349881));
#29074=CARTESIAN_POINT('Ctrl Pts',(-17.9156830597558,7.14035694592513,-1.24059156465032));
#29075=CARTESIAN_POINT('Ctrl Pts',(-17.8949697327359,7.06096666507544,-0.535461790250346));
#29076=CARTESIAN_POINT('Ctrl Pts',(-17.8980066839884,7.02765276946775,-0.245618317617947));
#29077=CARTESIAN_POINT('Ctrl Pts',(-17.927126208346,6.95890199759269,0.339579419829294));
#29078=CARTESIAN_POINT('Ctrl Pts',(-17.953750427197,6.92343386222213,0.634899618176173));
#29079=CARTESIAN_POINT('Ctrl Pts',(-18.0503200716021,6.831617083009,1.37543261696681));
#29080=CARTESIAN_POINT('Ctrl Pts',(-18.1355867099821,6.77411698191067,1.81821751025154));
#29081=CARTESIAN_POINT('Ctrl Pts',(-18.4000312193516,6.62749077357112,2.85337033648387));
#29082=CARTESIAN_POINT('Ctrl Pts',(-18.601881004032,6.53500943299842,3.4372063667673));
#29083=CARTESIAN_POINT('Ctrl Pts',(-18.848848760419,6.42588670458299,3.99999999896357));
#29084=CARTESIAN_POINT('Ctrl Pts',(-19.3495889825578,4.70792159533567,3.99999999956624));
#29085=CARTESIAN_POINT('Ctrl Pts',(-19.1434991430015,4.61593129472241,3.3707347727776));
#29086=CARTESIAN_POINT('Ctrl Pts',(-18.9788571709899,4.5742988058017,2.72191511865313));
#29087=CARTESIAN_POINT('Ctrl Pts',(-18.7872743073193,4.57376884638241,1.65242985326193));
#29088=CARTESIAN_POINT('Ctrl Pts',(-18.7318414111458,4.58975190711804,1.23816481391789));
#29089=CARTESIAN_POINT('Ctrl Pts',(-18.6691028433861,4.64223414506052,0.534321587091021));
#29090=CARTESIAN_POINT('Ctrl Pts',(-18.6522854566278,4.6710621449107,0.245020115824628));
#29091=CARTESIAN_POINT('Ctrl Pts',(-18.6361036142338,4.74381619739426,-0.339092505248901));
#29092=CARTESIAN_POINT('Ctrl Pts',(-18.6371609770871,4.78808280322809,-0.633870757439877));
#29093=CARTESIAN_POINT('Ctrl Pts',(-18.6623148159461,4.91873829075295,-1.37316019119144));
#29094=CARTESIAN_POINT('Ctrl Pts',(-18.6981725716345,5.0149597044225,-1.81522515791414));
#29095=CARTESIAN_POINT('Ctrl Pts',(-18.8280320498957,5.28817521451328,-2.85098834810475));
#29096=CARTESIAN_POINT('Ctrl Pts',(-18.9387067316056,5.48128662831983,-3.43595596316373));
#29097=CARTESIAN_POINT('Ctrl Pts',(-19.0766775587209,5.71414848024506,-3.99999999899274));
#29098=CARTESIAN_POINT('Origin',(0.,0.,-1.52655665885959E-15));
#29099=CARTESIAN_POINT('Ctrl Pts',(-19.9039912380639,0.634233661349713,
-3.99999999959214));
#29100=CARTESIAN_POINT('Ctrl Pts',(-19.6812984735855,0.667619141633553,
-3.3720921589878));
#29101=CARTESIAN_POINT('Ctrl Pts',(-19.5117100620242,0.663422606907901,
-2.72442970846294));
#29102=CARTESIAN_POINT('Ctrl Pts',(-19.3267092023953,0.61255498269846,-1.65557386072678));
#29103=CARTESIAN_POINT('Ctrl Pts',(-19.2773785775159,0.582223142381439,
-1.24056735630538));
#29104=CARTESIAN_POINT('Ctrl Pts',(-19.2307632060359,0.514706825016789,
-0.535449716736964));
#29105=CARTESIAN_POINT('Ctrl Pts',(-19.2222233880153,0.48236406576677,-0.245612043941133));
#29106=CARTESIAN_POINT('Ctrl Pts',(-19.2260726306597,0.407801406963018,
0.339574192515873));
#29107=CARTESIAN_POINT('Ctrl Pts',(-19.2389599748721,0.365366877205189,
0.634888638814313));
#29108=CARTESIAN_POINT('Ctrl Pts',(-19.2983007127978,0.246059610093303,
1.3754102996325));
#29109=CARTESIAN_POINT('Ctrl Pts',(-19.3587572800335,0.162864518453664,
1.81818944953874));
#29110=CARTESIAN_POINT('Ctrl Pts',(-19.5571030357074,-0.0653676914030244,
2.85334850600551));
#29111=CARTESIAN_POINT('Ctrl Pts',(-19.7151513706586,-0.221313315253387,
3.43719532453647));
#29112=CARTESIAN_POINT('Ctrl Pts',(-19.9099067854224,-0.408327477794065,
3.99999999896687));
#29113=CARTESIAN_POINT('Ctrl Pts',(-19.7928699973623,-2.19395004712364,
3.99999999956673));
#29114=CARTESIAN_POINT('Ctrl Pts',(-19.5677455202026,-2.20990600018682,
3.37073247625875));
#29115=CARTESIAN_POINT('Ctrl Pts',(-19.3987931331181,-2.19271733132894,
2.7219107420094));
#29116=CARTESIAN_POINT('Ctrl Pts',(-19.2185832617589,-2.12769046720652,
1.6524243156881));
#29117=CARTESIAN_POINT('Ctrl Pts',(-19.1719602065399,-2.09371236649188,
1.23816049895436));
#29118=CARTESIAN_POINT('Ctrl Pts',(-19.1309555250841,-2.02293768065745,
0.534319486362197));
#29119=CARTESIAN_POINT('Ctrl Pts',(-19.1250121674529,-1.99009647260577,
0.245019019702941));
#29120=CARTESIAN_POINT('Ctrl Pts',(-19.1346895408446,-1.9161957526751,-0.339091600369012));
#29121=CARTESIAN_POINT('Ctrl Pts',(-19.1508231264452,-1.87496049495226,
-0.633868851915709));
#29122=CARTESIAN_POINT('Ctrl Pts',(-19.2191464649171,-1.76078779531645,
-1.37315618389887));
#29123=CARTESIAN_POINT('Ctrl Pts',(-19.2857510759732,-1.6826333610479,-1.8152200200743));
#29124=CARTESIAN_POINT('Ctrl Pts',(-19.5012240036822,-1.47030870183375,
-2.85098431280495));
#29125=CARTESIAN_POINT('Ctrl Pts',(-19.6712726215212,-1.32669540341637,
-3.43595389094347));
#29126=CARTESIAN_POINT('Ctrl Pts',(-19.8805670113664,-1.15506486410126,
-3.99999999899386));
#29127=CARTESIAN_POINT('Origin',(0.,0.,-1.52655665885959E-15));
#29128=CARTESIAN_POINT('Ctrl Pts',(-18.9205613831265,-6.2115599078728,-3.9999999995661));
#29129=CARTESIAN_POINT('Ctrl Pts',(-18.7223245302125,-6.10368372786451,
-3.37073547209815));
#29130=CARTESIAN_POINT('Ctrl Pts',(-18.5614565921404,-6.04926209466741,
-2.72191645127299));
#29131=CARTESIAN_POINT('Ctrl Pts',(-18.3705057445077,-6.03370239487686,
-1.65243153951694));
#29132=CARTESIAN_POINT('Ctrl Pts',(-18.3139896008193,-6.04528699644354,
-1.23816612802062));
#29133=CARTESIAN_POINT('Ctrl Pts',(-18.2473265986844,-6.09268509357922,
-0.534322227065162));
#29134=CARTESIAN_POINT('Ctrl Pts',(-18.2282992017476,-6.12010477942166,
-0.245020449844545));
#29135=CARTESIAN_POINT('Ctrl Pts',(-18.2064590003801,-6.19136501241902,
0.339092780595737));
#29136=CARTESIAN_POINT('Ctrl Pts',(-18.2040399950647,-6.23557815835044,
0.63387133750551));
#29137=CARTESIAN_POINT('Ctrl Pts',(-18.2188652552551,-6.3678045190608,1.37316141091046));
#29138=CARTESIAN_POINT('Ctrl Pts',(-18.2470631112762,-6.46654273339332,
1.81522672156502));
#29139=CARTESIAN_POINT('Ctrl Pts',(-18.3550861881394,-6.74910453147274,
2.85098957614178));
#29140=CARTESIAN_POINT('Ctrl Pts',(-18.4502683407411,-6.95030377780392,
3.43595659386126));
#29141=CARTESIAN_POINT('Ctrl Pts',(-18.5695436021889,-7.19327254732061,
3.99999999898836));
#29142=CARTESIAN_POINT('Ctrl Pts',(-17.8488387937264,-8.83119885730778,
3.99999999956597));
#29143=CARTESIAN_POINT('Ctrl Pts',(-17.6318350798565,-8.76919556449981,
3.37073606759622));
#29144=CARTESIAN_POINT('Ctrl Pts',(-17.4789514598517,-8.69525791380816,
2.72191758653968));
#29145=CARTESIAN_POINT('Ctrl Pts',(-17.3318496791241,-8.5725165426358,1.65243297589238));
#29146=CARTESIAN_POINT('Ctrl Pts',(-17.299659216218,-8.52464104898616,1.23816724729049));
#29147=CARTESIAN_POINT('Ctrl Pts',(-17.2853335211172,-8.44410950931466,
0.534322771948021));
#29148=CARTESIAN_POINT('Ctrl Pts',(-17.2909809309559,-8.41121588889571,
0.245020734090218));
#29149=CARTESIAN_POINT('Ctrl Pts',(-17.3253503814445,-8.34508143892643,
-0.339093015497721));
#29150=CARTESIAN_POINT('Ctrl Pts',(-17.3546144576353,-8.31185087091257,
-0.633871832021433));
#29151=CARTESIAN_POINT('Ctrl Pts',(-17.4578673627859,-8.22793150915451,
-1.37316245071452));
#29152=CARTESIAN_POINT('Ctrl Pts',(-17.547186107118,-8.17727058956495,-1.81522805463407));
#29153=CARTESIAN_POINT('Ctrl Pts',(-17.8222838092909,-8.05144781004217,
-2.85099062310861));
#29154=CARTESIAN_POINT('Ctrl Pts',(-18.0311947505324,-7.97465658921225,
-3.43595713134647));
#29155=CARTESIAN_POINT('Ctrl Pts',(-18.2865666872494,-7.88496026156533,
-3.9999999989921));
#29156=CARTESIAN_POINT('Origin',(0.,0.,-1.52655665885959E-15));
#29157=CARTESIAN_POINT('Ctrl Pts',(-15.6550192929788,-12.3081879445576,
-3.9999999995905));
#29158=CARTESIAN_POINT('Ctrl Pts',(-15.5058897133018,-12.1394742461215,
-3.37210842588511));
#29159=CARTESIAN_POINT('Ctrl Pts',(-15.3732799472849,-12.0336838211982,
-2.72446133398417));
#29160=CARTESIAN_POINT('Ctrl Pts',(-15.1988603399449,-11.9537342169486,
-1.65561417381906));
#29161=CARTESIAN_POINT('Ctrl Pts',(-15.1415712421405,-11.9452603559542,
-1.24059920500475));
#29162=CARTESIAN_POINT('Ctrl Pts',(-15.0624597690894,-11.9670172783195,
-0.535465601238678));
#29163=CARTESIAN_POINT('Ctrl Pts',(-15.0351273125377,-11.9863044050087,
-0.245620297782277));
#29164=CARTESIAN_POINT('Ctrl Pts',(-14.9901468786537,-12.0458983790397,
0.33958107008003));
#29165=CARTESIAN_POINT('Ctrl Pts',(-14.9727426549024,-12.0866899354678,
0.634903084128853));
#29166=CARTESIAN_POINT('Ctrl Pts',(-14.9415120504093,-12.2162307198888,
1.37543966053627));
#29167=CARTESIAN_POINT('Ctrl Pts',(-14.934349177211,-12.3188242413817,1.81822636539706));
#29168=CARTESIAN_POINT('Ctrl Pts',(-14.9395904852347,-12.6211525532137,
2.85337722511011));
#29169=CARTESIAN_POINT('Ctrl Pts',(-14.960424681677,-12.8421986625469,3.43720985078044));
#29170=CARTESIAN_POINT('Ctrl Pts',(-14.9894054753209,-13.110638543934,3.99999999896253));
#29171=CARTESIAN_POINT('Ctrl Pts',(-13.751974213328,-14.403274793522,3.9999999995658));
#29172=CARTESIAN_POINT('Ctrl Pts',(-13.5692640748007,-14.2707912447243,
3.37073687076865));
#29173=CARTESIAN_POINT('Ctrl Pts',(-13.4508888393199,-14.1490232670549,
2.72191911720231));
#29174=CARTESIAN_POINT('Ctrl Pts',(-13.3546383743594,-13.9833721567228,
1.6524349127806));
#29175=CARTESIAN_POINT('Ctrl Pts',(-13.3407635887915,-13.9273739926909,
1.23816875677089));
#29176=CARTESIAN_POINT('Ctrl Pts',(-13.3548452422531,-13.8467992630841,
0.534323507098637));
#29177=CARTESIAN_POINT('Ctrl Pts',(-13.3714023668365,-13.81782084875,0.245021117745642));
#29178=CARTESIAN_POINT('Ctrl Pts',(-13.4263184597996,-13.7674297780966,
-0.339093331911454));
#29179=CARTESIAN_POINT('Ctrl Pts',(-13.4651832654341,-13.746212152059,-0.633872498514063));
#29180=CARTESIAN_POINT('Ctrl Pts',(-13.5909115034643,-13.7026683508362,
-1.37316385195566));
#29181=CARTESIAN_POINT('Ctrl Pts',(-13.6921708184002,-13.6856115284966,
-1.81522985087203));
#29182=CARTESIAN_POINT('Ctrl Pts',(-13.9937119583052,-13.6614659738392,
-2.85099203376423));
#29183=CARTESIAN_POINT('Ctrl Pts',(-14.2162878519877,-13.6607577216152,
-3.43595785577492));
#29184=CARTESIAN_POINT('Ctrl Pts',(-14.4869365444277,-13.6638131241373,
-3.99999999898768));
#29185=CARTESIAN_POINT('Origin',(0.,0.,-1.52655665885959E-15));
#29186=CARTESIAN_POINT('Ctrl Pts',(-10.5012771497262,-16.9202333839219,
-3.99999999956588));
#29187=CARTESIAN_POINT('Ctrl Pts',(-10.4187604568685,-16.7101716410219,
-3.37073654287492));
#29188=CARTESIAN_POINT('Ctrl Pts',(-10.3305099036574,-16.5650785907353,
-2.72191849220108));
#29189=CARTESIAN_POINT('Ctrl Pts',(-10.1942344309796,-16.4304182340015,
-1.65243412194127));
#29190=CARTESIAN_POINT('Ctrl Pts',(-10.1434939576109,-16.4029645969824,
-1.23816814046302));
#29191=CARTESIAN_POINT('Ctrl Pts',(-10.0619600213849,-16.3964234338767,
-0.534323206973444));
#29192=CARTESIAN_POINT('Ctrl Pts',(-10.0297590861916,-16.405197558861,-0.245020961131435));
#29193=CARTESIAN_POINT('Ctrl Pts',(-9.96722322847196,-16.445747510702,0.339093202692876));
#29194=CARTESIAN_POINT('Ctrl Pts',(-9.93695047232516,-16.4780618942896,
0.633872226361229));
#29195=CARTESIAN_POINT('Ctrl Pts',(-9.86331380880832,-16.5888828384849,
1.37316327975098));
#29196=CARTESIAN_POINT('Ctrl Pts',(-9.82144696478302,-16.6826460743033,
1.81522911734934));
#29197=CARTESIAN_POINT('Ctrl Pts',(-9.72257053474009,-16.9685368560364,
2.85099145769367));
#29198=CARTESIAN_POINT('Ctrl Pts',(-9.66615620033608,-17.1838459623691,
3.43595755998537));
#29199=CARTESIAN_POINT('Ctrl Pts',(-9.6013492080081,-17.4466390149939,3.99999999898783));
#29200=CARTESIAN_POINT('Ctrl Pts',(-7.99641857074021,-18.238103234253,3.99999999956596));
#29201=CARTESIAN_POINT('Ctrl Pts',(-7.87003904712881,-18.0511186750576,
3.37073613189377));
#29202=CARTESIAN_POINT('Ctrl Pts',(-7.80044962194119,-17.8962074550045,
2.72191770909427));
#29203=CARTESIAN_POINT('Ctrl Pts',(-7.7666597555164,-17.7076268935435,1.6524331309639));
#29204=CARTESIAN_POINT('Ctrl Pts',(-7.77277420580999,-17.6502604964735,
1.23816736813676));
#29205=CARTESIAN_POINT('Ctrl Pts',(-7.81356476654144,-17.5793613665421,
0.534322830796256));
#29206=CARTESIAN_POINT('Ctrl Pts',(-7.83903454756133,-17.557793473122,0.245020764801146));
#29207=CARTESIAN_POINT('Ctrl Pts',(-7.90787348529572,-17.5292237992452,
-0.339093040828276));
#29208=CARTESIAN_POINT('Ctrl Pts',(-7.95165126932984,-17.5225782933531,
-0.633871885375969));
#29209=CARTESIAN_POINT('Ctrl Pts',(-8.08468991868255,-17.524662026619,-1.37316256290256));
#29210=CARTESIAN_POINT('Ctrl Pts',(-8.18567626336398,-17.5432664999818,
-1.81522819845542));
#29211=CARTESIAN_POINT('Ctrl Pts',(-8.47729064196968,-17.6237100686022,
-2.85099073606036));
#29212=CARTESIAN_POINT('Ctrl Pts',(-8.68668612492522,-17.699169947002,-3.43595718934435));
#29213=CARTESIAN_POINT('Ctrl Pts',(-8.93996803629468,-17.7946084824509,
-3.99999999899206));
#29214=CARTESIAN_POINT('Origin',(0.,0.,-1.52655665885959E-15));
#29215=CARTESIAN_POINT('Ctrl Pts',(-4.08088993973066,-19.4914713872994,
-3.99999999959139));
#29216=CARTESIAN_POINT('Ctrl Pts',(-4.075097616853,-19.2663672599189,-3.37209958168756));
#29217=CARTESIAN_POINT('Ctrl Pts',(-4.04151488495295,-19.100085449018,-2.72444413832849));
#29218=CARTESIAN_POINT('Ctrl Pts',(-3.95929377669572,-18.9267270967929,
-1.65559225403134));
#29219=CARTESIAN_POINT('Ctrl Pts',(-3.92085570623925,-18.8834120879058,
-1.24058188697122));
#29220=CARTESIAN_POINT('Ctrl Pts',(-3.84626919930535,-18.8492280764763,
-0.535456963326743));
#29221=CARTESIAN_POINT('Ctrl Pts',(-3.81293438333759,-18.8464340988296,
-0.245615809434569));
#29222=CARTESIAN_POINT('Ctrl Pts',(-3.74017208754007,-18.8631726846702,
0.33957733005154));
#29223=CARTESIAN_POINT('Ctrl Pts',(-3.70061976632791,-18.8832332349247,
0.634895228803465));
#29224=CARTESIAN_POINT('Ctrl Pts',(-3.59342903055762,-18.96239114962,1.37542369564931));
#29225=CARTESIAN_POINT('Ctrl Pts',(-3.52199606602467,-19.0363769342966,
1.81820629365906));
#29226=CARTESIAN_POINT('Ctrl Pts',(-3.33167571844776,-19.2713421302941,
2.85336161053001));
#29227=CARTESIAN_POINT('Ctrl Pts',(-3.20554674526758,-19.4540672990858,
3.43720195324353));
#29228=CARTESIAN_POINT('Ctrl Pts',(-3.05519487086468,-19.6783359010447,
3.99999999896488));
#29229=CARTESIAN_POINT('Ctrl Pts',(-1.27637679201104,-19.8731472551927,
3.99999999956669));
#29230=CARTESIAN_POINT('Ctrl Pts',(-1.22157081634586,-19.6542137025961,
3.37073263858597));
#29231=CARTESIAN_POINT('Ctrl Pts',(-1.20916011335527,-19.4848433224616,
2.72191105135018));
#29232=CARTESIAN_POINT('Ctrl Pts',(-1.2419059761139,-19.2960794163494,1.65242470707477));
#29233=CARTESIAN_POINT('Ctrl Pts',(-1.26727187692857,-19.2442644111501,
1.23816080391726));
#29234=CARTESIAN_POINT('Ctrl Pts',(-1.32985096795119,-19.1915927623124,
0.534319634824896));
#29235=CARTESIAN_POINT('Ctrl Pts',(-1.36116119974521,-19.1800368758689,
0.245019097172672));
#29236=CARTESIAN_POINT('Ctrl Pts',(-1.43561967705555,-19.1767345012991,
-0.3390916643061));
#29237=CARTESIAN_POINT('Ctrl Pts',(-1.47903005465377,-19.1854625584864,
-0.633868986565802));
#29238=CARTESIAN_POINT('Ctrl Pts',(-1.6033324543231,-19.2329220526464,-1.37315646710162));
#29239=CARTESIAN_POINT('Ctrl Pts',(-1.69186532339641,-19.2849434365897,
-1.81522038319652));
#29240=CARTESIAN_POINT('Ctrl Pts',(-1.93838073553248,-19.4602730828495,
-2.85098459801236));
#29241=CARTESIAN_POINT('Ctrl Pts',(-2.10934078988132,-19.6028000727424,
-3.43595403741119));
#29242=CARTESIAN_POINT('Ctrl Pts',(-2.31470740137875,-19.7791114355451,
-3.99999999899378));
#29243=CARTESIAN_POINT('Origin',(0.,0.,-1.52655665885959E-15));
#29244=CARTESIAN_POINT('Ctrl Pts',(2.83169367195904,-19.7117383934115,-3.99999999959142));
#29245=CARTESIAN_POINT('Ctrl Pts',(2.7601464878485,-19.4982285387167,-3.37209935131022));
#29246=CARTESIAN_POINT('Ctrl Pts',(2.7348321530384,-19.3304887480299,-2.724443690446));
#29247=CARTESIAN_POINT('Ctrl Pts',(2.75280264993414,-19.1394639546591,-1.65559168311938));
#29248=CARTESIAN_POINT('Ctrl Pts',(2.77410799980605,-19.0856146013918,-1.24058143593821));
#29249=CARTESIAN_POINT('Ctrl Pts',(2.83250474307015,-19.0279820902413,-0.535456738393028));
#29250=CARTESIAN_POINT('Ctrl Pts',(2.86287361435655,-19.0139554414165,-0.245615692574478));
#29251=CARTESIAN_POINT('Ctrl Pts',(2.93697271462468,-19.0047984005023,0.339577232598883));
#29252=CARTESIAN_POINT('Ctrl Pts',(2.98100083826909,-19.0101214553008,0.634895024162846));
#29253=CARTESIAN_POINT('Ctrl Pts',(3.10880075780547,-19.0478441421225,1.3754232797282));
#29254=CARTESIAN_POINT('Ctrl Pts',(3.20123040637967,-19.0929364953614,1.818205770712));
#29255=CARTESIAN_POINT('Ctrl Pts',(3.46043591761268,-19.2486381221038,2.85336120369635));
#29256=CARTESIAN_POINT('Ctrl Pts',(3.64145416796019,-19.3772049873814,3.43720174746467));
#29257=CARTESIAN_POINT('Ctrl Pts',(3.85944318717447,-19.5365252237514,3.99999999896495));
#29258=CARTESIAN_POINT('Ctrl Pts',(5.59761479218166,-19.1111964089144,3.99999999956627));
#29259=CARTESIAN_POINT('Ctrl Pts',(5.57423581314006,-18.8867221808677,3.37073466344091));
#29260=CARTESIAN_POINT('Ctrl Pts',(5.52796963846509,-18.7233217839794,2.72191491027107));
#29261=CARTESIAN_POINT('Ctrl Pts',(5.43263718389282,-18.5571411928521,1.65242958960015));
#29262=CARTESIAN_POINT('Ctrl Pts',(5.39107901246981,-18.5171264390661,1.2381646084617));
#29263=CARTESIAN_POINT('Ctrl Pts',(5.31425879574368,-18.4890343760603,0.534321487064496));
#29264=CARTESIAN_POINT('Ctrl Pts',(5.28088432901487,-18.488884093517,0.245020063641224));
#29265=CARTESIAN_POINT('Ctrl Pts',(5.20978656133964,-18.5112472302137,-0.339092462136402));
#29266=CARTESIAN_POINT('Ctrl Pts',(5.17197924186115,-18.5342962315327,-0.633870666671581));
#29267=CARTESIAN_POINT('Ctrl Pts',(5.07140519544207,-18.6214078210074,-1.37316000034045));
#29268=CARTESIAN_POINT('Ctrl Pts',(5.00600388405473,-18.7005722398706,-1.81522491323566));
#29269=CARTESIAN_POINT('Ctrl Pts',(4.83432201950212,-18.9496415942878,-2.8509881559385));
#29270=CARTESIAN_POINT('Ctrl Pts',(4.72241993177592,-19.1420444152983,-3.43595586448725));
#29271=CARTESIAN_POINT('Ctrl Pts',(4.58974103596836,-19.377961625425,-3.99999999899278));
#29272=CARTESIAN_POINT('Origin',(0.,0.,-1.52655665885959E-15));
#29273=CARTESIAN_POINT('Ctrl Pts',(9.40271337324749,-17.5544894759802,-3.99999999956588));
#29274=CARTESIAN_POINT('Ctrl Pts',(9.26205290644762,-17.3779970458287,-3.3707365167023));
#29275=CARTESIAN_POINT('Ctrl Pts',(9.18052390875412,-17.2290232989961,-2.72191844231462));
#29276=CARTESIAN_POINT('Ctrl Pts',(9.13204235463654,-17.0436751051941,-1.65243405881907));
#29277=CARTESIAN_POINT('Ctrl Pts',(9.13363704400285,-16.98600575205,-1.23816809127292));
#29278=CARTESIAN_POINT('Ctrl Pts',(9.16873919747339,-16.9121247155165,-0.534323183023807));
#29279=CARTESIAN_POINT('Ctrl Pts',(9.19243827931401,-16.8886249515458,-0.245020948638851));
#29280=CARTESIAN_POINT('Ctrl Pts',(9.25882349418162,-16.8547422874094,0.339093192364722));
#29281=CARTESIAN_POINT('Ctrl Pts',(9.30194494783013,-16.8446825032557,0.633872204620666));
#29282=CARTESIAN_POINT('Ctrl Pts',(9.43473702861777,-16.836321751989,1.37316323404884));
#29283=CARTESIAN_POINT('Ctrl Pts',(9.53687179232336,-16.8469456166778,1.8152290587629));
#29284=CARTESIAN_POINT('Ctrl Pts',(9.83389869107151,-16.9042615007311,2.8509914116832));
#29285=CARTESIAN_POINT('Ctrl Pts',(10.0485690253218,-16.9630598055269,3.43595753636118));
#29286=CARTESIAN_POINT('Ctrl Pts',(10.3085579933225,-17.0383318324281,3.99999999898785));
#29287=CARTESIAN_POINT('Ctrl Pts',(11.7964514248447,-16.0441532441892,3.99999999956582));
#29288=CARTESIAN_POINT('Ctrl Pts',(11.6977078731048,-15.8412133261142,3.37073678763047));
#29289=CARTESIAN_POINT('Ctrl Pts',(11.5983454761403,-15.7034916683235,2.72191895897971));
#29290=CARTESIAN_POINT('Ctrl Pts',(11.4519247140414,-15.5799384566402,1.65243471248429));
#29291=CARTESIAN_POINT('Ctrl Pts',(11.3991866319042,-15.556550486245,1.23816860061448));
#29292=CARTESIAN_POINT('Ctrl Pts',(11.3173907762775,-15.5564265561472,0.534323430954352));
#29293=CARTESIAN_POINT('Ctrl Pts',(11.2859775000178,-15.5677000913787,0.245021077964069));
#29294=CARTESIAN_POINT('Ctrl Pts',(11.2268159107157,-15.6130315628983,-0.3390932992844));
#29295=CARTESIAN_POINT('Ctrl Pts',(11.1991718272383,-15.6476215182706,-0.633872429679788));
#29296=CARTESIAN_POINT('Ctrl Pts',(11.1344570739692,-15.7638783461539,-1.37316370730182));
#29297=CARTESIAN_POINT('Ctrl Pts',(11.1000758830408,-15.8606374078102,-1.81522966550313));
#29298=CARTESIAN_POINT('Ctrl Pts',(11.0239350595923,-16.1534046315318,-2.85099188820882));
#29299=CARTESIAN_POINT('Ctrl Pts',(10.9845876486587,-16.3724761407036,-3.43595778093133));
#29300=CARTESIAN_POINT('Ctrl Pts',(10.9405989703516,-16.6395436747412,-3.99999999899174));
#29301=CARTESIAN_POINT('Origin',(0.,0.,-1.52655665885959E-15));
#29302=CARTESIAN_POINT('Ctrl Pts',(14.8396644849569,-13.2798899662611,-3.9999999995905));
#29303=CARTESIAN_POINT('Ctrl Pts',(14.6476178493517,-13.1623228272254,-3.37210843275759));
#29304=CARTESIAN_POINT('Ctrl Pts',(14.5204071762085,-13.0500980157257,-2.72446134735375));
#29305=CARTESIAN_POINT('Ctrl Pts',(14.4113845387651,-12.8922113357332,-1.65561419086607));
#29306=CARTESIAN_POINT('Ctrl Pts',(14.3930912670047,-12.8372640574668,-1.24059921848));
#29307=CARTESIAN_POINT('Ctrl Pts',(14.4007800895373,-12.7555764141202,-0.535465607992792));
#29308=CARTESIAN_POINT('Ctrl Pts',(14.4150279702596,-12.725310024131,-0.245620301332475));
#29309=CARTESIAN_POINT('Ctrl Pts',(14.4659058080392,-12.6706645585297,0.339581072872028));
#29310=CARTESIAN_POINT('Ctrl Pts',(14.5030554377286,-12.6464413644873,0.634903090087537));
#29311=CARTESIAN_POINT('Ctrl Pts',(14.6252050701422,-12.5931907021199,1.37543967270944));
#29312=CARTESIAN_POINT('Ctrl Pts',(14.7249961464161,-12.5683214715053,1.81822638070561));
#29313=CARTESIAN_POINT('Ctrl Pts',(15.0236415549845,-12.5209843938585,2.85337723702139));
#29314=CARTESIAN_POINT('Ctrl Pts',(15.244947294886,-12.5031178193113,3.43720985680749));
#29315=CARTESIAN_POINT('Ctrl Pts',(15.5143414301618,-12.4850442338677,3.99999999896253));
#29316=CARTESIAN_POINT('Ctrl Pts',(16.5724493912429,-11.0419672484927,3.99999999959052));
#29317=CARTESIAN_POINT('Ctrl Pts',(16.4105423432717,-10.8854741265665,3.37210815126127));
#29318=CARTESIAN_POINT('Ctrl Pts',(16.2700411426964,-10.7904141902987,2.72446080000339));
#29319=CARTESIAN_POINT('Ctrl Pts',(16.0898865008145,-10.7243958472827,1.65561349312514));
#29320=CARTESIAN_POINT('Ctrl Pts',(16.0321092007946,-10.720442960367,1.24059866719413));
#29321=CARTESIAN_POINT('Ctrl Pts',(15.9549486870048,-10.7483398201034,0.535465332991227));
#29322=CARTESIAN_POINT('Ctrl Pts',(15.9292137549567,-10.7697119622927,0.245620158427659));
#29323=CARTESIAN_POINT('Ctrl Pts',(15.8890476878997,-10.8326513267222,-0.339580953843327));
#29324=CARTESIAN_POINT('Ctrl Pts',(15.874897584762,-10.8746826391374,-0.634902840058553));
#29325=CARTESIAN_POINT('Ctrl Pts',(15.8539268865206,-11.0062743746583,-1.37543916459227));
#29326=CARTESIAN_POINT('Ctrl Pts',(15.8548354618282,-11.1091136012863,-1.81822574191787));
#29327=CARTESIAN_POINT('Ctrl Pts',(15.8837809457042,-11.4100987454289,-2.85337674009904));
#29328=CARTESIAN_POINT('Ctrl Pts',(15.9218939692831,-11.6288289263462,-3.43720960548705));
#29329=CARTESIAN_POINT('Ctrl Pts',(15.971846987374,-11.894167618845,-3.9999999989626));
#29330=CARTESIAN_POINT('Origin',(0.,0.,-1.52655665885959E-15));
#29331=CARTESIAN_POINT('Ctrl Pts',(18.4867046541144,-7.40357147418018,-3.99999999956608));
#29332=CARTESIAN_POINT('Ctrl Pts',(18.2655049621798,-7.35878522980345,-3.37073552377234));
#29333=CARTESIAN_POINT('Ctrl Pts',(18.1072914318695,-7.29707069450407,-2.72191654976098));
#29334=CARTESIAN_POINT('Ctrl Pts',(17.9510130074857,-7.186249267535,-1.65243166413342));
#29335=CARTESIAN_POINT('Ctrl Pts',(17.9151655629091,-7.14104706416568,-1.238166225129));
#29336=CARTESIAN_POINT('Ctrl Pts',(17.8945656455494,-7.0618878542373,-0.534322274341816));
#29337=CARTESIAN_POINT('Ctrl Pts',(17.897614847696,-7.0286525779651,-0.245020474504692));
#29338=CARTESIAN_POINT('Ctrl Pts',(17.9266894795329,-6.96002545649323,0.339092800984476));
#29339=CARTESIAN_POINT('Ctrl Pts',(17.9532560787444,-6.92460131329069,0.633871380422906));
#29340=CARTESIAN_POINT('Ctrl Pts',(18.0496063618674,-6.83283953621556,1.37316150113643));
#29341=CARTESIAN_POINT('Ctrl Pts',(18.1346748807368,-6.77532690925219,1.81522683723282));
#29342=CARTESIAN_POINT('Ctrl Pts',(18.3990525834921,-6.62830792441045,2.85098966698316));
#29343=CARTESIAN_POINT('Ctrl Pts',(18.6012947101893,-6.53536228497352,3.43595664050605));
#29344=CARTESIAN_POINT('Ctrl Pts',(18.8488421544629,-6.42590608161792,3.99999999898834));
#29345=CARTESIAN_POINT('Ctrl Pts',(19.3495836398166,-4.70794355402034,3.99999999959111));
#29346=CARTESIAN_POINT('Ctrl Pts',(19.1439151849879,-4.61626238501579,3.37210239330695));
#29347=CARTESIAN_POINT('Ctrl Pts',(18.9793742258157,-4.57498815790177,2.72444960464601));
#29348=CARTESIAN_POINT('Ctrl Pts',(18.7875058402052,-4.5745672552028,1.65559922198222));
#29349=CARTESIAN_POINT('Ctrl Pts',(18.7318618872307,-4.59061344990958,1.24058739192793));
#29350=CARTESIAN_POINT('Ctrl Pts',(18.6688970666432,-4.64321781147727,0.535459708945694));
#29351=CARTESIAN_POINT('Ctrl Pts',(18.65202412042,-4.67210262964909,0.245617236089079));
#29352=CARTESIAN_POINT('Ctrl Pts',(18.6358070632848,-4.74498326107249,-0.339578518865884));
#29353=CARTESIAN_POINT('Ctrl Pts',(18.6368857612635,-4.78931905828187,-0.634897725707169));
#29354=CARTESIAN_POINT('Ctrl Pts',(18.6621860721811,-4.92014654177133,-1.37542877063301));
#29355=CARTESIAN_POINT('Ctrl Pts',(18.6982122204778,-5.01647273909291,-1.81821267443061));
#29356=CARTESIAN_POINT('Ctrl Pts',(18.8283538957884,-5.28940758861785,-2.85336657449289));
#29357=CARTESIAN_POINT('Ctrl Pts',(18.9389788671592,-5.48191375800988,-3.43720446401169));
#29358=CARTESIAN_POINT('Ctrl Pts',(19.0766716892569,-5.71416807537147,-3.99999999896414));
#29359=CARTESIAN_POINT('Ctrl Pts',(16.7190336201597,-4.91959556137297,-10.5713320220547));
#29360=CARTESIAN_POINT('Ctrl Pts',(16.9459555615988,-4.14841111729778,-3.52377734068488));
#29361=CARTESIAN_POINT('Ctrl Pts',(17.1194334972985,-3.36150582706258,3.52377734068489));
#29362=CARTESIAN_POINT('Ctrl Pts',(17.2378112556832,-2.56639217442552,10.5713320220547));
#29363=CARTESIAN_POINT('Ctrl Pts',(16.7186664266411,-4.91948445047195,-10.5713320220547));
#29364=CARTESIAN_POINT('Ctrl Pts',(16.9455832429635,-4.14831694361546,-3.52377734068489));
#29365=CARTESIAN_POINT('Ctrl Pts',(17.1190572273169,-3.36142894566319,3.5237773406849));
#29366=CARTESIAN_POINT('Ctrl Pts',(17.2374322458488,-2.56633277528584,10.5713320220547));
#29367=CARTESIAN_POINT('Ctrl Pts',(16.718299233125,-4.91937333957171,-10.5713320220547));
#29368=CARTESIAN_POINT('Ctrl Pts',(16.9452109243307,-4.14822276993388,-3.52377734068487));
#29369=CARTESIAN_POINT('Ctrl Pts',(17.1186809573378,-3.36135206426426,3.52377734068488));
#29370=CARTESIAN_POINT('Ctrl Pts',(17.2370532360168,-2.56627337614658,10.5713320220547));
#29371=CARTESIAN_POINT('Ctrl Pts',(16.7179320396407,-4.91926222868205,-10.5713320220547));
#29372=CARTESIAN_POINT('Ctrl Pts',(16.9448386057302,-4.14812859626138,-3.52377734068488));
#29373=CARTESIAN_POINT('Ctrl Pts',(17.1183046873915,-3.36127518287299,3.52377734068489));
#29374=CARTESIAN_POINT('Ctrl Pts',(17.2366742262179,-2.56621397701342,10.5713320220547));
#29375=CARTESIAN_POINT('Ctrl Pts',(16.7190706763197,-4.91946962582517,-10.5701811473657));
#29376=CARTESIAN_POINT('Ctrl Pts',(16.9459620956421,-4.14836742740649,-3.52339371578857));
#29377=CARTESIAN_POINT('Ctrl Pts',(17.1194210550923,-3.3615482144642,3.52339371578857));
#29378=CARTESIAN_POINT('Ctrl Pts',(17.2377919239458,-2.56652201742717,10.5701811473657));
#29379=CARTESIAN_POINT('Ctrl Pts',(16.7179320396407,-4.91926222868205,-10.5713320220547));
#29380=CARTESIAN_POINT('Ctrl Pts',(16.9448386057302,-4.14812859626139,-3.52377734068488));
#29381=CARTESIAN_POINT('Ctrl Pts',(17.1183046873915,-3.36127518287299,3.52377734068489));
#29382=CARTESIAN_POINT('Ctrl Pts',(17.2366742262179,-2.56621397701342,10.5713320220547));
#29383=CARTESIAN_POINT('Ctrl Pts',(14.0281517405305,-10.341153921307,-10.5713320220547));
#29384=CARTESIAN_POINT('Ctrl Pts',(14.5051492284884,-9.69408946487939,-3.52377734068488));
#29385=CARTESIAN_POINT('Ctrl Pts',(14.9373026246845,-9.01397331881983,3.52377734068489));
#29386=CARTESIAN_POINT('Ctrl Pts',(15.3204862161389,-8.30729846463996,10.5713320220547));
#29387=CARTESIAN_POINT('Ctrl Pts',(14.027844693657,-10.3409239236334,-10.5713320220547));
#29388=CARTESIAN_POINT('Ctrl Pts',(14.5048315727105,-9.69387363009204,-3.52377734068488));
#29389=CARTESIAN_POINT('Ctrl Pts',(14.9369753415466,-9.01377238202311,3.52377734068489));
#29390=CARTESIAN_POINT('Ctrl Pts',(15.3201503790965,-8.30711301870881,10.5713320220547));
#29391=CARTESIAN_POINT('Ctrl Pts',(14.0275376467855,-10.3406939259613,-10.5713320220547));
#29392=CARTESIAN_POINT('Ctrl Pts',(14.5045139169348,-9.69365779530623,-3.52377734068489));
#29393=CARTESIAN_POINT('Ctrl Pts',(14.9366480584109,-9.0135714452277,3.5237773406849));
#29394=CARTESIAN_POINT('Ctrl Pts',(15.3198145420564,-8.30692757277894,10.5713320220547));
#29395=CARTESIAN_POINT('Ctrl Pts',(14.0272305999403,-10.34046392831,-10.5713320220547));
#29396=CARTESIAN_POINT('Ctrl Pts',(14.5041962611863,-9.69344196054,-3.52377734068488));
#29397=CARTESIAN_POINT('Ctrl Pts',(14.9363207753034,-9.01337050845065,3.52377734068489));
#29398=CARTESIAN_POINT('Ctrl Pts',(15.3194787050451,-8.30674212686605,10.5713320220547));
#29399=CARTESIAN_POINT('Ctrl Pts',(14.0282296344247,-10.3410482545552,-10.5701811473657));
#29400=CARTESIAN_POINT('Ctrl Pts',(14.5051703113035,-9.69405064458535,-3.52339371578857));
#29401=CARTESIAN_POINT('Ctrl Pts',(14.93727643549,-9.0140088944632,3.52339371578857));
#29402=CARTESIAN_POINT('Ctrl Pts',(15.3204236413258,-8.30741386530685,10.5701811473657));
#29403=CARTESIAN_POINT('Ctrl Pts',(14.0272305999403,-10.3404639283101,-10.5713320220547));
#29404=CARTESIAN_POINT('Ctrl Pts',(14.5041962611863,-9.69344196054,-3.52377734068488));
#29405=CARTESIAN_POINT('Ctrl Pts',(14.9363207753034,-9.01337050845065,3.52377734068488));
#29406=CARTESIAN_POINT('Ctrl Pts',(15.3194787050451,-8.30674212686606,10.5713320220547));
#29407=CARTESIAN_POINT('Ctrl Pts',(9.64526772752331,-14.5154164991539,-10.5713320220547));
#29408=CARTESIAN_POINT('Ctrl Pts',(10.314807825219,-14.0705175534734,-3.52377734068489));
#29409=CARTESIAN_POINT('Ctrl Pts',(10.9535126044255,-13.5792225962495,3.52377734068489));
#29410=CARTESIAN_POINT('Ctrl Pts',(11.5552844326327,-13.046221957351,10.5713320220547));
#29411=CARTESIAN_POINT('Ctrl Pts',(9.64505786167931,-14.5150953558215,-10.5713320220547));
#29412=CARTESIAN_POINT('Ctrl Pts',(10.3145831462736,-14.0702060904417,-3.5237773406849));
#29413=CARTESIAN_POINT('Ctrl Pts',(10.9532737833079,-13.5789218399987,3.5237773406849));
#29414=CARTESIAN_POINT('Ctrl Pts',(11.5550322752861,-13.0459328321446,10.5713320220547));
#29415=CARTESIAN_POINT('Ctrl Pts',(9.64484799583672,-14.5147742124913,-10.5713320220547));
#29416=CARTESIAN_POINT('Ctrl Pts',(10.3143584673295,-14.0698946274123,-3.52377734068489));
#29417=CARTESIAN_POINT('Ctrl Pts',(10.953034962192,-13.5786210837499,3.52377734068489));
#29418=CARTESIAN_POINT('Ctrl Pts',(11.5547801179413,-13.0456437069402,10.5713320220547));
#29419=CARTESIAN_POINT('Ctrl Pts',(9.64463813001165,-14.5144530691896,-10.5713320220547));
#29420=CARTESIAN_POINT('Ctrl Pts',(10.3141337884043,-14.0695831644105,-3.52377734068489));
#29421=CARTESIAN_POINT('Ctrl Pts',(10.9527961410962,-13.5783203275278,3.52377734068489));
#29422=CARTESIAN_POINT('Ctrl Pts',(11.5545279606177,-13.0453545817615,10.5713320220547));
#29423=CARTESIAN_POINT('Ctrl Pts',(9.64537706399844,-14.5153438461678,-10.5701811473657));
#29424=CARTESIAN_POINT('Ctrl Pts',(10.3148409139074,-14.070488285077,-3.52339371578857));
#29425=CARTESIAN_POINT('Ctrl Pts',(10.953475827046,-13.579247069187,3.52339371578857));
#29426=CARTESIAN_POINT('Ctrl Pts',(11.55518616219,-13.0463089966596,10.5701811473657));
#29427=CARTESIAN_POINT('Ctrl Pts',(9.64463813001167,-14.5144530691896,-10.5713320220547));
#29428=CARTESIAN_POINT('Ctrl Pts',(10.3141337884043,-14.0695831644105,-3.52377734068489));
#29429=CARTESIAN_POINT('Ctrl Pts',(10.9527961410962,-13.5783203275278,3.52377734068489));
#29430=CARTESIAN_POINT('Ctrl Pts',(11.5545279606177,-13.0453545817615,10.5713320220547));
#29431=CARTESIAN_POINT('Ctrl Pts',(4.09902207758572,-16.9389056224709,-10.5713320220547));
#29432=CARTESIAN_POINT('Ctrl Pts',(4.88034836787775,-16.7498335663957,-3.52377734068489));
#29433=CARTESIAN_POINT('Ctrl Pts',(5.64856730744365,-16.5066172205901,3.52377734068489));
#29434=CARTESIAN_POINT('Ctrl Pts',(6.39634480871554,-16.2115785402758,10.5713320220547));
#29435=CARTESIAN_POINT('Ctrl Pts',(4.09893470568933,-16.9385320681052,-10.5713320220547));
#29436=CARTESIAN_POINT('Ctrl Pts',(4.88024376536137,-16.749464042158,-3.5237773406849));
#29437=CARTESIAN_POINT('Ctrl Pts',(5.6484457536978,-16.5062529205276,3.5237773406849));
#29438=CARTESIAN_POINT('Ctrl Pts',(6.39620674496223,-16.211220608561,10.5713320220547));
#29439=CARTESIAN_POINT('Ctrl Pts',(4.09884733379351,-16.9381585137421,-10.5713320220547));
#29440=CARTESIAN_POINT('Ctrl Pts',(4.88013916284558,-16.749094517923,-3.52377734068488));
#29441=CARTESIAN_POINT('Ctrl Pts',(5.64832419995282,-16.5058886204677,3.52377734068488));
#29442=CARTESIAN_POINT('Ctrl Pts',(6.39606868120983,-16.2108626768487,10.5713320220547));
#29443=CARTESIAN_POINT('Ctrl Pts',(4.09875996190443,-16.9377849594116,-10.5713320220547));
#29444=CARTESIAN_POINT('Ctrl Pts',(4.88003456033808,-16.7487249937203,-3.52377734068489));
#29445=CARTESIAN_POINT('Ctrl Pts',(5.64820264621756,-16.5055243204397,3.52377734068489));
#29446=CARTESIAN_POINT('Ctrl Pts',(6.39593061746862,-16.2105047451678,10.5713320220547));
#29447=CARTESIAN_POINT('Ctrl Pts',(4.09914966904931,-16.9388747462729,-10.5701811473657));
#29448=CARTESIAN_POINT('Ctrl Pts',(4.88038947145514,-16.7498173800975,-3.52339371578857));
#29449=CARTESIAN_POINT('Ctrl Pts',(5.64852437777395,-16.5066276390243,3.52339371578857));
#29450=CARTESIAN_POINT('Ctrl Pts',(6.39622269550887,-16.2116267200009,10.5701811473657));
#29451=CARTESIAN_POINT('Ctrl Pts',(4.09875996190444,-16.9377849594116,-10.5713320220547));
#29452=CARTESIAN_POINT('Ctrl Pts',(4.88003456033808,-16.7487249937204,-3.52377734068489));
#29453=CARTESIAN_POINT('Ctrl Pts',(5.64820264621756,-16.5055243204397,3.52377734068489));
#29454=CARTESIAN_POINT('Ctrl Pts',(6.39593061746862,-16.2105047451678,10.5713320220547));
#29455=CARTESIAN_POINT('Ctrl Pts',(-1.94162613003165,-17.3193127360958,
-10.5713320220547));
#29456=CARTESIAN_POINT('Ctrl Pts',(-1.14275312890046,-17.4088724499949,
-3.52377734068489));
#29457=CARTESIAN_POINT('Ctrl Pts',(-0.337678570790839,-17.4430701964027,
3.52377734068489));
#29458=CARTESIAN_POINT('Ctrl Pts',(0.465911600871797,-17.4215794938256,
10.5713320220547));
#29459=CARTESIAN_POINT('Ctrl Pts',(-1.94158046964024,-17.3189318268663,
-10.5713320220547));
#29460=CARTESIAN_POINT('Ctrl Pts',(-1.14272503838051,-17.4084894346279,
-3.52377734068488));
#29461=CARTESIAN_POINT('Ctrl Pts',(-0.337668195989274,-17.4426862924926,
3.52377734068488));
#29462=CARTESIAN_POINT('Ctrl Pts',(0.465904283238004,-17.4211959274498,
10.5713320220547));
#29463=CARTESIAN_POINT('Ctrl Pts',(-1.9415348092492,-17.3185509176396,-10.5713320220547));
#29464=CARTESIAN_POINT('Ctrl Pts',(-1.14269694786089,-17.4081064192637,
-3.5237773406849));
#29465=CARTESIAN_POINT('Ctrl Pts',(-0.337657821187734,-17.4423023885854,
3.52377734068489));
#29466=CARTESIAN_POINT('Ctrl Pts',(0.465896965604224,-17.4208123610767,
10.5713320220547));
#29467=CARTESIAN_POINT('Ctrl Pts',(-1.94148914886299,-17.3181700084457,
-10.5713320220547));
#29468=CARTESIAN_POINT('Ctrl Pts',(-1.14266885734454,-17.4077234039326,
-3.52377734068489));
#29469=CARTESIAN_POINT('Ctrl Pts',(-0.337647446388026,-17.4419184847113,
3.52377734068489));
#29470=CARTESIAN_POINT('Ctrl Pts',(0.46588964797019,-17.4204287947368,10.5713320220547));
#29471=CARTESIAN_POINT('Ctrl Pts',(-1.94149567299316,-17.319327360811,-10.5701811473657));
#29472=CARTESIAN_POINT('Ctrl Pts',(-1.14270896813208,-17.4088712981013,
-3.52339371578857));
#29473=CARTESIAN_POINT('Ctrl Pts',(-0.337722474799018,-17.4430653037166,
3.52339371578857));
#29474=CARTESIAN_POINT('Ctrl Pts',(0.465780373556112,-17.4215830027813,
10.5701811473657));
#29475=CARTESIAN_POINT('Ctrl Pts',(-1.94148914886299,-17.3181700084457,
-10.5713320220547));
#29476=CARTESIAN_POINT('Ctrl Pts',(-1.14266885734454,-17.4077234039326,
-3.52377734068489));
#29477=CARTESIAN_POINT('Ctrl Pts',(-0.337647446388026,-17.4419184847113,
3.52377734068488));
#29478=CARTESIAN_POINT('Ctrl Pts',(0.465889647970189,-17.4204287947368,
10.5713320220547));
#29479=CARTESIAN_POINT('Ctrl Pts',(-7.74808557101742,-15.6107551279143,
-10.5713320220547));
#29480=CARTESIAN_POINT('Ctrl Pts',(-7.02802173309331,-15.9681443885309,
-3.52377734068488));
#29481=CARTESIAN_POINT('Ctrl Pts',(-6.28319542978303,-16.2756314742303,
3.5237773406849));
#29482=CARTESIAN_POINT('Ctrl Pts',(-5.52071742216,-16.5302808452903,10.5713320220547));
#29483=CARTESIAN_POINT('Ctrl Pts',(-7.7479123856553,-15.6104128070958,-10.5713320220547));
#29484=CARTESIAN_POINT('Ctrl Pts',(-7.0278643376683,-15.9677940793406,-3.52377734068489));
#29485=CARTESIAN_POINT('Ctrl Pts',(-6.28305437778823,-16.2752742709501,
3.5237773406849));
#29486=CARTESIAN_POINT('Ctrl Pts',(-5.52059311105964,-16.5299179080192,
10.5713320220547));
#29487=CARTESIAN_POINT('Ctrl Pts',(-7.74773920029442,-15.6100704862797,
-10.5713320220547));
#29488=CARTESIAN_POINT('Ctrl Pts',(-7.0277069422445,-15.9674437701526,-3.52377734068487));
#29489=CARTESIAN_POINT('Ctrl Pts',(-6.28291332579438,-16.2749170676724,
3.52377734068489));
#29490=CARTESIAN_POINT('Ctrl Pts',(-5.52046879996019,-16.5295549707506,
10.5713320220547));
#29491=CARTESIAN_POINT('Ctrl Pts',(-7.74756601494938,-15.6097281654929,
-10.5713320220547));
#29492=CARTESIAN_POINT('Ctrl Pts',(-7.02754954683515,-15.9670934609948,
-3.52377734068488));
#29493=CARTESIAN_POINT('Ctrl Pts',(-6.28277227381364,-16.2745598644254,
3.5237773406849));
#29494=CARTESIAN_POINT('Ctrl Pts',(-5.52034448887238,-16.5291920335133,
10.5713320220547));
#29495=CARTESIAN_POINT('Ctrl Pts',(-7.74796798344821,-15.6108134895863,
-10.5701811473657));
#29496=CARTESIAN_POINT('Ctrl Pts',(-7.02797984157434,-15.9681584099774,
-3.52339371578857));
#29497=CARTESIAN_POINT('Ctrl Pts',(-6.28323501265835,-16.2756118605541,
3.52339371578857));
#29498=CARTESIAN_POINT('Ctrl Pts',(-5.52084193563372,-16.5302392602447,
10.5701811473657));
#29499=CARTESIAN_POINT('Ctrl Pts',(-7.74756601494938,-15.6097281654929,
-10.5713320220547));
#29500=CARTESIAN_POINT('Ctrl Pts',(-7.02754954683516,-15.9670934609948,
-3.52377734068488));
#29501=CARTESIAN_POINT('Ctrl Pts',(-6.28277227381364,-16.2745598644254,
3.5237773406849));
#29502=CARTESIAN_POINT('Ctrl Pts',(-5.52034448887238,-16.5291920335133,
10.5713320220547));
#29503=CARTESIAN_POINT('Ctrl Pts',(-12.620011542574,-12.019310061098,-10.5713320220547));
#29504=CARTESIAN_POINT('Ctrl Pts',(-12.0656071937211,-12.6014224490979,
-3.52377734068488));
#29505=CARTESIAN_POINT('Ctrl Pts',(-11.4708661898549,-13.1451113935275,
3.52377734068489));
#29506=CARTESIAN_POINT('Ctrl Pts',(-10.8414664469677,-13.6451863658503,
10.5713320220547));
#29507=CARTESIAN_POINT('Ctrl Pts',(-12.6197317209518,-12.0190476176333,
-10.5713320220547));
#29508=CARTESIAN_POINT('Ctrl Pts',(-12.0653394776022,-12.6011470985426,
-3.52377734068489));
#29509=CARTESIAN_POINT('Ctrl Pts',(-11.4706114736191,-13.1448239748645,
3.5237773406849));
#29510=CARTESIAN_POINT('Ctrl Pts',(-10.8412255008865,-13.6448878332752,
10.5713320220547));
#29511=CARTESIAN_POINT('Ctrl Pts',(-12.6194518993316,-12.0187851741704,
-10.5713320220547));
#29512=CARTESIAN_POINT('Ctrl Pts',(-12.0650717614852,-12.6008717479891,
-3.52377734068487));
#29513=CARTESIAN_POINT('Ctrl Pts',(-11.4703567573851,-13.1445365562034,
3.52377734068488));
#29514=CARTESIAN_POINT('Ctrl Pts',(-10.8409845548071,-13.6445893007021,
10.5713320220547));
#29515=CARTESIAN_POINT('Ctrl Pts',(-12.6191720777362,-12.0185227307296,
-10.5713320220547));
#29516=CARTESIAN_POINT('Ctrl Pts',(-12.0648040453921,-12.600596397459,-3.52377734068488));
#29517=CARTESIAN_POINT('Ctrl Pts',(-11.4701020411739,-13.1442491375668,
3.52377734068489));
#29518=CARTESIAN_POINT('Ctrl Pts',(-10.8407436087492,-13.6442907681545,
10.5713320220547));
#29519=CARTESIAN_POINT('Ctrl Pts',(-12.6199210072703,-12.0194051204477,
-10.5701811473657));
#29520=CARTESIAN_POINT('Ctrl Pts',(-12.065572624187,-12.601449952691,-3.52339371578857));
#29521=CARTESIAN_POINT('Ctrl Pts',(-11.4708966773184,-13.1450794245601,
3.52339371578857));
#29522=CARTESIAN_POINT('Ctrl Pts',(-10.8415692284369,-13.6451047025737,
10.5701811473657));
#29523=CARTESIAN_POINT('Ctrl Pts',(-12.6191720777362,-12.0185227307296,
-10.5713320220547));
#29524=CARTESIAN_POINT('Ctrl Pts',(-12.0648040453921,-12.600596397459,-3.52377734068488));
#29525=CARTESIAN_POINT('Ctrl Pts',(-11.4701020411739,-13.1442491375668,
3.52377734068489));
#29526=CARTESIAN_POINT('Ctrl Pts',(-10.8407436087492,-13.6442907681545,
10.5713320220547));
#29527=CARTESIAN_POINT('Ctrl Pts',(-15.9697778705622,-6.97815881478883,
-10.5713320220547));
#29528=CARTESIAN_POINT('Ctrl Pts',(-15.6479023573888,-7.71478298511549,
-3.52377734068489));
#29529=CARTESIAN_POINT('Ctrl Pts',(-15.2749811954754,-8.42909687758284,
3.52377734068489));
#29530=CARTESIAN_POINT('Ctrl Pts',(-14.8545746152671,-9.11428102918566,
10.5713320220547));
#29531=CARTESIAN_POINT('Ctrl Pts',(-15.9694251632972,-6.97800790323301,
-10.5713320220547));
#29532=CARTESIAN_POINT('Ctrl Pts',(-15.647556611091,-7.7146158045359,-3.52377734068489));
#29533=CARTESIAN_POINT('Ctrl Pts',(-15.2746435375359,-8.42891391046955,
3.52377734068488));
#29534=CARTESIAN_POINT('Ctrl Pts',(-14.8542460958585,-9.11408290874099,
10.5713320220547));
#29535=CARTESIAN_POINT('Ctrl Pts',(-15.9690724560347,-6.97785699167819,
-10.5713320220547));
#29536=CARTESIAN_POINT('Ctrl Pts',(-15.6472108647957,-7.71444862395734,
-3.5237773406849));
#29537=CARTESIAN_POINT('Ctrl Pts',(-15.2743058795987,-8.42873094335756,
3.52377734068489));
#29538=CARTESIAN_POINT('Ctrl Pts',(-14.8539175764522,-9.11388478829765,
10.5713320220547));
#29539=CARTESIAN_POINT('Ctrl Pts',(-15.9687197488033,-6.97770608013569,
-10.5713320220547));
#29540=CARTESIAN_POINT('Ctrl Pts',(-15.6468651185308,-7.71428144339257,
-3.52377734068489));
#29541=CARTESIAN_POINT('Ctrl Pts',(-15.2739682216914,-8.42854797626068,
3.52377734068489));
#29542=CARTESIAN_POINT('Ctrl Pts',(-14.8535890570749,-9.11368666787078,
10.5713320220547));
#29543=CARTESIAN_POINT('Ctrl Pts',(-15.9697253074178,-6.97827910625587,
-10.5701811473657));
#29544=CARTESIAN_POINT('Ctrl Pts',(-15.6478792794356,-7.71482065351599,
-3.52339371578857));
#29545=CARTESIAN_POINT('Ctrl Pts',(-15.274998910289,-8.4290564092534,3.52339371578858));
#29546=CARTESIAN_POINT('Ctrl Pts',(-14.8546432677697,-9.11416913747445,
10.5701811473657));
#29547=CARTESIAN_POINT('Ctrl Pts',(-15.9687197488033,-6.97770608013569,
-10.5713320220547));
#29548=CARTESIAN_POINT('Ctrl Pts',(-15.6468651185308,-7.71428144339257,
-3.52377734068489));
#29549=CARTESIAN_POINT('Ctrl Pts',(-15.2739682216914,-8.42854797626068,
3.52377734068489));
#29550=CARTESIAN_POINT('Ctrl Pts',(-14.8535890570749,-9.11368666787078,
10.5713320220547));
#29551=CARTESIAN_POINT('Ctrl Pts',(-17.3933532985407,-1.09533862876043,
-10.5713320220547));
#29552=CARTESIAN_POINT('Ctrl Pts',(-17.3428295583123,-1.89762683505751,
-3.52377734068489));
#29553=CARTESIAN_POINT('Ctrl Pts',(-17.2367080342085,-2.69640887798077,
3.5237773406849));
#29554=CARTESIAN_POINT('Ctrl Pts',(-17.0760018547927,-3.48405888793926,
10.5713320220547));
#29555=CARTESIAN_POINT('Ctrl Pts',(-17.3929702473346,-1.09531745127434,
-10.5713320220547));
#29556=CARTESIAN_POINT('Ctrl Pts',(-17.3424474839418,-1.89758798889885,
-3.52377734068489));
#29557=CARTESIAN_POINT('Ctrl Pts',(-17.2363281610962,-2.69635243095141,
3.5237773406849));
#29558=CARTESIAN_POINT('Ctrl Pts',(-17.0756253863458,-3.48398507587459,
10.5713320220547));
#29559=CARTESIAN_POINT('Ctrl Pts',(-17.3925871961311,-1.09529627378836,
-10.5713320220547));
#29560=CARTESIAN_POINT('Ctrl Pts',(-17.342065409574,-1.89754914274033,-3.52377734068488));
#29561=CARTESIAN_POINT('Ctrl Pts',(-17.2359482879864,-2.69629598392249,
3.52377734068489));
#29562=CARTESIAN_POINT('Ctrl Pts',(-17.0752489179014,-3.48391126381038,
10.5713320220547));
#29563=CARTESIAN_POINT('Ctrl Pts',(-17.392204144961,-1.09527509630334,-10.5713320220547));
#29564=CARTESIAN_POINT('Ctrl Pts',(-17.3416833352395,-1.89751029658436,
-3.52377734068489));
#29565=CARTESIAN_POINT('Ctrl Pts',(-17.2355684149098,-2.69623953689756,
3.5237773406849));
#29566=CARTESIAN_POINT('Ctrl Pts',(-17.07487244949,-3.48383745175174,10.5713320220547));
#29567=CARTESIAN_POINT('Ctrl Pts',(-17.3933450474466,-1.09546964341852,
-10.5701811473657));
#29568=CARTESIAN_POINT('Ctrl Pts',(-17.3428207554817,-1.89767012490037,
-3.52339371578857));
#29569=CARTESIAN_POINT('Ctrl Pts',(-17.2367108397044,-2.6963647913671,3.52339371578857));
#29570=CARTESIAN_POINT('Ctrl Pts',(-17.0760280978237,-3.48393026358512,
10.5701811473657));
#29571=CARTESIAN_POINT('Ctrl Pts',(-17.392204144961,-1.09527509630334,-10.5713320220547));
#29572=CARTESIAN_POINT('Ctrl Pts',(-17.3416833352395,-1.89751029658436,
-3.52377734068489));
#29573=CARTESIAN_POINT('Ctrl Pts',(-17.2355684149098,-2.69623953689756,
3.52377734068489));
#29574=CARTESIAN_POINT('Ctrl Pts',(-17.07487244949,-3.48383745175174,10.5713320220547));
#29575=CARTESIAN_POINT('Ctrl Pts',(-16.7190336201597,4.91959556137296,-10.5713320220547));
#29576=CARTESIAN_POINT('Ctrl Pts',(-16.9459555615988,4.14841111729777,-3.52377734068488));
#29577=CARTESIAN_POINT('Ctrl Pts',(-17.1194334972985,3.36150582706257,3.5237773406849));
#29578=CARTESIAN_POINT('Ctrl Pts',(-17.2378112556832,2.56639217442551,10.5713320220547));
#29579=CARTESIAN_POINT('Ctrl Pts',(-16.7186664266411,4.91948445047194,-10.5713320220547));
#29580=CARTESIAN_POINT('Ctrl Pts',(-16.9455832429635,4.14831694361545,-3.52377734068487));
#29581=CARTESIAN_POINT('Ctrl Pts',(-17.1190572273169,3.36142894566318,3.52377734068489));
#29582=CARTESIAN_POINT('Ctrl Pts',(-17.2374322458487,2.56633277528582,10.5713320220547));
#29583=CARTESIAN_POINT('Ctrl Pts',(-16.718299233125,4.91937333957173,-10.5713320220547));
#29584=CARTESIAN_POINT('Ctrl Pts',(-16.9452109243308,4.14822276993391,-3.52377734068489));
#29585=CARTESIAN_POINT('Ctrl Pts',(-17.1186809573379,3.36135206426428,3.52377734068491));
#29586=CARTESIAN_POINT('Ctrl Pts',(-17.2370532360169,2.56627337614659,10.5713320220547));
#29587=CARTESIAN_POINT('Ctrl Pts',(-16.7179320396407,4.91926222868204,-10.5713320220547));
#29588=CARTESIAN_POINT('Ctrl Pts',(-16.9448386057302,4.14812859626137,-3.52377734068488));
#29589=CARTESIAN_POINT('Ctrl Pts',(-17.1183046873915,3.36127518287297,3.5237773406849));
#29590=CARTESIAN_POINT('Ctrl Pts',(-17.2366742262179,2.5662139770134,10.5713320220547));
#29591=CARTESIAN_POINT('Ctrl Pts',(-16.7190706763197,4.91946962582517,-10.5701811473657));
#29592=CARTESIAN_POINT('Ctrl Pts',(-16.9459620956421,4.14836742740648,-3.52339371578857));
#29593=CARTESIAN_POINT('Ctrl Pts',(-17.1194210550923,3.36154821446419,3.52339371578858));
#29594=CARTESIAN_POINT('Ctrl Pts',(-17.2377919239458,2.56652201742716,10.5701811473657));
#29595=CARTESIAN_POINT('Ctrl Pts',(-16.7179320396407,4.91926222868204,-10.5713320220547));
#29596=CARTESIAN_POINT('Ctrl Pts',(-16.9448386057302,4.14812859626138,-3.52377734068488));
#29597=CARTESIAN_POINT('Ctrl Pts',(-17.1183046873915,3.36127518287298,3.52377734068489));
#29598=CARTESIAN_POINT('Ctrl Pts',(-17.2366742262179,2.5662139770134,10.5713320220547));
#29599=CARTESIAN_POINT('Ctrl Pts',(-14.0281517405305,10.341153921307,-10.5713320220547));
#29600=CARTESIAN_POINT('Ctrl Pts',(-14.5051492284884,9.69408946487939,-3.52377734068488));
#29601=CARTESIAN_POINT('Ctrl Pts',(-14.9373026246845,9.01397331881982,3.5237773406849));
#29602=CARTESIAN_POINT('Ctrl Pts',(-15.3204862161389,8.30729846463996,10.5713320220547));
#29603=CARTESIAN_POINT('Ctrl Pts',(-14.027844693657,10.3409239236334,-10.5713320220547));
#29604=CARTESIAN_POINT('Ctrl Pts',(-14.5048315727105,9.69387363009204,-3.52377734068488));
#29605=CARTESIAN_POINT('Ctrl Pts',(-14.9369753415466,9.01377238202311,3.52377734068489));
#29606=CARTESIAN_POINT('Ctrl Pts',(-15.3201503790965,8.30711301870881,10.5713320220547));
#29607=CARTESIAN_POINT('Ctrl Pts',(-14.0275376467855,10.3406939259613,-10.5713320220547));
#29608=CARTESIAN_POINT('Ctrl Pts',(-14.5045139169348,9.69365779530625,-3.52377734068488));
#29609=CARTESIAN_POINT('Ctrl Pts',(-14.936648058411,9.01357144522771,3.52377734068489));
#29610=CARTESIAN_POINT('Ctrl Pts',(-15.3198145420564,8.30692757277895,10.5713320220547));
#29611=CARTESIAN_POINT('Ctrl Pts',(-14.0272305999403,10.34046392831,-10.5713320220547));
#29612=CARTESIAN_POINT('Ctrl Pts',(-14.5041962611863,9.69344196054,-3.52377734068488));
#29613=CARTESIAN_POINT('Ctrl Pts',(-14.9363207753034,9.01337050845064,3.5237773406849));
#29614=CARTESIAN_POINT('Ctrl Pts',(-15.3194787050451,8.30674212686605,10.5713320220547));
#29615=CARTESIAN_POINT('Ctrl Pts',(-14.0282296344247,10.3410482545552,-10.5701811473657));
#29616=CARTESIAN_POINT('Ctrl Pts',(-14.5051703113035,9.69405064458536,-3.52339371578857));
#29617=CARTESIAN_POINT('Ctrl Pts',(-14.93727643549,9.0140088944632,3.52339371578858));
#29618=CARTESIAN_POINT('Ctrl Pts',(-15.3204236413258,8.30741386530686,10.5701811473657));
#29619=CARTESIAN_POINT('Ctrl Pts',(-14.0272305999403,10.3404639283101,-10.5713320220547));
#29620=CARTESIAN_POINT('Ctrl Pts',(-14.5041962611863,9.69344196054001,-3.52377734068488));
#29621=CARTESIAN_POINT('Ctrl Pts',(-14.9363207753034,9.01337050845065,3.52377734068489));
#29622=CARTESIAN_POINT('Ctrl Pts',(-15.3194787050451,8.30674212686606,10.5713320220547));
#29623=CARTESIAN_POINT('Ctrl Pts',(-9.6452677275233,14.5154164991539,-10.5713320220547));
#29624=CARTESIAN_POINT('Ctrl Pts',(-10.314807825219,14.0705175534734,-3.52377734068489));
#29625=CARTESIAN_POINT('Ctrl Pts',(-10.9535126044255,13.5792225962495,3.52377734068488));
#29626=CARTESIAN_POINT('Ctrl Pts',(-11.5552844326327,13.046221957351,10.5713320220547));
#29627=CARTESIAN_POINT('Ctrl Pts',(-9.6450578616793,14.5150953558215,-10.5713320220547));
#29628=CARTESIAN_POINT('Ctrl Pts',(-10.3145831462735,14.0702060904417,-3.52377734068488));
#29629=CARTESIAN_POINT('Ctrl Pts',(-10.9532737833079,13.5789218399987,3.52377734068487));
#29630=CARTESIAN_POINT('Ctrl Pts',(-11.5550322752861,13.0459328321446,10.5713320220547));
#29631=CARTESIAN_POINT('Ctrl Pts',(-9.64484799583676,14.5147742124914,-10.5713320220547));
#29632=CARTESIAN_POINT('Ctrl Pts',(-10.3143584673296,14.0698946274124,-3.5237773406849));
#29633=CARTESIAN_POINT('Ctrl Pts',(-10.9530349621921,13.5786210837499,3.52377734068489));
#29634=CARTESIAN_POINT('Ctrl Pts',(-11.5547801179413,13.0456437069403,10.5713320220547));
#29635=CARTESIAN_POINT('Ctrl Pts',(-9.64463813001165,14.5144530691896,-10.5713320220547));
#29636=CARTESIAN_POINT('Ctrl Pts',(-10.3141337884043,14.0695831644105,-3.52377734068489));
#29637=CARTESIAN_POINT('Ctrl Pts',(-10.9527961410962,13.5783203275278,3.52377734068488));
#29638=CARTESIAN_POINT('Ctrl Pts',(-11.5545279606177,13.0453545817615,10.5713320220547));
#29639=CARTESIAN_POINT('Ctrl Pts',(-9.64537706399843,14.5153438461678,-10.5701811473657));
#29640=CARTESIAN_POINT('Ctrl Pts',(-10.3148409139074,14.070488285077,-3.52339371578857));
#29641=CARTESIAN_POINT('Ctrl Pts',(-10.953475827046,13.579247069187,3.52339371578858));
#29642=CARTESIAN_POINT('Ctrl Pts',(-11.55518616219,13.0463089966596,10.5701811473657));
#29643=CARTESIAN_POINT('Ctrl Pts',(-9.64463813001165,14.5144530691896,-10.5713320220547));
#29644=CARTESIAN_POINT('Ctrl Pts',(-10.3141337884043,14.0695831644105,-3.52377734068489));
#29645=CARTESIAN_POINT('Ctrl Pts',(-10.9527961410962,13.5783203275278,3.52377734068488));
#29646=CARTESIAN_POINT('Ctrl Pts',(-11.5545279606177,13.0453545817615,10.5713320220547));
#29647=CARTESIAN_POINT('Ctrl Pts',(-4.09902207758572,16.9389056224709,-10.5713320220547));
#29648=CARTESIAN_POINT('Ctrl Pts',(-4.88034836787776,16.7498335663957,-3.52377734068489));
#29649=CARTESIAN_POINT('Ctrl Pts',(-5.64856730744365,16.5066172205901,3.5237773406849));
#29650=CARTESIAN_POINT('Ctrl Pts',(-6.39634480871554,16.2115785402758,10.5713320220547));
#29651=CARTESIAN_POINT('Ctrl Pts',(-4.09893470568933,16.9385320681052,-10.5713320220547));
#29652=CARTESIAN_POINT('Ctrl Pts',(-4.88024376536137,16.749464042158,-3.52377734068488));
#29653=CARTESIAN_POINT('Ctrl Pts',(-5.6484457536978,16.5062529205276,3.52377734068489));
#29654=CARTESIAN_POINT('Ctrl Pts',(-6.39620674496223,16.211220608561,10.5713320220547));
#29655=CARTESIAN_POINT('Ctrl Pts',(-4.09884733379353,16.9381585137421,-10.5713320220547));
#29656=CARTESIAN_POINT('Ctrl Pts',(-4.8801391628456,16.7490945179231,-3.5237773406849));
#29657=CARTESIAN_POINT('Ctrl Pts',(-5.64832419995286,16.5058886204678,3.52377734068491));
#29658=CARTESIAN_POINT('Ctrl Pts',(-6.39606868120986,16.2108626768488,10.5713320220547));
#29659=CARTESIAN_POINT('Ctrl Pts',(-4.09875996190443,16.9377849594116,-10.5713320220547));
#29660=CARTESIAN_POINT('Ctrl Pts',(-4.88003456033808,16.7487249937203,-3.52377734068489));
#29661=CARTESIAN_POINT('Ctrl Pts',(-5.64820264621756,16.5055243204397,3.5237773406849));
#29662=CARTESIAN_POINT('Ctrl Pts',(-6.39593061746862,16.2105047451678,10.5713320220547));
#29663=CARTESIAN_POINT('Ctrl Pts',(-4.09914966904931,16.9388747462729,-10.5701811473657));
#29664=CARTESIAN_POINT('Ctrl Pts',(-4.88038947145514,16.7498173800975,-3.52339371578857));
#29665=CARTESIAN_POINT('Ctrl Pts',(-5.64852437777395,16.5066276390242,3.52339371578857));
#29666=CARTESIAN_POINT('Ctrl Pts',(-6.39622269550887,16.2116267200009,10.5701811473657));
#29667=CARTESIAN_POINT('Ctrl Pts',(-4.09875996190443,16.9377849594116,-10.5713320220547));
#29668=CARTESIAN_POINT('Ctrl Pts',(-4.88003456033808,16.7487249937203,-3.52377734068489));
#29669=CARTESIAN_POINT('Ctrl Pts',(-5.64820264621756,16.5055243204397,3.5237773406849));
#29670=CARTESIAN_POINT('Ctrl Pts',(-6.39593061746862,16.2105047451678,10.5713320220547));
#29671=CARTESIAN_POINT('Ctrl Pts',(1.94162613003165,17.3193127360958,-10.5713320220547));
#29672=CARTESIAN_POINT('Ctrl Pts',(1.14275312890046,17.4088724499949,-3.52377734068488));
#29673=CARTESIAN_POINT('Ctrl Pts',(0.337678570790843,17.4430701964027,3.52377734068491));
#29674=CARTESIAN_POINT('Ctrl Pts',(-0.465911600871794,17.4215794938256,
10.5713320220547));
#29675=CARTESIAN_POINT('Ctrl Pts',(1.94158046964025,17.3189318268663,-10.5713320220547));
#29676=CARTESIAN_POINT('Ctrl Pts',(1.14272503838051,17.4084894346279,-3.52377734068488));
#29677=CARTESIAN_POINT('Ctrl Pts',(0.337668195989281,17.4426862924926,3.52377734068491));
#29678=CARTESIAN_POINT('Ctrl Pts',(-0.465904283238001,17.4211959274498,
10.5713320220547));
#29679=CARTESIAN_POINT('Ctrl Pts',(1.94153480924917,17.3185509176394,-10.5713320220547));
#29680=CARTESIAN_POINT('Ctrl Pts',(1.14269694786086,17.4081064192635,-3.52377734068488));
#29681=CARTESIAN_POINT('Ctrl Pts',(0.337657821187732,17.4423023885852,3.52377734068491));
#29682=CARTESIAN_POINT('Ctrl Pts',(-0.465896965604222,17.4208123610765,
10.5713320220547));
#29683=CARTESIAN_POINT('Ctrl Pts',(1.94148914886299,17.3181700084457,-10.5713320220547));
#29684=CARTESIAN_POINT('Ctrl Pts',(1.14266885734454,17.4077234039326,-3.52377734068488));
#29685=CARTESIAN_POINT('Ctrl Pts',(0.33764744638803,17.4419184847113,3.52377734068491));
#29686=CARTESIAN_POINT('Ctrl Pts',(-0.465889647970186,17.4204287947368,
10.5713320220547));
#29687=CARTESIAN_POINT('Ctrl Pts',(1.94149567299317,17.319327360811,-10.5701811473657));
#29688=CARTESIAN_POINT('Ctrl Pts',(1.14270896813208,17.4088712981013,-3.52339371578857));
#29689=CARTESIAN_POINT('Ctrl Pts',(0.337722474799024,17.4430653037166,3.52339371578858));
#29690=CARTESIAN_POINT('Ctrl Pts',(-0.465780373556106,17.4215830027813,
10.5701811473657));
#29691=CARTESIAN_POINT('Ctrl Pts',(1.941489148863,17.3181700084458,-10.5713320220547));
#29692=CARTESIAN_POINT('Ctrl Pts',(1.14266885734455,17.4077234039326,-3.52377734068489));
#29693=CARTESIAN_POINT('Ctrl Pts',(0.337647446388033,17.4419184847113,3.52377734068488));
#29694=CARTESIAN_POINT('Ctrl Pts',(-0.465889647970182,17.4204287947368,
10.5713320220547));
#29695=CARTESIAN_POINT('Ctrl Pts',(7.74808557101742,15.6107551279143,-10.5713320220547));
#29696=CARTESIAN_POINT('Ctrl Pts',(7.02802173309331,15.9681443885309,-3.52377734068488));
#29697=CARTESIAN_POINT('Ctrl Pts',(6.28319542978303,16.2756314742303,3.52377734068489));
#29698=CARTESIAN_POINT('Ctrl Pts',(5.52071742216,16.5302808452903,10.5713320220547));
#29699=CARTESIAN_POINT('Ctrl Pts',(7.7479123856553,15.6104128070958,-10.5713320220547));
#29700=CARTESIAN_POINT('Ctrl Pts',(7.0278643376683,15.9677940793406,-3.52377734068488));
#29701=CARTESIAN_POINT('Ctrl Pts',(6.28305437778823,16.2752742709501,3.52377734068488));
#29702=CARTESIAN_POINT('Ctrl Pts',(5.52059311105964,16.5299179080192,10.5713320220547));
#29703=CARTESIAN_POINT('Ctrl Pts',(7.74773920029438,15.6100704862796,-10.5713320220547));
#29704=CARTESIAN_POINT('Ctrl Pts',(7.02770694224446,15.9674437701526,-3.52377734068489));
#29705=CARTESIAN_POINT('Ctrl Pts',(6.28291332579435,16.2749170676723,3.52377734068489));
#29706=CARTESIAN_POINT('Ctrl Pts',(5.52046879996016,16.5295549707505,10.5713320220547));
#29707=CARTESIAN_POINT('Ctrl Pts',(7.74756601494938,15.6097281654929,-10.5713320220547));
#29708=CARTESIAN_POINT('Ctrl Pts',(7.02754954683516,15.9670934609948,-3.52377734068488));
#29709=CARTESIAN_POINT('Ctrl Pts',(6.28277227381364,16.2745598644254,3.52377734068489));
#29710=CARTESIAN_POINT('Ctrl Pts',(5.52034448887238,16.5291920335133,10.5713320220547));
#29711=CARTESIAN_POINT('Ctrl Pts',(7.74796798344821,15.6108134895863,-10.5701811473657));
#29712=CARTESIAN_POINT('Ctrl Pts',(7.02797984157433,15.9681584099774,-3.52339371578857));
#29713=CARTESIAN_POINT('Ctrl Pts',(6.28323501265834,16.2756118605541,3.52339371578857));
#29714=CARTESIAN_POINT('Ctrl Pts',(5.52084193563372,16.5302392602447,10.5701811473657));
#29715=CARTESIAN_POINT('Ctrl Pts',(7.74756601494938,15.6097281654929,-10.5713320220547));
#29716=CARTESIAN_POINT('Ctrl Pts',(7.02754954683516,15.9670934609948,-3.52377734068488));
#29717=CARTESIAN_POINT('Ctrl Pts',(6.28277227381364,16.2745598644254,3.52377734068488));
#29718=CARTESIAN_POINT('Ctrl Pts',(5.52034448887238,16.5291920335133,10.5713320220547));
#29719=CARTESIAN_POINT('Ctrl Pts',(12.620011542574,12.019310061098,-10.5713320220547));
#29720=CARTESIAN_POINT('Ctrl Pts',(12.0656071937211,12.6014224490979,-3.52377734068488));
#29721=CARTESIAN_POINT('Ctrl Pts',(11.4708661898549,13.1451113935275,3.5237773406849));
#29722=CARTESIAN_POINT('Ctrl Pts',(10.8414664469677,13.6451863658503,10.5713320220547));
#29723=CARTESIAN_POINT('Ctrl Pts',(12.6197317209518,12.0190476176333,-10.5713320220547));
#29724=CARTESIAN_POINT('Ctrl Pts',(12.0653394776022,12.6011470985426,-3.52377734068489));
#29725=CARTESIAN_POINT('Ctrl Pts',(11.4706114736191,13.1448239748645,3.5237773406849));
#29726=CARTESIAN_POINT('Ctrl Pts',(10.8412255008865,13.6448878332752,10.5713320220547));
#29727=CARTESIAN_POINT('Ctrl Pts',(12.6194518993315,12.0187851741703,-10.5713320220547));
#29728=CARTESIAN_POINT('Ctrl Pts',(12.0650717614851,12.600871747989,-3.52377734068487));
#29729=CARTESIAN_POINT('Ctrl Pts',(11.470356757385,13.1445365562033,3.52377734068489));
#29730=CARTESIAN_POINT('Ctrl Pts',(10.840984554807,13.644589300702,10.5713320220547));
#29731=CARTESIAN_POINT('Ctrl Pts',(12.6191720777362,12.0185227307296,-10.5713320220547));
#29732=CARTESIAN_POINT('Ctrl Pts',(12.0648040453922,12.600596397459,-3.52377734068488));
#29733=CARTESIAN_POINT('Ctrl Pts',(11.4701020411739,13.1442491375668,3.5237773406849));
#29734=CARTESIAN_POINT('Ctrl Pts',(10.8407436087492,13.6442907681545,10.5713320220547));
#29735=CARTESIAN_POINT('Ctrl Pts',(12.6199210072703,12.0194051204477,-10.5701811473657));
#29736=CARTESIAN_POINT('Ctrl Pts',(12.065572624187,12.601449952691,-3.52339371578857));
#29737=CARTESIAN_POINT('Ctrl Pts',(11.4708966773184,13.1450794245601,3.52339371578857));
#29738=CARTESIAN_POINT('Ctrl Pts',(10.8415692284369,13.6451047025737,10.5701811473657));
#29739=CARTESIAN_POINT('Ctrl Pts',(12.6191720777363,12.0185227307296,-10.5713320220547));
#29740=CARTESIAN_POINT('Ctrl Pts',(12.0648040453922,12.600596397459,-3.52377734068488));
#29741=CARTESIAN_POINT('Ctrl Pts',(11.4701020411739,13.1442491375668,3.52377734068489));
#29742=CARTESIAN_POINT('Ctrl Pts',(10.8407436087492,13.6442907681545,10.5713320220547));
#29743=CARTESIAN_POINT('Ctrl Pts',(15.9697778705622,6.97815881478883,-10.5713320220547));
#29744=CARTESIAN_POINT('Ctrl Pts',(15.6479023573888,7.71478298511549,-3.52377734068488));
#29745=CARTESIAN_POINT('Ctrl Pts',(15.2749811954754,8.42909687758284,3.52377734068489));
#29746=CARTESIAN_POINT('Ctrl Pts',(14.8545746152671,9.11428102918567,10.5713320220547));
#29747=CARTESIAN_POINT('Ctrl Pts',(15.9694251632972,6.97800790323301,-10.5713320220547));
#29748=CARTESIAN_POINT('Ctrl Pts',(15.647556611091,7.7146158045359,-3.52377734068489));
#29749=CARTESIAN_POINT('Ctrl Pts',(15.2746435375359,8.42891391046955,3.5237773406849));
#29750=CARTESIAN_POINT('Ctrl Pts',(14.8542460958585,9.11408290874099,10.5713320220547));
#29751=CARTESIAN_POINT('Ctrl Pts',(15.9690724560348,6.9778569916782,-10.5713320220547));
#29752=CARTESIAN_POINT('Ctrl Pts',(15.6472108647957,7.71444862395735,-3.52377734068488));
#29753=CARTESIAN_POINT('Ctrl Pts',(15.2743058795988,8.42873094335758,3.52377734068489));
#29754=CARTESIAN_POINT('Ctrl Pts',(14.8539175764522,9.11388478829766,10.5713320220547));
#29755=CARTESIAN_POINT('Ctrl Pts',(15.9687197488033,6.97770608013569,-10.5713320220547));
#29756=CARTESIAN_POINT('Ctrl Pts',(15.6468651185308,7.71428144339258,-3.52377734068488));
#29757=CARTESIAN_POINT('Ctrl Pts',(15.2739682216914,8.42854797626068,3.52377734068489));
#29758=CARTESIAN_POINT('Ctrl Pts',(14.8535890570749,9.11368666787079,10.5713320220547));
#29759=CARTESIAN_POINT('Ctrl Pts',(15.9697253074178,6.97827910625586,-10.5701811473657));
#29760=CARTESIAN_POINT('Ctrl Pts',(15.6478792794356,7.71482065351598,-3.52339371578857));
#29761=CARTESIAN_POINT('Ctrl Pts',(15.274998910289,8.42905640925339,3.52339371578857));
#29762=CARTESIAN_POINT('Ctrl Pts',(14.8546432677697,9.11416913747444,10.5701811473657));
#29763=CARTESIAN_POINT('Ctrl Pts',(15.9687197488033,6.97770608013569,-10.5713320220547));
#29764=CARTESIAN_POINT('Ctrl Pts',(15.6468651185308,7.71428144339258,-3.52377734068488));
#29765=CARTESIAN_POINT('Ctrl Pts',(15.2739682216914,8.42854797626069,3.52377734068489));
#29766=CARTESIAN_POINT('Ctrl Pts',(14.8535890570749,9.11368666787079,10.5713320220547));
#29767=CARTESIAN_POINT('Ctrl Pts',(17.3933532985407,1.09533862876043,-10.5713320220547));
#29768=CARTESIAN_POINT('Ctrl Pts',(17.3428295583123,1.89762683505751,-3.52377734068489));
#29769=CARTESIAN_POINT('Ctrl Pts',(17.2367080342085,2.69640887798077,3.52377734068489));
#29770=CARTESIAN_POINT('Ctrl Pts',(17.0760018547927,3.48405888793926,10.5713320220547));
#29771=CARTESIAN_POINT('Ctrl Pts',(17.3929702473346,1.09531745127435,-10.5713320220547));
#29772=CARTESIAN_POINT('Ctrl Pts',(17.3424474839418,1.89758798889885,-3.5237773406849));
#29773=CARTESIAN_POINT('Ctrl Pts',(17.2363281610961,2.69635243095141,3.5237773406849));
#29774=CARTESIAN_POINT('Ctrl Pts',(17.0756253863458,3.48398507587458,10.5713320220547));
#29775=CARTESIAN_POINT('Ctrl Pts',(17.3925871961311,1.09529627378836,-10.5713320220547));
#29776=CARTESIAN_POINT('Ctrl Pts',(17.342065409574,1.89754914274033,-3.52377734068488));
#29777=CARTESIAN_POINT('Ctrl Pts',(17.2359482879864,2.69629598392249,3.52377734068488));
#29778=CARTESIAN_POINT('Ctrl Pts',(17.0752489179014,3.48391126381038,10.5713320220547));
#29779=CARTESIAN_POINT('Ctrl Pts',(17.392204144961,1.09527509630334,-10.5713320220547));
#29780=CARTESIAN_POINT('Ctrl Pts',(17.3416833352395,1.89751029658436,-3.52377734068489));
#29781=CARTESIAN_POINT('Ctrl Pts',(17.2355684149098,2.69623953689756,3.52377734068489));
#29782=CARTESIAN_POINT('Ctrl Pts',(17.07487244949,3.48383745175174,10.5713320220547));
#29783=CARTESIAN_POINT('Ctrl Pts',(17.3933450474466,1.09546964341852,-10.5701811473657));
#29784=CARTESIAN_POINT('Ctrl Pts',(17.3428207554817,1.89767012490037,-3.52339371578856));
#29785=CARTESIAN_POINT('Ctrl Pts',(17.2367108397044,2.6963647913671,3.52339371578857));
#29786=CARTESIAN_POINT('Ctrl Pts',(17.0760280978237,3.48393026358512,10.5701811473657));
#29787=CARTESIAN_POINT('Ctrl Pts',(17.392204144961,1.09527509630334,-10.5713320220547));
#29788=CARTESIAN_POINT('Ctrl Pts',(17.3416833352395,1.89751029658436,-3.52377734068489));
#29789=CARTESIAN_POINT('Ctrl Pts',(17.2355684149098,2.69623953689757,3.52377734068489));
#29790=CARTESIAN_POINT('Ctrl Pts',(17.07487244949,3.48383745175174,10.5713320220547));
#29791=CARTESIAN_POINT('Ctrl Pts',(15.5239408288993,-7.92059131757518,-10.5701811473657));
#29792=CARTESIAN_POINT('Ctrl Pts',(15.8892473389622,-7.20460984356022,-3.52339371578857));
#29793=CARTESIAN_POINT('Ctrl Pts',(16.2049399509463,-6.46331998146985,3.52339371578857));
#29794=CARTESIAN_POINT('Ctrl Pts',(16.4680054423355,-5.70379719401242,10.5701811473657));
#29795=CARTESIAN_POINT('Ctrl Pts',(15.5298720746603,-7.92356091115868,-10.5701811473657));
#29796=CARTESIAN_POINT('Ctrl Pts',(15.8953265065073,-7.20730043136479,-3.52339371578857));
#29797=CARTESIAN_POINT('Ctrl Pts',(16.2111160582657,-6.46573988486005,3.52339371578858));
#29798=CARTESIAN_POINT('Ctrl Pts',(16.4742895766427,-5.70592035635592,10.5701811473657));
#29799=CARTESIAN_POINT('Ctrl Pts',(15.5915703928396,-7.95274424871187,-10.5701811473657));
#29800=CARTESIAN_POINT('Ctrl Pts',(15.9583566411062,-7.23364522935241,-3.52339371578857));
#29801=CARTESIAN_POINT('Ctrl Pts',(16.2753221711908,-6.4891298445003,3.52339371578857));
#29802=CARTESIAN_POINT('Ctrl Pts',(16.5394232800143,-5.72631521703215,10.5701811473657));
#29803=CARTESIAN_POINT('Ctrl Pts',(15.8812835900794,-8.05295157643048,-10.5701811473657));
#29804=CARTESIAN_POINT('Ctrl Pts',(16.2527035030447,-7.32048471228393,-3.52339371578857));
#29805=CARTESIAN_POINT('Ctrl Pts',(16.5733417616638,-6.56230076343565,3.52339371578858));
#29806=CARTESIAN_POINT('Ctrl Pts',(16.8401885277462,-5.78560696131593,10.5701811473657));
#29807=CARTESIAN_POINT('Ctrl Pts',(16.634287410633,-8.21708494426133,-10.5701811473657));
#29808=CARTESIAN_POINT('Ctrl Pts',(17.013264495319,-7.44989503894739,-3.52339371578857));
#29809=CARTESIAN_POINT('Ctrl Pts',(17.3390909478701,-6.65644300411585,3.52339371578858));
#29810=CARTESIAN_POINT('Ctrl Pts',(17.6086335808629,-5.84431570465351,10.5701811473657));
#29811=CARTESIAN_POINT('Ctrl Pts',(17.5952076964926,-8.2428856289747,-10.5701811473657));
#29812=CARTESIAN_POINT('Ctrl Pts',(17.9754084721853,-7.43136071700242,-3.52339371578857));
#29813=CARTESIAN_POINT('Ctrl Pts',(18.2992890487802,-6.59354486117992,3.52339371578857));
#29814=CARTESIAN_POINT('Ctrl Pts',(18.5639288924223,-5.73733748808268,10.5701811473657));
#29815=CARTESIAN_POINT('Ctrl Pts',(18.2493498865067,-8.18298767653124,-10.5701811473657));
#29816=CARTESIAN_POINT('Ctrl Pts',(18.6267584093738,-7.34130729556355,-3.52339371578857));
#29817=CARTESIAN_POINT('Ctrl Pts',(18.9458430528698,-6.47348072287577,3.52339371578857));
#29818=CARTESIAN_POINT('Ctrl Pts',(19.2035582177828,-5.58779118888971,10.5701811473657));
#29819=CARTESIAN_POINT('Ctrl Pts',(15.5239408288993,-7.92059131757518,-10.5701811473657));
#29820=CARTESIAN_POINT('Ctrl Pts',(15.8892473389622,-7.20460984356022,-3.52339371578857));
#29821=CARTESIAN_POINT('Ctrl Pts',(16.2049399509463,-6.46331998146985,3.52339371578857));
#29822=CARTESIAN_POINT('Ctrl Pts',(16.4680054423355,-5.70379719401242,10.5701811473657));
#29823=CARTESIAN_POINT('Origin',(-1078.88931916128,445.504381323311,-6.00190077337249));
#29824=CARTESIAN_POINT('Origin',(-1110.51158560065,359.500118245023,6.00190077400118));
#29825=CARTESIAN_POINT('Ctrl Pts',(18.8787605016016,-6.60245423484101,-10.5701811473657));
#29826=CARTESIAN_POINT('Ctrl Pts',(19.1832730585148,-5.73174473391652,-3.52339371578857));
#29827=CARTESIAN_POINT('Ctrl Pts',(19.4274506997862,-4.83994031365006,3.52339371578858));
#29828=CARTESIAN_POINT('Ctrl Pts',(19.6089627989182,-3.93555306794902,10.5701811473657));
#29829=CARTESIAN_POINT('Ctrl Pts',(18.3002407630201,-5.94487823810955,-10.5701811473657));
#29830=CARTESIAN_POINT('Ctrl Pts',(18.5743713266435,-5.10071352016191,-3.52339371578857));
#29831=CARTESIAN_POINT('Ctrl Pts',(18.7901959736259,-4.23795805225981,3.52339371578858));
#29832=CARTESIAN_POINT('Ctrl Pts',(18.9452775557869,-3.36405225652747,10.5701811473657));
#29833=CARTESIAN_POINT('Ctrl Pts',(17.5094185149336,-5.30743865086107,-10.5701811473657));
#29834=CARTESIAN_POINT('Ctrl Pts',(17.7541962099834,-4.49986483819949,-3.52339371578858));
#29835=CARTESIAN_POINT('Ctrl Pts',(17.9430400877725,-3.6753928330489,3.52339371578858));
#29836=CARTESIAN_POINT('Ctrl Pts',(18.0740960265747,-2.84177666010401,10.5701811473657));
#29837=CARTESIAN_POINT('Ctrl Pts',(16.8624899954198,-4.96810854518302,-10.5701811473657));
#29838=CARTESIAN_POINT('Ctrl Pts',(17.0916172376515,-4.19037035031441,-3.52339371578857));
#29839=CARTESIAN_POINT('Ctrl Pts',(17.2668789301514,-3.39682252271119,3.52339371578857));
#29840=CARTESIAN_POINT('Ctrl Pts',(17.3865489833807,-2.59491537643409,10.5701811473657));
#29841=CARTESIAN_POINT('Ctrl Pts',(16.7285940831805,-4.92235069975673,-10.5701811473657));
#29842=CARTESIAN_POINT('Ctrl Pts',(16.9555961741675,-4.15074972008885,-3.52339371578857));
#29843=CARTESIAN_POINT('Ctrl Pts',(17.1292100097174,-3.36359754540394,3.52339371578857));
#29844=CARTESIAN_POINT('Ctrl Pts',(17.2476216804283,-2.56806206701449,10.5701811473657));
#29845=CARTESIAN_POINT('Ctrl Pts',(16.7190706763204,-4.91946962582535,-10.5701811473657));
#29846=CARTESIAN_POINT('Ctrl Pts',(16.9459621050428,-4.14836742961574,-3.52339371578857));
#29847=CARTESIAN_POINT('Ctrl Pts',(17.1194210645505,-3.3615482164125,3.52339371578858));
#29848=CARTESIAN_POINT('Ctrl Pts',(17.2377919239465,-2.56652201742733,10.5701811473657));
#29849=CARTESIAN_POINT('Origin',(-1137.04624834432,263.822186184469,6.0019007738112));
#29850=CARTESIAN_POINT('Origin',(-1112.84749639278,352.202734986488,-6.00190077339977));
#29851=CARTESIAN_POINT('Ctrl Pts',(18.3844122993175,-7.87485773895016,-8.00000002680495));
#29852=CARTESIAN_POINT('Ctrl Pts',(18.4531333976134,-7.71442347504144,-6.66666668453664));
#29853=CARTESIAN_POINT('Ctrl Pts',(18.5197542958142,-7.55308960393423,-5.33333334226832));
#29854=CARTESIAN_POINT('Ctrl Pts',(18.5842521656445,-7.39091140819174,-4.));
#29855=CARTESIAN_POINT('Ctrl Pts',(18.6077644958072,-7.35342624084015,-8.00000002680495));
#29856=CARTESIAN_POINT('Ctrl Pts',(18.6719352556694,-7.19104283587996,-6.66666668453664));
#29857=CARTESIAN_POINT('Ctrl Pts',(18.7339802713311,-7.02781946759158,-5.33333334226832));
#29858=CARTESIAN_POINT('Ctrl Pts',(18.7938783394501,-6.86381191269435,-4.));
#29859=CARTESIAN_POINT('Ctrl Pts',(18.8089193180918,-6.8224871635213,-8.00000002680495));
#29860=CARTESIAN_POINT('Ctrl Pts',(18.8684567600673,-6.65834835144208,-6.66666668453663));
#29861=CARTESIAN_POINT('Ctrl Pts',(18.9258454793725,-6.49343022987757,-5.33333334226832));
#29862=CARTESIAN_POINT('Ctrl Pts',(18.9810658661254,-6.32778915551913,-4.));
#29863=CARTESIAN_POINT('Ctrl Pts',(18.9871493773879,-6.2839604168677,-8.00000002680495));
#29864=CARTESIAN_POINT('Ctrl Pts',(19.041987277425,-6.11826627965564,-6.66666668453664));
#29865=CARTESIAN_POINT('Ctrl Pts',(19.0946561219624,-5.9518542763067,-5.33333334226832));
#29866=CARTESIAN_POINT('Ctrl Pts',(19.1451378635268,-5.78478142945372,-4.));
#29867=CARTESIAN_POINT('Ctrl Pts',(18.9455935099938,-6.40815781282579,4.));
#29868=CARTESIAN_POINT('Ctrl Pts',(19.0015152367791,-6.24282631897105,5.33333334226731));
#29869=CARTESIAN_POINT('Ctrl Pts',(19.0552726553178,-6.07676277090729,6.66666668453462));
#29870=CARTESIAN_POINT('Ctrl Pts',(19.1068473451265,-5.91002407186587,8.00000002680193));
#29871=CARTESIAN_POINT('Ctrl Pts',(19.1273461422817,-5.87080970260819,4.));
#29872=CARTESIAN_POINT('Ctrl Pts',(19.1785786299635,-5.70389209169295,5.33333334226731));
#29873=CARTESIAN_POINT('Ctrl Pts',(19.2276260236414,-5.53630389074425,6.66666668453462));
#29874=CARTESIAN_POINT('Ctrl Pts',(19.2744715615271,-5.36810236813545,8.00000002680193));
#29875=CARTESIAN_POINT('Ctrl Pts',(19.2862238713926,-5.32572490778714,4.));
#29876=CARTESIAN_POINT('Ctrl Pts',(19.332699596505,-5.15742082701962,5.33333334226731));
#29877=CARTESIAN_POINT('Ctrl Pts',(19.3769720788243,-4.98850842595596,6.66666668453462));
#29878=CARTESIAN_POINT('Ctrl Pts',(19.4190261906145,-4.81904542613222,8.00000002680193));
#29879=CARTESIAN_POINT('Ctrl Pts',(19.4216521852328,-4.7748744900616,4.));
#29880=CARTESIAN_POINT('Ctrl Pts',(19.4633208261226,-4.60538860052123,5.33333334226731));
#29881=CARTESIAN_POINT('Ctrl Pts',(19.5027707748587,-4.43535723991919,6.66666668453462));
#29882=CARTESIAN_POINT('Ctrl Pts',(19.5399885135466,-4.26483867109501,8.00000002680193));
#29883=CARTESIAN_POINT('Ctrl Pts',(11.8787308647727,-12.7524216806657,-10.5701811473657));
#29884=CARTESIAN_POINT('Ctrl Pts',(12.4668867829649,-12.2045613578439,-3.52339371578857));
#29885=CARTESIAN_POINT('Ctrl Pts',(13.017076865761,-11.6159499769718,3.52339371578858));
#29886=CARTESIAN_POINT('Ctrl Pts',(13.5240496594282,-10.9922057153483,10.5701811473657));
#29887=CARTESIAN_POINT('Ctrl Pts',(11.8855676953483,-12.7596503467191,-10.5701811473657));
#29888=CARTESIAN_POINT('Ctrl Pts',(12.4741202082517,-12.211467931193,-3.52339371578857));
#29889=CARTESIAN_POINT('Ctrl Pts',(13.0244969705684,-11.6225403214586,3.52339371578858));
#29890=CARTESIAN_POINT('Ctrl Pts',(13.5318181449491,-10.9984223461031,10.5701811473657));
#29891=CARTESIAN_POINT('Ctrl Pts',(11.9863857707243,-12.8589190332262,-10.5701811473657));
#29892=CARTESIAN_POINT('Ctrl Pts',(12.5794765862922,-12.3060905992801,-3.52339371578857));
#29893=CARTESIAN_POINT('Ctrl Pts',(13.1341887566198,-11.7121827924549,3.52339371578858));
#29894=CARTESIAN_POINT('Ctrl Pts',(13.6453640718532,-11.0828372673367,10.5701811473657));
#29895=CARTESIAN_POINT('Ctrl Pts',(12.5792608243648,-13.285711771797,-10.5701811473657));
#29896=CARTESIAN_POINT('Ctrl Pts',(13.1920348426239,-12.7055397408982,-3.52339371578857));
#29897=CARTESIAN_POINT('Ctrl Pts',(13.7645381666776,-12.0829230390925,3.52339371578858));
#29898=CARTESIAN_POINT('Ctrl Pts',(14.2914372818011,-11.4237804859428,10.5701811473657));
#29899=CARTESIAN_POINT('Ctrl Pts',(13.5031269323654,-13.7078792049972,-10.5701811473657));
#29900=CARTESIAN_POINT('Ctrl Pts',(14.1354964096488,-13.0850867185779,-3.52339371578858));
#29901=CARTESIAN_POINT('Ctrl Pts',(14.7242713589907,-12.4185498968891,3.52339371578858));
#29902=CARTESIAN_POINT('Ctrl Pts',(15.264700349594,-11.7144915590678,10.5701811473657));
#29903=CARTESIAN_POINT('Ctrl Pts',(14.3500311789428,-13.9311379708684,-10.5701811473657));
#29904=CARTESIAN_POINT('Ctrl Pts',(14.9925508077551,-13.2692985198616,-3.52339371578857));
#29905=CARTESIAN_POINT('Ctrl Pts',(15.5892064466918,-12.5629417452578,3.52339371578858));
#29906=CARTESIAN_POINT('Ctrl Pts',(16.1343031376281,-11.818809680468,10.5701811473657));
#29907=CARTESIAN_POINT('Ctrl Pts',(11.8787308647727,-12.7524216806657,-10.5701811473657));
#29908=CARTESIAN_POINT('Ctrl Pts',(12.4668867829649,-12.2045613578439,-3.52339371578857));
#29909=CARTESIAN_POINT('Ctrl Pts',(13.017076865761,-11.6159499769718,3.52339371578858));
#29910=CARTESIAN_POINT('Ctrl Pts',(13.5240496594282,-10.9922057153483,10.5701811473657));
#29911=CARTESIAN_POINT('Origin',(-861.45285953215,787.639059256792,-6.00190077325071));
#29912=CARTESIAN_POINT('Origin',(-920.583260311475,717.636939968545,6.00190077196125));
#29913=CARTESIAN_POINT('Ctrl Pts',(15.482059589238,-12.6611938961255,-10.5701811473657));
#29914=CARTESIAN_POINT('Ctrl Pts',(16.0660079802072,-11.9471440316185,-3.52339371578857));
#29915=CARTESIAN_POINT('Ctrl Pts',(16.6004749835089,-11.1926356705744,3.52339371578857));
#29916=CARTESIAN_POINT('Ctrl Pts',(17.0803592190431,-10.4048704436167,10.5701811473657));
#29917=CARTESIAN_POINT('Ctrl Pts',(15.1633330965618,-11.8454091804831,-10.5701811473657));
#29918=CARTESIAN_POINT('Ctrl Pts',(15.7096529021536,-11.1459119989603,-3.52339371578858));
#29919=CARTESIAN_POINT('Ctrl Pts',(16.2075414790933,-10.4090034289244,3.52339371578858));
#29920=CARTESIAN_POINT('Ctrl Pts',(16.6521638829793,-9.64084162637057,10.5701811473657));
#29921=CARTESIAN_POINT('Ctrl Pts',(14.6381973737281,-10.9759350631358,-10.5701811473657));
#29922=CARTESIAN_POINT('Ctrl Pts',(15.1444196786519,-10.3007828129816,-3.52339371578856));
#29923=CARTESIAN_POINT('Ctrl Pts',(15.6038611719969,-9.59062414299819,3.52339371578856));
#29924=CARTESIAN_POINT('Ctrl Pts',(16.0121269935487,-8.85210494768689,10.5701811473657));
#29925=CARTESIAN_POINT('Ctrl Pts',(14.1463497701535,-10.4358061880711,-10.5701811473657));
#29926=CARTESIAN_POINT('Ctrl Pts',(14.6276610777785,-9.78333747767764,-3.52339371578858));
#29927=CARTESIAN_POINT('Ctrl Pts',(15.0637626772863,-9.09759146195833,3.52339371578858));
#29928=CARTESIAN_POINT('Ctrl Pts',(15.4504841403386,-8.38497480280354,10.5701811473657));
#29929=CARTESIAN_POINT('Ctrl Pts',(14.0361933242568,-10.3470127754477,-10.5701811473657));
#29930=CARTESIAN_POINT('Ctrl Pts',(14.5134085917165,-9.69958431635719,-3.52339371578856));
#29931=CARTESIAN_POINT('Ctrl Pts',(14.9457741314539,-9.01928265528841,3.52339371578856));
#29932=CARTESIAN_POINT('Ctrl Pts',(15.3291338629752,-8.31222301326043,10.5701811473657));
#29933=CARTESIAN_POINT('Ctrl Pts',(14.0282296344253,-10.3410482545556,-10.5701811473657));
#29934=CARTESIAN_POINT('Ctrl Pts',(14.5051703193816,-9.6940506498766,-3.52339371578857));
#29935=CARTESIAN_POINT('Ctrl Pts',(14.9372764437114,-9.0140088995289,3.52339371578857));
#29936=CARTESIAN_POINT('Ctrl Pts',(15.3204236413265,-8.30741386530727,10.5701811473657));
#29937=CARTESIAN_POINT('Origin',(-978.241467171257,636.804482391533,6.00190077666473));
#29938=CARTESIAN_POINT('Origin',(-925.274150566318,711.578571311876,-6.00190077008327));
#29939=CARTESIAN_POINT('Ctrl Pts',(14.5823366026094,-13.687785036601,-8.00000002680495));
#29940=CARTESIAN_POINT('Ctrl Pts',(14.7017850615068,-13.5605301425735,-6.66666668453664));
#29941=CARTESIAN_POINT('Ctrl Pts',(14.8195676616555,-13.4317115835623,-5.33333334226832));
#29942=CARTESIAN_POINT('Ctrl Pts',(14.9356440437436,-13.3013735004543,-4.));
#29943=CARTESIAN_POINT('Ctrl Pts',(14.9705590892051,-13.2741906558372,-8.00000002680495));
#29944=CARTESIAN_POINT('Ctrl Pts',(15.0863982741561,-13.1435478609434,-6.66666668453664));
#29945=CARTESIAN_POINT('Ctrl Pts',(15.200527197346,-13.0113887113723,-5.33333334226832));
#29946=CARTESIAN_POINT('Ctrl Pts',(15.3129068573893,-12.8777583681252,-4.));
#29947=CARTESIAN_POINT('Ctrl Pts',(15.3411746506633,-12.8440701239422,-8.00000002680495));
#29948=CARTESIAN_POINT('Ctrl Pts',(15.4532603255808,-12.7101930978845,-6.66666668453664));
#29949=CARTESIAN_POINT('Ctrl Pts',(15.5635934012027,-12.5748488540185,-5.33333334226832));
#29950=CARTESIAN_POINT('Ctrl Pts',(15.6721361751441,-12.4380836433366,-4.));
#29951=CARTESIAN_POINT('Ctrl Pts',(15.6928431172612,-12.3989787844414,-8.00000002680495));
#29952=CARTESIAN_POINT('Ctrl Pts',(15.801044619823,-12.2620328928261,-6.66666668453664));
#29953=CARTESIAN_POINT('Ctrl Pts',(15.9074534016166,-12.1236705670264,-5.33333334226832));
#29954=CARTESIAN_POINT('Ctrl Pts',(16.0120330006756,-11.9839392181901,-4.));
#29955=CARTESIAN_POINT('Ctrl Pts',(15.6113153641544,-12.5014732172219,4.));
#29956=CARTESIAN_POINT('Ctrl Pts',(15.7204112993806,-12.3652387894732,5.33333334226731));
#29957=CARTESIAN_POINT('Ctrl Pts',(15.8277238274038,-12.2275762187696,6.66666668453462));
#29958=CARTESIAN_POINT('Ctrl Pts',(15.9332161765804,-12.0885326764813,8.00000002680193));
#29959=CARTESIAN_POINT('Ctrl Pts',(15.9658908491962,-12.0586942246021,4.));
#29960=CARTESIAN_POINT('Ctrl Pts',(16.0711228250241,-11.9193655201257,5.33333334226731));
#29961=CARTESIAN_POINT('Ctrl Pts',(16.1745308394401,-11.7786593209788,6.66666668453462));
#29962=CARTESIAN_POINT('Ctrl Pts',(16.2760795545783,-11.6366237089603,8.00000002680193));
#29963=CARTESIAN_POINT('Ctrl Pts',(16.3016170584982,-11.6008214488879,4.));
#29964=CARTESIAN_POINT('Ctrl Pts',(16.4028533402584,-11.4585629803066,5.33333334226731));
#29965=CARTESIAN_POINT('Ctrl Pts',(16.5022273088191,-11.3149793242161,6.66666668453462));
#29966=CARTESIAN_POINT('Ctrl Pts',(16.5997050068301,-11.1701195471274,8.00000002680193));
#29967=CARTESIAN_POINT('Ctrl Pts',(16.6172799844809,-11.1295105875044,4.));
#29968=CARTESIAN_POINT('Ctrl Pts',(16.7144032870754,-10.9844974623052,5.33333334226731));
#29969=CARTESIAN_POINT('Ctrl Pts',(16.8096282631161,-10.8382129245663,6.66666668453462));
#29970=CARTESIAN_POINT('Ctrl Pts',(16.9029222828724,-10.6907071000555,8.00000002680193));
#29971=CARTESIAN_POINT('Ctrl Pts',(6.80077064695807,-16.0461217833684,-10.5701811473657));
#29972=CARTESIAN_POINT('Ctrl Pts',(7.54083568928884,-15.7324626522293,-3.52339371578857));
#29973=CARTESIAN_POINT('Ctrl Pts',(8.25916219897089,-15.3675249720875,3.52339371578858));
#29974=CARTESIAN_POINT('Ctrl Pts',(8.94889389387818,-14.9547919997346,10.5701811473657));
#29975=CARTESIAN_POINT('Ctrl Pts',(6.80340542685227,-16.0522091553154,-10.5701811473657));
#29976=CARTESIAN_POINT('Ctrl Pts',(7.54376312530152,-15.7384313756399,-3.52339371578856));
#29977=CARTESIAN_POINT('Ctrl Pts',(8.26233788774653,-15.3733486508924,3.52339371578856));
#29978=CARTESIAN_POINT('Ctrl Pts',(8.95234307759566,-14.960457800119,10.5701811473657));
#29979=CARTESIAN_POINT('Ctrl Pts',(6.8319106026398,-16.1142229628811,-10.5701811473657));
#29980=CARTESIAN_POINT('Ctrl Pts',(7.57511310971885,-15.7991268108376,-3.52339371578859));
#29981=CARTESIAN_POINT('Ctrl Pts',(8.29648793938073,-15.4325364319894,3.52339371578859));
#29982=CARTESIAN_POINT('Ctrl Pts',(8.98912891724076,-15.0179474459438,10.5701811473657));
#29983=CARTESIAN_POINT('Ctrl Pts',(6.98943179288394,-16.3772101395062,-10.5701811473657));
#29984=CARTESIAN_POINT('Ctrl Pts',(7.74477657805409,-16.0548520865028,-3.52339371578856));
#29985=CARTESIAN_POINT('Ctrl Pts',(8.477750844465,-15.6801517612296,3.52339371578856));
#29986=CARTESIAN_POINT('Ctrl Pts',(9.18141647930957,-15.2566955850336,10.5701811473657));
#29987=CARTESIAN_POINT('Ctrl Pts',(7.46076357859375,-16.9869629346763,-10.5701811473657));
#29988=CARTESIAN_POINT('Ctrl Pts',(8.24421702180967,-16.6428631545587,-3.52339371578859));
#29989=CARTESIAN_POINT('Ctrl Pts',(9.0038352824957,-16.2444807757536,3.5233937157886));
#29990=CARTESIAN_POINT('Ctrl Pts',(9.73234227367015,-15.7956138465041,10.5701811473657));
#29991=CARTESIAN_POINT('Ctrl Pts',(8.18028559447488,-17.6243975759657,-10.5701811473657));
#29992=CARTESIAN_POINT('Ctrl Pts',(8.99317441419842,-17.2471218084677,-3.52339371578856));
#29993=CARTESIAN_POINT('Ctrl Pts',(9.77981895378818,-16.8135040854819,3.52339371578856));
#29994=CARTESIAN_POINT('Ctrl Pts',(10.5329043010263,-16.3277184354797,10.5701811473657));
#29995=CARTESIAN_POINT('Ctrl Pts',(8.71988860141418,-17.9989872709252,-10.5701811473657));
#29996=CARTESIAN_POINT('Ctrl Pts',(9.55002197921109,-17.5968162782051,-3.52339371578857));
#29997=CARTESIAN_POINT('Ctrl Pts',(10.3522831255593,-17.137126276613,3.52339371578858));
#29998=CARTESIAN_POINT('Ctrl Pts',(11.1190146190996,-16.6243049148002,10.5701811473657));
#29999=CARTESIAN_POINT('Ctrl Pts',(6.80077064695807,-16.0461217833684,-10.5701811473657));
#30000=CARTESIAN_POINT('Ctrl Pts',(7.54083568928885,-15.7324626522293,-3.52339371578856));
#30001=CARTESIAN_POINT('Ctrl Pts',(8.25916219897089,-15.3675249720875,3.52339371578858));
#30002=CARTESIAN_POINT('Ctrl Pts',(8.94889389387819,-14.9547919997346,10.5701811473657));
#30003=CARTESIAN_POINT('Origin',(-540.112471297088,1034.77284228466,-6.00190077473124));
#30004=CARTESIAN_POINT('Origin',(-619.619007474887,989.216155519852,6.00190077308503));
#30005=CARTESIAN_POINT('Ctrl Pts',(10.2179937997566,-17.1928067231421,-10.5701811473657));
#30006=CARTESIAN_POINT('Ctrl Pts',(11.0109452310822,-16.7215414469562,-3.52339371578858));
#30007=CARTESIAN_POINT('Ctrl Pts',(11.771236988334,-16.1953339887957,3.52339371578858));
#30008=CARTESIAN_POINT('Ctrl Pts',(12.4916122395345,-15.6192068930627,10.5701811473657));
#30009=CARTESIAN_POINT('Ctrl Pts',(10.2026262038395,-16.5361084032577,-10.5701811473657));
#30010=CARTESIAN_POINT('Ctrl Pts',(10.9653007820263,-16.0655207639423,-3.52339371578859));
#30011=CARTESIAN_POINT('Ctrl Pts',(11.6953369617914,-15.5421842200282,3.5233937157886));
#30012=CARTESIAN_POINT('Ctrl Pts',(12.3858181753482,-14.9709041379195,10.5701811473657));
#30013=CARTESIAN_POINT('Ctrl Pts',(10.067006500551,-15.5844556949571,-10.5701811473657));
#30014=CARTESIAN_POINT('Ctrl Pts',(10.7857775294981,-15.1201581991617,-3.52339371578856));
#30015=CARTESIAN_POINT('Ctrl Pts',(11.4723756631221,-14.6060460787458,3.52339371578856));
#30016=CARTESIAN_POINT('Ctrl Pts',(12.1202404623054,-14.047051303605,10.5701811473657));
#30017=CARTESIAN_POINT('Ctrl Pts',(9.81776698398881,-14.8551880626945,-10.5701811473657));
#30018=CARTESIAN_POINT('Ctrl Pts',(10.5029081614888,-14.4023723984214,-3.52339371578859));
#30019=CARTESIAN_POINT('Ctrl Pts',(11.1566607063147,-13.9021132965593,3.52339371578859));
#30020=CARTESIAN_POINT('Ctrl Pts',(11.7728006532305,-13.3591289277863,10.5701811473657));
#30021=CARTESIAN_POINT('Ctrl Pts',(9.685058394327,-14.578848428518,-10.5701811473657));
#30022=CARTESIAN_POINT('Ctrl Pts',(10.357449939268,-14.132166033665,-3.52339371578857));
#30023=CARTESIAN_POINT('Ctrl Pts',(10.9988888810636,-13.6388849853685,3.52339371578857));
#30024=CARTESIAN_POINT('Ctrl Pts',(11.6032469575355,-13.103733729196,10.5701811473657));
#30025=CARTESIAN_POINT('Ctrl Pts',(9.64900602019209,-14.5208962185842,-10.5701811473657));
#30026=CARTESIAN_POINT('Ctrl Pts',(10.3187301172288,-14.0758617811295,-3.52339371578858));
#30027=CARTESIAN_POINT('Ctrl Pts',(10.9576028212757,-13.584458939098,3.52339371578859));
#30028=CARTESIAN_POINT('Ctrl Pts',(11.5595462325571,-13.0513077914043,10.5701811473657));
#30029=CARTESIAN_POINT('Ctrl Pts',(9.6453770639989,-14.5153438461684,-10.5701811473657));
#30030=CARTESIAN_POINT('Ctrl Pts',(10.3148409196886,-14.070488292812,-3.52339371578858));
#30031=CARTESIAN_POINT('Ctrl Pts',(10.9534758330391,-13.5792470767591,3.52339371578858));
#30032=CARTESIAN_POINT('Ctrl Pts',(11.5551861621905,-13.0463089966602,10.5701811473657));
#30033=CARTESIAN_POINT('Origin',(-701.455017753282,932.97478721464,6.0000000302541));
#30034=CARTESIAN_POINT('Origin',(-626.092649606386,985.134825973644,-6.00000002004485));
#30035=CARTESIAN_POINT('Ctrl Pts',(9.02141589925907,-17.8497634486454,-8.00000002680495));
#30036=CARTESIAN_POINT('Ctrl Pts',(9.17718447174341,-17.7710367428009,-6.66666668453663));
#30037=CARTESIAN_POINT('Ctrl Pts',(9.33192245397616,-17.6902709152619,-5.33333334226832));
#30038=CARTESIAN_POINT('Ctrl Pts',(9.48557682353725,-17.6074936411964,-4.));
#30039=CARTESIAN_POINT('Ctrl Pts',(9.52768331452379,-17.5938917715508,-8.00000002680495));
#30040=CARTESIAN_POINT('Ctrl Pts',(9.68121900925412,-17.5107470358699,-6.66666668453663));
#30041=CARTESIAN_POINT('Ctrl Pts',(9.83366620747201,-17.4255924489156,-5.33333334226832));
#30042=CARTESIAN_POINT('Ctrl Pts',(9.98497281389113,-17.3384571088881,-4.));
#30043=CARTESIAN_POINT('Ctrl Pts',(10.0230579087404,-17.3164686691292,-8.00000002680495));
#30044=CARTESIAN_POINT('Ctrl Pts',(10.1741726299965,-17.2290009742501,-6.66666668453663));
#30045=CARTESIAN_POINT('Ctrl Pts',(10.3241422646724,-17.1395551213611,-5.33333334226832));
#30046=CARTESIAN_POINT('Ctrl Pts',(10.4729155653442,-17.0481616772035,-4.));
#30047=CARTESIAN_POINT('Ctrl Pts',(10.5057483754947,-17.0184973211735,-8.00000002680495));
#30048=CARTESIAN_POINT('Ctrl Pts',(10.6542627824881,-16.9268173707899,-6.66666668453663));
#30049=CARTESIAN_POINT('Ctrl Pts',(10.8015770320273,-16.8331932610413,-5.33333334226832));
#30050=CARTESIAN_POINT('Ctrl Pts',(10.9476406455038,-16.7376570731065,-4.));
#30051=CARTESIAN_POINT('Ctrl Pts',(10.3940821869213,-17.0869264495264,4.));
#30052=CARTESIAN_POINT('Ctrl Pts',(10.5431937507156,-16.9962209704763,5.33333334226731));
#30053=CARTESIAN_POINT('Ctrl Pts',(10.6911179135796,-16.9035635148428,6.66666668453462));
#30054=CARTESIAN_POINT('Ctrl Pts',(10.8378039879122,-16.8089858325717,8.00000002680193));
#30055=CARTESIAN_POINT('Ctrl Pts',(10.8787134882441,-16.7921222557363,4.));
#30056=CARTESIAN_POINT('Ctrl Pts',(11.0252524228747,-16.6971875557313,5.33333334226731));
#30057=CARTESIAN_POINT('Ctrl Pts',(11.1705485253506,-16.6003346026057,6.66666668453462));
#30058=CARTESIAN_POINT('Ctrl Pts',(11.3145521439962,-16.5015964922092,8.00000002680193));
#30059=CARTESIAN_POINT('Ctrl Pts',(11.3507946421043,-16.4766877133626,4.));
#30060=CARTESIAN_POINT('Ctrl Pts',(11.4945808908437,-16.3776333277898,5.33333334226731));
#30061=CARTESIAN_POINT('Ctrl Pts',(11.6370703784336,-16.2766967246661,6.66666668453462));
#30062=CARTESIAN_POINT('Ctrl Pts',(11.7782144136678,-16.1739123973319,8.00000002680193));
#30063=CARTESIAN_POINT('Ctrl Pts',(11.8086185726673,-16.1417634540114,4.));
#30064=CARTESIAN_POINT('Ctrl Pts',(11.9494820332864,-16.0387138162183,5.33333334226731));
#30065=CARTESIAN_POINT('Ctrl Pts',(12.0889964991502,-15.9338201755235,6.66666668453462));
#30066=CARTESIAN_POINT('Ctrl Pts',(12.2271141643192,-15.8271184747163,8.00000002680193));
#30067=CARTESIAN_POINT('Ctrl Pts',(0.902537120435115,-17.4044227834609,
-10.5701811473657));
#30068=CARTESIAN_POINT('Ctrl Pts',(1.70524852060254,-17.3627967643357,-3.52339371578857));
#30069=CARTESIAN_POINT('Ctrl Pts',(2.5050706787327,-17.2655496550558,3.52339371578858));
#30070=CARTESIAN_POINT('Ctrl Pts',(3.29436945311861,-17.1136096597291,10.5701811473657));
#30071=CARTESIAN_POINT('Ctrl Pts',(0.903127939532488,-17.4143548929054,
-10.5701811473657));
#30072=CARTESIAN_POINT('Ctrl Pts',(1.70635018607402,-17.3727370626202,-3.52339371578859));
#30073=CARTESIAN_POINT('Ctrl Pts',(2.50651861700806,-17.2753677032605,3.52339371578859));
#30074=CARTESIAN_POINT('Ctrl Pts',(3.29632448506016,-17.1233653614123,10.5701811473657));
#30075=CARTESIAN_POINT('Ctrl Pts',(0.916537850406112,-17.5552227079071,
-10.5701811473657));
#30076=CARTESIAN_POINT('Ctrl Pts',(1.72622304155972,-17.5129629857505,-3.52339371578856));
#30077=CARTESIAN_POINT('Ctrl Pts',(2.53291653419385,-17.4145668679413,3.52339371578856));
#30078=CARTESIAN_POINT('Ctrl Pts',(3.3290350496456,-17.2610373846323,10.5701811473657));
#30079=CARTESIAN_POINT('Ctrl Pts',(1.09636149928822,-18.2632687859998,-10.5701811473657));
#30080=CARTESIAN_POINT('Ctrl Pts',(1.93870102381171,-18.2127147721516,-3.52339371578858));
#30081=CARTESIAN_POINT('Ctrl Pts',(2.77747866403969,-18.1037632822212,3.52339371578859));
#30082=CARTESIAN_POINT('Ctrl Pts',(3.60479546944612,-17.9375150149138,10.5701811473657));
#30083=CARTESIAN_POINT('Ctrl Pts',(1.53274044321678,-19.1804873760835,-10.5701811473657));
#30084=CARTESIAN_POINT('Ctrl Pts',(2.41748686096404,-19.1098799173874,-3.52339371578856));
#30085=CARTESIAN_POINT('Ctrl Pts',(3.29695624953644,-18.9777403313293,3.52339371578857));
#30086=CARTESIAN_POINT('Ctrl Pts',(4.16350885073651,-18.785781413085,10.5701811473657));
#30087=CARTESIAN_POINT('Ctrl Pts',(2.03799876670532,-19.8958930693475,-10.5701811473657));
#30088=CARTESIAN_POINT('Ctrl Pts',(2.95561955666073,-19.8018982920477,-3.52339371578857));
#30089=CARTESIAN_POINT('Ctrl Pts',(3.86672167605729,-19.6443204619612,3.52339371578858));
#30090=CARTESIAN_POINT('Ctrl Pts',(4.76260883832891,-19.4246636277973,10.5701811473657));
#30091=CARTESIAN_POINT('Ctrl Pts',(0.902537120435115,-17.4044227834609,
-10.5701811473657));
#30092=CARTESIAN_POINT('Ctrl Pts',(1.70524852060254,-17.3627967643357,-3.52339371578857));
#30093=CARTESIAN_POINT('Ctrl Pts',(2.5050706787327,-17.2655496550558,3.52339371578858));
#30094=CARTESIAN_POINT('Ctrl Pts',(3.29436945311861,-17.1136096597291,10.5701811473657));
#30095=CARTESIAN_POINT('Origin',(-153.626547848111,1157.09774892851,-6.00190077405241));
#30096=CARTESIAN_POINT('Origin',(-243.919557730996,1141.48130344756,6.00190077308281));
#30097=CARTESIAN_POINT('Ctrl Pts',(3.72148715324783,-19.6507133122286,-10.5701811473657));
#30098=CARTESIAN_POINT('Ctrl Pts',(4.62779997921165,-19.4790741719563,-3.52339371578857));
#30099=CARTESIAN_POINT('Ctrl Pts',(5.52221408340464,-19.244636002305,3.52339371578858));
#30100=CARTESIAN_POINT('Ctrl Pts',(6.39619246301095,-18.9496364684737,10.5701811473657));
#30101=CARTESIAN_POINT('Ctrl Pts',(3.93165039025385,-19.0283627195926,-10.5701811473657));
#30102=CARTESIAN_POINT('Ctrl Pts',(4.80928051528301,-18.8470050560371,-3.52339371578858));
#30103=CARTESIAN_POINT('Ctrl Pts',(5.67428176607205,-18.6049166463696,3.52339371578858));
#30104=CARTESIAN_POINT('Ctrl Pts',(6.51851116280462,-18.3042474524345,10.5701811473657));
#30105=CARTESIAN_POINT('Ctrl Pts',(4.12969891987871,-18.0877210849008,-10.5701811473657));
#30106=CARTESIAN_POINT('Ctrl Pts',(4.96392184787266,-17.8972583245914,-3.52339371578857));
#30107=CARTESIAN_POINT('Ctrl Pts',(5.78495026151904,-17.6489806267712,3.52339371578857));
#30108=CARTESIAN_POINT('Ctrl Pts',(6.58493150569049,-17.3452801729859,10.5701811473657));
#30109=CARTESIAN_POINT('Ctrl Pts',(4.14491130701941,-17.3171860509474,-10.5701811473657));
#30110=CARTESIAN_POINT('Ctrl Pts',(4.94360549410753,-17.1260105963806,-3.52339371578858));
#30111=CARTESIAN_POINT('Ctrl Pts',(5.72903079998526,-16.8795171054837,3.52339371578858));
#30112=CARTESIAN_POINT('Ctrl Pts',(6.49372455310477,-16.5800109738984,10.5701811473657));
#30113=CARTESIAN_POINT('Ctrl Pts',(4.11471950693849,-17.0121225239123,-10.5701811473657));
#30114=CARTESIAN_POINT('Ctrl Pts',(4.89933525670706,-16.8223498262056,-3.52339371578858));
#30115=CARTESIAN_POINT('Ctrl Pts',(5.6708029003471,-16.5782020953567,3.52339371578858));
#30116=CARTESIAN_POINT('Ctrl Pts',(6.42174623445712,-16.2820270448621,10.5701811473657));
#30117=CARTESIAN_POINT('Ctrl Pts',(4.10066074919594,-16.9453334457776,-10.5701811473657));
#30118=CARTESIAN_POINT('Ctrl Pts',(4.88220628322697,-16.756197000563,-3.52339371578857));
#30119=CARTESIAN_POINT('Ctrl Pts',(5.65061991930358,-16.5129367098777,3.52339371578857));
#30120=CARTESIAN_POINT('Ctrl Pts',(6.3986101329639,-16.2178152824268,10.5701811473657));
#30121=CARTESIAN_POINT('Ctrl Pts',(4.09914966904953,-16.9388747462736,-10.5701811473657));
#30122=CARTESIAN_POINT('Ctrl Pts',(4.8803894742422,-16.7498173893433,-3.52339371578857));
#30123=CARTESIAN_POINT('Ctrl Pts',(5.64852438081578,-16.5066276481894,3.52339371578858));
#30124=CARTESIAN_POINT('Ctrl Pts',(6.39622269550912,-16.2116267200016,10.5701811473657));
#30125=CARTESIAN_POINT('Origin',(-340.055933549895,1116.62126860139,6.00000003060113));
#30126=CARTESIAN_POINT('Origin',(-251.39868836428,1139.86022417391,-6.00000002196444));
#30127=CARTESIAN_POINT('Ctrl Pts',(2.37237929653944,-19.8587969543311,-8.00000002680495));
#30128=CARTESIAN_POINT('Ctrl Pts',(2.54567999386982,-19.838094039277,-6.66666668453664));
#30129=CARTESIAN_POINT('Ctrl Pts',(2.71870967383992,-19.8151224939882,-5.33333334226832));
#30130=CARTESIAN_POINT('Ctrl Pts',(2.89140904620798,-19.78989018988,-4.));
#30131=CARTESIAN_POINT('Ctrl Pts',(2.93562831848091,-19.7915098814272,-8.00000002680495));
#30132=CARTESIAN_POINT('Ctrl Pts',(3.10834185226059,-19.765891687168,-6.66666668453664));
#30133=CARTESIAN_POINT('Ctrl Pts',(3.2807199435204,-19.738012562765,-5.33333334226832));
#30134=CARTESIAN_POINT('Ctrl Pts',(3.45270368653351,-19.7078820339451,-4.));
#30135=CARTESIAN_POINT('Ctrl Pts',(3.4960124584432,-19.70024552896,-8.00000002680495));
#30136=CARTESIAN_POINT('Ctrl Pts',(3.66792956043857,-19.6697370601475,-6.66666668453663));
#30137=CARTESIAN_POINT('Ctrl Pts',(3.83944720291044,-19.6369780881742,-5.33333334226832));
#30138=CARTESIAN_POINT('Ctrl Pts',(4.01050677459148,-19.6019798087299,-4.));
#30139=CARTESIAN_POINT('Ctrl Pts',(4.05150533131066,-19.5853339147016,-8.00000002680495));
#30140=CARTESIAN_POINT('Ctrl Pts',(4.22241961341302,-19.549977860618,-6.66666668453664));
#30141=CARTESIAN_POINT('Ctrl Pts',(4.39287105807657,-19.5123844163009,-5.33333334226832));
#30142=CARTESIAN_POINT('Ctrl Pts',(4.56280125851603,-19.4725664634964,-4.));
#30143=CARTESIAN_POINT('Ctrl Pts',(3.92316929763006,-19.6114441758411,4.));
#30144=CARTESIAN_POINT('Ctrl Pts',(4.09431143474655,-19.5772080649333,5.33333334226731));
#30145=CARTESIAN_POINT('Ctrl Pts',(4.26500539528167,-19.5407315809978,6.66666668453462));
#30146=CARTESIAN_POINT('Ctrl Pts',(4.43519268934985,-19.5020272230437,8.00000002680193));
#30147=CARTESIAN_POINT('Ctrl Pts',(4.47940272789801,-19.5001725174983,4.));
#30148=CARTESIAN_POINT('Ctrl Pts',(4.64957386313053,-19.4610823478722,5.33333334226731));
#30149=CARTESIAN_POINT('Ctrl Pts',(4.81923319936554,-19.4197645363123,6.66666668453462));
#30150=CARTESIAN_POINT('Ctrl Pts',(4.98832275984285,-19.3762332008709,8.00000002680193));
#30151=CARTESIAN_POINT('Ctrl Pts',(5.03089887198511,-19.3652222695934,4.));
#30152=CARTESIAN_POINT('Ctrl Pts',(5.19989234404657,-19.3213193878163,5.33333334226731));
#30153=CARTESIAN_POINT('Ctrl Pts',(5.36831101554159,-19.2752042816616,6.66666668453462));
#30154=CARTESIAN_POINT('Ctrl Pts',(5.53609733428556,-19.2268927108936,8.00000002680193));
#30155=CARTESIAN_POINT('Ctrl Pts',(5.57566348434081,-19.207081420908,4.));
#30156=CARTESIAN_POINT('Ctrl Pts',(5.74327689071064,-19.1584245776895,5.33333334226731));
#30157=CARTESIAN_POINT('Ctrl Pts',(5.91025334280012,-19.107573555172,6.66666668453462));
#30158=CARTESIAN_POINT('Ctrl Pts',(6.07653562456276,-19.054545777935,8.00000002680193));
#30159=CARTESIAN_POINT('Ctrl Pts',(-5.10455570284158,-16.6634935339443,
-10.5701811473657));
#30160=CARTESIAN_POINT('Ctrl Pts',(-4.33601678645625,-16.8989213390741,
-3.52339371578858));
#30161=CARTESIAN_POINT('Ctrl Pts',(-3.55116933626636,-17.0810942372497,
3.52339371578857));
#30162=CARTESIAN_POINT('Ctrl Pts',(-2.75750456340204,-17.2082734247813,
10.5701811473657));
#30163=CARTESIAN_POINT('Ctrl Pts',(-5.10739749599094,-16.673028735929,-10.5701811473657));
#30164=CARTESIAN_POINT('Ctrl Pts',(-4.33838134178576,-16.9086389558014,
-3.52339371578857));
#30165=CARTESIAN_POINT('Ctrl Pts',(-3.55316668960767,-17.0908154087531,
3.52339371578856));
#30166=CARTESIAN_POINT('Ctrl Pts',(-2.75900408080094,-17.2181094459668,
10.5701811473657));
#30167=CARTESIAN_POINT('Ctrl Pts',(-5.14297547152451,-16.8099873002577,
-10.5701811473657));
#30168=CARTESIAN_POINT('Ctrl Pts',(-4.36766659600894,-17.0472047963177,
-3.52339371578858));
#30169=CARTESIAN_POINT('Ctrl Pts',(-3.57596927094015,-17.230648054227,3.52339371578858));
#30170=CARTESIAN_POINT('Ctrl Pts',(-2.77535240081307,-17.3586661004476,
10.5701811473657));
#30171=CARTESIAN_POINT('Ctrl Pts',(-5.21616227492136,-17.5368363517824,
-10.5701811473657));
#30172=CARTESIAN_POINT('Ctrl Pts',(-4.40733153621249,-17.7774282041583,
-3.52339371578857));
#30173=CARTESIAN_POINT('Ctrl Pts',(-3.58187484240087,-17.9619260440222,
3.52339371578856));
#30174=CARTESIAN_POINT('Ctrl Pts',(-2.74759107678734,-18.0886627859074,
10.5701811473657));
#30175=CARTESIAN_POINT('Ctrl Pts',(-5.11980806768305,-18.5479914974656,
-10.5701811473657));
#30176=CARTESIAN_POINT('Ctrl Pts',(-4.26426917104801,-18.7842432821223,
-3.52339371578859));
#30177=CARTESIAN_POINT('Ctrl Pts',(-3.39264383327087,-18.9608689271937,
3.52339371578858));
#30178=CARTESIAN_POINT('Ctrl Pts',(-2.51269688917417,-19.0768649830916,
10.5701811473657));
#30179=CARTESIAN_POINT('Ctrl Pts',(-4.8897033552575,-19.3930621535491,-10.5701811473657));
#30180=CARTESIAN_POINT('Ctrl Pts',(-3.99527368840475,-19.6185807284257,
-3.52339371578858));
#30181=CARTESIAN_POINT('Ctrl Pts',(-3.08522288423935,-19.7821212566383,
3.52339371578857));
#30182=CARTESIAN_POINT('Ctrl Pts',(-2.1682371957995,-19.8821227754128,10.5701811473657));
#30183=CARTESIAN_POINT('Ctrl Pts',(-5.10455570284158,-16.6634935339443,
-10.5701811473657));
#30184=CARTESIAN_POINT('Ctrl Pts',(-4.33601678645625,-16.8989213390741,
-3.52339371578858));
#30185=CARTESIAN_POINT('Ctrl Pts',(-3.55116933626636,-17.0810942372497,
3.52339371578857));
#30186=CARTESIAN_POINT('Ctrl Pts',(-2.75750456340204,-17.2082734247813,
10.5701811473657));
#30187=CARTESIAN_POINT('Origin',(251.389004560051,1139.85959012119,-6.00190077265366));
#30188=CARTESIAN_POINT('Origin',(161.200190535201,1156.06695970641,6.00190077397515));
#30189=CARTESIAN_POINT('Ctrl Pts',(-3.22388576724348,-19.738453862219,-10.5701811473657));
#30190=CARTESIAN_POINT('Ctrl Pts',(-2.31352624920543,-19.8871430713012,
-3.52339371578857));
#30191=CARTESIAN_POINT('Ctrl Pts',(-1.39286933918329,-19.9727508933579,
3.52339371578858));
#30192=CARTESIAN_POINT('Ctrl Pts',(-0.470702522298841,-19.9944602189378,
10.5701811473657));
#30193=CARTESIAN_POINT('Ctrl Pts',(-2.81354048537626,-19.2255156632198,
-10.5701811473657));
#30194=CARTESIAN_POINT('Ctrl Pts',(-1.92680995902448,-19.3552623862032,
-3.52339371578858));
#30195=CARTESIAN_POINT('Ctrl Pts',(-1.03117555411549,-19.4236215458326,
3.5233937157886));
#30196=CARTESIAN_POINT('Ctrl Pts',(-0.135024498952067,-19.4298283822643,
10.5701811473657));
#30197=CARTESIAN_POINT('Ctrl Pts',(-2.3057142289943,-18.4093435092557,-10.5701811473657));
#30198=CARTESIAN_POINT('Ctrl Pts',(-1.45665899888873,-18.5156881042564,
-3.52339371578854));
#30199=CARTESIAN_POINT('Ctrl Pts',(-0.600227987416887,-18.5631911577295,
3.52339371578856));
#30200=CARTESIAN_POINT('Ctrl Pts',(0.255380157229872,-18.5514157821675,
10.5701811473657));
#30201=CARTESIAN_POINT('Ctrl Pts',(-2.02788285372484,-17.6904768579848,
-10.5701811473657));
#30202=CARTESIAN_POINT('Ctrl Pts',(-1.21196996348224,-17.7840001943942,
-3.52339371578858));
#30203=CARTESIAN_POINT('Ctrl Pts',(-0.389605628258797,-17.8210031964624,
3.5233937157886));
#30204=CARTESIAN_POINT('Ctrl Pts',(0.431408578760403,-17.8011001617737,
10.5701811473657));
#30205=CARTESIAN_POINT('Ctrl Pts',(-1.95191613165044,-17.3934844692986,
-10.5701811473657));
#30206=CARTESIAN_POINT('Ctrl Pts',(-1.14971241617157,-17.4835108568284,
-3.52339371578855));
#30207=CARTESIAN_POINT('Ctrl Pts',(-0.341266322086584,-17.5179443719088,
3.52339371578856));
#30208=CARTESIAN_POINT('Ctrl Pts',(0.465687420824633,-17.4964686092598,
10.5701811473657));
#30209=CARTESIAN_POINT('Ctrl Pts',(-1.94228472746017,-17.3259133729229,
-10.5701811473657));
#30210=CARTESIAN_POINT('Ctrl Pts',(-1.14318368222263,-17.4154875665979,
-3.52339371578858));
#30211=CARTESIAN_POINT('Ctrl Pts',(-0.337911139204659,-17.449710608455,
3.5233937157886));
#30212=CARTESIAN_POINT('Ctrl Pts',(0.465907217907244,-17.4282149009259,
10.5701811473657));
#30213=CARTESIAN_POINT('Ctrl Pts',(-1.9414956729932,-17.3193273608118,-10.5701811473657));
#30214=CARTESIAN_POINT('Ctrl Pts',(-1.14270896867536,-17.4088713077428,
-3.52339371578857));
#30215=CARTESIAN_POINT('Ctrl Pts',(-0.337722475075313,-17.4430653133694,
3.52339371578858));
#30216=CARTESIAN_POINT('Ctrl Pts',(0.465780373556093,-17.4215830027821,
10.5701811473657));
#30217=CARTESIAN_POINT('Origin',(62.3589149196093,1165.5867454631,6.00000002996901));
#30218=CARTESIAN_POINT('Origin',(153.617664909995,1157.10165684081,-6.00000002140803));
#30219=CARTESIAN_POINT('Ctrl Pts',(-4.5628012619323,-19.4725664626959,-8.00000002680495));
#30220=CARTESIAN_POINT('Ctrl Pts',(-4.39287106149983,-19.5123844155302,
-6.66666668453663));
#30221=CARTESIAN_POINT('Ctrl Pts',(-4.22241961684288,-19.5499778598772,
-5.33333334226832));
#30222=CARTESIAN_POINT('Ctrl Pts',(-4.05150533474672,-19.5853339139908,
-4.));
#30223=CARTESIAN_POINT('Ctrl Pts',(-4.01050677803046,-19.6019798080263,
-8.00000002680495));
#30224=CARTESIAN_POINT('Ctrl Pts',(-3.83944720635556,-19.6369780875006,
-6.66666668453663));
#30225=CARTESIAN_POINT('Ctrl Pts',(-3.66792956388944,-19.669737059504,-5.33333334226832));
#30226=CARTESIAN_POINT('Ctrl Pts',(-3.49601246189942,-19.7002455283466,
-4.));
#30227=CARTESIAN_POINT('Ctrl Pts',(-3.45270368999107,-19.7078820333394,
-8.00000002680495));
#30228=CARTESIAN_POINT('Ctrl Pts',(-3.28071994698324,-19.7380125621894,
-6.66666668453664));
#30229=CARTESIAN_POINT('Ctrl Pts',(-3.10834185572832,-19.7658916866227,
-5.33333334226832));
#30230=CARTESIAN_POINT('Ctrl Pts',(-2.93562832195314,-19.7915098809122,
-4.));
#30231=CARTESIAN_POINT('Ctrl Pts',(-2.89140904967993,-19.7898901893727,
-8.00000002680495));
#30232=CARTESIAN_POINT('Ctrl Pts',(-2.71870967731629,-19.8151224935112,
-6.66666668453663));
#30233=CARTESIAN_POINT('Ctrl Pts',(-2.54567999735022,-19.8380940388304,
-5.33333334226832));
#30234=CARTESIAN_POINT('Ctrl Pts',(-2.37237930002347,-19.8587969539149,
-4.));
#30235=CARTESIAN_POINT('Ctrl Pts',(-3.02093570876772,-19.770532300459,4.));
#30236=CARTESIAN_POINT('Ctrl Pts',(-2.84840526585423,-19.7968949379402,
5.33333334226731));
#30237=CARTESIAN_POINT('Ctrl Pts',(-2.67552971846301,-19.8209990280008,
6.66666668453462));
#30238=CARTESIAN_POINT('Ctrl Pts',(-2.50236830402083,-19.8428363111485,
8.00000002680193));
#30239=CARTESIAN_POINT('Ctrl Pts',(-2.46019011037601,-19.8562141817544,
4.));
#30240=CARTESIAN_POINT('Ctrl Pts',(-2.28691192490911,-19.8776833938736,
5.33333334226731));
#30241=CARTESIAN_POINT('Ctrl Pts',(-2.11335277477,-19.8968842617394,6.66666668453462));
#30242=CARTESIAN_POINT('Ctrl Pts',(-1.93957196895072,-19.9138102227615,
8.00000002680193));
#30243=CARTESIAN_POINT('Ctrl Pts',(-1.8957975502552,-19.9180252198692,4.));
#30244=CARTESIAN_POINT('Ctrl Pts',(-1.72197996168025,-19.9345691773675,
5.33333334226731));
#30245=CARTESIAN_POINT('Ctrl Pts',(-1.5479458836573,-19.9488377305707,6.66666668453462));
#30246=CARTESIAN_POINT('Ctrl Pts',(-1.37375478770641,-19.9608260048063,
8.00000002680193));
#30247=CARTESIAN_POINT('Ctrl Pts',(-1.32979890822622,-19.9557419021113,
4.));
#30248=CARTESIAN_POINT('Ctrl Pts',(-1.15565220662434,-19.967346586858,5.33333334226731));
#30249=CARTESIAN_POINT('Ctrl Pts',(-0.981353592741149,-19.9766715663146,
6.66666668453462));
#30250=CARTESIAN_POINT('Ctrl Pts',(-0.806962791630511,-19.9837136451893,
8.00000002680193));
#30251=CARTESIAN_POINT('Ctrl Pts',(-10.4959637731368,-13.9127010372614,
-10.5701811473657));
#30252=CARTESIAN_POINT('Ctrl Pts',(-9.85429447627607,-14.3967865988031,
-3.52339371578858));
#30253=CARTESIAN_POINT('Ctrl Pts',(-9.17908591963407,-14.8364067643287,
3.52339371578858));
#30254=CARTESIAN_POINT('Ctrl Pts',(-8.47678283314334,-15.2273654477372,
10.5701811473657));
#30255=CARTESIAN_POINT('Ctrl Pts',(-10.4999182019386,-13.9180265095572,
-10.5701811473657));
#30256=CARTESIAN_POINT('Ctrl Pts',(-9.85799982437182,-14.4023061944638,
-3.52339371578858));
#30257=CARTESIAN_POINT('Ctrl Pts',(-9.18254152903514,-14.8420688308859,
3.52339371578858));
#30258=CARTESIAN_POINT('Ctrl Pts',(-8.47996496835057,-15.2331854286516,
10.5701811473657));
#30259=CARTESIAN_POINT('Ctrl Pts',(-10.5393711248066,-13.973719613416,-10.5701811473657));
#30260=CARTESIAN_POINT('Ctrl Pts',(-9.89488859896267,-14.459803788681,-3.52339371578858));
#30261=CARTESIAN_POINT('Ctrl Pts',(-9.21672460434447,-14.9012375244241,
3.52339371578859));
#30262=CARTESIAN_POINT('Ctrl Pts',(-8.51135952136975,-15.2937877139302,
10.5701811473657));
#30263=CARTESIAN_POINT('Ctrl Pts',(-10.6883641017228,-14.2416305529824,
-10.5701811473657));
#30264=CARTESIAN_POINT('Ctrl Pts',(-10.0315214461224,-14.7345992990542,
-3.52339371578858));
#30265=CARTESIAN_POINT('Ctrl Pts',(-9.34053431369458,-15.1820234679673,
3.52339371578859));
#30266=CARTESIAN_POINT('Ctrl Pts',(-8.62197769029708,-15.5796876954148,
10.5701811473657));
#30267=CARTESIAN_POINT('Ctrl Pts',(-10.9807596939227,-14.9546925405834,
-10.5701811473657));
#30268=CARTESIAN_POINT('Ctrl Pts',(-10.2910338072701,-15.4611332407784,
-3.52339371578857));
#30269=CARTESIAN_POINT('Ctrl Pts',(-9.56621540573719,-15.9197907568141,
3.52339371578858));
#30270=CARTESIAN_POINT('Ctrl Pts',(-8.81323173181656,-16.3262628571379,
10.5701811473657));
#30271=CARTESIAN_POINT('Ctrl Pts',(-11.1730334267767,-15.896534887177,-10.5701811473657));
#30272=CARTESIAN_POINT('Ctrl Pts',(-10.4398585735504,-16.4118793808757,
-3.52339371578858));
#30273=CARTESIAN_POINT('Ctrl Pts',(-9.67101229504736,-16.8763246803408,
3.52339371578859));
#30274=CARTESIAN_POINT('Ctrl Pts',(-8.8737668624215,-17.2856229001588,10.5701811473657));
#30275=CARTESIAN_POINT('Ctrl Pts',(-11.2276360580494,-16.5511403577636,
-10.5701811473657));
#30276=CARTESIAN_POINT('Ctrl Pts',(-10.464278995546,-17.068971461469,-3.52339371578858));
#30277=CARTESIAN_POINT('Ctrl Pts',(-9.66504512535763,-17.5339049951292,
3.52339371578858));
#30278=CARTESIAN_POINT('Ctrl Pts',(-8.83756297427066,-17.9415032611597,
10.5701811473657));
#30279=CARTESIAN_POINT('Ctrl Pts',(-10.4959637731368,-13.9127010372614,
-10.5701811473657));
#30280=CARTESIAN_POINT('Ctrl Pts',(-9.85429447627607,-14.3967865988031,
-3.52339371578858));
#30281=CARTESIAN_POINT('Ctrl Pts',(-9.17908591963407,-14.8364067643287,
3.52339371578858));
#30282=CARTESIAN_POINT('Ctrl Pts',(-8.47678283314334,-15.2273654477372,
10.5701811473657));
#30283=CARTESIAN_POINT('Origin',(626.083332913132,985.137542209956,-6.00190077217363));
#30284=CARTESIAN_POINT('Origin',(546.876816795099,1031.21387892502,6.00190077273223));
#30285=CARTESIAN_POINT('Ctrl Pts',(-9.78041048471869,-17.4454455678722,
-10.5701811473657));
#30286=CARTESIAN_POINT('Ctrl Pts',(-8.97580706795737,-17.8965290132744,
-3.52339371578857));
#30287=CARTESIAN_POINT('Ctrl Pts',(-8.13995216290365,-18.2918572602622,
3.52339371578859));
#30288=CARTESIAN_POINT('Ctrl Pts',(-7.28082383659005,-18.6276569801929,
10.5701811473657));
#30289=CARTESIAN_POINT('Ctrl Pts',(-9.21937685503484,-17.1037876794706,
-10.5701811473657));
#30290=CARTESIAN_POINT('Ctrl Pts',(-8.43049871558726,-17.5289894193433,
-3.52339371578856));
#30291=CARTESIAN_POINT('Ctrl Pts',(-7.61225788394638,-17.8995510247446,
3.52339371578858));
#30292=CARTESIAN_POINT('Ctrl Pts',(-6.7722742133858,-18.2118852554664,10.5701811473657));
#30293=CARTESIAN_POINT('Ctrl Pts',(-8.46303091716765,-16.5105131633497,
-10.5701811473657));
#30294=CARTESIAN_POINT('Ctrl Pts',(-7.70155197642183,-16.9008383860245,
-3.52339371578858));
#30295=CARTESIAN_POINT('Ctrl Pts',(-6.91301848801586,-17.2383936822946,
3.5233937157886));
#30296=CARTESIAN_POINT('Ctrl Pts',(-6.10498241256954,-17.5199636690347,
10.5701811473657));
#30297=CARTESIAN_POINT('Ctrl Pts',(-7.95608662604428,-15.9300303080035,
-10.5701811473657));
#30298=CARTESIAN_POINT('Ctrl Pts',(-7.22136616880224,-16.2969721407607,
-3.52339371578855));
#30299=CARTESIAN_POINT('Ctrl Pts',(-6.46125271583016,-16.6130088782682,
3.52339371578857));
#30300=CARTESIAN_POINT('Ctrl Pts',(-5.68294448515699,-16.8751095401972,
10.5701811473657));
#30301=CARTESIAN_POINT('Ctrl Pts',(-7.78312379466279,-15.6769313836482,
-10.5701811473657));
#30302=CARTESIAN_POINT('Ctrl Pts',(-7.0600897208263,-16.0358983454305,-3.52339371578857));
#30303=CARTESIAN_POINT('Ctrl Pts',(-6.31217625428559,-16.3447602199671,
3.52339371578859));
#30304=CARTESIAN_POINT('Ctrl Pts',(-5.54654263333713,-16.6005740390878,
10.5701811473657));
#30305=CARTESIAN_POINT('Ctrl Pts',(-7.75096200091494,-15.6167324440469,
-10.5701811473657));
#30306=CARTESIAN_POINT('Ctrl Pts',(-7.03068882400192,-15.97421330688,-3.52339371578857));
#30307=CARTESIAN_POINT('Ctrl Pts',(-6.28568512728736,-16.2817918773532,
3.52339371578859));
#30308=CARTESIAN_POINT('Ctrl Pts',(-5.52299098368707,-16.5365145893167,
10.5701811473657));
#30309=CARTESIAN_POINT('Ctrl Pts',(-7.74796798344853,-15.610813489587,-10.5701811473657));
#30310=CARTESIAN_POINT('Ctrl Pts',(-7.02797984538244,-15.9681584188516,
-3.52339371578857));
#30311=CARTESIAN_POINT('Ctrl Pts',(-6.28323501621945,-16.2756118695303,
3.52339371578859));
#30312=CARTESIAN_POINT('Ctrl Pts',(-5.52084193563401,-16.5302392602455,
10.5701811473657));
#30313=CARTESIAN_POINT('Origin',(457.252357934138,1073.96525857621,6.0000000290552));
#30314=CARTESIAN_POINT('Origin',(540.105460663215,1034.77955266834,-6.00000002228318));
#30315=CARTESIAN_POINT('Ctrl Pts',(-10.9476406484403,-16.7376570711859,
-8.00000002680495));
#30316=CARTESIAN_POINT('Ctrl Pts',(-10.8015770349805,-16.8331932591463,
-6.66666668453663));
#30317=CARTESIAN_POINT('Ctrl Pts',(-10.6542627854578,-16.9268173689207,
-5.33333334226832));
#30318=CARTESIAN_POINT('Ctrl Pts',(-10.5057483784805,-17.0184973193304,
-4.));
#30319=CARTESIAN_POINT('Ctrl Pts',(-10.4729155683351,-17.0481616753661,
-8.00000002680495));
#30320=CARTESIAN_POINT('Ctrl Pts',(-10.3241422676794,-17.1395551195498,
-6.66666668453663));
#30321=CARTESIAN_POINT('Ctrl Pts',(-10.1741726330192,-17.2290009724651,
-5.33333334226832));
#30322=CARTESIAN_POINT('Ctrl Pts',(-10.0230579117785,-17.3164686673708,
-4.));
#30323=CARTESIAN_POINT('Ctrl Pts',(-9.98497281693299,-17.3384571071364,
-8.00000002680495));
#30324=CARTESIAN_POINT('Ctrl Pts',(-9.83366621052917,-17.4255924471903,
-6.66666668453663));
#30325=CARTESIAN_POINT('Ctrl Pts',(-9.68121901232622,-17.5107470341715,
-5.33333334226832));
#30326=CARTESIAN_POINT('Ctrl Pts',(-9.52768331761047,-17.5938917698793,
-4.));
#30327=CARTESIAN_POINT('Ctrl Pts',(-9.48557682662632,-17.6074936395323,
-8.00000002680495));
#30328=CARTESIAN_POINT('Ctrl Pts',(-9.33192245707975,-17.6902709136247,
-6.66666668453663));
#30329=CARTESIAN_POINT('Ctrl Pts',(-9.17718447486117,-17.7710367411908,
-5.33333334226832));
#30330=CARTESIAN_POINT('Ctrl Pts',(-9.02141590239064,-17.8497634470626,
-4.));
#30331=CARTESIAN_POINT('Ctrl Pts',(-9.60067128442543,-17.5450024476604,
4.));
#30332=CARTESIAN_POINT('Ctrl Pts',(-9.44756225340845,-17.6287841103792,
5.33333334226731));
#30333=CARTESIAN_POINT('Ctrl Pts',(-9.29335646154787,-17.7105614654362,
6.66666668453462));
#30334=CARTESIAN_POINT('Ctrl Pts',(-9.13810674890371,-17.7903064910541,
8.00000002680193));
#30335=CARTESIAN_POINT('Ctrl Pts',(-9.10304771279965,-17.8173033691799,
4.));
#30336=CARTESIAN_POINT('Ctrl Pts',(-8.94756238357933,-17.896742459211,5.33333334226731));
#30337=CARTESIAN_POINT('Ctrl Pts',(-8.79103721450315,-17.9741460984632,
6.66666668453462));
#30338=CARTESIAN_POINT('Ctrl Pts',(-8.63352569325523,-18.0494878352489,
8.00000002680193));
#30339=CARTESIAN_POINT('Ctrl Pts',(-8.59383280894276,-18.0684203698839,
4.));
#30340=CARTESIAN_POINT('Ctrl Pts',(-8.43615607031084,-18.1434157212207,
5.33333334226731));
#30341=CARTESIAN_POINT('Ctrl Pts',(-8.27749766403898,-18.2163469356839,
6.66666668453462));
#30342=CARTESIAN_POINT('Ctrl Pts',(-8.11791180783962,-18.2871890921223,
8.00000002680193));
#30343=CARTESIAN_POINT('Ctrl Pts',(-8.07486792671951,-18.2974453945363,
4.));
#30344=CARTESIAN_POINT('Ctrl Pts',(-7.91519259223034,-18.3679119110009,
5.33333334226731));
#30345=CARTESIAN_POINT('Ctrl Pts',(-7.75459480176133,-18.436288162287,6.66666668453462));
#30346=CARTESIAN_POINT('Ctrl Pts',(-7.59312958565075,-18.5025507186311,
8.00000002680193));
#30347=CARTESIAN_POINT('Ctrl Pts',(-14.6214037084642,-9.48383146588572,
-10.5701811473657));
#30348=CARTESIAN_POINT('Ctrl Pts',(-14.1839988183597,-10.1581869207755,
-3.52339371578858));
#30349=CARTESIAN_POINT('Ctrl Pts',(-13.6998692722136,-10.8022296735859,
3.52339371578857));
#30350=CARTESIAN_POINT('Ctrl Pts',(-13.1736359892169,-11.4098124657167,
10.5701811473657));
#30351=CARTESIAN_POINT('Ctrl Pts',(-14.629709758007,-9.48930918495498,-10.5701811473657));
#30352=CARTESIAN_POINT('Ctrl Pts',(-14.1920565364589,-10.1641111402022,
-3.52339371578859));
#30353=CARTESIAN_POINT('Ctrl Pts',(-13.7076479822362,-10.8083926490174,
3.52339371578858));
#30354=CARTESIAN_POINT('Ctrl Pts',(-13.1811071587349,-11.4163834238845,
10.5701811473657));
#30355=CARTESIAN_POINT('Ctrl Pts',(-14.7449772223306,-9.57135777968372,
-10.5701811473657));
#30356=CARTESIAN_POINT('Ctrl Pts',(-14.3035366338093,-10.2514358632125,
-3.52339371578857));
#30357=CARTESIAN_POINT('Ctrl Pts',(-13.814976378559,-10.9008517199746,3.52339371578856));
#30358=CARTESIAN_POINT('Ctrl Pts',(-13.2839566880577,-11.5135458371245,
10.5701811473657));
#30359=CARTESIAN_POINT('Ctrl Pts',(-15.2682377029356,-10.0811139468335,
-10.5701811473657));
#30360=CARTESIAN_POINT('Ctrl Pts',(-14.803286880418,-10.7853243667584,-3.52339371578858));
#30361=CARTESIAN_POINT('Ctrl Pts',(-14.2895432842683,-11.4572463383408,
3.52339371578858));
#30362=CARTESIAN_POINT('Ctrl Pts',(-13.7319096587417,-12.0905995751469,
10.5701811473657));
#30363=CARTESIAN_POINT('Ctrl Pts',(-15.8444191030467,-10.9176358492754,
-10.5701811473657));
#30364=CARTESIAN_POINT('Ctrl Pts',(-15.3408980412456,-11.6485449936037,
-3.52339371578858));
#30365=CARTESIAN_POINT('Ctrl Pts',(-14.7867271085875,-12.3441180329291,
3.52339371578857));
#30366=CARTESIAN_POINT('Ctrl Pts',(-14.1872095083049,-12.9985951401617,
10.5701811473657));
#30367=CARTESIAN_POINT('Ctrl Pts',(-16.211349445681,-11.7129052395219,-10.5701811473657));
#30368=CARTESIAN_POINT('Ctrl Pts',(-15.6711371857387,-12.4605907660142,
-3.52339371578858));
#30369=CARTESIAN_POINT('Ctrl Pts',(-15.0791197221122,-13.1708394318101,
3.52339371578857));
#30370=CARTESIAN_POINT('Ctrl Pts',(-14.4409477424756,-13.8368720561798,
10.5701811473657));
#30371=CARTESIAN_POINT('Ctrl Pts',(-14.6214037084642,-9.48383146588572,
-10.5701811473657));
#30372=CARTESIAN_POINT('Ctrl Pts',(-14.1839988183597,-10.1581869207755,
-3.52339371578858));
#30373=CARTESIAN_POINT('Ctrl Pts',(-13.6998692722136,-10.8022296735859,
3.52339371578857));
#30374=CARTESIAN_POINT('Ctrl Pts',(-13.1736359892169,-11.4098124657167,
10.5701811473657));
#30375=CARTESIAN_POINT('Origin',(925.262771311062,711.593367601486,-6.00190077290402));
#30376=CARTESIAN_POINT('Origin',(866.592027874508,781.98118522266,6.0019007749759));
#30377=CARTESIAN_POINT('Ctrl Pts',(-15.1572749937985,-13.048259399505,-10.5701811473657));
#30378=CARTESIAN_POINT('Ctrl Pts',(-14.5554747099748,-13.7473298360336,
-3.52339371578857));
#30379=CARTESIAN_POINT('Ctrl Pts',(-13.9052382267708,-14.4046961615238,
3.52339371578859));
#30380=CARTESIAN_POINT('Ctrl Pts',(-13.2127719211995,-15.0140839465072,
10.5701811473657));
#30381=CARTESIAN_POINT('Ctrl Pts',(-14.5132212402647,-12.9190907809461,
-10.5701811473657));
#30382=CARTESIAN_POINT('Ctrl Pts',(-13.9173458198838,-13.5884619754075,
-3.52339371578857));
#30383=CARTESIAN_POINT('Ctrl Pts',(-13.2751904647928,-14.2165308697908,
3.52339371578859));
#30384=CARTESIAN_POINT('Ctrl Pts',(-12.5926885865131,-14.7973204175046,
10.5701811473657));
#30385=CARTESIAN_POINT('Ctrl Pts',(-13.5995757049001,-12.6202782881533,
-10.5701811473657));
#30386=CARTESIAN_POINT('Ctrl Pts',(-13.0175186447629,-13.2475051691757,
-3.52339371578856));
#30387=CARTESIAN_POINT('Ctrl Pts',(-12.3919905548983,-13.8343977109152,
3.52339371578858));
#30388=CARTESIAN_POINT('Ctrl Pts',(-11.7289876157166,-14.3753515760175,
10.5701811473657));
#30389=CARTESIAN_POINT('Ctrl Pts',(-12.9246670155629,-12.248189293022,-10.5701811473657));
#30390=CARTESIAN_POINT('Ctrl Pts',(-12.3597571218172,-12.8442910215617,
-3.52339371578857));
#30391=CARTESIAN_POINT('Ctrl Pts',(-11.7535751536795,-13.4012425136373,
3.52339371578859));
#30392=CARTESIAN_POINT('Ctrl Pts',(-11.1118483586176,-13.9137336641164,
10.5701811473657));
#30393=CARTESIAN_POINT('Ctrl Pts',(-12.6755702093799,-12.069510984306,-10.5701811473657));
#30394=CARTESIAN_POINT('Ctrl Pts',(-12.1189143573446,-12.6541218069529,
-3.52339371578856));
#30395=CARTESIAN_POINT('Ctrl Pts',(-11.5217426633956,-13.2001584938273,
3.52339371578858));
#30396=CARTESIAN_POINT('Ctrl Pts',(-10.8897758786539,-13.7024069727144,
10.5701811473657));
#30397=CARTESIAN_POINT('Ctrl Pts',(-12.6247588650341,-12.0239431039853,
-10.5701811473657));
#30398=CARTESIAN_POINT('Ctrl Pts',(-12.0701891316818,-12.6062131680627,
-3.52339371578857));
#30399=CARTESIAN_POINT('Ctrl Pts',(-11.4753127221783,-13.1500487521764,
3.52339371578859));
#30400=CARTESIAN_POINT('Ctrl Pts',(-10.8457349619751,-13.6502665652626,
10.5701811473657));
#30401=CARTESIAN_POINT('Ctrl Pts',(-12.6199210072709,-12.0194051204483,
-10.5701811473657));
#30402=CARTESIAN_POINT('Ctrl Pts',(-12.0655726308006,-12.6014499597276,
-3.52339371578857));
#30403=CARTESIAN_POINT('Ctrl Pts',(-11.4708966837347,-13.145079431777,3.52339371578859));
#30404=CARTESIAN_POINT('Ctrl Pts',(-10.8415692284374,-13.6451047025743,
10.5701811473657));
#30405=CARTESIAN_POINT('Origin',(796.999839514323,852.799843231391,6.00190076950591));
#30406=CARTESIAN_POINT('Origin',(861.440263999451,787.652834922883,-6.00190077470093));
#30407=CARTESIAN_POINT('Ctrl Pts',(-16.0120330027781,-11.983939215381,-8.00000002680495));
#30408=CARTESIAN_POINT('Ctrl Pts',(-15.9074534037436,-12.1236705642356,
-6.66666668453663));
#30409=CARTESIAN_POINT('Ctrl Pts',(-15.8010446219743,-12.262032890054,-5.33333334226832));
#30410=CARTESIAN_POINT('Ctrl Pts',(-15.6928431194365,-12.3989787816882,
-4.));
#30411=CARTESIAN_POINT('Ctrl Pts',(-15.6721361773262,-12.4380836405871,
-8.00000002680495));
#30412=CARTESIAN_POINT('Ctrl Pts',(-15.5635934034088,-12.574848851288,-6.66666668453663));
#30413=CARTESIAN_POINT('Ctrl Pts',(-15.4532603278107,-12.7101930951734,
-5.33333334226832));
#30414=CARTESIAN_POINT('Ctrl Pts',(-15.3411746529166,-12.8440701212508,
-4.));
#30415=CARTESIAN_POINT('Ctrl Pts',(-15.3129068596485,-12.8777583654387,
-8.00000002680495));
#30416=CARTESIAN_POINT('Ctrl Pts',(-15.2005271996287,-13.0113887087055,
-6.66666668453663));
#30417=CARTESIAN_POINT('Ctrl Pts',(-15.086398276462,-13.1435478582967,-5.33333334226832));
#30418=CARTESIAN_POINT('Ctrl Pts',(-14.970559091534,-13.2741906532108,-4.));
#30419=CARTESIAN_POINT('Ctrl Pts',(-14.9356440460772,-13.3013734978339,
-8.00000002680495));
#30420=CARTESIAN_POINT('Ctrl Pts',(-14.819567664012,-13.4317115809623,-6.66666668453663));
#30421=CARTESIAN_POINT('Ctrl Pts',(-14.7017850638858,-13.5605301399942,
-5.33333334226832));
#30422=CARTESIAN_POINT('Ctrl Pts',(-14.5823366050108,-13.6877850340427,
-4.));
#30423=CARTESIAN_POINT('Ctrl Pts',(-15.0224242123638,-13.2032863630154,
4.));
#30424=CARTESIAN_POINT('Ctrl Pts',(-14.9072038020326,-13.3343817459623,
5.33333334226731));
#30425=CARTESIAN_POINT('Ctrl Pts',(-14.7902672600361,-13.4639688100905,
6.66666668453462));
#30426=CARTESIAN_POINT('Ctrl Pts',(-14.6716546557766,-13.5920031511778,
8.00000002680193));
#30427=CARTESIAN_POINT('Ctrl Pts',(-14.6479434143837,-13.6293628148902,
4.));
#30428=CARTESIAN_POINT('Ctrl Pts',(-14.529004766833,-13.7571902561793,5.33333334226731));
#30429=CARTESIAN_POINT('Ctrl Pts',(-14.4083928242758,-13.8834606455681,
6.66666668453462));
#30430=CARTESIAN_POINT('Ctrl Pts',(-14.2861488016842,-14.0081308327355,
8.00000002680193));
#30431=CARTESIAN_POINT('Ctrl Pts',(-14.2553249994075,-14.0394973618063,
4.));
#30432=CARTESIAN_POINT('Ctrl Pts',(-14.1328072524584,-14.1638985607967,
5.33333334226731));
#30433=CARTESIAN_POINT('Ctrl Pts',(-14.0086610632827,-14.2866958557057,
6.66666668453462));
#30434=CARTESIAN_POINT('Ctrl Pts',(-13.8829288563289,-14.4078472847614,
8.00000002680193));
#30435=CARTESIAN_POINT('Ctrl Pts',(-13.845988700892,-14.4322069308464,4.));
#30436=CARTESIAN_POINT('Ctrl Pts',(-13.7200439354119,-14.5530359771683,
5.33333334226731));
#30437=CARTESIAN_POINT('Ctrl Pts',(-13.5925174320586,-14.6722163152528,
6.66666668453462));
#30438=CARTESIAN_POINT('Ctrl Pts',(-13.4634528889838,-14.78970710684,8.00000002680193));
#30439=CARTESIAN_POINT('Ctrl Pts',(-16.9832865676143,-3.9110718532786,-10.5701811473657));
#30440=CARTESIAN_POINT('Ctrl Pts',(-16.8029035694212,-4.69435998123014,
-3.52339371578858));
#30441=CARTESIAN_POINT('Ctrl Pts',(-16.5682462020274,-5.46514426027785,
3.52339371578857));
#30442=CARTESIAN_POINT('Ctrl Pts',(-16.2815542228302,-6.21606770943294,
10.5701811473657));
#30443=CARTESIAN_POINT('Ctrl Pts',(-16.9897389834304,-3.91260954390051,
-10.5701811473657));
#30444=CARTESIAN_POINT('Ctrl Pts',(-16.8092899584403,-4.69620648496864,
-3.52339371578857));
#30445=CARTESIAN_POINT('Ctrl Pts',(-16.5745328586343,-5.46726043199346,
3.52339371578856));
#30446=CARTESIAN_POINT('Ctrl Pts',(-16.2877328914428,-6.21848063638771,
10.5701811473657));
#30447=CARTESIAN_POINT('Ctrl Pts',(-17.0557613661602,-3.92991270646709,
-10.5701811473657));
#30448=CARTESIAN_POINT('Ctrl Pts',(-16.8745079936752,-4.71654017008887,
-3.52339371578859));
#30449=CARTESIAN_POINT('Ctrl Pts',(-16.6387524141882,-5.4906135647581,3.52339371578858));
#30450=CARTESIAN_POINT('Ctrl Pts',(-16.3507378099998,-6.2447243917162,10.5701811473657));
#30451=CARTESIAN_POINT('Ctrl Pts',(-17.3421065865861,-4.03937349046946,
-10.5701811473657));
#30452=CARTESIAN_POINT('Ctrl Pts',(-17.1558101221976,-4.83921977956265,
-3.52339371578857));
#30453=CARTESIAN_POINT('Ctrl Pts',(-16.9140820327623,-5.62612468710591,
3.52339371578857));
#30454=CARTESIAN_POINT('Ctrl Pts',(-16.6192493625611,-6.39263245314736,
10.5701811473657));
#30455=CARTESIAN_POINT('Ctrl Pts',(-18.0244436775357,-4.39766136660583,
-10.5701811473657));
#30456=CARTESIAN_POINT('Ctrl Pts',(-17.8216168089674,-5.228964691362,-3.52339371578859));
#30457=CARTESIAN_POINT('Ctrl Pts',(-17.5611932309208,-6.04622142745372,
3.52339371578858));
#30458=CARTESIAN_POINT('Ctrl Pts',(-17.2456495103602,-6.84160568476503,
10.5701811473657));
#30459=CARTESIAN_POINT('Ctrl Pts',(-18.7771350612562,-4.99556415374903,
-10.5701811473657));
#30460=CARTESIAN_POINT('Ctrl Pts',(-18.5467476225913,-5.86161661525365,
-3.52339371578857));
#30461=CARTESIAN_POINT('Ctrl Pts',(-18.2563169179228,-6.71160718410693,
3.52339371578856));
#30462=CARTESIAN_POINT('Ctrl Pts',(-17.9086833416741,-7.5376072656065,10.5701811473657));
#30463=CARTESIAN_POINT('Ctrl Pts',(-19.2397349758694,-5.46192256062901,
-10.5701811473657));
#30464=CARTESIAN_POINT('Ctrl Pts',(-18.9878250124769,-6.34928060711398,
-3.52339371578858));
#30465=CARTESIAN_POINT('Ctrl Pts',(-18.6744299210032,-7.21917793504633,
3.52339371578857));
#30466=CARTESIAN_POINT('Ctrl Pts',(-18.3025409945928,-8.06331154931088,
10.5701811473657));
#30467=CARTESIAN_POINT('Ctrl Pts',(-16.9832865676143,-3.9110718532786,-10.5701811473657));
#30468=CARTESIAN_POINT('Ctrl Pts',(-16.8029035694212,-4.69435998123014,
-3.52339371578857));
#30469=CARTESIAN_POINT('Ctrl Pts',(-16.5682462020274,-5.46514426027785,
3.52339371578857));
#30470=CARTESIAN_POINT('Ctrl Pts',(-16.2815542228302,-6.21606770943294,
10.5701811473657));
#30471=CARTESIAN_POINT('Origin',(1112.84186408303,352.22053088442,-6.00190077374882));
#30472=CARTESIAN_POINT('Origin',(1081.78345087015,438.430019756215,6.0019007731347));
#30473=CARTESIAN_POINT('Ctrl Pts',(-18.7059453597305,-7.07725995777758,
-10.5701811473657));
#30474=CARTESIAN_POINT('Ctrl Pts',(-18.3795342330452,-7.93999903151655,
-3.52339371578857));
#30475=CARTESIAN_POINT('Ctrl Pts',(-17.9933443266979,-8.78011521479376,
3.52339371578858));
#30476=CARTESIAN_POINT('Ctrl Pts',(-17.551061745707,-9.58958976753269,10.5701811473657));
#30477=CARTESIAN_POINT('Ctrl Pts',(-18.0565552078921,-7.17616029669807,
-10.5701811473657));
#30478=CARTESIAN_POINT('Ctrl Pts',(-17.7255539028776,-8.00896482032151,
-3.52339371578857));
#30479=CARTESIAN_POINT('Ctrl Pts',(-17.3369374692435,-8.81878654729076,
3.52339371578857));
#30480=CARTESIAN_POINT('Ctrl Pts',(-16.8942372196888,-9.59797954490641,
10.5701811473657));
#30481=CARTESIAN_POINT('Ctrl Pts',(-17.0958111919986,-7.20785561730533,
-10.5701811473657));
#30482=CARTESIAN_POINT('Ctrl Pts',(-16.7633806977716,-7.99633131329317,
-3.52339371578859));
#30483=CARTESIAN_POINT('Ctrl Pts',(-16.3763053385158,-8.76177323989865,
3.52339371578859));
#30484=CARTESIAN_POINT('Ctrl Pts',(-15.9383034918166,-9.4968639410666,10.5701811473657));
#30485=CARTESIAN_POINT('Ctrl Pts',(-16.3343420851164,-7.08903734849994,
-10.5701811473657));
#30486=CARTESIAN_POINT('Ctrl Pts',(-16.0073792251724,-7.84240030692992,
-3.52339371578856));
#30487=CARTESIAN_POINT('Ctrl Pts',(-15.6282430292672,-8.57309000696062,
3.52339371578857));
#30488=CARTESIAN_POINT('Ctrl Pts',(-15.2004993921048,-9.27415764976285,
10.5701811473657));
#30489=CARTESIAN_POINT('Ctrl Pts',(-16.0391560118722,-7.00633068060142,
-10.5701811473657));
#30490=CARTESIAN_POINT('Ctrl Pts',(-15.7160192927446,-7.74607267098129,
-3.52339371578858));
#30491=CARTESIAN_POINT('Ctrl Pts',(-15.3416169168209,-8.46342410640397,
3.52339371578859));
#30492=CARTESIAN_POINT('Ctrl Pts',(-14.9195414893457,-9.15152866611954,
10.5701811473657));
#30493=CARTESIAN_POINT('Ctrl Pts',(-15.9758234884504,-6.98088877109859,
-10.5701811473657));
#30494=CARTESIAN_POINT('Ctrl Pts',(-15.6538464930777,-7.7177176733025,-3.52339371578857));
#30495=CARTESIAN_POINT('Ctrl Pts',(-15.2808482452117,-8.43221567345478,
3.52339371578858));
#30496=CARTESIAN_POINT('Ctrl Pts',(-14.8603232378632,-9.11759493697741,
10.5701811473657));
#30497=CARTESIAN_POINT('Ctrl Pts',(-15.9697253074185,-6.97827910625621,
-10.5701811473657));
#30498=CARTESIAN_POINT('Ctrl Pts',(-15.647879288057,-7.71482065786623,-3.52339371578857));
#30499=CARTESIAN_POINT('Ctrl Pts',(-15.2749989187867,-8.42905641384053,
3.52339371578858));
#30500=CARTESIAN_POINT('Ctrl Pts',(-14.8546432677704,-9.11416913747482,
10.5701811473657));
#30501=CARTESIAN_POINT('Origin',(1040.60718933536,528.788968262105,6.00000003130594));
#30502=CARTESIAN_POINT('Origin',(1078.88826202955,445.514028129078,-6.00000002167999));
#30503=CARTESIAN_POINT('Ctrl Pts',(-19.1451378645417,-5.78478142609487,
-8.00000002680495));
#30504=CARTESIAN_POINT('Ctrl Pts',(-19.0946561230066,-5.95185427295671,
-6.66666668453663));
#30505=CARTESIAN_POINT('Ctrl Pts',(-19.0419872784984,-6.11826627631489,
-5.33333334226832));
#30506=CARTESIAN_POINT('Ctrl Pts',(-18.9871493784903,-6.28396041353657,
-4.));
#30507=CARTESIAN_POINT('Ctrl Pts',(-18.9810658672356,-6.32778915218907,
-8.00000002680495));
#30508=CARTESIAN_POINT('Ctrl Pts',(-18.9258454805117,-6.4934302265572,-6.66666668453663));
#30509=CARTESIAN_POINT('Ctrl Pts',(-18.8684567612354,-6.65834834813178,
-5.33333334226832));
#30510=CARTESIAN_POINT('Ctrl Pts',(-18.8089193192887,-6.82248716022144,
-4.));
#30511=CARTESIAN_POINT('Ctrl Pts',(-18.7938783406543,-6.86381190939714,
-8.00000002680495));
#30512=CARTESIAN_POINT('Ctrl Pts',(-18.733980272564,-7.02781946430487,-6.66666668453663));
#30513=CARTESIAN_POINT('Ctrl Pts',(-18.671935256931,-7.19104283260413,-5.33333334226832));
#30514=CARTESIAN_POINT('Ctrl Pts',(-18.6077644970973,-7.35342623757559,
-4.));
#30515=CARTESIAN_POINT('Ctrl Pts',(-18.5842521669411,-7.3909114049313,-8.00000002680495));
#30516=CARTESIAN_POINT('Ctrl Pts',(-18.5197542971393,-7.5530896006851,-6.66666668453663));
#30517=CARTESIAN_POINT('Ctrl Pts',(-18.4531333989669,-7.714423471804,-5.33333334226832));
#30518=CARTESIAN_POINT('Ctrl Pts',(-18.3844123006991,-7.87485773572478,
-4.));
#30519=CARTESIAN_POINT('Ctrl Pts',(-18.6322510729221,-7.26905908323709,
4.));
#30520=CARTESIAN_POINT('Ctrl Pts',(-18.5688165652349,-7.43165614846694,
5.33333334226731));
#30521=CARTESIAN_POINT('Ctrl Pts',(-18.5032535458669,-7.5934228092312,6.66666668453462));
#30522=CARTESIAN_POINT('Ctrl Pts',(-18.4355844806013,-7.75430363466721,
8.00000002680193));
#30523=CARTESIAN_POINT('Ctrl Pts',(-18.4260809595722,-7.79751995715235,
4.));
#30524=CARTESIAN_POINT('Ctrl Pts',(-18.3580347499332,-7.95831787374795,
5.33333334226731));
#30525=CARTESIAN_POINT('Ctrl Pts',(-18.2878836142101,-8.11822494076053,
6.66666668453462));
#30526=CARTESIAN_POINT('Ctrl Pts',(-18.215651523529,-8.2771865138012,8.00000002680193));
#30527=CARTESIAN_POINT('Ctrl Pts',(-18.1974146087534,-8.31720377098127,
4.));
#30528=CARTESIAN_POINT('Ctrl Pts',(-18.1248333019387,-8.47600619706092,
5.33333334226731));
#30529=CARTESIAN_POINT('Ctrl Pts',(-18.0501731924764,-8.63385840635456,
6.66666668453462));
#30530=CARTESIAN_POINT('Ctrl Pts',(-17.9734597945365,-8.7907064576789,8.00000002680193));
#30531=CARTESIAN_POINT('Ctrl Pts',(-17.9470788927071,-8.82623131460692,
4.));
#30532=CARTESIAN_POINT('Ctrl Pts',(-17.8700554936997,-8.9828491245528,5.33333334226731));
#30533=CARTESIAN_POINT('Ctrl Pts',(-17.7909818558573,-9.13845864174832,
6.66666668453462));
#30534=CARTESIAN_POINT('Ctrl Pts',(-17.7098850745029,-9.2930065451338,8.00000002680193));
#30535=CARTESIAN_POINT('Ctrl Pts',(-17.2967344200949,2.13342074610697,-10.5701811473657));
#30536=CARTESIAN_POINT('Ctrl Pts',(-17.3951301655649,1.33567605342619,-3.52339371578857));
#30537=CARTESIAN_POINT('Ctrl Pts',(-17.438248118605,0.531118207758816,3.52339371578858));
#30538=CARTESIAN_POINT('Ctrl Pts',(-17.4256767270215,-0.272573448002652,
10.5701811473657));
#30539=CARTESIAN_POINT('Ctrl Pts',(-17.30661823314,2.13456359558458,-10.5701811473657));
#30540=CARTESIAN_POINT('Ctrl Pts',(-17.4051107505851,1.33631723941113,-3.52339371578859));
#30541=CARTESIAN_POINT('Ctrl Pts',(-17.44816844044,0.531397153098151,3.52339371578859));
#30542=CARTESIAN_POINT('Ctrl Pts',(-17.4356237054098,-0.272804718797141,
10.5701811473657));
#30543=CARTESIAN_POINT('Ctrl Pts',(-17.4476874812993,2.1458310833851,-10.5701811473657));
#30544=CARTESIAN_POINT('Ctrl Pts',(-17.5466701372071,1.34110850589665,-3.52339371578856));
#30545=CARTESIAN_POINT('Ctrl Pts',(-17.5898512960806,0.529582293917762,
3.52339371578856));
#30546=CARTESIAN_POINT('Ctrl Pts',(-17.5768988000171,-0.28110150741043,
10.5701811473657));
#30547=CARTESIAN_POINT('Ctrl Pts',(-18.1762105609743,2.0916981433591,-10.5701811473657));
#30548=CARTESIAN_POINT('Ctrl Pts',(-18.272695299601,1.25337703656126,-3.52339371578858));
#30549=CARTESIAN_POINT('Ctrl Pts',(-18.3110538115194,0.408420040147072,
3.52339371578859));
#30550=CARTESIAN_POINT('Ctrl Pts',(-18.2909932845622,-0.435196672672694,
10.5701811473657));
#30551=CARTESIAN_POINT('Ctrl Pts',(-19.1552502593208,1.82120200778524,-10.5701811473657));
#30552=CARTESIAN_POINT('Ctrl Pts',(-19.2393500897156,0.937636019605693,
-3.52339371578856));
#30553=CARTESIAN_POINT('Ctrl Pts',(-19.2619362575252,0.0485819488860323,
3.52339371578857));
#30554=CARTESIAN_POINT('Ctrl Pts',(-19.2233689066293,-0.83813908750873,
10.5701811473657));
#30555=CARTESIAN_POINT('Ctrl Pts',(-19.947524519721,1.44784858846758,-10.5701811473657));
#30556=CARTESIAN_POINT('Ctrl Pts',(-20.0143009122587,0.527846498406004,
-3.52339371578857));
#30557=CARTESIAN_POINT('Ctrl Pts',(-20.0173282661883,-0.396777035596819,
3.52339371578858));
#30558=CARTESIAN_POINT('Ctrl Pts',(-19.9565776860253,-1.31719666779067,
10.5701811473657));
#30559=CARTESIAN_POINT('Ctrl Pts',(-17.2967344200949,2.13342074610697,-10.5701811473657));
#30560=CARTESIAN_POINT('Ctrl Pts',(-17.3951301655649,1.33567605342619,-3.52339371578857));
#30561=CARTESIAN_POINT('Ctrl Pts',(-17.438248118605,0.531118207758816,3.52339371578858));
#30562=CARTESIAN_POINT('Ctrl Pts',(-17.4256767270215,-0.272573448002652,
10.5701811473657));
#30563=CARTESIAN_POINT('Origin',(1166.19580421585,-49.6353000928601,-6.00190077381567));
#30564=CARTESIAN_POINT('Origin',(1166.49582424222,41.9977233811867,6.00190077396116));
#30565=CARTESIAN_POINT('Ctrl Pts',(-19.9984042844753,-0.25263884473002,
-10.5701811473657));
#30566=CARTESIAN_POINT('Ctrl Pts',(-19.9867522990396,-1.1749875663182,-3.52339371578857));
#30567=CARTESIAN_POINT('Ctrl Pts',(-19.9111891512377,-2.09652327146644,
3.52339371578858));
#30568=CARTESIAN_POINT('Ctrl Pts',(-19.7724360761246,-3.00845008713017,
10.5701811473657));
#30569=CARTESIAN_POINT('Ctrl Pts',(-19.4220030588742,-0.567679276212883,
-10.5701811473657));
#30570=CARTESIAN_POINT('Ctrl Pts',(-19.3957994976135,-1.46346865540102,
-3.52339371578857));
#30571=CARTESIAN_POINT('Ctrl Pts',(-19.3075948457377,-2.35736680471636,
3.52339371578857));
#30572=CARTESIAN_POINT('Ctrl Pts',(-19.158092388734,-3.24098111754682,10.5701811473657));
#30573=CARTESIAN_POINT('Ctrl Pts',(-18.5300476618897,-0.926064023779522,
-10.5701811473657));
#30574=CARTESIAN_POINT('Ctrl Pts',(-18.487339750091,-1.78068674224966,-3.52339371578858));
#30575=CARTESIAN_POINT('Ctrl Pts',(-18.385403393272,-2.63235550918581,3.52339371578858));
#30576=CARTESIAN_POINT('Ctrl Pts',(-18.225232117009,-3.47292027106663,10.5701811473657));
#30577=CARTESIAN_POINT('Ctrl Pts',(-17.7738570494612,-1.07484441701443,
-10.5701811473657));
#30578=CARTESIAN_POINT('Ctrl Pts',(-17.7242777697192,-1.89460191404476,
-3.52339371578857));
#30579=CARTESIAN_POINT('Ctrl Pts',(-17.617916529176,-2.71089820703327,3.52339371578857));
#30580=CARTESIAN_POINT('Ctrl Pts',(-17.4557482454186,-3.51598323773522,
10.5701811473657));
#30581=CARTESIAN_POINT('Ctrl Pts',(-17.4681851433452,-1.09808483323811,
-10.5701811473657));
#30582=CARTESIAN_POINT('Ctrl Pts',(-17.4175426144497,-1.90373418987339,
-3.52339371578858));
#30583=CARTESIAN_POINT('Ctrl Pts',(-17.311067802437,-2.70587750222895,3.52339371578858));
#30584=CARTESIAN_POINT('Ctrl Pts',(-17.1497922579605,-3.49684257752213,
10.5701811473657));
#30585=CARTESIAN_POINT('Ctrl Pts',(-17.3999680211064,-1.09583622546326,
-10.5701811473657));
#30586=CARTESIAN_POINT('Ctrl Pts',(-17.3494189412302,-1.898351525751,-3.52339371578857));
#30587=CARTESIAN_POINT('Ctrl Pts',(-17.2432879485624,-2.69733293825569,
3.52339371578857));
#30588=CARTESIAN_POINT('Ctrl Pts',(-17.0825372162436,-3.48520679791294,
10.5701811473657));
#30589=CARTESIAN_POINT('Ctrl Pts',(-17.3933450474474,-1.09546964341861,
-10.5701811473657));
#30590=CARTESIAN_POINT('Ctrl Pts',(-17.342820765071,-1.89767012603957,-3.52339371578857));
#30591=CARTESIAN_POINT('Ctrl Pts',(-17.2367108492585,-2.6963647927712,3.52339371578858));
#30592=CARTESIAN_POINT('Ctrl Pts',(-17.0760280978245,-3.48393026358523,
10.5701811473657));
#30593=CARTESIAN_POINT('Origin',(1158.70737566477,140.990471381257,6.00000003038105));
#30594=CARTESIAN_POINT('Origin',(1166.19811020393,49.6447266790377,-6.00000002178777));
#30595=CARTESIAN_POINT('Ctrl Pts',(-19.9690565476993,1.1121063774595,-8.00000002680495));
#30596=CARTESIAN_POINT('Ctrl Pts',(-19.9787615067239,0.937843483654576,
-6.66666668453663));
#30597=CARTESIAN_POINT('Ctrl Pts',(-19.9861852394339,0.763453546341202,
-5.33333334226832));
#30598=CARTESIAN_POINT('Ctrl Pts',(-19.9913252020177,0.588996321866058,
-4.));
#30599=CARTESIAN_POINT('Ctrl Pts',(-20.0005988828589,0.545730096184685,
-8.00000002680495));
#30600=CARTESIAN_POINT('Ctrl Pts',(-20.0053612769335,0.371191916320092,
-6.66666668453664));
#30601=CARTESIAN_POINT('Ctrl Pts',(-20.0078388404912,0.196591476450452,
-5.33333334226832));
#30602=CARTESIAN_POINT('Ctrl Pts',(-20.0080307256696,0.0219884415173641,
-4.));
#30603=CARTESIAN_POINT('Ctrl Pts',(-20.0080307256734,-0.0219884380071468,
-8.00000002680495));
#30604=CARTESIAN_POINT('Ctrl Pts',(-20.0078388405257,-0.196591472940268,
-6.66666668453663));
#30605=CARTESIAN_POINT('Ctrl Pts',(-20.0053612769986,-0.371191912810343,
-5.33333334226832));
#30606=CARTESIAN_POINT('Ctrl Pts',(-20.0005988829546,-0.545730092675771,
-4.));
#30607=CARTESIAN_POINT('Ctrl Pts',(-19.991325202121,-0.588996318358771,
-8.00000002680495));
#30608=CARTESIAN_POINT('Ctrl Pts',(-19.9861852395679,-0.763453542834817,
-6.66666668453663));
#30609=CARTESIAN_POINT('Ctrl Pts',(-19.9787615068885,-0.937843480149494,
-5.33333334226832));
#30610=CARTESIAN_POINT('Ctrl Pts',(-19.9690565478944,-1.11210637395612,
-4.));
#30611=CARTESIAN_POINT('Ctrl Pts',(-19.9947534713468,-0.458075998134003,
4.));
#30612=CARTESIAN_POINT('Ctrl Pts',(-19.9907560041241,-0.632563139902935,
5.33333334226731));
#30613=CARTESIAN_POINT('Ctrl Pts',(-19.9844743751274,-0.806997950593388,
6.66666668453462));
#30614=CARTESIAN_POINT('Ctrl Pts',(-19.9759107368159,-0.981320658482395,
8.00000002680193));
#30615=CARTESIAN_POINT('Ctrl Pts',(-19.9817612010437,-1.02518111344366,
4.));
#30616=CARTESIAN_POINT('Ctrl Pts',(-19.972814806454,-1.19955490347979,5.33333334226731));
#30617=CARTESIAN_POINT('Ctrl Pts',(-19.9615857398537,-1.37381149585751,
6.66666668453462));
#30618=CARTESIAN_POINT('Ctrl Pts',(-19.9480778372514,-1.54789134303979,
8.00000002680193));
#30619=CARTESIAN_POINT('Ctrl Pts',(-19.9446274510471,-1.59173265652136,
4.));
#30620=CARTESIAN_POINT('Ctrl Pts',(-19.9307369611545,-1.76578239343086,
5.33333334226731));
#30621=CARTESIAN_POINT('Ctrl Pts',(-19.9145680424726,-1.93965021101785,
6.66666668453462));
#30622=CARTESIAN_POINT('Ctrl Pts',(-19.8961262215074,-2.11327669479037,
8.00000002680193));
#30623=CARTESIAN_POINT('Ctrl Pts',(-19.8834864993867,-2.15568194052487,
4.));
#30624=CARTESIAN_POINT('Ctrl Pts',(-19.8646746255167,-2.32919809478258,
5.33333334226731));
#30625=CARTESIAN_POINT('Ctrl Pts',(-19.8435913009115,-2.50246798676344,
6.66666668453462));
#30626=CARTESIAN_POINT('Ctrl Pts',(-19.8202437499699,-2.67543224391478,
8.00000002680193));
#30627=CARTESIAN_POINT('Ctrl Pts',(-15.5239408288993,7.92059131757517,-10.5701811473657));
#30628=CARTESIAN_POINT('Ctrl Pts',(-15.8892473389622,7.2046098435602,-3.52339371578858));
#30629=CARTESIAN_POINT('Ctrl Pts',(-16.2049399509463,6.46331998146983,3.52339371578858));
#30630=CARTESIAN_POINT('Ctrl Pts',(-16.4680054423355,5.7037971940124,10.5701811473657));
#30631=CARTESIAN_POINT('Ctrl Pts',(-15.5328376975401,7.92504570795004,-10.5701811473657));
#30632=CARTESIAN_POINT('Ctrl Pts',(-15.8984067225336,7.20862592241769,-3.52339371578858));
#30633=CARTESIAN_POINT('Ctrl Pts',(-16.2141665992448,6.4669750542426,3.52339371578858));
#30634=CARTESIAN_POINT('Ctrl Pts',(-16.4774316437956,5.70698193752737,10.5701811473657));
#30635=CARTESIAN_POINT('Ctrl Pts',(-15.6615319819844,7.98385473667208,-10.5701811473657));
#30636=CARTESIAN_POINT('Ctrl Pts',(-16.0297765846167,7.2615169309867,-3.52339371578857));
#30637=CARTESIAN_POINT('Ctrl Pts',(-16.3479082547577,6.51370272165337,3.52339371578857));
#30638=CARTESIAN_POINT('Ctrl Pts',(-16.6130070797081,5.74747912119454,10.5701811473657));
#30639=CARTESIAN_POINT('Ctrl Pts',(-16.3646266973296,8.18213889106893,-10.5701811473657));
#30640=CARTESIAN_POINT('Ctrl Pts',(-16.7420154026786,7.42737444544043,-3.52339371578858));
#30641=CARTESIAN_POINT('Ctrl Pts',(-17.0670469793702,6.64649736821331,3.52339371578859));
#30642=CARTESIAN_POINT('Ctrl Pts',(-17.3367301609262,5.8468958518967,10.5701811473657));
#30643=CARTESIAN_POINT('Ctrl Pts',(-17.3771604885591,8.26285160192196,-10.5701811473657));
#30644=CARTESIAN_POINT('Ctrl Pts',(-17.7583858480757,7.46133495538845,-3.52339371578858));
#30645=CARTESIAN_POINT('Ctrl Pts',(-18.0836843042383,6.63362228641827,3.52339371578858));
#30646=CARTESIAN_POINT('Ctrl Pts',(-18.3507193026914,5.78718621735566,10.5701811473657));
#30647=CARTESIAN_POINT('Ctrl Pts',(-18.2493498864903,8.18298767653274,-10.5701811473657));
#30648=CARTESIAN_POINT('Ctrl Pts',(-18.6267584091773,7.34130729564938,-3.52339371578858));
#30649=CARTESIAN_POINT('Ctrl Pts',(-18.9458430530205,6.47348072277112,3.52339371578858));
#30650=CARTESIAN_POINT('Ctrl Pts',(-19.2035582177667,5.58779118889344,10.5701811473657));
#30651=CARTESIAN_POINT('Ctrl Pts',(-15.5239408288993,7.92059131757517,-10.5701811473657));
#30652=CARTESIAN_POINT('Ctrl Pts',(-15.8892473389622,7.2046098435602,-3.52339371578858));
#30653=CARTESIAN_POINT('Ctrl Pts',(-16.2049399509463,6.46331998146983,3.52339371578858));
#30654=CARTESIAN_POINT('Ctrl Pts',(-16.4680054423355,5.7037971940124,10.5701811473657));
#30655=CARTESIAN_POINT('Origin',(1078.88931916181,-445.504381322801,-6.00190077291764));
#30656=CARTESIAN_POINT('Origin',(1110.51158560098,-359.500118244419,6.00190077332084));
#30657=CARTESIAN_POINT('Ctrl Pts',(-18.8787605074989,6.60245424154421,-10.5701811473657));
#30658=CARTESIAN_POINT('Ctrl Pts',(-19.1832730647213,5.73174474034773,-3.52339371578858));
#30659=CARTESIAN_POINT('Ctrl Pts',(-19.427450706283,4.83994031978785,3.52339371578858));
#30660=CARTESIAN_POINT('Ctrl Pts',(-19.6089628056837,3.93555307377479,10.5701811473657));
#30661=CARTESIAN_POINT('Ctrl Pts',(-18.4448707027188,6.10927224303739,-10.5701811473657));
#30662=CARTESIAN_POINT('Ctrl Pts',(-18.7266254214233,5.25854342785787,-3.52339371578856));
#30663=CARTESIAN_POINT('Ctrl Pts',(-18.949471334084,4.38838616553552,3.52339371578856));
#30664=CARTESIAN_POINT('Ctrl Pts',(-19.1111988723671,3.50692746437597,10.5701811473657));
#30665=CARTESIAN_POINT('Ctrl Pts',(-17.7292751069179,5.46743648480893,-10.5701811473657));
#30666=CARTESIAN_POINT('Ctrl Pts',(-17.981440982012,4.64974685659201,-3.52339371578859));
#30667=CARTESIAN_POINT('Ctrl Pts',(-18.1769404144146,3.81457658575116,3.52339371578859));
#30668=CARTESIAN_POINT('Ctrl Pts',(-18.3139187283814,2.96992227885496,10.5701811473657));
#30669=CARTESIAN_POINT('Ctrl Pts',(-17.0695785919953,5.06899457590414,-10.5701811473657));
#30670=CARTESIAN_POINT('Ctrl Pts',(-17.3033628853044,4.28171739274745,-3.52339371578857));
#30671=CARTESIAN_POINT('Ctrl Pts',(-17.4826059195935,3.47827239356548,3.52339371578857));
#30672=CARTESIAN_POINT('Ctrl Pts',(-17.6055728776112,2.66627511145608,10.5701811473657));
#30673=CARTESIAN_POINT('Ctrl Pts',(-16.7902899423754,4.94260967296501,-10.5701811473657));
#30674=CARTESIAN_POINT('Ctrl Pts',(-17.018249840101,4.16822615260271,-3.52339371578858));
#30675=CARTESIAN_POINT('Ctrl Pts',(-17.1925455301966,3.37804172155667,3.52339371578858));
#30676=CARTESIAN_POINT('Ctrl Pts',(-17.3115220795561,2.57961819216749,10.5701811473657));
#30677=CARTESIAN_POINT('Ctrl Pts',(-16.7254196142394,4.92139034178336,-10.5701811473657));
#30678=CARTESIAN_POINT('Ctrl Pts',(-16.9523954149176,4.14998383249092,-3.52339371578857));
#30679=CARTESIAN_POINT('Ctrl Pts',(-17.1259326414904,3.36288795769156,3.52339371578857));
#30680=CARTESIAN_POINT('Ctrl Pts',(-17.244345094947,2.56754871715414,10.5701811473657));
#30681=CARTESIAN_POINT('Ctrl Pts',(-16.7190706763204,4.91946962582534,-10.5701811473657));
#30682=CARTESIAN_POINT('Ctrl Pts',(-16.9459621050428,4.14836742961573,-3.52339371578858));
#30683=CARTESIAN_POINT('Ctrl Pts',(-17.1194210645505,3.36154821641249,3.52339371578858));
#30684=CARTESIAN_POINT('Ctrl Pts',(-17.2377919239465,2.56652201742732,10.5701811473657));
#30685=CARTESIAN_POINT('Origin',(1137.05035178694,-263.813557134597,6.00000003104242));
#30686=CARTESIAN_POINT('Origin',(1112.84725512312,-352.212461496002,-6.00000002249655));
#30687=CARTESIAN_POINT('Ctrl Pts',(-18.3844122993175,7.87485773895015,-8.00000002680495));
#30688=CARTESIAN_POINT('Ctrl Pts',(-18.4531333976134,7.71442347504143,-6.66666668453663));
#30689=CARTESIAN_POINT('Ctrl Pts',(-18.5197542958142,7.55308960393422,-5.33333334226832));
#30690=CARTESIAN_POINT('Ctrl Pts',(-18.5842521656445,7.39091140819173,-4.));
#30691=CARTESIAN_POINT('Ctrl Pts',(-18.6077644958072,7.35342624084014,-8.00000002680495));
#30692=CARTESIAN_POINT('Ctrl Pts',(-18.6719352556694,7.19104283587995,-6.66666668453663));
#30693=CARTESIAN_POINT('Ctrl Pts',(-18.7339802713311,7.02781946759157,-5.33333334226832));
#30694=CARTESIAN_POINT('Ctrl Pts',(-18.7938783394501,6.86381191269434,-4.));
#30695=CARTESIAN_POINT('Ctrl Pts',(-18.8089193180918,6.82248716352129,-8.00000002680495));
#30696=CARTESIAN_POINT('Ctrl Pts',(-18.8684567600673,6.65834835144207,-6.66666668453664));
#30697=CARTESIAN_POINT('Ctrl Pts',(-18.9258454793725,6.49343022987756,-5.33333334226832));
#30698=CARTESIAN_POINT('Ctrl Pts',(-18.9810658661255,6.32778915551912,-4.));
#30699=CARTESIAN_POINT('Ctrl Pts',(-18.9871493773879,6.28396041686769,-8.00000002680495));
#30700=CARTESIAN_POINT('Ctrl Pts',(-19.041987277425,6.11826627965563,-6.66666668453663));
#30701=CARTESIAN_POINT('Ctrl Pts',(-19.0946561219624,5.95185427630669,-5.33333334226832));
#30702=CARTESIAN_POINT('Ctrl Pts',(-19.1451378635268,5.78478142945371,-4.));
#30703=CARTESIAN_POINT('Ctrl Pts',(-18.9455935099938,6.40815781282578,4.));
#30704=CARTESIAN_POINT('Ctrl Pts',(-19.0015152367791,6.24282631897104,5.33333334226731));
#30705=CARTESIAN_POINT('Ctrl Pts',(-19.0552726553178,6.07676277090728,6.66666668453462));
#30706=CARTESIAN_POINT('Ctrl Pts',(-19.1068473451265,5.91002407186586,8.00000002680193));
#30707=CARTESIAN_POINT('Ctrl Pts',(-19.1273461422817,5.87080970260818,4.));
#30708=CARTESIAN_POINT('Ctrl Pts',(-19.1785786299635,5.70389209169293,5.33333334226731));
#30709=CARTESIAN_POINT('Ctrl Pts',(-19.2276260236414,5.53630389074424,6.66666668453462));
#30710=CARTESIAN_POINT('Ctrl Pts',(-19.2744715615271,5.36810236813544,8.00000002680193));
#30711=CARTESIAN_POINT('Ctrl Pts',(-19.2862238713926,5.32572490778712,4.));
#30712=CARTESIAN_POINT('Ctrl Pts',(-19.332699596505,5.15742082701961,5.33333334226731));
#30713=CARTESIAN_POINT('Ctrl Pts',(-19.3769720788243,4.98850842595595,6.66666668453462));
#30714=CARTESIAN_POINT('Ctrl Pts',(-19.4190261906145,4.81904542613221,8.00000002680193));
#30715=CARTESIAN_POINT('Ctrl Pts',(-19.4216521852328,4.77487449006159,4.));
#30716=CARTESIAN_POINT('Ctrl Pts',(-19.4633208261226,4.60538860052122,5.33333334226731));
#30717=CARTESIAN_POINT('Ctrl Pts',(-19.5027707748587,4.43535723991918,6.66666668453462));
#30718=CARTESIAN_POINT('Ctrl Pts',(-19.5399885135466,4.264838671095,8.00000002680193));
#30719=CARTESIAN_POINT('Ctrl Pts',(-11.8787308647727,12.7524216806657,-10.5701811473657));
#30720=CARTESIAN_POINT('Ctrl Pts',(-12.4668867829649,12.2045613578439,-3.52339371578857));
#30721=CARTESIAN_POINT('Ctrl Pts',(-13.017076865761,11.6159499769718,3.52339371578858));
#30722=CARTESIAN_POINT('Ctrl Pts',(-13.5240496594282,10.9922057153483,10.5701811473657));
#30723=CARTESIAN_POINT('Ctrl Pts',(-11.8855676953475,12.7596503467182,-10.5701811473657));
#30724=CARTESIAN_POINT('Ctrl Pts',(-12.4741202082508,12.2114679311921,-3.52339371578859));
#30725=CARTESIAN_POINT('Ctrl Pts',(-13.0244969705674,11.6225403214579,3.52339371578859));
#30726=CARTESIAN_POINT('Ctrl Pts',(-13.5318181449482,10.9984223461024,10.5701811473657));
#30727=CARTESIAN_POINT('Ctrl Pts',(-11.9863857707236,12.8589190332253,-10.5701811473657));
#30728=CARTESIAN_POINT('Ctrl Pts',(-12.5794765862914,12.3060905992793,-3.52339371578856));
#30729=CARTESIAN_POINT('Ctrl Pts',(-13.134188756619,11.7121827924541,3.52339371578857));
#30730=CARTESIAN_POINT('Ctrl Pts',(-13.6453640718523,11.082837267336,10.5701811473657));
#30731=CARTESIAN_POINT('Ctrl Pts',(-12.5792608243633,13.2857117717956,-10.5701811473657));
#30732=CARTESIAN_POINT('Ctrl Pts',(-13.1920348426224,12.7055397408969,-3.52339371578859));
#30733=CARTESIAN_POINT('Ctrl Pts',(-13.764538166676,12.0829230390914,3.52339371578859));
#30734=CARTESIAN_POINT('Ctrl Pts',(-14.2914372817995,11.4237804859417,10.5701811473657));
#30735=CARTESIAN_POINT('Ctrl Pts',(-13.5031269323654,13.7078792049972,-10.5701811473657));
#30736=CARTESIAN_POINT('Ctrl Pts',(-14.1354964096488,13.0850867185779,-3.52339371578856));
#30737=CARTESIAN_POINT('Ctrl Pts',(-14.7242713589907,12.4185498968891,3.52339371578857));
#30738=CARTESIAN_POINT('Ctrl Pts',(-15.264700349594,11.7144915590679,10.5701811473657));
#30739=CARTESIAN_POINT('Ctrl Pts',(-14.3500311789428,13.9311379708684,-10.5701811473657));
#30740=CARTESIAN_POINT('Ctrl Pts',(-14.9925508077551,13.2692985198616,-3.52339371578857));
#30741=CARTESIAN_POINT('Ctrl Pts',(-15.5892064466918,12.5629417452578,3.52339371578858));
#30742=CARTESIAN_POINT('Ctrl Pts',(-16.1343031376281,11.818809680468,10.5701811473657));
#30743=CARTESIAN_POINT('Ctrl Pts',(-11.8787308647727,12.7524216806657,-10.5701811473657));
#30744=CARTESIAN_POINT('Ctrl Pts',(-12.4668867829649,12.2045613578439,-3.52339371578857));
#30745=CARTESIAN_POINT('Ctrl Pts',(-13.017076865761,11.6159499769718,3.52339371578858));
#30746=CARTESIAN_POINT('Ctrl Pts',(-13.5240496594282,10.9922057153483,10.5701811473657));
#30747=CARTESIAN_POINT('Origin',(861.452859530637,-787.639059256886,-6.00190077370807));
#30748=CARTESIAN_POINT('Origin',(920.583260312982,-717.636939968109,6.00190077196441));
#30749=CARTESIAN_POINT('Ctrl Pts',(-15.482059589238,12.6611938961255,-10.5701811473657));
#30750=CARTESIAN_POINT('Ctrl Pts',(-16.0660079802072,11.9471440316185,-3.52339371578857));
#30751=CARTESIAN_POINT('Ctrl Pts',(-16.6004749835089,11.1926356705744,3.52339371578858));
#30752=CARTESIAN_POINT('Ctrl Pts',(-17.0803592190431,10.4048704436167,10.5701811473657));
#30753=CARTESIAN_POINT('Ctrl Pts',(-15.243014719731,12.0493553593938,-10.5701811473657));
#30754=CARTESIAN_POINT('Ctrl Pts',(-15.7987439407825,11.346297558895,-3.52339371578858));
#30755=CARTESIAN_POINT('Ctrl Pts',(-16.3057619116501,10.6048349916867,3.5233937157886));
#30756=CARTESIAN_POINT('Ctrl Pts',(-16.7592127169954,9.83184883068219,10.5701811473657));
#30757=CARTESIAN_POINT('Ctrl Pts',(-14.7900894187725,11.2014790072182,-10.5701811473657));
#30758=CARTESIAN_POINT('Ctrl Pts',(-15.3067141545056,10.5193479063346,-3.52339371578855));
#30759=CARTESIAN_POINT('Ctrl Pts',(-15.7760686536943,9.80141015840479,3.52339371578856));
#30760=CARTESIAN_POINT('Ctrl Pts',(-16.1936749515119,9.0545440817974,10.5701811473657));
#30761=CARTESIAN_POINT('Ctrl Pts',(-14.3064567126843,10.601436531037,-10.5701811473657));
#30762=CARTESIAN_POINT('Ctrl Pts',(-14.7954067429393,9.94159690905795,-3.52339371578859));
#30763=CARTESIAN_POINT('Ctrl Pts',(-15.2386344956153,9.24791058685751,3.5233937157886));
#30764=CARTESIAN_POINT('Ctrl Pts',(-15.6319050654347,8.52693990941373,10.5701811473657));
#30765=CARTESIAN_POINT('Ctrl Pts',(-14.087237713241,10.3871512277472,-10.5701811473657));
#30766=CARTESIAN_POINT('Ctrl Pts',(-14.566304709585,9.7374356249061,-3.52339371578856));
#30767=CARTESIAN_POINT('Ctrl Pts',(-15.000348095257,9.05451802789469,3.52339371578857));
#30768=CARTESIAN_POINT('Ctrl Pts',(-15.3852264106871,8.34493770554008,10.5701811473657));
#30769=CARTESIAN_POINT('Ctrl Pts',(-14.0335387609796,10.345024601817,-10.5701811473657));
#30770=CARTESIAN_POINT('Ctrl Pts',(-14.5106628108441,9.69776989328862,-3.52339371578858));
#30771=CARTESIAN_POINT('Ctrl Pts',(-14.9429371059958,9.01749493499381,3.52339371578859));
#30772=CARTESIAN_POINT('Ctrl Pts',(-15.3262304557589,8.31061996394269,10.5701811473657));
#30773=CARTESIAN_POINT('Ctrl Pts',(-14.0282296344253,10.3410482545556,-10.5701811473657));
#30774=CARTESIAN_POINT('Ctrl Pts',(-14.5051703193816,9.69405064987659,-3.52339371578857));
#30775=CARTESIAN_POINT('Ctrl Pts',(-14.9372764437114,9.01400889952889,3.52339371578858));
#30776=CARTESIAN_POINT('Ctrl Pts',(-15.3204236413265,8.30741386530726,10.5701811473657));
#30777=CARTESIAN_POINT('Origin',(978.241467157012,-636.804482366658,6.00190077771329));
#30778=CARTESIAN_POINT('Origin',(925.27415056307,-711.578571311033,-6.00190076986674));
#30779=CARTESIAN_POINT('Ctrl Pts',(-14.5823366026094,13.687785036601,-8.00000002680495));
#30780=CARTESIAN_POINT('Ctrl Pts',(-14.7017850615068,13.5605301425734,-6.66666668453663));
#30781=CARTESIAN_POINT('Ctrl Pts',(-14.8195676616555,13.4317115835623,-5.33333334226832));
#30782=CARTESIAN_POINT('Ctrl Pts',(-14.9356440437436,13.3013735004542,-4.));
#30783=CARTESIAN_POINT('Ctrl Pts',(-14.9705590892051,13.2741906558372,-8.00000002680495));
#30784=CARTESIAN_POINT('Ctrl Pts',(-15.0863982741561,13.1435478609434,-6.66666668453664));
#30785=CARTESIAN_POINT('Ctrl Pts',(-15.200527197346,13.0113887113723,-5.33333334226832));
#30786=CARTESIAN_POINT('Ctrl Pts',(-15.3129068573893,12.8777583681252,-4.));
#30787=CARTESIAN_POINT('Ctrl Pts',(-15.3411746506633,12.8440701239422,-8.00000002680495));
#30788=CARTESIAN_POINT('Ctrl Pts',(-15.4532603255808,12.7101930978845,-6.66666668453663));
#30789=CARTESIAN_POINT('Ctrl Pts',(-15.5635934012027,12.5748488540185,-5.33333334226832));
#30790=CARTESIAN_POINT('Ctrl Pts',(-15.6721361751441,12.4380836433366,-4.));
#30791=CARTESIAN_POINT('Ctrl Pts',(-15.6928431172612,12.3989787844414,-8.00000002680495));
#30792=CARTESIAN_POINT('Ctrl Pts',(-15.801044619823,12.2620328928261,-6.66666668453663));
#30793=CARTESIAN_POINT('Ctrl Pts',(-15.9074534016166,12.1236705670264,-5.33333334226832));
#30794=CARTESIAN_POINT('Ctrl Pts',(-16.0120330006756,11.9839392181901,-4.));
#30795=CARTESIAN_POINT('Ctrl Pts',(-15.6113153641544,12.5014732172219,4.));
#30796=CARTESIAN_POINT('Ctrl Pts',(-15.7204112993806,12.3652387894732,5.33333334226731));
#30797=CARTESIAN_POINT('Ctrl Pts',(-15.8277238274038,12.2275762187696,6.66666668453462));
#30798=CARTESIAN_POINT('Ctrl Pts',(-15.9332161765804,12.0885326764813,8.00000002680193));
#30799=CARTESIAN_POINT('Ctrl Pts',(-15.9658908491962,12.0586942246021,4.));
#30800=CARTESIAN_POINT('Ctrl Pts',(-16.0711228250241,11.9193655201257,5.33333334226731));
#30801=CARTESIAN_POINT('Ctrl Pts',(-16.1745308394401,11.7786593209788,6.66666668453462));
#30802=CARTESIAN_POINT('Ctrl Pts',(-16.2760795545783,11.6366237089603,8.00000002680193));
#30803=CARTESIAN_POINT('Ctrl Pts',(-16.3016170584982,11.6008214488879,4.));
#30804=CARTESIAN_POINT('Ctrl Pts',(-16.4028533402584,11.4585629803066,5.33333334226731));
#30805=CARTESIAN_POINT('Ctrl Pts',(-16.502227308819,11.3149793242161,6.66666668453462));
#30806=CARTESIAN_POINT('Ctrl Pts',(-16.5997050068301,11.1701195471274,8.00000002680193));
#30807=CARTESIAN_POINT('Ctrl Pts',(-16.6172799844809,11.1295105875044,4.));
#30808=CARTESIAN_POINT('Ctrl Pts',(-16.7144032870754,10.9844974623052,5.33333334226731));
#30809=CARTESIAN_POINT('Ctrl Pts',(-16.8096282631161,10.8382129245662,6.66666668453462));
#30810=CARTESIAN_POINT('Ctrl Pts',(-16.9029222828724,10.6907071000555,8.00000002680193));
#30811=CARTESIAN_POINT('Ctrl Pts',(-6.80077064695807,16.0461217833684,-10.5701811473657));
#30812=CARTESIAN_POINT('Ctrl Pts',(-7.54083568928884,15.7324626522293,-3.52339371578857));
#30813=CARTESIAN_POINT('Ctrl Pts',(-8.25916219897089,15.3675249720875,3.52339371578858));
#30814=CARTESIAN_POINT('Ctrl Pts',(-8.94889389387818,14.9547919997346,10.5701811473657));
#30815=CARTESIAN_POINT('Ctrl Pts',(-6.80340542685265,16.0522091553162,-10.5701811473657));
#30816=CARTESIAN_POINT('Ctrl Pts',(-7.54376312530191,15.7384313756406,-3.52339371578856));
#30817=CARTESIAN_POINT('Ctrl Pts',(-8.26233788774701,15.3733486508931,3.52339371578857));
#30818=CARTESIAN_POINT('Ctrl Pts',(-8.95234307759614,14.9604578001197,10.5701811473657));
#30819=CARTESIAN_POINT('Ctrl Pts',(-6.83191060264015,16.1142229628818,-10.5701811473657));
#30820=CARTESIAN_POINT('Ctrl Pts',(-7.57511310971921,15.7991268108383,-3.52339371578858));
#30821=CARTESIAN_POINT('Ctrl Pts',(-8.29648793938119,15.4325364319901,3.52339371578859));
#30822=CARTESIAN_POINT('Ctrl Pts',(-8.98912891724121,15.0179474459445,10.5701811473657));
#30823=CARTESIAN_POINT('Ctrl Pts',(-6.98943179288406,16.3772101395067,-10.5701811473657));
#30824=CARTESIAN_POINT('Ctrl Pts',(-7.74477657805422,16.0548520865033,-3.52339371578856));
#30825=CARTESIAN_POINT('Ctrl Pts',(-8.47775084446518,15.6801517612301,3.52339371578857));
#30826=CARTESIAN_POINT('Ctrl Pts',(-9.18141647930976,15.2566955850341,10.5701811473657));
#30827=CARTESIAN_POINT('Ctrl Pts',(-7.46076357859445,16.9869629346774,-10.5701811473657));
#30828=CARTESIAN_POINT('Ctrl Pts',(-8.24421702181037,16.6428631545598,-3.52339371578858));
#30829=CARTESIAN_POINT('Ctrl Pts',(-9.00383528249654,16.2444807757546,3.52339371578859));
#30830=CARTESIAN_POINT('Ctrl Pts',(-9.73234227367099,15.7956138465051,10.5701811473657));
#30831=CARTESIAN_POINT('Ctrl Pts',(-8.18028559447402,17.6243975759645,-10.5701811473657));
#30832=CARTESIAN_POINT('Ctrl Pts',(-8.99317441419756,17.2471218084664,-3.52339371578856));
#30833=CARTESIAN_POINT('Ctrl Pts',(-9.77981895378716,16.8135040854808,3.52339371578857));
#30834=CARTESIAN_POINT('Ctrl Pts',(-10.5329043010252,16.3277184354786,10.5701811473657));
#30835=CARTESIAN_POINT('Ctrl Pts',(-8.71988860141417,17.9989872709252,-10.5701811473657));
#30836=CARTESIAN_POINT('Ctrl Pts',(-9.55002197921108,17.5968162782051,-3.52339371578857));
#30837=CARTESIAN_POINT('Ctrl Pts',(-10.3522831255593,17.137126276613,3.52339371578858));
#30838=CARTESIAN_POINT('Ctrl Pts',(-11.1190146190996,16.6243049148002,10.5701811473657));
#30839=CARTESIAN_POINT('Ctrl Pts',(-6.80077064695807,16.0461217833684,-10.5701811473657));
#30840=CARTESIAN_POINT('Ctrl Pts',(-7.54083568928884,15.7324626522293,-3.52339371578857));
#30841=CARTESIAN_POINT('Ctrl Pts',(-8.25916219897089,15.3675249720875,3.52339371578858));
#30842=CARTESIAN_POINT('Ctrl Pts',(-8.94889389387818,14.9547919997346,10.5701811473657));
#30843=CARTESIAN_POINT('Origin',(540.112471297657,-1034.77284228394,-6.00190077359785));
#30844=CARTESIAN_POINT('Origin',(619.61900747461,-989.216155520019,6.00190077285814));
#30845=CARTESIAN_POINT('Ctrl Pts',(-10.2179937997566,17.1928067231421,-10.5701811473657));
#30846=CARTESIAN_POINT('Ctrl Pts',(-11.0109452310822,16.7215414469562,-3.52339371578858));
#30847=CARTESIAN_POINT('Ctrl Pts',(-11.771236988334,16.1953339887957,3.52339371578858));
#30848=CARTESIAN_POINT('Ctrl Pts',(-12.4916122395345,15.6192068930627,10.5701811473657));
#30849=CARTESIAN_POINT('Ctrl Pts',(-10.2026262038394,16.5361084032577,-10.5701811473657));
#30850=CARTESIAN_POINT('Ctrl Pts',(-10.9653007820263,16.0655207639422,-3.52339371578858));
#30851=CARTESIAN_POINT('Ctrl Pts',(-11.6953369617913,15.5421842200282,3.52339371578858));
#30852=CARTESIAN_POINT('Ctrl Pts',(-12.3858181753482,14.9709041379195,10.5701811473657));
#30853=CARTESIAN_POINT('Ctrl Pts',(-10.0670065005512,15.5844556949577,-10.5701811473657));
#30854=CARTESIAN_POINT('Ctrl Pts',(-10.7857775294983,15.1201581991623,-3.52339371578857));
#30855=CARTESIAN_POINT('Ctrl Pts',(-11.4723756631224,14.6060460787463,3.52339371578857));
#30856=CARTESIAN_POINT('Ctrl Pts',(-12.1202404623057,14.0470513036056,10.5701811473657));
#30857=CARTESIAN_POINT('Ctrl Pts',(-9.81776698398909,14.8551880626951,-10.5701811473657));
#30858=CARTESIAN_POINT('Ctrl Pts',(-10.5029081614891,14.402372398422,-3.52339371578859));
#30859=CARTESIAN_POINT('Ctrl Pts',(-11.1566607063151,13.9021132965599,3.52339371578859));
#30860=CARTESIAN_POINT('Ctrl Pts',(-11.7728006532308,13.3591289277869,10.5701811473657));
#30861=CARTESIAN_POINT('Ctrl Pts',(-9.68505839432707,14.5788484285183,-10.5701811473657));
#30862=CARTESIAN_POINT('Ctrl Pts',(-10.3574499392681,14.1321660336653,-3.52339371578856));
#30863=CARTESIAN_POINT('Ctrl Pts',(-10.9988888810637,13.6388849853688,3.52339371578856));
#30864=CARTESIAN_POINT('Ctrl Pts',(-11.6032469575356,13.1037337291963,10.5701811473657));
#30865=CARTESIAN_POINT('Ctrl Pts',(-9.64900602019246,14.5208962185849,-10.5701811473657));
#30866=CARTESIAN_POINT('Ctrl Pts',(-10.3187301172292,14.0758617811302,-3.52339371578859));
#30867=CARTESIAN_POINT('Ctrl Pts',(-10.9576028212762,13.5844589390986,3.52339371578859));
#30868=CARTESIAN_POINT('Ctrl Pts',(-11.5595462325576,13.0513077914049,10.5701811473657));
#30869=CARTESIAN_POINT('Ctrl Pts',(-9.6453770639989,14.5153438461684,-10.5701811473657));
#30870=CARTESIAN_POINT('Ctrl Pts',(-10.3148409196886,14.070488292812,-3.52339371578858));
#30871=CARTESIAN_POINT('Ctrl Pts',(-10.9534758330391,13.5792470767591,3.52339371578858));
#30872=CARTESIAN_POINT('Ctrl Pts',(-11.5551861621905,13.0463089966602,10.5701811473657));
#30873=CARTESIAN_POINT('Origin',(701.455017736501,-932.974787184144,6.000000029911));
#30874=CARTESIAN_POINT('Origin',(626.092649606612,-985.134825974761,-6.00000001913359));
#30875=CARTESIAN_POINT('Ctrl Pts',(-9.02141589925906,17.8497634486454,-8.00000002680495));
#30876=CARTESIAN_POINT('Ctrl Pts',(-9.1771844717434,17.7710367428009,-6.66666668453663));
#30877=CARTESIAN_POINT('Ctrl Pts',(-9.33192245397615,17.6902709152619,-5.33333334226832));
#30878=CARTESIAN_POINT('Ctrl Pts',(-9.48557682353725,17.6074936411964,-4.));
#30879=CARTESIAN_POINT('Ctrl Pts',(-9.52768331452378,17.5938917715508,-8.00000002680495));
#30880=CARTESIAN_POINT('Ctrl Pts',(-9.68121900925411,17.5107470358699,-6.66666668453663));
#30881=CARTESIAN_POINT('Ctrl Pts',(-9.833666207472,17.4255924489156,-5.33333334226832));
#30882=CARTESIAN_POINT('Ctrl Pts',(-9.98497281389112,17.3384571088881,-4.));
#30883=CARTESIAN_POINT('Ctrl Pts',(-10.0230579087404,17.3164686691292,-8.00000002680495));
#30884=CARTESIAN_POINT('Ctrl Pts',(-10.1741726299965,17.2290009742501,-6.66666668453664));
#30885=CARTESIAN_POINT('Ctrl Pts',(-10.3241422646724,17.1395551213611,-5.33333334226831));
#30886=CARTESIAN_POINT('Ctrl Pts',(-10.4729155653442,17.0481616772035,-4.));
#30887=CARTESIAN_POINT('Ctrl Pts',(-10.5057483754947,17.0184973211735,-8.00000002680495));
#30888=CARTESIAN_POINT('Ctrl Pts',(-10.6542627824881,16.9268173707899,-6.66666668453663));
#30889=CARTESIAN_POINT('Ctrl Pts',(-10.8015770320273,16.8331932610413,-5.33333334226832));
#30890=CARTESIAN_POINT('Ctrl Pts',(-10.9476406455038,16.7376570731065,-4.));
#30891=CARTESIAN_POINT('Ctrl Pts',(-10.3940821869213,17.0869264495264,4.));
#30892=CARTESIAN_POINT('Ctrl Pts',(-10.5431937507156,16.9962209704763,5.33333334226731));
#30893=CARTESIAN_POINT('Ctrl Pts',(-10.6911179135796,16.9035635148428,6.66666668453462));
#30894=CARTESIAN_POINT('Ctrl Pts',(-10.8378039879122,16.8089858325717,8.00000002680193));
#30895=CARTESIAN_POINT('Ctrl Pts',(-10.8787134882441,16.7921222557363,4.));
#30896=CARTESIAN_POINT('Ctrl Pts',(-11.0252524228747,16.6971875557313,5.33333334226731));
#30897=CARTESIAN_POINT('Ctrl Pts',(-11.1705485253505,16.6003346026057,6.66666668453462));
#30898=CARTESIAN_POINT('Ctrl Pts',(-11.3145521439962,16.5015964922092,8.00000002680193));
#30899=CARTESIAN_POINT('Ctrl Pts',(-11.3507946421043,16.4766877133626,4.));
#30900=CARTESIAN_POINT('Ctrl Pts',(-11.4945808908437,16.3776333277898,5.33333334226731));
#30901=CARTESIAN_POINT('Ctrl Pts',(-11.6370703784336,16.2766967246661,6.66666668453462));
#30902=CARTESIAN_POINT('Ctrl Pts',(-11.7782144136678,16.1739123973319,8.00000002680193));
#30903=CARTESIAN_POINT('Ctrl Pts',(-11.8086185726672,16.1417634540114,4.));
#30904=CARTESIAN_POINT('Ctrl Pts',(-11.9494820332864,16.0387138162183,5.33333334226731));
#30905=CARTESIAN_POINT('Ctrl Pts',(-12.0889964991502,15.9338201755236,6.66666668453462));
#30906=CARTESIAN_POINT('Ctrl Pts',(-12.2271141643192,15.8271184747163,8.00000002680193));
#30907=CARTESIAN_POINT('Ctrl Pts',(-0.902537120435117,17.4044227834609,
-10.5701811473657));
#30908=CARTESIAN_POINT('Ctrl Pts',(-1.70524852060254,17.3627967643357,-3.52339371578858));
#30909=CARTESIAN_POINT('Ctrl Pts',(-2.5050706787327,17.2655496550558,3.52339371578857));
#30910=CARTESIAN_POINT('Ctrl Pts',(-3.29436945311861,17.1136096597291,10.5701811473657));
#30911=CARTESIAN_POINT('Ctrl Pts',(-0.903127939532374,17.4143548929044,
-10.5701811473657));
#30912=CARTESIAN_POINT('Ctrl Pts',(-1.7063501860739,17.3727370626192,-3.52339371578857));
#30913=CARTESIAN_POINT('Ctrl Pts',(-2.50651861700781,17.2753677032595,3.52339371578856));
#30914=CARTESIAN_POINT('Ctrl Pts',(-3.29632448505991,17.1233653614113,10.5701811473657));
#30915=CARTESIAN_POINT('Ctrl Pts',(-0.916537850406108,17.5552227079068,
-10.5701811473657));
#30916=CARTESIAN_POINT('Ctrl Pts',(-1.72622304155971,17.5129629857501,-3.52339371578858));
#30917=CARTESIAN_POINT('Ctrl Pts',(-2.5329165341938,17.4145668679409,3.52339371578857));
#30918=CARTESIAN_POINT('Ctrl Pts',(-3.32903504964555,17.261037384632,10.5701811473657));
#30919=CARTESIAN_POINT('Ctrl Pts',(-1.0963614992881,18.2632687859986,-10.5701811473657));
#30920=CARTESIAN_POINT('Ctrl Pts',(-1.93870102381158,18.2127147721504,-3.52339371578857));
#30921=CARTESIAN_POINT('Ctrl Pts',(-2.7774786640394,18.1037632822201,3.52339371578856));
#30922=CARTESIAN_POINT('Ctrl Pts',(-3.60479546944582,17.9375150149126,10.5701811473657));
#30923=CARTESIAN_POINT('Ctrl Pts',(-1.53274044321679,19.1804873760836,-10.5701811473657));
#30924=CARTESIAN_POINT('Ctrl Pts',(-2.41748686096405,19.1098799173875,-3.52339371578859));
#30925=CARTESIAN_POINT('Ctrl Pts',(-3.29695624953646,18.9777403313294,3.52339371578858));
#30926=CARTESIAN_POINT('Ctrl Pts',(-4.16350885073652,18.7857814130851,10.5701811473657));
#30927=CARTESIAN_POINT('Ctrl Pts',(-2.03799876670532,19.8958930693474,-10.5701811473657));
#30928=CARTESIAN_POINT('Ctrl Pts',(-2.95561955666072,19.8018982920477,-3.52339371578858));
#30929=CARTESIAN_POINT('Ctrl Pts',(-3.86672167605728,19.6443204619612,3.52339371578857));
#30930=CARTESIAN_POINT('Ctrl Pts',(-4.7626088383289,19.4246636277973,10.5701811473657));
#30931=CARTESIAN_POINT('Ctrl Pts',(-0.902537120435117,17.4044227834609,
-10.5701811473657));
#30932=CARTESIAN_POINT('Ctrl Pts',(-1.70524852060254,17.3627967643357,-3.52339371578858));
#30933=CARTESIAN_POINT('Ctrl Pts',(-2.5050706787327,17.2655496550558,3.52339371578857));
#30934=CARTESIAN_POINT('Ctrl Pts',(-3.29436945311861,17.1136096597291,10.5701811473657));
#30935=CARTESIAN_POINT('Origin',(153.626547848438,-1157.09774893006,-6.0019007738202));
#30936=CARTESIAN_POINT('Origin',(243.9195577298,-1141.48130344627,6.00190077262389));
#30937=CARTESIAN_POINT('Ctrl Pts',(-3.72148715324784,19.6507133122285,-10.5701811473657));
#30938=CARTESIAN_POINT('Ctrl Pts',(-4.62779997921166,19.4790741719562,-3.52339371578858));
#30939=CARTESIAN_POINT('Ctrl Pts',(-5.52221408340464,19.244636002305,3.52339371578858));
#30940=CARTESIAN_POINT('Ctrl Pts',(-6.39619246301094,18.9496364684737,10.5701811473657));
#30941=CARTESIAN_POINT('Ctrl Pts',(-3.93165039025384,19.0283627195925,-10.5701811473657));
#30942=CARTESIAN_POINT('Ctrl Pts',(-4.809280515283,18.847005056037,-3.52339371578858));
#30943=CARTESIAN_POINT('Ctrl Pts',(-5.67428176607203,18.6049166463695,3.52339371578858));
#30944=CARTESIAN_POINT('Ctrl Pts',(-6.5185111628046,18.3042474524344,10.5701811473657));
#30945=CARTESIAN_POINT('Ctrl Pts',(-4.12969891987873,18.0877210849009,-10.5701811473657));
#30946=CARTESIAN_POINT('Ctrl Pts',(-4.96392184787269,17.8972583245915,-3.52339371578858));
#30947=CARTESIAN_POINT('Ctrl Pts',(-5.78495026151908,17.6489806267713,3.52339371578858));
#30948=CARTESIAN_POINT('Ctrl Pts',(-6.58493150569053,17.345280172986,10.5701811473657));
#30949=CARTESIAN_POINT('Ctrl Pts',(-4.14491130701936,17.3171860509472,-10.5701811473657));
#30950=CARTESIAN_POINT('Ctrl Pts',(-4.94360549410748,17.1260105963803,-3.52339371578858));
#30951=CARTESIAN_POINT('Ctrl Pts',(-5.72903079998517,16.8795171054834,3.52339371578858));
#30952=CARTESIAN_POINT('Ctrl Pts',(-6.49372455310468,16.5800109738981,10.5701811473657));
#30953=CARTESIAN_POINT('Ctrl Pts',(-4.11471950693847,17.0121225239124,-10.5701811473657));
#30954=CARTESIAN_POINT('Ctrl Pts',(-4.89933525670704,16.8223498262057,-3.52339371578858));
#30955=CARTESIAN_POINT('Ctrl Pts',(-5.6708029003471,16.5782020953568,3.52339371578858));
#30956=CARTESIAN_POINT('Ctrl Pts',(-6.42174623445712,16.2820270448622,10.5701811473657));
#30957=CARTESIAN_POINT('Ctrl Pts',(-4.10066074919594,16.9453334457781,-10.5701811473657));
#30958=CARTESIAN_POINT('Ctrl Pts',(-4.88220628322697,16.7561970005635,-3.52339371578857));
#30959=CARTESIAN_POINT('Ctrl Pts',(-5.65061991930365,16.5129367098782,3.52339371578857));
#30960=CARTESIAN_POINT('Ctrl Pts',(-6.39861013296397,16.2178152824273,10.5701811473657));
#30961=CARTESIAN_POINT('Ctrl Pts',(-4.09914966904954,16.9388747462736,-10.5701811473657));
#30962=CARTESIAN_POINT('Ctrl Pts',(-4.88038947424221,16.7498173893433,-3.52339371578858));
#30963=CARTESIAN_POINT('Ctrl Pts',(-5.64852438081578,16.5066276481894,3.52339371578858));
#30964=CARTESIAN_POINT('Ctrl Pts',(-6.39622269550912,16.2116267200016,10.5701811473657));
#30965=CARTESIAN_POINT('Origin',(340.055933547788,-1116.62126860195,6.00000003014708));
#30966=CARTESIAN_POINT('Origin',(251.398688376256,-1139.86022419539,-6.00000002075048));
#30967=CARTESIAN_POINT('Ctrl Pts',(-2.37237929653944,19.8587969543311,-8.00000002680495));
#30968=CARTESIAN_POINT('Ctrl Pts',(-2.54567999386982,19.838094039277,-6.66666668453663));
#30969=CARTESIAN_POINT('Ctrl Pts',(-2.71870967383992,19.8151224939882,-5.33333334226832));
#30970=CARTESIAN_POINT('Ctrl Pts',(-2.89140904620798,19.7898901898799,-4.));
#30971=CARTESIAN_POINT('Ctrl Pts',(-2.93562831848091,19.7915098814272,-8.00000002680495));
#30972=CARTESIAN_POINT('Ctrl Pts',(-3.10834185226059,19.765891687168,-6.66666668453663));
#30973=CARTESIAN_POINT('Ctrl Pts',(-3.2807199435204,19.738012562765,-5.33333334226832));
#30974=CARTESIAN_POINT('Ctrl Pts',(-3.45270368653352,19.7078820339451,-4.));
#30975=CARTESIAN_POINT('Ctrl Pts',(-3.49601245844321,19.70024552896,-8.00000002680495));
#30976=CARTESIAN_POINT('Ctrl Pts',(-3.66792956043858,19.6697370601475,-6.66666668453664));
#30977=CARTESIAN_POINT('Ctrl Pts',(-3.83944720291044,19.6369780881742,-5.33333334226832));
#30978=CARTESIAN_POINT('Ctrl Pts',(-4.01050677459149,19.6019798087299,-4.));
#30979=CARTESIAN_POINT('Ctrl Pts',(-4.05150533131066,19.5853339147016,-8.00000002680495));
#30980=CARTESIAN_POINT('Ctrl Pts',(-4.22241961341303,19.549977860618,-6.66666668453663));
#30981=CARTESIAN_POINT('Ctrl Pts',(-4.39287105807657,19.5123844163008,-5.33333334226832));
#30982=CARTESIAN_POINT('Ctrl Pts',(-4.56280125851603,19.4725664634964,-4.));
#30983=CARTESIAN_POINT('Ctrl Pts',(-3.92316929763007,19.6114441758411,4.));
#30984=CARTESIAN_POINT('Ctrl Pts',(-4.09431143474655,19.5772080649333,5.33333334226731));
#30985=CARTESIAN_POINT('Ctrl Pts',(-4.26500539528168,19.5407315809978,6.66666668453462));
#30986=CARTESIAN_POINT('Ctrl Pts',(-4.43519268934985,19.5020272230437,8.00000002680193));
#30987=CARTESIAN_POINT('Ctrl Pts',(-4.47940272789802,19.5001725174983,4.));
#30988=CARTESIAN_POINT('Ctrl Pts',(-4.64957386313053,19.4610823478722,5.33333334226731));
#30989=CARTESIAN_POINT('Ctrl Pts',(-4.81923319936555,19.4197645363123,6.66666668453462));
#30990=CARTESIAN_POINT('Ctrl Pts',(-4.98832275984285,19.3762332008709,8.00000002680193));
#30991=CARTESIAN_POINT('Ctrl Pts',(-5.03089887198512,19.3652222695934,4.));
#30992=CARTESIAN_POINT('Ctrl Pts',(-5.19989234404657,19.3213193878163,5.33333334226731));
#30993=CARTESIAN_POINT('Ctrl Pts',(-5.3683110155416,19.2752042816616,6.66666668453462));
#30994=CARTESIAN_POINT('Ctrl Pts',(-5.53609733428556,19.2268927108936,8.00000002680193));
#30995=CARTESIAN_POINT('Ctrl Pts',(-5.57566348434081,19.207081420908,4.));
#30996=CARTESIAN_POINT('Ctrl Pts',(-5.74327689071064,19.1584245776895,5.33333334226731));
#30997=CARTESIAN_POINT('Ctrl Pts',(-5.91025334280012,19.107573555172,6.66666668453462));
#30998=CARTESIAN_POINT('Ctrl Pts',(-6.07653562456277,19.054545777935,8.00000002680193));
#30999=CARTESIAN_POINT('Ctrl Pts',(5.10455570284159,16.6634935339443,-10.5701811473657));
#31000=CARTESIAN_POINT('Ctrl Pts',(4.33601678645625,16.8989213390741,-3.52339371578858));
#31001=CARTESIAN_POINT('Ctrl Pts',(3.55116933626636,17.0810942372497,3.52339371578858));
#31002=CARTESIAN_POINT('Ctrl Pts',(2.75750456340205,17.2082734247813,10.5701811473657));
#31003=CARTESIAN_POINT('Ctrl Pts',(5.10739749599088,16.6730287359292,-10.5701811473657));
#31004=CARTESIAN_POINT('Ctrl Pts',(4.33838134178569,16.9086389558016,-3.52339371578858));
#31005=CARTESIAN_POINT('Ctrl Pts',(3.55316668960757,17.0908154087533,3.52339371578858));
#31006=CARTESIAN_POINT('Ctrl Pts',(2.75900408080085,17.218109445967,10.5701811473657));
#31007=CARTESIAN_POINT('Ctrl Pts',(5.14297547152441,16.8099873002576,-10.5701811473657));
#31008=CARTESIAN_POINT('Ctrl Pts',(4.36766659600884,17.0472047963176,-3.52339371578858));
#31009=CARTESIAN_POINT('Ctrl Pts',(3.57596927094007,17.2306480542269,3.52339371578858));
#31010=CARTESIAN_POINT('Ctrl Pts',(2.77535240081299,17.3586661004475,10.5701811473657));
#31011=CARTESIAN_POINT('Ctrl Pts',(5.2161622749215,17.536836351783,-10.5701811473657));
#31012=CARTESIAN_POINT('Ctrl Pts',(4.40733153621265,17.7774282041587,-3.52339371578858));
#31013=CARTESIAN_POINT('Ctrl Pts',(3.58187484240095,17.9619260440227,3.52339371578858));
#31014=CARTESIAN_POINT('Ctrl Pts',(2.74759107678742,18.0886627859078,10.5701811473657));
#31015=CARTESIAN_POINT('Ctrl Pts',(5.11980806768289,18.5479914974658,-10.5701811473657));
#31016=CARTESIAN_POINT('Ctrl Pts',(4.26426917104784,18.7842432821225,-3.52339371578857));
#31017=CARTESIAN_POINT('Ctrl Pts',(3.39264383327069,18.9608689271939,3.52339371578857));
#31018=CARTESIAN_POINT('Ctrl Pts',(2.51269688917399,19.0768649830918,10.5701811473657));
#31019=CARTESIAN_POINT('Ctrl Pts',(4.8897033552574,19.3930621535495,-10.5701811473657));
#31020=CARTESIAN_POINT('Ctrl Pts',(3.99527368840464,19.6185807284261,-3.52339371578858));
#31021=CARTESIAN_POINT('Ctrl Pts',(3.08522288423924,19.7821212566387,3.52339371578858));
#31022=CARTESIAN_POINT('Ctrl Pts',(2.16823719579937,19.8821227754131,10.5701811473657));
#31023=CARTESIAN_POINT('Ctrl Pts',(5.10455570284159,16.6634935339443,-10.5701811473657));
#31024=CARTESIAN_POINT('Ctrl Pts',(4.33601678645625,16.8989213390741,-3.52339371578858));
#31025=CARTESIAN_POINT('Ctrl Pts',(3.55116933626636,17.0810942372497,3.52339371578858));
#31026=CARTESIAN_POINT('Ctrl Pts',(2.75750456340205,17.2082734247813,10.5701811473657));
#31027=CARTESIAN_POINT('Origin',(-251.389004561992,-1139.85959012281,-6.00190077378154));
#31028=CARTESIAN_POINT('Origin',(-161.200190539747,-1156.06695970508,6.00190077397284));
#31029=CARTESIAN_POINT('Ctrl Pts',(3.22388576724349,19.7384538622191,-10.5701811473657));
#31030=CARTESIAN_POINT('Ctrl Pts',(2.31352624920544,19.8871430713012,-3.52339371578857));
#31031=CARTESIAN_POINT('Ctrl Pts',(1.39286933918331,19.9727508933579,3.52339371578858));
#31032=CARTESIAN_POINT('Ctrl Pts',(0.470702522298857,19.9944602189378,10.5701811473657));
#31033=CARTESIAN_POINT('Ctrl Pts',(2.81354048537629,19.2255156632199,-10.5701811473657));
#31034=CARTESIAN_POINT('Ctrl Pts',(1.92680995902451,19.3552623862032,-3.52339371578858));
#31035=CARTESIAN_POINT('Ctrl Pts',(1.03117555411552,19.4236215458326,3.52339371578858));
#31036=CARTESIAN_POINT('Ctrl Pts',(0.135024498952097,19.4298283822644,10.5701811473657));
#31037=CARTESIAN_POINT('Ctrl Pts',(2.30571422899442,18.4093435092564,-10.5701811473657));
#31038=CARTESIAN_POINT('Ctrl Pts',(1.45665899888885,18.5156881042572,-3.52339371578857));
#31039=CARTESIAN_POINT('Ctrl Pts',(0.600227987416909,18.5631911577303,3.52339371578857));
#31040=CARTESIAN_POINT('Ctrl Pts',(-0.255380157229852,18.5514157821683,
10.5701811473657));
#31041=CARTESIAN_POINT('Ctrl Pts',(2.02788285372489,17.6904768579854,-10.5701811473657));
#31042=CARTESIAN_POINT('Ctrl Pts',(1.21196996348229,17.7840001943948,-3.52339371578857));
#31043=CARTESIAN_POINT('Ctrl Pts',(0.389605628258776,17.8210031964629,3.52339371578858));
#31044=CARTESIAN_POINT('Ctrl Pts',(-0.431408578760428,17.8011001617743,
10.5701811473657));
#31045=CARTESIAN_POINT('Ctrl Pts',(1.95191613165048,17.393484469299,-10.5701811473657));
#31046=CARTESIAN_POINT('Ctrl Pts',(1.1497124161716,17.4835108568289,-3.52339371578858));
#31047=CARTESIAN_POINT('Ctrl Pts',(0.341266322086565,17.5179443719092,3.52339371578859));
#31048=CARTESIAN_POINT('Ctrl Pts',(-0.465687420824652,17.4964686092602,
10.5701811473657));
#31049=CARTESIAN_POINT('Ctrl Pts',(1.94228472746027,17.3259133729239,-10.5701811473657));
#31050=CARTESIAN_POINT('Ctrl Pts',(1.14318368222273,17.4154875665989,-3.52339371578856));
#31051=CARTESIAN_POINT('Ctrl Pts',(0.337911139204634,17.449710608456,3.52339371578856));
#31052=CARTESIAN_POINT('Ctrl Pts',(-0.465907217907272,17.4282149009269,
10.5701811473657));
#31053=CARTESIAN_POINT('Ctrl Pts',(1.94149567299321,17.3193273608118,-10.5701811473657));
#31054=CARTESIAN_POINT('Ctrl Pts',(1.14270896867536,17.4088713077428,-3.52339371578857));
#31055=CARTESIAN_POINT('Ctrl Pts',(0.337722475075321,17.4430653133694,3.52339371578858));
#31056=CARTESIAN_POINT('Ctrl Pts',(-0.465780373556084,17.4215830027821,
10.5701811473657));
#31057=CARTESIAN_POINT('Origin',(-62.3589149167327,-1165.58674546341,6.00000002996953));
#31058=CARTESIAN_POINT('Origin',(-153.617664909702,-1157.1016568393,-6.00000002073243));
#31059=CARTESIAN_POINT('Ctrl Pts',(4.56280126193231,19.4725664626959,-8.00000002680495));
#31060=CARTESIAN_POINT('Ctrl Pts',(4.39287106149983,19.5123844155302,-6.66666668453663));
#31061=CARTESIAN_POINT('Ctrl Pts',(4.22241961684288,19.5499778598772,-5.33333334226832));
#31062=CARTESIAN_POINT('Ctrl Pts',(4.05150533474672,19.5853339139908,-4.));
#31063=CARTESIAN_POINT('Ctrl Pts',(4.01050677803047,19.6019798080263,-8.00000002680495));
#31064=CARTESIAN_POINT('Ctrl Pts',(3.83944720635556,19.6369780875006,-6.66666668453663));
#31065=CARTESIAN_POINT('Ctrl Pts',(3.66792956388945,19.669737059504,-5.33333334226832));
#31066=CARTESIAN_POINT('Ctrl Pts',(3.49601246189943,19.7002455283466,-4.));
#31067=CARTESIAN_POINT('Ctrl Pts',(3.45270368999108,19.7078820333394,-8.00000002680495));
#31068=CARTESIAN_POINT('Ctrl Pts',(3.28071994698325,19.7380125621894,-6.66666668453664));
#31069=CARTESIAN_POINT('Ctrl Pts',(3.10834185572833,19.7658916866227,-5.33333334226832));
#31070=CARTESIAN_POINT('Ctrl Pts',(2.93562832195315,19.7915098809122,-4.));
#31071=CARTESIAN_POINT('Ctrl Pts',(2.89140904967993,19.7898901893727,-8.00000002680495));
#31072=CARTESIAN_POINT('Ctrl Pts',(2.71870967731629,19.8151224935112,-6.66666668453663));
#31073=CARTESIAN_POINT('Ctrl Pts',(2.54567999735023,19.8380940388304,-5.33333334226832));
#31074=CARTESIAN_POINT('Ctrl Pts',(2.37237930002348,19.8587969539149,-4.));
#31075=CARTESIAN_POINT('Ctrl Pts',(3.02093570876773,19.770532300459,4.));
#31076=CARTESIAN_POINT('Ctrl Pts',(2.84840526585424,19.7968949379402,5.33333334226731));
#31077=CARTESIAN_POINT('Ctrl Pts',(2.67552971846302,19.8209990280008,6.66666668453462));
#31078=CARTESIAN_POINT('Ctrl Pts',(2.50236830402084,19.8428363111485,8.00000002680193));
#31079=CARTESIAN_POINT('Ctrl Pts',(2.46019011037602,19.8562141817544,4.));
#31080=CARTESIAN_POINT('Ctrl Pts',(2.28691192490912,19.8776833938736,5.33333334226731));
#31081=CARTESIAN_POINT('Ctrl Pts',(2.11335277477001,19.8968842617394,6.66666668453462));
#31082=CARTESIAN_POINT('Ctrl Pts',(1.93957196895072,19.9138102227615,8.00000002680193));
#31083=CARTESIAN_POINT('Ctrl Pts',(1.89579755025521,19.9180252198692,4.));
#31084=CARTESIAN_POINT('Ctrl Pts',(1.72197996168025,19.9345691773675,5.33333334226731));
#31085=CARTESIAN_POINT('Ctrl Pts',(1.5479458836573,19.9488377305707,6.66666668453462));
#31086=CARTESIAN_POINT('Ctrl Pts',(1.37375478770642,19.9608260048063,8.00000002680193));
#31087=CARTESIAN_POINT('Ctrl Pts',(1.32979890822623,19.9557419021113,4.));
#31088=CARTESIAN_POINT('Ctrl Pts',(1.15565220662434,19.967346586858,5.33333334226731));
#31089=CARTESIAN_POINT('Ctrl Pts',(0.981353592741155,19.9766715663146,6.66666668453462));
#31090=CARTESIAN_POINT('Ctrl Pts',(0.806962791630517,19.9837136451893,8.00000002680193));
#31091=CARTESIAN_POINT('Ctrl Pts',(10.4959637731368,13.9127010372614,-10.5701811473657));
#31092=CARTESIAN_POINT('Ctrl Pts',(9.85429447627608,14.3967865988031,-3.52339371578857));
#31093=CARTESIAN_POINT('Ctrl Pts',(9.17908591963408,14.8364067643287,3.52339371578858));
#31094=CARTESIAN_POINT('Ctrl Pts',(8.47678283314335,15.2273654477372,10.5701811473657));
#31095=CARTESIAN_POINT('Ctrl Pts',(10.4999182019387,13.9180265095573,-10.5701811473657));
#31096=CARTESIAN_POINT('Ctrl Pts',(9.85799982437194,14.402306194464,-3.52339371578857));
#31097=CARTESIAN_POINT('Ctrl Pts',(9.18254152903524,14.8420688308861,3.52339371578857));
#31098=CARTESIAN_POINT('Ctrl Pts',(8.47996496835067,15.2331854286518,10.5701811473657));
#31099=CARTESIAN_POINT('Ctrl Pts',(10.5393711248066,13.9737196134162,-10.5701811473657));
#31100=CARTESIAN_POINT('Ctrl Pts',(9.89488859896274,14.4598037886812,-3.52339371578858));
#31101=CARTESIAN_POINT('Ctrl Pts',(9.21672460434453,14.9012375244243,3.52339371578858));
#31102=CARTESIAN_POINT('Ctrl Pts',(8.5113595213698,15.2937877139304,10.5701811473657));
#31103=CARTESIAN_POINT('Ctrl Pts',(10.6883641017233,14.2416305529831,-10.5701811473657));
#31104=CARTESIAN_POINT('Ctrl Pts',(10.0315214461228,14.7345992990549,-3.52339371578856));
#31105=CARTESIAN_POINT('Ctrl Pts',(9.34053431369493,15.182023467968,3.52339371578857));
#31106=CARTESIAN_POINT('Ctrl Pts',(8.62197769029742,15.5796876954155,10.5701811473657));
#31107=CARTESIAN_POINT('Ctrl Pts',(10.9807596939229,14.9546925405841,-10.5701811473657));
#31108=CARTESIAN_POINT('Ctrl Pts',(10.2910338072703,15.461133240779,-3.5233937157886));
#31109=CARTESIAN_POINT('Ctrl Pts',(9.56621540573734,15.9197907568147,3.5233937157886));
#31110=CARTESIAN_POINT('Ctrl Pts',(8.81323173181671,16.3262628571385,10.5701811473657));
#31111=CARTESIAN_POINT('Ctrl Pts',(11.1730334267774,15.8965348871784,-10.5701811473657));
#31112=CARTESIAN_POINT('Ctrl Pts',(10.4398585735511,16.4118793808771,-3.52339371578856));
#31113=CARTESIAN_POINT('Ctrl Pts',(9.67101229504786,16.8763246803423,3.52339371578856));
#31114=CARTESIAN_POINT('Ctrl Pts',(8.87376686242201,17.2856229001603,10.5701811473657));
#31115=CARTESIAN_POINT('Ctrl Pts',(11.2276360580494,16.5511403577636,-10.5701811473657));
#31116=CARTESIAN_POINT('Ctrl Pts',(10.464278995546,17.068971461469,-3.52339371578857));
#31117=CARTESIAN_POINT('Ctrl Pts',(9.66504512535763,17.5339049951292,3.52339371578858));
#31118=CARTESIAN_POINT('Ctrl Pts',(8.83756297427067,17.9415032611597,10.5701811473657));
#31119=CARTESIAN_POINT('Ctrl Pts',(10.4959637731368,13.9127010372614,-10.5701811473657));
#31120=CARTESIAN_POINT('Ctrl Pts',(9.85429447627608,14.3967865988031,-3.52339371578857));
#31121=CARTESIAN_POINT('Ctrl Pts',(9.17908591963408,14.8364067643287,3.52339371578858));
#31122=CARTESIAN_POINT('Ctrl Pts',(8.47678283314335,15.2273654477372,10.5701811473657));
#31123=CARTESIAN_POINT('Origin',(-626.083332913132,-985.137542209956,-6.00190077217363));
#31124=CARTESIAN_POINT('Origin',(-546.876816795099,-1031.21387892502,6.00190077273223));
#31125=CARTESIAN_POINT('Ctrl Pts',(9.78041047709324,17.4454455632284,-10.5701811473657));
#31126=CARTESIAN_POINT('Ctrl Pts',(8.97580706054609,17.896529008279,-3.52339371578857));
#31127=CARTESIAN_POINT('Ctrl Pts',(8.13995215573091,18.2918572549299,3.52339371578858));
#31128=CARTESIAN_POINT('Ctrl Pts',(7.28082382967794,18.6276569745418,10.5701811473657));
#31129=CARTESIAN_POINT('Ctrl Pts',(9.21937684849878,17.1037876754904,-10.5701811473657));
#31130=CARTESIAN_POINT('Ctrl Pts',(8.43049870923998,17.5289894151062,-3.52339371578857));
#31131=CARTESIAN_POINT('Ctrl Pts',(7.61225787779935,17.8995510201292,3.52339371578859));
#31132=CARTESIAN_POINT('Ctrl Pts',(6.77227420746117,18.2118852506227,10.5701811473657));
#31133=CARTESIAN_POINT('Ctrl Pts',(8.46303091459466,16.5105131605735,-10.5701811473657));
#31134=CARTESIAN_POINT('Ctrl Pts',(7.70155197397604,16.9008383831229,-3.52339371578856));
#31135=CARTESIAN_POINT('Ctrl Pts',(6.91301848570708,17.2383936792967,3.52339371578858));
#31136=CARTESIAN_POINT('Ctrl Pts',(6.10498241040404,17.5199636659301,10.5701811473657));
#31137=CARTESIAN_POINT('Ctrl Pts',(7.95608662513995,15.9300303069687,-10.5701811473657));
#31138=CARTESIAN_POINT('Ctrl Pts',(7.22136616794635,16.2969721396903,-3.52339371578857));
#31139=CARTESIAN_POINT('Ctrl Pts',(6.46125271502429,16.6130088771473,3.52339371578859));
#31140=CARTESIAN_POINT('Ctrl Pts',(5.68294448440402,16.8751095390476,10.5701811473657));
#31141=CARTESIAN_POINT('Ctrl Pts',(7.78312379454569,15.6769313834283,-10.5701811473657));
#31142=CARTESIAN_POINT('Ctrl Pts',(7.06008972071931,16.035898345205,-3.52339371578856));
#31143=CARTESIAN_POINT('Ctrl Pts',(6.31217625418917,16.3447602197371,3.52339371578858));
#31144=CARTESIAN_POINT('Ctrl Pts',(5.54654263325149,16.6005740388537,10.5701811473657));
#31145=CARTESIAN_POINT('Ctrl Pts',(7.7509620009088,15.6167324440349,-10.5701811473657));
#31146=CARTESIAN_POINT('Ctrl Pts',(7.0306888239964,15.9742133068677,-3.52339371578857));
#31147=CARTESIAN_POINT('Ctrl Pts',(6.2856851272823,16.2817918773406,3.52339371578859));
#31148=CARTESIAN_POINT('Ctrl Pts',(5.52299098368265,16.536514589304,10.5701811473657));
#31149=CARTESIAN_POINT('Ctrl Pts',(7.74796798344852,15.610813489587,-10.5701811473657));
#31150=CARTESIAN_POINT('Ctrl Pts',(7.02797984538244,15.9681584188516,-3.52339371578857));
#31151=CARTESIAN_POINT('Ctrl Pts',(6.28323501621944,16.2756118695303,3.52339371578858));
#31152=CARTESIAN_POINT('Ctrl Pts',(5.52084193563401,16.5302392602455,10.5701811473657));
#31153=CARTESIAN_POINT('Origin',(-457.260143339527,-1073.95971906824,6.00190077300612));
#31154=CARTESIAN_POINT('Origin',(-540.095923847419,-1034.78147929382,-6.00190077463665));
#31155=CARTESIAN_POINT('Ctrl Pts',(10.9476406484403,16.7376570711859,-8.00000002680495));
#31156=CARTESIAN_POINT('Ctrl Pts',(10.8015770349805,16.8331932591463,-6.66666668453663));
#31157=CARTESIAN_POINT('Ctrl Pts',(10.6542627854578,16.9268173689207,-5.33333334226832));
#31158=CARTESIAN_POINT('Ctrl Pts',(10.5057483784805,17.0184973193304,-4.));
#31159=CARTESIAN_POINT('Ctrl Pts',(10.4729155683351,17.0481616753661,-8.00000002680495));
#31160=CARTESIAN_POINT('Ctrl Pts',(10.3241422676794,17.1395551195499,-6.66666668453664));
#31161=CARTESIAN_POINT('Ctrl Pts',(10.1741726330192,17.2290009724651,-5.33333334226832));
#31162=CARTESIAN_POINT('Ctrl Pts',(10.0230579117785,17.3164686673708,-4.));
#31163=CARTESIAN_POINT('Ctrl Pts',(9.98497281693299,17.3384571071364,-8.00000002680495));
#31164=CARTESIAN_POINT('Ctrl Pts',(9.83366621052916,17.4255924471904,-6.66666668453663));
#31165=CARTESIAN_POINT('Ctrl Pts',(9.68121901232621,17.5107470341715,-5.33333334226832));
#31166=CARTESIAN_POINT('Ctrl Pts',(9.52768331761046,17.5938917698793,-4.));
#31167=CARTESIAN_POINT('Ctrl Pts',(9.48557682662632,17.6074936395323,-8.00000002680495));
#31168=CARTESIAN_POINT('Ctrl Pts',(9.33192245707975,17.6902709136248,-6.66666668453663));
#31169=CARTESIAN_POINT('Ctrl Pts',(9.17718447486116,17.7710367411908,-5.33333334226832));
#31170=CARTESIAN_POINT('Ctrl Pts',(9.02141590239063,17.8497634470626,-4.));
#31171=CARTESIAN_POINT('Ctrl Pts',(9.60067128442543,17.5450024476604,4.));
#31172=CARTESIAN_POINT('Ctrl Pts',(9.44756225340845,17.6287841103792,5.33333334226731));
#31173=CARTESIAN_POINT('Ctrl Pts',(9.29335646154787,17.7105614654362,6.66666668453462));
#31174=CARTESIAN_POINT('Ctrl Pts',(9.13810674890371,17.7903064910541,8.00000002680193));
#31175=CARTESIAN_POINT('Ctrl Pts',(9.10304771279964,17.8173033691799,4.));
#31176=CARTESIAN_POINT('Ctrl Pts',(8.94756238357932,17.8967424592111,5.33333334226731));
#31177=CARTESIAN_POINT('Ctrl Pts',(8.79103721450315,17.9741460984632,6.66666668453462));
#31178=CARTESIAN_POINT('Ctrl Pts',(8.63352569325523,18.049487835249,8.00000002680193));
#31179=CARTESIAN_POINT('Ctrl Pts',(8.59383280894276,18.0684203698839,4.));
#31180=CARTESIAN_POINT('Ctrl Pts',(8.43615607031084,18.1434157212207,5.33333334226731));
#31181=CARTESIAN_POINT('Ctrl Pts',(8.27749766403898,18.2163469356839,6.66666668453462));
#31182=CARTESIAN_POINT('Ctrl Pts',(8.11791180783962,18.2871890921223,8.00000002680193));
#31183=CARTESIAN_POINT('Ctrl Pts',(8.0748679267195,18.2974453945363,4.));
#31184=CARTESIAN_POINT('Ctrl Pts',(7.91519259223033,18.3679119110009,5.33333334226731));
#31185=CARTESIAN_POINT('Ctrl Pts',(7.75459480176132,18.436288162287,6.66666668453462));
#31186=CARTESIAN_POINT('Ctrl Pts',(7.59312958565075,18.5025507186311,8.00000002680193));
#31187=CARTESIAN_POINT('Ctrl Pts',(14.6214037084642,9.48383146588571,-10.5701811473657));
#31188=CARTESIAN_POINT('Ctrl Pts',(14.1839988183597,10.1581869207755,-3.52339371578857));
#31189=CARTESIAN_POINT('Ctrl Pts',(13.6998692722136,10.8022296735859,3.52339371578858));
#31190=CARTESIAN_POINT('Ctrl Pts',(13.1736359892169,11.4098124657167,10.5701811473657));
#31191=CARTESIAN_POINT('Ctrl Pts',(14.6297097580075,9.48930918495536,-10.5701811473657));
#31192=CARTESIAN_POINT('Ctrl Pts',(14.1920565364594,10.1641111402026,-3.52339371578859));
#31193=CARTESIAN_POINT('Ctrl Pts',(13.7076479822366,10.8083926490179,3.5233937157886));
#31194=CARTESIAN_POINT('Ctrl Pts',(13.1811071587353,11.4163834238849,10.5701811473657));
#31195=CARTESIAN_POINT('Ctrl Pts',(14.7449772223308,9.57135777968399,-10.5701811473657));
#31196=CARTESIAN_POINT('Ctrl Pts',(14.3035366338095,10.2514358632128,-3.52339371578855));
#31197=CARTESIAN_POINT('Ctrl Pts',(13.8149763785592,10.9008517199749,3.52339371578857));
#31198=CARTESIAN_POINT('Ctrl Pts',(13.2839566880579,11.5135458371248,10.5701811473657));
#31199=CARTESIAN_POINT('Ctrl Pts',(15.2682377029358,10.0811139468336,-10.5701811473657));
#31200=CARTESIAN_POINT('Ctrl Pts',(14.8032868804182,10.7853243667585,-3.52339371578858));
#31201=CARTESIAN_POINT('Ctrl Pts',(14.2895432842685,11.4572463383409,3.52339371578859));
#31202=CARTESIAN_POINT('Ctrl Pts',(13.7319096587419,12.090599575147,10.5701811473657));
#31203=CARTESIAN_POINT('Ctrl Pts',(15.8444191030467,10.9176358492752,-10.5701811473657));
#31204=CARTESIAN_POINT('Ctrl Pts',(15.3408980412456,11.6485449936036,-3.52339371578856));
#31205=CARTESIAN_POINT('Ctrl Pts',(14.7867271085875,12.344118032929,3.52339371578858));
#31206=CARTESIAN_POINT('Ctrl Pts',(14.1872095083049,12.9985951401616,10.5701811473657));
#31207=CARTESIAN_POINT('Ctrl Pts',(16.211349445681,11.7129052395219,-10.5701811473657));
#31208=CARTESIAN_POINT('Ctrl Pts',(15.6711371857387,12.4605907660142,-3.52339371578857));
#31209=CARTESIAN_POINT('Ctrl Pts',(15.0791197221122,13.1708394318101,3.52339371578858));
#31210=CARTESIAN_POINT('Ctrl Pts',(14.4409477424756,13.8368720561798,10.5701811473657));
#31211=CARTESIAN_POINT('Ctrl Pts',(14.6214037084642,9.48383146588571,-10.5701811473657));
#31212=CARTESIAN_POINT('Ctrl Pts',(14.1839988183597,10.1581869207755,-3.52339371578857));
#31213=CARTESIAN_POINT('Ctrl Pts',(13.6998692722136,10.8022296735859,3.52339371578858));
#31214=CARTESIAN_POINT('Ctrl Pts',(13.1736359892169,11.4098124657167,10.5701811473657));
#31215=CARTESIAN_POINT('Origin',(-925.262771311062,-711.593367601486,-6.00190077290402));
#31216=CARTESIAN_POINT('Origin',(-866.592027872364,-781.981185220022,6.00190077473778));
#31217=CARTESIAN_POINT('Ctrl Pts',(15.1572733542511,13.0482590706843,-10.5701811473657));
#31218=CARTESIAN_POINT('Ctrl Pts',(14.5554730855096,13.7473294316085,-3.52339371578856));
#31219=CARTESIAN_POINT('Ctrl Pts',(13.9052366228784,14.4046956825171,3.52339371578859));
#31220=CARTESIAN_POINT('Ctrl Pts',(13.2127703426728,15.0140833946989,10.5701811473657));
#31221=CARTESIAN_POINT('Ctrl Pts',(14.5132203124649,12.9190904765551,-10.5701811473657));
#31222=CARTESIAN_POINT('Ctrl Pts',(13.9173449061403,13.5884616281791,-3.52339371578857));
#31223=CARTESIAN_POINT('Ctrl Pts',(13.275189568012,14.216530480834,3.5233937157886));
#31224=CARTESIAN_POINT('Ctrl Pts',(12.5926877095625,14.7973199880585,10.5701811473657));
#31225=CARTESIAN_POINT('Ctrl Pts',(13.5995754203915,12.6202781311691,-10.5701811473657));
#31226=CARTESIAN_POINT('Ctrl Pts',(13.0175183674916,13.2475049990765,-3.52339371578855));
#31227=CARTESIAN_POINT('Ctrl Pts',(12.3919902857833,13.8343975281826,3.52339371578858));
#31228=CARTESIAN_POINT('Ctrl Pts',(11.7289873555787,14.3753513812935,10.5701811473657));
#31229=CARTESIAN_POINT('Ctrl Pts',(12.9246670167664,12.2481892936844,-10.5701811473657));
#31230=CARTESIAN_POINT('Ctrl Pts',(12.3597571229874,12.8442910222742,-3.52339371578857));
#31231=CARTESIAN_POINT('Ctrl Pts',(11.7535751548201,13.4012425144143,3.5233937157886));
#31232=CARTESIAN_POINT('Ctrl Pts',(11.1118483597182,13.9137336649384,10.5701811473657));
#31233=CARTESIAN_POINT('Ctrl Pts',(12.6755702095651,12.069510984472,-10.5701811473657));
#31234=CARTESIAN_POINT('Ctrl Pts',(12.1189143575221,12.6541218071276,-3.52339371578855));
#31235=CARTESIAN_POINT('Ctrl Pts',(11.5217426635648,13.2001584940098,3.52339371578858));
#31236=CARTESIAN_POINT('Ctrl Pts',(10.8897758788143,13.7024069729043,10.5701811473657));
#31237=CARTESIAN_POINT('Ctrl Pts',(12.624758865043,12.0239431039938,-10.5701811473657));
#31238=CARTESIAN_POINT('Ctrl Pts',(12.0701891316902,12.6062131680716,-3.52339371578857));
#31239=CARTESIAN_POINT('Ctrl Pts',(11.4753127221865,13.1500487521856,3.52339371578859));
#31240=CARTESIAN_POINT('Ctrl Pts',(10.8457349619827,13.6502665652722,10.5701811473657));
#31241=CARTESIAN_POINT('Ctrl Pts',(12.6199210072709,12.0194051204483,-10.5701811473657));
#31242=CARTESIAN_POINT('Ctrl Pts',(12.0655726308006,12.6014499597276,-3.52339371578856));
#31243=CARTESIAN_POINT('Ctrl Pts',(11.4708966837348,13.145079431777,3.52339371578859));
#31244=CARTESIAN_POINT('Ctrl Pts',(10.8415692284374,13.6451047025743,10.5701811473657));
#31245=CARTESIAN_POINT('Origin',(-796.994418233151,-852.807711458368,6.00000003080237));
#31246=CARTESIAN_POINT('Origin',(-861.44856672619,-787.647762729537,-6.00000001934937));
#31247=CARTESIAN_POINT('Ctrl Pts',(16.0120330027781,11.983939215381,-8.00000002680495));
#31248=CARTESIAN_POINT('Ctrl Pts',(15.9074534037436,12.1236705642356,-6.66666668453663));
#31249=CARTESIAN_POINT('Ctrl Pts',(15.8010446219743,12.262032890054,-5.33333334226832));
#31250=CARTESIAN_POINT('Ctrl Pts',(15.6928431194365,12.3989787816882,-4.));
#31251=CARTESIAN_POINT('Ctrl Pts',(15.6721361773263,12.4380836405871,-8.00000002680495));
#31252=CARTESIAN_POINT('Ctrl Pts',(15.5635934034088,12.574848851288,-6.66666668453663));
#31253=CARTESIAN_POINT('Ctrl Pts',(15.4532603278107,12.7101930951734,-5.33333334226832));
#31254=CARTESIAN_POINT('Ctrl Pts',(15.3411746529166,12.8440701212508,-4.));
#31255=CARTESIAN_POINT('Ctrl Pts',(15.3129068596486,12.8777583654387,-8.00000002680495));
#31256=CARTESIAN_POINT('Ctrl Pts',(15.2005271996287,13.0113887087055,-6.66666668453663));
#31257=CARTESIAN_POINT('Ctrl Pts',(15.086398276462,13.1435478582967,-5.33333334226832));
#31258=CARTESIAN_POINT('Ctrl Pts',(14.970559091534,13.2741906532108,-4.));
#31259=CARTESIAN_POINT('Ctrl Pts',(14.9356440460772,13.3013734978339,-8.00000002680495));
#31260=CARTESIAN_POINT('Ctrl Pts',(14.819567664012,13.4317115809623,-6.66666668453663));
#31261=CARTESIAN_POINT('Ctrl Pts',(14.7017850638858,13.5605301399942,-5.33333334226832));
#31262=CARTESIAN_POINT('Ctrl Pts',(14.5823366050108,13.6877850340427,-4.));
#31263=CARTESIAN_POINT('Ctrl Pts',(15.0224242123638,13.2032863630154,4.));
#31264=CARTESIAN_POINT('Ctrl Pts',(14.9072038020326,13.3343817459623,5.33333334226731));
#31265=CARTESIAN_POINT('Ctrl Pts',(14.7902672600361,13.4639688100905,6.66666668453462));
#31266=CARTESIAN_POINT('Ctrl Pts',(14.6716546557766,13.5920031511778,8.00000002680193));
#31267=CARTESIAN_POINT('Ctrl Pts',(14.6479434143837,13.6293628148902,4.));
#31268=CARTESIAN_POINT('Ctrl Pts',(14.529004766833,13.7571902561793,5.33333334226731));
#31269=CARTESIAN_POINT('Ctrl Pts',(14.4083928242758,13.8834606455681,6.66666668453462));
#31270=CARTESIAN_POINT('Ctrl Pts',(14.2861488016842,14.0081308327355,8.00000002680193));
#31271=CARTESIAN_POINT('Ctrl Pts',(14.2553249994075,14.0394973618063,4.));
#31272=CARTESIAN_POINT('Ctrl Pts',(14.1328072524584,14.1638985607967,5.33333334226731));
#31273=CARTESIAN_POINT('Ctrl Pts',(14.0086610632827,14.2866958557057,6.66666668453462));
#31274=CARTESIAN_POINT('Ctrl Pts',(13.882928856329,14.4078472847614,8.00000002680193));
#31275=CARTESIAN_POINT('Ctrl Pts',(13.845988700892,14.4322069308464,4.));
#31276=CARTESIAN_POINT('Ctrl Pts',(13.7200439354119,14.5530359771683,5.33333334226731));
#31277=CARTESIAN_POINT('Ctrl Pts',(13.5925174320586,14.6722163152528,6.66666668453462));
#31278=CARTESIAN_POINT('Ctrl Pts',(13.4634528889838,14.78970710684,8.00000002680193));
#31279=CARTESIAN_POINT('Ctrl Pts',(16.9832865676143,3.91107185327861,-10.5701811473657));
#31280=CARTESIAN_POINT('Ctrl Pts',(16.8029035694212,4.69435998123015,-3.52339371578857));
#31281=CARTESIAN_POINT('Ctrl Pts',(16.5682462020274,5.46514426027785,3.52339371578857));
#31282=CARTESIAN_POINT('Ctrl Pts',(16.2815542228302,6.21606770943294,10.5701811473657));
#31283=CARTESIAN_POINT('Ctrl Pts',(16.9897389834306,3.91260954390058,-10.5701811473657));
#31284=CARTESIAN_POINT('Ctrl Pts',(16.8092899584406,4.69620648496871,-3.52339371578858));
#31285=CARTESIAN_POINT('Ctrl Pts',(16.5745328586345,5.46726043199356,3.52339371578858));
#31286=CARTESIAN_POINT('Ctrl Pts',(16.287732891443,6.21848063638781,10.5701811473657));
#31287=CARTESIAN_POINT('Ctrl Pts',(17.0557613661601,3.92991270646709,-10.5701811473657));
#31288=CARTESIAN_POINT('Ctrl Pts',(16.8745079936752,4.71654017008886,-3.52339371578856));
#31289=CARTESIAN_POINT('Ctrl Pts',(16.6387524141881,5.49061356475807,3.52339371578857));
#31290=CARTESIAN_POINT('Ctrl Pts',(16.3507378099998,6.24472439171618,10.5701811473657));
#31291=CARTESIAN_POINT('Ctrl Pts',(17.3421065865863,4.03937349046947,-10.5701811473657));
#31292=CARTESIAN_POINT('Ctrl Pts',(17.1558101221977,4.83921977956265,-3.52339371578857));
#31293=CARTESIAN_POINT('Ctrl Pts',(16.9140820327625,5.62612468710593,3.52339371578857));
#31294=CARTESIAN_POINT('Ctrl Pts',(16.6192493625613,6.39263245314738,10.5701811473657));
#31295=CARTESIAN_POINT('Ctrl Pts',(18.0244436775359,4.39766136660597,-10.5701811473657));
#31296=CARTESIAN_POINT('Ctrl Pts',(17.8216168089676,5.22896469136215,-3.52339371578856));
#31297=CARTESIAN_POINT('Ctrl Pts',(17.5611932309209,6.04622142745388,3.52339371578857));
#31298=CARTESIAN_POINT('Ctrl Pts',(17.2456495103603,6.84160568476519,10.5701811473657));
#31299=CARTESIAN_POINT('Ctrl Pts',(18.7771350612562,4.99556415374892,-10.5701811473657));
#31300=CARTESIAN_POINT('Ctrl Pts',(18.5467476225913,5.86161661525353,-3.52339371578857));
#31301=CARTESIAN_POINT('Ctrl Pts',(18.2563169179228,6.7116071841068,3.52339371578858));
#31302=CARTESIAN_POINT('Ctrl Pts',(17.9086833416741,7.53760726560638,10.5701811473657));
#31303=CARTESIAN_POINT('Ctrl Pts',(19.2397349758694,5.46192256062902,-10.5701811473657));
#31304=CARTESIAN_POINT('Ctrl Pts',(18.9878250124769,6.34928060711398,-3.52339371578857));
#31305=CARTESIAN_POINT('Ctrl Pts',(18.6744299210032,7.21917793504633,3.52339371578857));
#31306=CARTESIAN_POINT('Ctrl Pts',(18.3025409945928,8.06331154931088,10.5701811473657));
#31307=CARTESIAN_POINT('Ctrl Pts',(16.9832865676143,3.91107185327861,-10.5701811473657));
#31308=CARTESIAN_POINT('Ctrl Pts',(16.8029035694212,4.69435998123015,-3.52339371578857));
#31309=CARTESIAN_POINT('Ctrl Pts',(16.5682462020274,5.46514426027785,3.52339371578857));
#31310=CARTESIAN_POINT('Ctrl Pts',(16.2815542228302,6.21606770943294,10.5701811473657));
#31311=CARTESIAN_POINT('Origin',(-1112.8418640586,-352.220530871087,-6.00190077429466));
#31312=CARTESIAN_POINT('Origin',(-1081.78345086687,-438.4300197552,6.00190077312313));
#31313=CARTESIAN_POINT('Ctrl Pts',(18.7059453597305,7.07725995777758,-10.5701811473657));
#31314=CARTESIAN_POINT('Ctrl Pts',(18.3795342330452,7.93999903151655,-3.52339371578857));
#31315=CARTESIAN_POINT('Ctrl Pts',(17.9933443266979,8.78011521479376,3.52339371578857));
#31316=CARTESIAN_POINT('Ctrl Pts',(17.5510617457069,9.58958976753269,10.5701811473657));
#31317=CARTESIAN_POINT('Ctrl Pts',(18.0565552078921,7.17616029669805,-10.5701811473657));
#31318=CARTESIAN_POINT('Ctrl Pts',(17.7255539028776,8.0089648203215,-3.52339371578857));
#31319=CARTESIAN_POINT('Ctrl Pts',(17.3369374692435,8.81878654729075,3.52339371578857));
#31320=CARTESIAN_POINT('Ctrl Pts',(16.8942372196888,9.59797954490639,10.5701811473657));
#31321=CARTESIAN_POINT('Ctrl Pts',(17.0958111919983,7.20785561730521,-10.5701811473657));
#31322=CARTESIAN_POINT('Ctrl Pts',(16.7633806977713,7.99633131329305,-3.52339371578856));
#31323=CARTESIAN_POINT('Ctrl Pts',(16.3763053385156,8.76177323989849,3.52339371578857));
#31324=CARTESIAN_POINT('Ctrl Pts',(15.9383034918164,9.49686394106645,10.5701811473657));
#31325=CARTESIAN_POINT('Ctrl Pts',(16.3343420851163,7.08903734850001,-10.5701811473657));
#31326=CARTESIAN_POINT('Ctrl Pts',(16.0073792251723,7.84240030692999,-3.52339371578856));
#31327=CARTESIAN_POINT('Ctrl Pts',(15.6282430292671,8.57309000696066,3.52339371578857));
#31328=CARTESIAN_POINT('Ctrl Pts',(15.2004993921047,9.27415764976289,10.5701811473657));
#31329=CARTESIAN_POINT('Ctrl Pts',(16.039156011872,7.00633068060153,-10.5701811473657));
#31330=CARTESIAN_POINT('Ctrl Pts',(15.7160192927444,7.7460726709814,-3.52339371578857));
#31331=CARTESIAN_POINT('Ctrl Pts',(15.3416169168207,8.46342410640404,3.52339371578857));
#31332=CARTESIAN_POINT('Ctrl Pts',(14.9195414893454,9.15152866611962,10.5701811473657));
#31333=CARTESIAN_POINT('Ctrl Pts',(15.9758234884508,6.98088877109892,-10.5701811473657));
#31334=CARTESIAN_POINT('Ctrl Pts',(15.6538464930781,7.71771767330283,-3.52339371578856));
#31335=CARTESIAN_POINT('Ctrl Pts',(15.2808482452121,8.43221567345516,3.52339371578857));
#31336=CARTESIAN_POINT('Ctrl Pts',(14.8603232378636,9.11759493697779,10.5701811473657));
#31337=CARTESIAN_POINT('Ctrl Pts',(15.9697253074185,6.97827910625622,-10.5701811473657));
#31338=CARTESIAN_POINT('Ctrl Pts',(15.647879288057,7.71482065786624,-3.52339371578857));
#31339=CARTESIAN_POINT('Ctrl Pts',(15.2749989187868,8.42905641384053,3.52339371578857));
#31340=CARTESIAN_POINT('Ctrl Pts',(14.8546432677704,9.11416913747482,10.5701811473657));
#31341=CARTESIAN_POINT('Origin',(-1040.60718933536,-528.788968262105,6.00000003130594));
#31342=CARTESIAN_POINT('Origin',(-1078.88826202927,-445.514028128251,-6.00000002213574));
#31343=CARTESIAN_POINT('Ctrl Pts',(19.1451378645417,5.78478142609488,-8.00000002680495));
#31344=CARTESIAN_POINT('Ctrl Pts',(19.0946561230066,5.95185427295671,-6.66666668453663));
#31345=CARTESIAN_POINT('Ctrl Pts',(19.0419872784984,6.11826627631489,-5.33333334226832));
#31346=CARTESIAN_POINT('Ctrl Pts',(18.9871493784903,6.28396041353657,-4.));
#31347=CARTESIAN_POINT('Ctrl Pts',(18.9810658672356,6.32778915218908,-8.00000002680495));
#31348=CARTESIAN_POINT('Ctrl Pts',(18.9258454805117,6.4934302265572,-6.66666668453664));
#31349=CARTESIAN_POINT('Ctrl Pts',(18.8684567612354,6.65834834813178,-5.33333334226832));
#31350=CARTESIAN_POINT('Ctrl Pts',(18.8089193192887,6.82248716022144,-4.));
#31351=CARTESIAN_POINT('Ctrl Pts',(18.7938783406543,6.86381190939714,-8.00000002680495));
#31352=CARTESIAN_POINT('Ctrl Pts',(18.733980272564,7.02781946430488,-6.66666668453663));
#31353=CARTESIAN_POINT('Ctrl Pts',(18.671935256931,7.19104283260414,-5.33333334226832));
#31354=CARTESIAN_POINT('Ctrl Pts',(18.6077644970973,7.35342623757559,-4.));
#31355=CARTESIAN_POINT('Ctrl Pts',(18.5842521669411,7.3909114049313,-8.00000002680495));
#31356=CARTESIAN_POINT('Ctrl Pts',(18.5197542971393,7.5530896006851,-6.66666668453663));
#31357=CARTESIAN_POINT('Ctrl Pts',(18.4531333989669,7.714423471804,-5.33333334226832));
#31358=CARTESIAN_POINT('Ctrl Pts',(18.3844123006991,7.87485773572478,-4.));
#31359=CARTESIAN_POINT('Ctrl Pts',(18.6322510729221,7.2690590832371,4.));
#31360=CARTESIAN_POINT('Ctrl Pts',(18.5688165652349,7.43165614846694,5.33333334226731));
#31361=CARTESIAN_POINT('Ctrl Pts',(18.5032535458669,7.5934228092312,6.66666668453462));
#31362=CARTESIAN_POINT('Ctrl Pts',(18.4355844806013,7.75430363466721,8.00000002680193));
#31363=CARTESIAN_POINT('Ctrl Pts',(18.4260809595722,7.79751995715235,4.));
#31364=CARTESIAN_POINT('Ctrl Pts',(18.3580347499332,7.95831787374795,5.33333334226731));
#31365=CARTESIAN_POINT('Ctrl Pts',(18.2878836142101,8.11822494076053,6.66666668453462));
#31366=CARTESIAN_POINT('Ctrl Pts',(18.215651523529,8.2771865138012,8.00000002680193));
#31367=CARTESIAN_POINT('Ctrl Pts',(18.1974146087534,8.31720377098127,4.));
#31368=CARTESIAN_POINT('Ctrl Pts',(18.1248333019387,8.47600619706092,5.33333334226731));
#31369=CARTESIAN_POINT('Ctrl Pts',(18.0501731924764,8.63385840635456,6.66666668453462));
#31370=CARTESIAN_POINT('Ctrl Pts',(17.9734597945365,8.7907064576789,8.00000002680193));
#31371=CARTESIAN_POINT('Ctrl Pts',(17.9470788927071,8.82623131460692,4.));
#31372=CARTESIAN_POINT('Ctrl Pts',(17.8700554936997,8.9828491245528,5.33333334226731));
#31373=CARTESIAN_POINT('Ctrl Pts',(17.7909818558573,9.13845864174832,6.66666668453462));
#31374=CARTESIAN_POINT('Ctrl Pts',(17.7098850745029,9.2930065451338,8.00000002680193));
#31375=CARTESIAN_POINT('Ctrl Pts',(17.2967344200949,-2.13342074610697,-10.5701811473657));
#31376=CARTESIAN_POINT('Ctrl Pts',(17.3951301655649,-1.33567605342618,-3.52339371578857));
#31377=CARTESIAN_POINT('Ctrl Pts',(17.438248118605,-0.531118207758813,3.52339371578858));
#31378=CARTESIAN_POINT('Ctrl Pts',(17.4256767270215,0.272573448002655,10.5701811473657));
#31379=CARTESIAN_POINT('Ctrl Pts',(17.3066182331392,-2.13456359558476,-10.5701811473657));
#31380=CARTESIAN_POINT('Ctrl Pts',(17.4051107505843,-1.33631723941131,-3.52339371578858));
#31381=CARTESIAN_POINT('Ctrl Pts',(17.4481684404393,-0.531397153098441,
3.52339371578859));
#31382=CARTESIAN_POINT('Ctrl Pts',(17.4356237054091,0.272804718796849,10.5701811473657));
#31383=CARTESIAN_POINT('Ctrl Pts',(17.4476874812992,-2.14583108338521,-10.5701811473657));
#31384=CARTESIAN_POINT('Ctrl Pts',(17.5466701372069,-1.34110850589676,-3.52339371578856));
#31385=CARTESIAN_POINT('Ctrl Pts',(17.5898512960804,-0.529582293917894,
3.52339371578857));
#31386=CARTESIAN_POINT('Ctrl Pts',(17.5768988000169,0.281101507410299,10.5701811473657));
#31387=CARTESIAN_POINT('Ctrl Pts',(18.176210560974,-2.09169814335911,-10.5701811473657));
#31388=CARTESIAN_POINT('Ctrl Pts',(18.2726952996008,-1.25337703656127,-3.52339371578858));
#31389=CARTESIAN_POINT('Ctrl Pts',(18.3110538115191,-0.408420040147124,
3.52339371578859));
#31390=CARTESIAN_POINT('Ctrl Pts',(18.290993284562,0.435196672672641,10.5701811473657));
#31391=CARTESIAN_POINT('Ctrl Pts',(19.1552502593208,-1.82120200778524,-10.5701811473657));
#31392=CARTESIAN_POINT('Ctrl Pts',(19.2393500897156,-0.937636019605692,
-3.52339371578856));
#31393=CARTESIAN_POINT('Ctrl Pts',(19.2619362575252,-0.0485819488860309,
3.52339371578857));
#31394=CARTESIAN_POINT('Ctrl Pts',(19.2233689066293,0.838139087508731,10.5701811473657));
#31395=CARTESIAN_POINT('Ctrl Pts',(19.947524519721,-1.44784858846757,-10.5701811473657));
#31396=CARTESIAN_POINT('Ctrl Pts',(20.0143009122587,-0.527846498406002,
-3.52339371578857));
#31397=CARTESIAN_POINT('Ctrl Pts',(20.0173282661883,0.396777035596821,3.52339371578858));
#31398=CARTESIAN_POINT('Ctrl Pts',(19.9565776860253,1.31719666779067,10.5701811473657));
#31399=CARTESIAN_POINT('Ctrl Pts',(17.2967344200949,-2.13342074610697,-10.5701811473657));
#31400=CARTESIAN_POINT('Ctrl Pts',(17.3951301655649,-1.33567605342618,-3.52339371578857));
#31401=CARTESIAN_POINT('Ctrl Pts',(17.438248118605,-0.531118207758813,3.52339371578858));
#31402=CARTESIAN_POINT('Ctrl Pts',(17.4256767270215,0.272573448002655,10.5701811473657));
#31403=CARTESIAN_POINT('Origin',(-1166.1958042159,49.6353000922384,-6.00190077381557));
#31404=CARTESIAN_POINT('Origin',(-1166.49582424371,-41.9977233820896,6.00190077373936));
#31405=CARTESIAN_POINT('Ctrl Pts',(19.9984057517891,0.252638042748192,-10.5701811473657));
#31406=CARTESIAN_POINT('Ctrl Pts',(19.9867538035289,1.17498683179843,-3.52339371578858));
#31407=CARTESIAN_POINT('Ctrl Pts',(19.911190687624,2.09652260757975,3.52339371578857));
#31408=CARTESIAN_POINT('Ctrl Pts',(19.7724376400266,3.00844949518813,10.5701811473657));
#31409=CARTESIAN_POINT('Ctrl Pts',(19.2298702051233,0.672692451092664,-10.5701811473657));
#31410=CARTESIAN_POINT('Ctrl Pts',(19.1987473490918,1.55970602327824,-3.52339371578858));
#31411=CARTESIAN_POINT('Ctrl Pts',(19.1064764398699,2.44424738876731,3.52339371578858));
#31412=CARTESIAN_POINT('Ctrl Pts',(18.9533120809235,3.31849128411775,10.5701811473657));
#31413=CARTESIAN_POINT('Ctrl Pts',(18.2687424654252,1.00123000436807,-10.5701811473657));
#31414=CARTESIAN_POINT('Ctrl Pts',(18.2225517496899,1.84382007141717,-3.52339371578857));
#31415=CARTESIAN_POINT('Ctrl Pts',(18.1180183606275,2.68316133395875,3.52339371578856));
#31416=CARTESIAN_POINT('Ctrl Pts',(17.9560571362275,3.51132808353326,10.5701811473657));
#31417=CARTESIAN_POINT('Ctrl Pts',(17.5447630935932,1.09882677893604,-10.5701811473657));
#31418=CARTESIAN_POINT('Ctrl Pts',(17.4940701434606,1.90802775378534,-3.52339371578858));
#31419=CARTESIAN_POINT('Ctrl Pts',(17.3873513571379,2.71366344201221,3.52339371578858));
#31420=CARTESIAN_POINT('Ctrl Pts',(17.225536025983,3.50813923868159,10.5701811473657));
#31421=CARTESIAN_POINT('Ctrl Pts',(17.4032795079184,1.09601951648447,-10.5701811473657));
#31422=CARTESIAN_POINT('Ctrl Pts',(17.3526886200656,1.89872655096413,-3.52339371578857));
#31423=CARTESIAN_POINT('Ctrl Pts',(17.2466103605934,2.69778706986935,3.52339371578856));
#31424=CARTESIAN_POINT('Ctrl Pts',(17.0857917754359,3.48584506507326,10.5701811473657));
#31425=CARTESIAN_POINT('Ctrl Pts',(17.3933450474474,1.09546964341861,-10.5701811473657));
#31426=CARTESIAN_POINT('Ctrl Pts',(17.342820765071,1.89767012603957,-3.52339371578858));
#31427=CARTESIAN_POINT('Ctrl Pts',(17.2367108492585,2.6963647927712,3.52339371578857));
#31428=CARTESIAN_POINT('Ctrl Pts',(17.0760280978245,3.48393026358523,10.5701811473657));
#31429=CARTESIAN_POINT('Origin',(-1158.70647098178,-140.980959266364,6.00190077354629));
#31430=CARTESIAN_POINT('Origin',(-1166.19501035542,-49.6539491257549,-6.00190077350844));
#31431=CARTESIAN_POINT('Ctrl Pts',(19.9690565476993,-1.11210637745949,-8.00000002680495));
#31432=CARTESIAN_POINT('Ctrl Pts',(19.9787615067239,-0.937843483654575,
-6.66666668453663));
#31433=CARTESIAN_POINT('Ctrl Pts',(19.9861852394339,-0.7634535463412,-5.33333334226832));
#31434=CARTESIAN_POINT('Ctrl Pts',(19.9913252020177,-0.588996321866056,
-4.));
#31435=CARTESIAN_POINT('Ctrl Pts',(20.0005988828589,-0.545730096184683,
-8.00000002680495));
#31436=CARTESIAN_POINT('Ctrl Pts',(20.0053612769335,-0.371191916320091,
-6.66666668453663));
#31437=CARTESIAN_POINT('Ctrl Pts',(20.0078388404912,-0.19659147645045,-5.33333334226832));
#31438=CARTESIAN_POINT('Ctrl Pts',(20.0080307256696,-0.0219884415173625,
-4.));
#31439=CARTESIAN_POINT('Ctrl Pts',(20.0080307256734,0.0219884380071485,
-8.00000002680495));
#31440=CARTESIAN_POINT('Ctrl Pts',(20.0078388405257,0.19659147294027,-6.66666668453663));
#31441=CARTESIAN_POINT('Ctrl Pts',(20.0053612769986,0.371191912810345,-5.33333334226832));
#31442=CARTESIAN_POINT('Ctrl Pts',(20.0005988829546,0.545730092675773,-4.));
#31443=CARTESIAN_POINT('Ctrl Pts',(19.991325202121,0.588996318358773,-8.00000002680495));
#31444=CARTESIAN_POINT('Ctrl Pts',(19.9861852395679,0.763453542834819,-6.66666668453663));
#31445=CARTESIAN_POINT('Ctrl Pts',(19.9787615068885,0.937843480149496,-5.33333334226832));
#31446=CARTESIAN_POINT('Ctrl Pts',(19.9690565478945,1.11210637395612,-4.));
#31447=CARTESIAN_POINT('Ctrl Pts',(19.9947534713468,0.458075998134004,4.));
#31448=CARTESIAN_POINT('Ctrl Pts',(19.9907560041241,0.632563139902936,5.33333334226731));
#31449=CARTESIAN_POINT('Ctrl Pts',(19.9844743751274,0.806997950593389,6.66666668453462));
#31450=CARTESIAN_POINT('Ctrl Pts',(19.9759107368159,0.981320658482397,8.00000002680193));
#31451=CARTESIAN_POINT('Ctrl Pts',(19.9817612010437,1.02518111344366,4.));
#31452=CARTESIAN_POINT('Ctrl Pts',(19.972814806454,1.19955490347979,5.33333334226731));
#31453=CARTESIAN_POINT('Ctrl Pts',(19.9615857398537,1.37381149585751,6.66666668453462));
#31454=CARTESIAN_POINT('Ctrl Pts',(19.9480778372514,1.54789134303979,8.00000002680193));
#31455=CARTESIAN_POINT('Ctrl Pts',(19.9446274510471,1.59173265652136,4.));
#31456=CARTESIAN_POINT('Ctrl Pts',(19.9307369611545,1.76578239343086,5.33333334226731));
#31457=CARTESIAN_POINT('Ctrl Pts',(19.9145680424726,1.93965021101785,6.66666668453462));
#31458=CARTESIAN_POINT('Ctrl Pts',(19.8961262215074,2.11327669479037,8.00000002680193));
#31459=CARTESIAN_POINT('Ctrl Pts',(19.8834864993867,2.15568194052487,4.));
#31460=CARTESIAN_POINT('Ctrl Pts',(19.8646746255167,2.32919809478258,5.33333334226731));
#31461=CARTESIAN_POINT('Ctrl Pts',(19.8435913009115,2.50246798676344,6.66666668453462));
#31462=CARTESIAN_POINT('Ctrl Pts',(19.8202437499699,2.67543224391478,8.00000002680193));
#31463=CARTESIAN_POINT('Ctrl Pts',(16.67120375536,-5.07536776045385,-12.));
#31464=CARTESIAN_POINT('Ctrl Pts',(16.9369493898684,-4.20246557304822,-4.));
#31465=CARTESIAN_POINT('Ctrl Pts',(17.1339941352951,-3.30865780933793,4.));
#31466=CARTESIAN_POINT('Ctrl Pts',(17.2599160133439,-2.4049307201863,12.));
#31467=CARTESIAN_POINT('Ctrl Pts',(16.0568250729579,-4.88832681229369,-12.));
#31468=CARTESIAN_POINT('Ctrl Pts',(16.312777266322,-4.04759341747401,-4.00000000000001));
#31469=CARTESIAN_POINT('Ctrl Pts',(16.5025603830837,-3.1867248730455,4.00000000000001));
#31470=CARTESIAN_POINT('Ctrl Pts',(16.6238417013591,-2.31630255698834,12.));
#31471=CARTESIAN_POINT('Ctrl Pts',(15.4424463905558,-4.70128586413353,-12.));
#31472=CARTESIAN_POINT('Ctrl Pts',(15.6886051427755,-3.89272126189979,-3.99999999999999));
#31473=CARTESIAN_POINT('Ctrl Pts',(15.8711266308723,-3.06479193675307,3.99999999999999));
#31474=CARTESIAN_POINT('Ctrl Pts',(15.9877673893743,-2.22767439379039,12.));
#31475=CARTESIAN_POINT('Ctrl Pts',(14.8280677081537,-4.51424491597337,-12.));
#31476=CARTESIAN_POINT('Ctrl Pts',(15.0644330192291,-3.73784910632557,-4.));
#31477=CARTESIAN_POINT('Ctrl Pts',(15.2396928786609,-2.94285900046064,4.));
#31478=CARTESIAN_POINT('Ctrl Pts',(15.3516930773895,-2.13904623059243,12.));
#31479=CARTESIAN_POINT('',(14.8280677332334,-4.51424491927473,-11.9999999957355));
#31480=CARTESIAN_POINT('',(15.3044692038576,-4.65928020123585,-12.));
#31481=CARTESIAN_POINT('Ctrl Pts',(15.3516930767777,-2.13904623498331,11.9999999562994));
#31482=CARTESIAN_POINT('Ctrl Pts',(15.3237029275181,-2.33992852728642,10.0007056240913));
#31483=CARTESIAN_POINT('Ctrl Pts',(15.2917618106915,-2.54031911975201,8.00083387021915));
#31484=CARTESIAN_POINT('Ctrl Pts',(15.2558790213823,-2.74010132749604,5.99999995642121));
#31485=CARTESIAN_POINT('Ctrl Pts',(15.2200100350179,-2.9398066855075,3.9999356985046));
#31486=CARTESIAN_POINT('Ctrl Pts',(15.1802231246131,-3.13878875107566,2.00006422723888));
#31487=CARTESIAN_POINT('Ctrl Pts',(15.1365413257817,-3.33693222779593,2.22044604925032E-15));
#31488=CARTESIAN_POINT('Ctrl Pts',(15.0928595269503,-3.53507570451619,-2.00006422723888));
#31489=CARTESIAN_POINT('Ctrl Pts',(15.0452912745672,-3.73234233124902,-3.99993569850461));
#31490=CARTESIAN_POINT('Ctrl Pts',(14.9938641476362,-3.92861781320467,-5.99999995642121));
#31491=CARTESIAN_POINT('Ctrl Pts',(14.9424246385123,-4.12494055272706,-8.00054577305927));
#31492=CARTESIAN_POINT('Ctrl Pts',(14.8871467284008,-4.32018647843707,-10.0004173920443));
#31493=CARTESIAN_POINT('Ctrl Pts',(14.8280677289536,-4.51424492140107,-11.9999999914697));
#31494=CARTESIAN_POINT('Ctrl Pts',(15.5228520082561,-7.92019304563387,-10.5713320279724));
#31495=CARTESIAN_POINT('Ctrl Pts',(15.8881799221207,-7.20418383869531,-3.52377734265747));
#31496=CARTESIAN_POINT('Ctrl Pts',(16.20388659607,-6.46286199768348,3.52377734265748));
#31497=CARTESIAN_POINT('Ctrl Pts',(16.4669580190248,-5.70330482702815,10.5713320279724));
#31498=CARTESIAN_POINT('Ctrl Pts',(15.5231950610407,-7.92036478087607,-10.5713320279724));
#31499=CARTESIAN_POINT('Ctrl Pts',(15.8885308963887,-7.20433975023758,-3.52377734265747));
#31500=CARTESIAN_POINT('Ctrl Pts',(16.2042443952,-6.46300153666839,3.52377734265748));
#31501=CARTESIAN_POINT('Ctrl Pts',(16.4673214812396,-5.70342760090494,10.5713320279724));
#31502=CARTESIAN_POINT('Ctrl Pts',(15.5235381138555,-7.92053651613241,-10.5713320279724));
#31503=CARTESIAN_POINT('Ctrl Pts',(15.8888818706875,-7.20449566179256,-3.52377734265747));
#31504=CARTESIAN_POINT('Ctrl Pts',(16.2046021943615,-6.46314107566464,3.52377734265748));
#31505=CARTESIAN_POINT('Ctrl Pts',(16.4676849434863,-5.70355037479156,10.5713320279724));
#31506=CARTESIAN_POINT('Ctrl Pts',(15.5238811666727,-7.92070825138992,-10.5713320279724));
#31507=CARTESIAN_POINT('Ctrl Pts',(15.8892328449888,-7.20465157334867,-3.52377734265747));
#31508=CARTESIAN_POINT('Ctrl Pts',(16.2049599935256,-6.46328061466174,3.52377734265748));
#31509=CARTESIAN_POINT('Ctrl Pts',(16.4680484057355,-5.703673148679,10.5713320279724));
#31510=CARTESIAN_POINT('Ctrl Pts',(15.5228507477964,-7.92019248660846,-10.5713320134286));
#31511=CARTESIAN_POINT('Ctrl Pts',(15.8881669516022,-7.20417811498612,-3.52377733780954));
#31512=CARTESIAN_POINT('Ctrl Pts',(16.2038734814214,-6.462856612406,3.52377733780954));
#31513=CARTESIAN_POINT('Ctrl Pts',(16.466956742565,-5.70330430555752,10.5713320134286));
#31514=CARTESIAN_POINT('Ctrl Pts',(13.7402020358534,-7.17334281440039,-12.));
#31515=CARTESIAN_POINT('Ctrl Pts',(14.1157973873101,-6.45390751815578,-4.));
#31516=CARTESIAN_POINT('Ctrl Pts',(14.4347687202385,-5.70491981764189,4.));
#31517=CARTESIAN_POINT('Ctrl Pts',(14.6931953939549,-4.93558590585175,12.));
#31518=CARTESIAN_POINT('Ctrl Pts',(14.3095066403964,-7.4705594843989,-12.));
#31519=CARTESIAN_POINT('Ctrl Pts',(14.7006642203029,-6.72131546876617,-4.00000000000001));
#31520=CARTESIAN_POINT('Ctrl Pts',(15.0328516506424,-5.94129458944342,4.00000000000001));
#31521=CARTESIAN_POINT('Ctrl Pts',(15.3019858448814,-5.14008448418318,12.));
#31522=CARTESIAN_POINT('Ctrl Pts',(14.8788112449393,-7.76777615439741,-12.));
#31523=CARTESIAN_POINT('Ctrl Pts',(15.2855310532957,-6.98872341937657,-4.));
#31524=CARTESIAN_POINT('Ctrl Pts',(15.6309345810462,-6.17766936124495,4.));
#31525=CARTESIAN_POINT('Ctrl Pts',(15.9107762958078,-5.34458306251461,12.));
#31526=CARTESIAN_POINT('Ctrl Pts',(15.4481158494822,-8.06499282439593,-12.));
#31527=CARTESIAN_POINT('Ctrl Pts',(15.8703978862885,-7.25613136998697,-4.));
#31528=CARTESIAN_POINT('Ctrl Pts',(16.2290175114501,-6.41404413304648,4.));
#31529=CARTESIAN_POINT('Ctrl Pts',(16.5195667467343,-5.54908164084604,12.));
#31530=CARTESIAN_POINT('',(13.740202059893,-7.17334282227374,-11.9999999957355));
#31531=CARTESIAN_POINT('Ctrl Pts',(13.7402020552943,-7.1733428235737,-11.9999999914697));
#31532=CARTESIAN_POINT('Ctrl Pts',(13.8340813002562,-6.99352153777388,-10.0004173920443));
#31533=CARTESIAN_POINT('Ctrl Pts',(13.9244439127861,-6.81183164507366,-8.00054577305927));
#31534=CARTESIAN_POINT('Ctrl Pts',(14.0112327972984,-6.62837502710201,-5.9999999564212));
#31535=CARTESIAN_POINT('Ctrl Pts',(14.09800079054,-6.44496256964578,-3.99993569850461));
#31536=CARTESIAN_POINT('Ctrl Pts',(14.1811591229608,-6.25986380572143,-2.00006422723887));
#31537=CARTESIAN_POINT('Ctrl Pts',(14.2606595952488,-6.07318597677024,-2.22044604925031E-15));
#31538=CARTESIAN_POINT('Ctrl Pts',(14.3401600675367,-5.88650814781905,2.00006422723888));
#31539=CARTESIAN_POINT('Ctrl Pts',(14.4159873282975,-5.69828730098519,3.99993569850461));
#31540=CARTESIAN_POINT('Ctrl Pts',(14.4880974587037,-5.50863250063969,5.99999995642122));
#31541=CARTESIAN_POINT('Ctrl Pts',(14.5602353382114,-5.31890471817277,8.00083387021916));
#31542=CARTESIAN_POINT('Ctrl Pts',(14.6286115396895,-5.127851533001,10.0007056240913));
#31543=CARTESIAN_POINT('Ctrl Pts',(14.6931953925432,-4.93558591005429,11.9999999562994));
#31544=CARTESIAN_POINT('',(13.7402020549027,-7.17334282434542,-12.));
#31545=CARTESIAN_POINT('Origin',(2.22044604925031E-15,-4.16333634234434E-16,
-6.));
#31546=CARTESIAN_POINT('',(15.364994223987,-2.04131143860991,-11.9999999957355));
#31547=CARTESIAN_POINT('Origin',(2.22044604925031E-15,-4.16333634234434E-16,
-12.));
#31548=CARTESIAN_POINT('Ctrl Pts',(15.3649942201102,-2.04131144140431,-11.9999999914697));
#31549=CARTESIAN_POINT('Ctrl Pts',(15.3917093519036,-1.84022611326084,-10.0004173920443));
#31550=CARTESIAN_POINT('Ctrl Pts',(15.4144808289508,-1.63858762813028,-8.00054577305927));
#31551=CARTESIAN_POINT('Ctrl Pts',(15.4332898445205,-1.43651125126802,-5.99999995642121));
#31552=CARTESIAN_POINT('Ctrl Pts',(15.4520943325031,-1.23448351695164,-3.99993569850461));
#31553=CARTESIAN_POINT('Ctrl Pts',(15.466930098069,-1.03210574960204,-2.00006422723889));
#31554=CARTESIAN_POINT('Ctrl Pts',(15.4777885274135,-0.829495208345887,
-6.66133814775094E-15));
#31555=CARTESIAN_POINT('Ctrl Pts',(15.4886469567579,-0.626884667089731,
2.00006422723887));
#31556=CARTESIAN_POINT('Ctrl Pts',(15.495525953138,-0.42408047564849,3.99993569850462));
#31557=CARTESIAN_POINT('Ctrl Pts',(15.4984215485681,-0.22120014213042,5.99999995642122));
#31558=CARTESIAN_POINT('Ctrl Pts',(15.5013182582685,-0.0182417370997565,
8.00083387021916));
#31559=CARTESIAN_POINT('Ctrl Pts',(15.5002268324596,0.184675569413392,10.0007056240913));
#31560=CARTESIAN_POINT('Ctrl Pts',(15.4951570864913,0.387435135136788,11.9999999562994));
#31561=CARTESIAN_POINT('Origin',(2.22044604925031E-15,-4.16333634234434E-16,
-6.));
#31562=CARTESIAN_POINT('',(12.3898631351355,-9.31350049042594,-11.9999999957355));
#31563=CARTESIAN_POINT('Ctrl Pts',(13.6942758009489,-7.26063422894488,11.9999999562994));
#31564=CARTESIAN_POINT('Ctrl Pts',(13.5992678738299,-7.43982864180721,10.0007056240913));
#31565=CARTESIAN_POINT('Ctrl Pts',(13.500715422892,-7.617209697467,8.00083387021915));
#31566=CARTESIAN_POINT('Ctrl Pts',(13.3986670912385,-7.79267092710594,5.99999995642121));
#31567=CARTESIAN_POINT('Ctrl Pts',(13.2966580142668,-7.9680646625034,3.9999356985046));
#31568=CARTESIAN_POINT('Ctrl Pts',(13.1912146735706,-8.14143871638738,2.00006422723888));
#31569=CARTESIAN_POINT('Ctrl Pts',(13.0823981492392,-8.31269262422126,-4.44089209850063E-15));
#31570=CARTESIAN_POINT('Ctrl Pts',(12.9735816249078,-8.48394653205514,-2.00006422723888));
#31571=CARTESIAN_POINT('Ctrl Pts',(12.8614129292112,-8.65304722502548,-3.99993569850461));
#31572=CARTESIAN_POINT('Ctrl Pts',(12.7459570690561,-8.81989673373664,-5.99999995642121));
#31573=CARTESIAN_POINT('Ctrl Pts',(12.630473410406,-8.98678641507513,-8.00054577305927));
#31574=CARTESIAN_POINT('Ctrl Pts',(12.5117511266867,-9.15135141196428,-10.0004173920443));
#31575=CARTESIAN_POINT('Ctrl Pts',(12.3898631303866,-9.31350049096029,-11.9999999914697));
#31576=CARTESIAN_POINT('Origin',(2.22044604925031E-15,-4.16333634234434E-16,
-12.));
#31577=CARTESIAN_POINT('Ctrl Pts',(10.4581387236936,-11.4401631786859,-12.));
#31578=CARTESIAN_POINT('Ctrl Pts',(11.0571442669941,-10.8925763156096,-4.));
#31579=CARTESIAN_POINT('Ctrl Pts',(11.613048155468,-10.2978527213822,4.));
#31580=CARTESIAN_POINT('Ctrl Pts',(12.1190174885494,-9.66330244953633,12.));
#31581=CARTESIAN_POINT('Ctrl Pts',(10.8914559714904,-11.9141691326998,-12.));
#31582=CARTESIAN_POINT('Ctrl Pts',(11.5152804085056,-11.3438938315843,-4.00000000000001));
#31583=CARTESIAN_POINT('Ctrl Pts',(12.0942173384564,-10.7245287597614,4.00000000000001));
#31584=CARTESIAN_POINT('Ctrl Pts',(12.6211507498191,-10.0636868518367,12.));
#31585=CARTESIAN_POINT('Ctrl Pts',(11.3247732192872,-12.3881750867137,-12.));
#31586=CARTESIAN_POINT('Ctrl Pts',(11.9734165500172,-11.795211347559,-3.99999999999999));
#31587=CARTESIAN_POINT('Ctrl Pts',(12.5753865214448,-11.1512047981406,3.99999999999999));
#31588=CARTESIAN_POINT('Ctrl Pts',(13.1232840110888,-10.4640712541372,12.));
#31589=CARTESIAN_POINT('Ctrl Pts',(11.7580904670839,-12.8621810407276,-12.));
#31590=CARTESIAN_POINT('Ctrl Pts',(12.4315526915288,-12.2465288635337,-4.));
#31591=CARTESIAN_POINT('Ctrl Pts',(13.0565557044332,-11.5778808365199,4.));
#31592=CARTESIAN_POINT('Ctrl Pts',(13.6254172723585,-10.8644556564376,12.));
#31593=CARTESIAN_POINT('',(10.4581387435906,-11.4401631943065,-11.9999999957355));
#31594=CARTESIAN_POINT('Ctrl Pts',(10.4581387388246,-11.4401631939552,-11.9999999914697));
#31595=CARTESIAN_POINT('Ctrl Pts',(10.6078588745025,-11.303295051446,-10.0004173920443));
#31596=CARTESIAN_POINT('Ctrl Pts',(10.7549135578339,-11.163468233693,-8.00054577305927));
#31597=CARTESIAN_POINT('Ctrl Pts',(10.8992142909491,-11.0207589502706,-5.99999995642121));
#31598=CARTESIAN_POINT('Ctrl Pts',(11.0434802889055,-10.8780840189234,-3.99993569850461));
#31599=CARTESIAN_POINT('Ctrl Pts',(11.184931066005,-10.7325899011204,-2.00006422723888));
#31600=CARTESIAN_POINT('Ctrl Pts',(11.3234846509767,-10.584360885717,0.));
#31601=CARTESIAN_POINT('Ctrl Pts',(11.4620382359483,-10.4361318703137,2.00006422723888));
#31602=CARTESIAN_POINT('Ctrl Pts',(11.5976678743505,-10.2851965800591,3.9999356985046));
#31603=CARTESIAN_POINT('Ctrl Pts',(11.7302949937737,-10.1316424808146,5.99999995642121));
#31604=CARTESIAN_POINT('Ctrl Pts',(11.8629731501784,-9.97802929156078,8.00083387021915));
#31605=CARTESIAN_POINT('Ctrl Pts',(11.99256979992,-9.82188406150686,10.0007056240913));
#31606=CARTESIAN_POINT('Ctrl Pts',(12.1190174857855,-9.66330245300261,11.9999999562994));
#31607=CARTESIAN_POINT('',(10.4581387381927,-11.4401631945464,-12.));
#31608=CARTESIAN_POINT('Ctrl Pts',(11.8778429311088,-12.7516740731249,-10.5713320220547));
#31609=CARTESIAN_POINT('Ctrl Pts',(12.466019210595,-12.2037861517057,-3.52377734068488));
#31610=CARTESIAN_POINT('Ctrl Pts',(13.0162331940139,-11.6151497981962,3.52377734068489));
#31611=CARTESIAN_POINT('Ctrl Pts',(13.5232327823929,-10.9913838744951,10.5713320220547));
#31612=CARTESIAN_POINT('Ctrl Pts',(13.9299291396692,-10.4711731300928,-12.));
#31613=CARTESIAN_POINT('Ctrl Pts',(14.4781984826686,-9.74180374592263,-4.));
#31614=CARTESIAN_POINT('Ctrl Pts',(14.9690602353605,-8.96929245803532,4.));
#31615=CARTESIAN_POINT('Ctrl Pts',(15.3964809635174,-8.1631345999333,12.));
#31616=CARTESIAN_POINT('Ctrl Pts',(13.4165737973453,-10.0852822463105,-12.));
#31617=CARTESIAN_POINT('Ctrl Pts',(13.9446379409184,-9.38279208500909,-4.00000000000001));
#31618=CARTESIAN_POINT('Ctrl Pts',(14.4174101182391,-8.63874991513855,4.00000000000001));
#31619=CARTESIAN_POINT('Ctrl Pts',(14.8290792433535,-7.86230114163155,12.));
#31620=CARTESIAN_POINT('Ctrl Pts',(12.9032184550213,-9.6993913625282,-12.));
#31621=CARTESIAN_POINT('Ctrl Pts',(13.4110773991682,-9.02378042409555,-4.));
#31622=CARTESIAN_POINT('Ctrl Pts',(13.8657600011178,-8.30820737224178,4.));
#31623=CARTESIAN_POINT('Ctrl Pts',(14.2616775231895,-7.56146768332979,12.));
#31624=CARTESIAN_POINT('Ctrl Pts',(12.3898631126974,-9.3135004787459,-12.));
#31625=CARTESIAN_POINT('Ctrl Pts',(12.877516857418,-8.66476876318201,-4.));
#31626=CARTESIAN_POINT('Ctrl Pts',(13.3141098839964,-7.977664829345,4.));
#31627=CARTESIAN_POINT('Ctrl Pts',(13.6942758030256,-7.26063422502805,12.));
#31628=CARTESIAN_POINT('',(12.787929093689,-9.61272797390185,-12.));
#31629=CARTESIAN_POINT('Ctrl Pts',(11.8778439250753,-12.7516750288689,-10.5713320279724));
#31630=CARTESIAN_POINT('Ctrl Pts',(12.4660294414806,-12.2037959661548,-3.52377734265748));
#31631=CARTESIAN_POINT('Ctrl Pts',(13.0162436756369,-11.6151593444016,3.52377734265748));
#31632=CARTESIAN_POINT('Ctrl Pts',(13.5232338028988,-10.9913848018556,10.5713320279724));
#31633=CARTESIAN_POINT('Ctrl Pts',(11.878107552328,-12.7519537381656,-10.5713320279724));
#31634=CARTESIAN_POINT('Ctrl Pts',(12.4663059245166,-12.2040625153446,-3.52377734265747));
#31635=CARTESIAN_POINT('Ctrl Pts',(13.0165321716897,-11.6154128426606,3.52377734265748));
#31636=CARTESIAN_POINT('Ctrl Pts',(13.523533354515,-10.9916244829556,10.5713320279724));
#31637=CARTESIAN_POINT('Ctrl Pts',(11.8783711796043,-12.7522324474859,-10.5713320279724));
#31638=CARTESIAN_POINT('Ctrl Pts',(12.4665824075774,-12.2043290645569,-3.52377734265747));
#31639=CARTESIAN_POINT('Ctrl Pts',(13.0168206677681,-11.615666340941,3.52377734265748));
#31640=CARTESIAN_POINT('Ctrl Pts',(13.5238329061577,-10.9918641640757,10.5713320279724));
#31641=CARTESIAN_POINT('Ctrl Pts',(11.8786348068824,-12.7525111568082,-10.5713320279724));
#31642=CARTESIAN_POINT('Ctrl Pts',(12.46685889064,-12.2045956137711,-3.52377734265748));
#31643=CARTESIAN_POINT('Ctrl Pts',(13.0171091638486,-11.6159198392231,3.52377734265748));
#31644=CARTESIAN_POINT('Ctrl Pts',(13.5241324578026,-10.9921038451975,10.5713320279724));
#31645=CARTESIAN_POINT('Ctrl Pts',(9.50849948587549,-14.604000482186,-12.));
#31646=CARTESIAN_POINT('Ctrl Pts',(10.2731631630064,-14.1061366133278,-4.));
#31647=CARTESIAN_POINT('Ctrl Pts',(10.998636751241,-13.548098063635,4.));
#31648=CARTESIAN_POINT('Ctrl Pts',(11.6760030816321,-12.9367439718926,12.));
#31649=CARTESIAN_POINT('Ctrl Pts',(9.15808571423198,-14.0658037985085,-12.));
#31650=CARTESIAN_POINT('Ctrl Pts',(9.89456947890248,-13.5862875518289,-3.99999999999999));
#31651=CARTESIAN_POINT('Ctrl Pts',(10.5933074148231,-13.0488142230957,3.99999999999998));
#31652=CARTESIAN_POINT('Ctrl Pts',(11.2457109746983,-12.4599901733872,12.));
#31653=CARTESIAN_POINT('Ctrl Pts',(8.80767194258846,-13.5276071148311,-12.));
#31654=CARTESIAN_POINT('Ctrl Pts',(9.5159757947985,-13.0664384903301,-4.00000000000001));
#31655=CARTESIAN_POINT('Ctrl Pts',(10.1879780784053,-12.5495303825563,4.00000000000001));
#31656=CARTESIAN_POINT('Ctrl Pts',(10.8154188677646,-11.9832363748819,12.));
#31657=CARTESIAN_POINT('Ctrl Pts',(8.45725817094494,-12.9894104311537,-12.));
#31658=CARTESIAN_POINT('Ctrl Pts',(9.13738211069453,-12.5465894288312,-4.));
#31659=CARTESIAN_POINT('Ctrl Pts',(9.78264874198742,-12.0502465420169,4.));
#31660=CARTESIAN_POINT('Ctrl Pts',(10.3851267608308,-11.5064825763765,12.));
#31661=CARTESIAN_POINT('',(8.45725818803503,-12.9894104498036,-11.9999999957355));
#31662=CARTESIAN_POINT('',(8.72897600508842,-13.4067388841598,-12.));
#31663=CARTESIAN_POINT('Ctrl Pts',(10.3851267575397,-11.5064825793469,11.9999999562994));
#31664=CARTESIAN_POINT('Ctrl Pts',(10.2345604107395,-11.6423756219493,10.0007056240913));
#31665=CARTESIAN_POINT('Ctrl Pts',(10.0812835057528,-11.7753523676252,8.00083387021916));
#31666=CARTESIAN_POINT('Ctrl Pts',(9.92537816662527,-11.9053294053327,5.99999995642122));
#31667=CARTESIAN_POINT('Ctrl Pts',(9.76953279922271,-12.0352564450914,3.99993569850462));
#31668=CARTESIAN_POINT('Ctrl Pts',(9.61115105130115,-12.1621110176642,2.00006422723887));
#31669=CARTESIAN_POINT('Ctrl Pts',(9.45032468026494,-12.2858196078884,-6.66133814958239E-15));
#31670=CARTESIAN_POINT('Ctrl Pts',(9.28949830922873,-12.4095281981127,-2.00006422723888));
#31671=CARTESIAN_POINT('Ctrl Pts',(9.1262583703532,-12.5300669180878,-3.9999356985046));
#31672=CARTESIAN_POINT('Ctrl Pts',(8.9606994576558,-12.6473659403674,-5.9999999564212));
#31673=CARTESIAN_POINT('Ctrl Pts',(8.79510068306996,-12.7646932049232,-8.00054577305927));
#31674=CARTESIAN_POINT('Ctrl Pts',(8.62725368531363,-12.878728305646,-10.0004173920443));
#31675=CARTESIAN_POINT('Ctrl Pts',(8.45725818338972,-12.9894104486815,-11.9999999914697));
#31676=CARTESIAN_POINT('Ctrl Pts',(5.91466953576707,-14.3271310247952,-12.));
#31677=CARTESIAN_POINT('Ctrl Pts',(6.66483636200898,-14.0174396520956,-4.));
#31678=CARTESIAN_POINT('Ctrl Pts',(7.39062259281096,-13.648712606804,4.));
#31679=CARTESIAN_POINT('Ctrl Pts',(8.08310721637552,-13.2254821026516,12.));
#31680=CARTESIAN_POINT('Ctrl Pts',(6.1597349716519,-14.9207541491876,-12.));
#31681=CARTESIAN_POINT('Ctrl Pts',(6.94098383200368,-14.5982311802709,-4.00000000000002));
#31682=CARTESIAN_POINT('Ctrl Pts',(7.69684192361464,-14.2142264844647,4.00000000000002));
#31683=CARTESIAN_POINT('Ctrl Pts',(8.41801860598166,-13.7734600609591,12.));
#31684=CARTESIAN_POINT('Ctrl Pts',(6.40480040753673,-15.51437727358,-12.));
#31685=CARTESIAN_POINT('Ctrl Pts',(7.21713130199838,-15.1790227084462,-3.99999999999999));
#31686=CARTESIAN_POINT('Ctrl Pts',(8.00306125441832,-14.7797403621254,3.99999999999999));
#31687=CARTESIAN_POINT('Ctrl Pts',(8.75292999558781,-14.3214380192667,12.));
#31688=CARTESIAN_POINT('Ctrl Pts',(6.64986584342156,-16.1080003979724,-12.));
#31689=CARTESIAN_POINT('Ctrl Pts',(7.49327877199308,-15.7598142366215,-4.));
#31690=CARTESIAN_POINT('Ctrl Pts',(8.30928058522199,-15.3452542397861,4.));
#31691=CARTESIAN_POINT('Ctrl Pts',(9.08784138519396,-14.8694159775742,12.));
#31692=CARTESIAN_POINT('',(5.91466954912158,-14.3271310462789,-11.9999999957355));
#31693=CARTESIAN_POINT('Ctrl Pts',(5.91466954476316,-14.3271310443187,-11.9999999914697));
#31694=CARTESIAN_POINT('Ctrl Pts',(6.10217211316044,-14.2497243630455,-10.0004173920443));
#31695=CARTESIAN_POINT('Ctrl Pts',(6.28818190218767,-14.1686257980847,-8.00054577305927));
#31696=CARTESIAN_POINT('Ctrl Pts',(6.47258968583999,-14.0838766949572,-5.99999995642121));
#31697=CARTESIAN_POINT('Ctrl Pts',(6.65695308001832,-13.9991479920971,-3.99993569850461));
#31698=CARTESIAN_POINT('Ctrl Pts',(6.83963525048719,-13.910807258287,-2.00006422723888));
#31699=CARTESIAN_POINT('Ctrl Pts',(7.02053034096174,-13.8189056633163,-6.66133814775094E-15));
#31700=CARTESIAN_POINT('Ctrl Pts',(7.20142543143629,-13.7270040683457,2.00006422723887));
#31701=CARTESIAN_POINT('Ctrl Pts',(7.38049851140845,-13.6315593582429,3.9999356985046));
#31702=CARTESIAN_POINT('Ctrl Pts',(7.55764583187841,-13.5326268506854,5.99999995642121));
#31703=CARTESIAN_POINT('Ctrl Pts',(7.7348613213967,-13.4336562723579,8.00083387021915));
#31704=CARTESIAN_POINT('Ctrl Pts',(7.91004715080014,-13.3312524166245,10.0007056240913));
#31705=CARTESIAN_POINT('Ctrl Pts',(8.08310721259279,-13.2254821049635,11.9999999562994));
#31706=CARTESIAN_POINT('',(5.9146695439671,-14.3271310446582,-12.));
#31707=CARTESIAN_POINT('Ctrl Pts',(6.8001919590846,-16.04511557088,-10.5713320220547));
#31708=CARTESIAN_POINT('Ctrl Pts',(7.54028557404929,-15.7314374695154,-3.52377734068488));
#31709=CARTESIAN_POINT('Ctrl Pts',(8.25864308411528,-15.3664844972649,3.52377734068489));
#31710=CARTESIAN_POINT('Ctrl Pts',(8.94840736668245,-14.9537403335486,10.5713320220547));
#31711=CARTESIAN_POINT('Ctrl Pts',(6.80019256622394,-16.0451168089422,-10.5713320279724));
#31712=CARTESIAN_POINT('Ctrl Pts',(7.54029183119773,-15.7314501912497,-3.52377734265748));
#31713=CARTESIAN_POINT('Ctrl Pts',(8.25864966862457,-15.3664970526898,3.52377734265747));
#31714=CARTESIAN_POINT('Ctrl Pts',(8.94840800846834,-14.9537415540161,10.5713320279724));
#31715=CARTESIAN_POINT('Ctrl Pts',(6.80034497061742,-16.0454688758496,-10.5713320279724));
#31716=CARTESIAN_POINT('Ctrl Pts',(7.54046047507781,-15.731795228331,-3.52377734265747));
#31717=CARTESIAN_POINT('Ctrl Pts',(8.25883406472935,-15.3668339346014,3.52377734265747));
#31718=CARTESIAN_POINT('Ctrl Pts',(8.94860751915148,-14.9540692332704,10.5713320279724));
#31719=CARTESIAN_POINT('Ctrl Pts',(6.80049737502495,-16.0458209427872,-10.5713320279724));
#31720=CARTESIAN_POINT('Ctrl Pts',(7.54062911897337,-15.732140265442,-3.52377734265749));
#31721=CARTESIAN_POINT('Ctrl Pts',(8.25901846085091,-15.3671708165418,3.52377734265748));
#31722=CARTESIAN_POINT('Ctrl Pts',(8.94880702985273,-14.9543969125528,10.5713320279724));
#31723=CARTESIAN_POINT('Ctrl Pts',(6.80064977943359,-16.0461730097273,-10.5713320279724));
#31724=CARTESIAN_POINT('Ctrl Pts',(7.54079776287007,-15.7324853025553,-3.52377734265748));
#31725=CARTESIAN_POINT('Ctrl Pts',(8.25920285697386,-15.3675076984845,3.52377734265747));
#31726=CARTESIAN_POINT('Ctrl Pts',(8.94900654055539,-14.9547245918374,10.5713320279724));
#31727=CARTESIAN_POINT('Origin',(2.22044604925031E-15,-4.16333634234434E-16,
-12.));
#31728=CARTESIAN_POINT('Origin',(2.22044604925031E-15,-4.16333634234434E-16,
-12.));
#31729=CARTESIAN_POINT('',(3.50458308761994,-15.0986058056538,-11.9999999957355));
#31730=CARTESIAN_POINT('Origin',(2.22044604925031E-15,-4.16333634234434E-16,
-12.));
#31731=CARTESIAN_POINT('',(3.61717958430867,-15.5836992225952,-12.));
#31732=CARTESIAN_POINT('',(0.65780391580271,-15.4860354481354,-11.9999999957355));
#31733=CARTESIAN_POINT('',(0.657803911513399,-15.4860354448496,-12.));
#31734=CARTESIAN_POINT('',(-1.87079645529993,-15.3866864696526,-11.9999999957355));
#31735=CARTESIAN_POINT('Origin',(2.22044604925031E-15,-4.16333634234434E-16,
-12.));
#31736=CARTESIAN_POINT('',(-1.93090207822381,-15.8810354438797,-12.));
#31737=CARTESIAN_POINT('',(-4.67840257791378,-14.7770954254049,-11.9999999957355));
#31738=CARTESIAN_POINT('',(-4.67840258082059,-14.7770954208502,-12.));
#31739=CARTESIAN_POINT('',(-7.02053033569551,-13.8189056621041,-11.9999999957355));
#31740=CARTESIAN_POINT('Origin',(2.22044604925031E-15,-4.16333634234434E-16,
-12.));
#31741=CARTESIAN_POINT('',(-7.24608845304286,-14.2628844115113,-12.));
#31742=CARTESIAN_POINT('',(-9.45032467486545,-12.285819607669,-11.9999999957355));
#31743=CARTESIAN_POINT('',(-9.45032467603913,-12.2858196023947,-12.));
#31744=CARTESIAN_POINT('',(-11.3234846456134,-10.5843608863791,-11.9999999957355));
#31745=CARTESIAN_POINT('Origin',(2.22044604925031E-15,-4.16333634234434E-16,
-12.));
#31746=CARTESIAN_POINT('',(-11.6872896195489,-10.9244190213593,-12.));
#31747=CARTESIAN_POINT('',(-13.0823981440903,-8.31269262586177,-11.9999999957355));
#31748=CARTESIAN_POINT('',(-13.0823981433893,-8.31269262050417,-12.));
#31749=CARTESIAN_POINT('',(-14.2606595904354,-6.07318597922667,-11.9999999957355));
#31750=CARTESIAN_POINT('Origin',(2.22044604925031E-15,-4.16333634234434E-16,
-12.));
#31751=CARTESIAN_POINT('',(-14.7188311719128,-6.26830746997787,-12.));
#31752=CARTESIAN_POINT('',(-15.1365413215044,-3.33693223109852,-11.9999999957355));
#31753=CARTESIAN_POINT('',(-15.1365413190133,-3.33693222630378,-12.));
#31754=CARTESIAN_POINT('',(-15.4777885237305,-0.829495212300453,-11.9999999957355));
#31755=CARTESIAN_POINT('Origin',(2.22044604925031E-15,-4.16333634234434E-16,
-12.));
#31756=CARTESIAN_POINT('',(-15.9750644581313,-0.856145527351446,-12.));
#31757=CARTESIAN_POINT('',(-15.364994223987,2.04131143860991,-11.9999999957355));
#31758=CARTESIAN_POINT('',(-15.3649942200062,2.04131144226347,-12.));
#31759=CARTESIAN_POINT('',(-14.8280677332333,4.51424491927474,-11.9999999957355));
#31760=CARTESIAN_POINT('Origin',(2.22044604925031E-15,-4.16333634234434E-16,
-12.));
#31761=CARTESIAN_POINT('',(-15.3044692038576,4.65928020123584,-12.));
#31762=CARTESIAN_POINT('',(-13.740202059893,7.17334282227373,-11.9999999957355));
#31763=CARTESIAN_POINT('',(-13.7402020549027,7.17334282434542,-12.));
#31764=CARTESIAN_POINT('',(-12.3898631351355,9.31350049042594,-11.9999999957355));
#31765=CARTESIAN_POINT('Origin',(2.22044604925031E-15,-4.16333634234434E-16,
-12.));
#31766=CARTESIAN_POINT('',(-12.787929093689,9.61272797390186,-12.));
#31767=CARTESIAN_POINT('',(-10.4581387435906,11.4401631943064,-11.9999999957355));
#31768=CARTESIAN_POINT('',(-10.4581387381927,11.4401631945464,-12.));
#31769=CARTESIAN_POINT('',(-8.45725818803502,12.9894104498036,-11.9999999957355));
#31770=CARTESIAN_POINT('Origin',(2.22044604925031E-15,-4.16333634234434E-16,
-12.));
#31771=CARTESIAN_POINT('',(-8.72897600508841,13.4067388841599,-12.));
#31772=CARTESIAN_POINT('',(-5.91466954912156,14.3271310462789,-11.9999999957355));
#31773=CARTESIAN_POINT('',(-5.91466954396709,14.3271310446582,-12.));
#31774=CARTESIAN_POINT('',(-3.50458308761994,15.0986058056538,-11.9999999957355));
#31775=CARTESIAN_POINT('Origin',(2.22044604925031E-15,-4.16333634234434E-16,
-12.));
#31776=CARTESIAN_POINT('',(-3.61717958430867,15.5836992225952,-12.));
#31777=CARTESIAN_POINT('',(-0.657803915802711,15.4860354481354,-11.9999999957355));
#31778=CARTESIAN_POINT('',(-0.6578039115134,15.4860354448496,-12.));
#31779=CARTESIAN_POINT('',(1.87079645529994,15.3866864696526,-11.9999999957355));
#31780=CARTESIAN_POINT('Origin',(2.22044604925031E-15,-4.16333634234434E-16,
-12.));
#31781=CARTESIAN_POINT('',(1.93090207822382,15.8810354438797,-12.));
#31782=CARTESIAN_POINT('',(4.67840257791379,14.7770954254049,-11.9999999957355));
#31783=CARTESIAN_POINT('',(4.6784025808206,14.7770954208502,-12.));
#31784=CARTESIAN_POINT('',(7.02053033569551,13.8189056621041,-11.9999999957355));
#31785=CARTESIAN_POINT('Origin',(2.22044604925031E-15,-4.16333634234434E-16,
-12.));
#31786=CARTESIAN_POINT('',(7.24608845304286,14.2628844115113,-12.));
#31787=CARTESIAN_POINT('',(9.45032467486545,12.285819607669,-11.9999999957355));
#31788=CARTESIAN_POINT('',(9.45032467603913,12.2858196023947,-12.));
#31789=CARTESIAN_POINT('',(11.3234846456134,10.5843608863791,-11.9999999957355));
#31790=CARTESIAN_POINT('Origin',(2.22044604925031E-15,-4.16333634234434E-16,
-12.));
#31791=CARTESIAN_POINT('',(11.6872896195489,10.9244190213593,-12.));
#31792=CARTESIAN_POINT('',(13.0823981440903,8.31269262586177,-11.9999999957355));
#31793=CARTESIAN_POINT('',(13.0823981433893,8.31269262050417,-12.));
#31794=CARTESIAN_POINT('',(14.2606595904354,6.07318597922668,-11.9999999957355));
#31795=CARTESIAN_POINT('Origin',(2.22044604925031E-15,-4.16333634234434E-16,
-12.));
#31796=CARTESIAN_POINT('',(14.7188311719128,6.26830746997787,-12.));
#31797=CARTESIAN_POINT('',(15.1365413215044,3.33693223109852,-11.9999999957355));
#31798=CARTESIAN_POINT('',(15.1365413190133,3.33693222630378,-12.));
#31799=CARTESIAN_POINT('',(15.4777885237305,0.829495212300455,-11.9999999957355));
#31800=CARTESIAN_POINT('Origin',(2.22044604925031E-15,-4.16333634234434E-16,
-12.));
#31801=CARTESIAN_POINT('',(15.9750644581313,0.856145527351446,-12.));
#31802=CARTESIAN_POINT('',(15.3649942200062,-2.04131144226347,-12.));
#31803=CARTESIAN_POINT('Origin',(2.22044604925031E-15,-4.16333634234434E-16,
-6.));
#31804=CARTESIAN_POINT('Ctrl Pts',(5.82337815902385,-14.3644793130828,11.9999999562994));
#31805=CARTESIAN_POINT('Ctrl Pts',(5.63541391608915,-14.4406802789199,10.0007056240913));
#31806=CARTESIAN_POINT('Ctrl Pts',(5.44590001392117,-14.5132137565555,8.00083387021915));
#31807=CARTESIAN_POINT('Ctrl Pts',(5.25494215213615,-14.5820294533272,5.99999995642121));
#31808=CARTESIAN_POINT('Ctrl Pts',(5.06405774564414,-14.6508186789333,3.9999356985046));
#31809=CARTESIAN_POINT('Ctrl Pts',(4.87184076676219,-14.7158532365687,2.00006422723887));
#31810=CARTESIAN_POINT('Ctrl Pts',(4.67840258291259,-14.7770954274579,-2.22044604925031E-15));
#31811=CARTESIAN_POINT('Ctrl Pts',(4.48496439906298,-14.8383376183471,-2.00006422723887));
#31812=CARTESIAN_POINT('Ctrl Pts',(4.29034236280191,-14.895775616736,-3.99993569850461));
#31813=CARTESIAN_POINT('Ctrl Pts',(4.0946492458228,-14.949376159348,-5.99999995642121));
#31814=CARTESIAN_POINT('Ctrl Pts',(3.89890901149391,-15.0029896074497,-8.00054577305927));
#31815=CARTESIAN_POINT('Ctrl Pts',(3.70218212478788,-15.05274049588,-10.0004173920443));
#31816=CARTESIAN_POINT('Ctrl Pts',(3.50458308363856,-15.0986058030105,-11.9999999914697));
#31817=CARTESIAN_POINT('Ctrl Pts',(3.94020446357842,-16.9753698440352,-12.));
#31818=CARTESIAN_POINT('Ctrl Pts',(4.82903275014493,-16.7690612207615,-4.));
#31819=CARTESIAN_POINT('Ctrl Pts',(5.70161535233114,-16.4928030941281,4.));
#31820=CARTESIAN_POINT('Ctrl Pts',(6.54722690864904,-16.1499910948348,12.));
#31821=CARTESIAN_POINT('Ctrl Pts',(3.794997335032,-16.3497818234513,-12.));
#31822=CARTESIAN_POINT('Ctrl Pts',(4.65106990943784,-16.1510762276491,-3.99999999999999));
#31823=CARTESIAN_POINT('Ctrl Pts',(5.49149549661271,-15.8849989557599,3.99999999999999));
#31824=CARTESIAN_POINT('Ctrl Pts',(6.30594399347681,-15.5548205003623,12.));
#31825=CARTESIAN_POINT('Ctrl Pts',(3.64979020648557,-15.7241938028674,-12.));
#31826=CARTESIAN_POINT('Ctrl Pts',(4.47310706873074,-15.5330912345367,-4.00000000000001));
#31827=CARTESIAN_POINT('Ctrl Pts',(5.28137564089428,-15.2771948173917,4.00000000000001));
#31828=CARTESIAN_POINT('Ctrl Pts',(6.06466107830459,-14.9596499058898,12.));
#31829=CARTESIAN_POINT('Ctrl Pts',(3.50458307793915,-15.0986057822834,-12.));
#31830=CARTESIAN_POINT('Ctrl Pts',(4.29514422802365,-14.9151062414243,-4.));
#31831=CARTESIAN_POINT('Ctrl Pts',(5.07125578517585,-14.6693906790234,4.));
#31832=CARTESIAN_POINT('Ctrl Pts',(5.82337816313236,-14.3644793114172,12.));
#31833=CARTESIAN_POINT('Ctrl Pts',(0.902337623732299,-17.403280701153,-10.5713320279724));
#31834=CARTESIAN_POINT('Ctrl Pts',(1.70508374321692,-17.361659351802,-3.52377734265747));
#31835=CARTESIAN_POINT('Ctrl Pts',(2.50494062688806,-17.2644084310805,3.52377734265748));
#31836=CARTESIAN_POINT('Ctrl Pts',(3.29427214377962,-17.1124563810414,10.5713320279724));
#31837=CARTESIAN_POINT('Ctrl Pts',(0.902360423042107,-17.4036636612004,
-10.5713320279724));
#31838=CARTESIAN_POINT('Ctrl Pts',(1.70512420699455,-17.3620412602053,-3.52377734265748));
#31839=CARTESIAN_POINT('Ctrl Pts',(2.50499868214735,-17.264788063709,3.52377734265749));
#31840=CARTESIAN_POINT('Ctrl Pts',(3.29434754959081,-17.1128325354912,10.5713320279724));
#31841=CARTESIAN_POINT('Ctrl Pts',(0.902383222354776,-17.404046621281,-10.5713320279724));
#31842=CARTESIAN_POINT('Ctrl Pts',(1.70516467077662,-17.3624231686417,-3.52377734265746));
#31843=CARTESIAN_POINT('Ctrl Pts',(2.50505673741252,-17.2651676963705,3.52377734265747));
#31844=CARTESIAN_POINT('Ctrl Pts',(3.29442295540941,-17.1132086899734,10.5713320279724));
#31845=CARTESIAN_POINT('Ctrl Pts',(0.902406021667647,-17.4044295813643,
-10.5713320279724));
#31846=CARTESIAN_POINT('Ctrl Pts',(1.70520513455892,-17.3628050770807,-3.52377734265747));
#31847=CARTESIAN_POINT('Ctrl Pts',(2.50511479267822,-17.2655473290345,3.52377734265748));
#31848=CARTESIAN_POINT('Ctrl Pts',(3.29449836122858,-17.1135848444583,10.5713320279724));
#31849=CARTESIAN_POINT('Ctrl Pts',(0.902337477632692,-17.4032793300502,
-10.5713320134286));
#31850=CARTESIAN_POINT('Ctrl Pts',(1.70508221483526,-17.361645257149,-3.52377733780954));
#31851=CARTESIAN_POINT('Ctrl Pts',(2.50493873335086,-17.2643943808229,3.52377733780954));
#31852=CARTESIAN_POINT('Ctrl Pts',(3.29427195715649,-17.1124550148594,10.5713320134286));
#31853=CARTESIAN_POINT('Ctrl Pts',(0.657803910601427,-15.4860354233799,
-12.));
#31854=CARTESIAN_POINT('Ctrl Pts',(1.46865082925679,-15.4515928911625,-4.));
#31855=CARTESIAN_POINT('Ctrl Pts',(2.2767788714881,-15.3533363183005,4.));
#31856=CARTESIAN_POINT('Ctrl Pts',(3.07225491994942,-15.1924734268593,12.));
#31857=CARTESIAN_POINT('Ctrl Pts',(0.685059026225968,-16.1276760084048,
-12.));
#31858=CARTESIAN_POINT('Ctrl Pts',(1.52950216735065,-16.0918064016704,-4.00000000000001));
#31859=CARTESIAN_POINT('Ctrl Pts',(2.37111377949615,-15.9894787155008,4.));
#31860=CARTESIAN_POINT('Ctrl Pts',(3.19954918153982,-15.8219507121087,12.));
#31861=CARTESIAN_POINT('Ctrl Pts',(0.712314141850509,-16.7693165934297,
-12.));
#31862=CARTESIAN_POINT('Ctrl Pts',(1.59035350544451,-16.7320199121783,-4.));
#31863=CARTESIAN_POINT('Ctrl Pts',(2.4654486875042,-16.6256211127012,3.99999999999999));
#31864=CARTESIAN_POINT('Ctrl Pts',(3.32684344313023,-16.4514279973581,12.));
#31865=CARTESIAN_POINT('Ctrl Pts',(0.739569257475051,-17.4109571784546,
-12.));
#31866=CARTESIAN_POINT('Ctrl Pts',(1.65120484353838,-17.3722334226862,-4.));
#31867=CARTESIAN_POINT('Ctrl Pts',(2.55978359551225,-17.2617635099015,4.));
#31868=CARTESIAN_POINT('Ctrl Pts',(3.45413770472063,-17.0809052826075,12.));
#31869=CARTESIAN_POINT('Ctrl Pts',(0.657803912377566,-15.4860354448028,
-11.9999999914697));
#31870=CARTESIAN_POINT('Ctrl Pts',(0.860473336502315,-15.4774266129281,
-10.0004173920443));
#31871=CARTESIAN_POINT('Ctrl Pts',(1.06300270545654,-15.4648379845811,-8.00054577305927));
#31872=CARTESIAN_POINT('Ctrl Pts',(1.26527523936852,-15.4482710543491,-5.99999995642121));
#31873=CARTESIAN_POINT('Ctrl Pts',(1.46749908351692,-15.4317081120036,-3.99993569850461));
#31874=CARTESIAN_POINT('Ctrl Pts',(1.66937848149492,-15.4111759584542,-2.00006422723887));
#31875=CARTESIAN_POINT('Ctrl Pts',(1.87079645983396,-15.3866864725929,2.22030256658689E-15));
#31876=CARTESIAN_POINT('Ctrl Pts',(2.072214438173,-15.3621969867316,2.00006422723887));
#31877=CARTESIAN_POINT('Ctrl Pts',(2.2731321034333,-15.3337548974327,3.9999356985046));
#31878=CARTESIAN_POINT('Ctrl Pts',(2.47343304368529,-15.301376702062,5.99999995642121));
#31879=CARTESIAN_POINT('Ctrl Pts',(2.67381106285918,-15.2689860470573,8.00083387021915));
#31880=CARTESIAN_POINT('Ctrl Pts',(2.87345607543091,-15.2326749819658,10.0007056240913));
#31881=CARTESIAN_POINT('Ctrl Pts',(3.07225491560408,-15.192473427738,11.9999999562994));
#31882=CARTESIAN_POINT('Origin',(2.22044604925031E-15,-4.16333634234434E-16,
-6.));
#31883=CARTESIAN_POINT('Origin',(2.22044604925031E-15,-4.16333634234434E-16,
-6.));
#31884=CARTESIAN_POINT('Ctrl Pts',(0.559244210621348,-15.4899078445247,
11.9999999562994));
#31885=CARTESIAN_POINT('Ctrl Pts',(0.356553333306836,-15.4972257725099,
10.0007056240913));
#31886=CARTESIAN_POINT('Ctrl Pts',(0.15366060748641,-15.5005673742223,8.00083387021916));
#31887=CARTESIAN_POINT('Ctrl Pts',(-0.0493174405869348,-15.499921541416,
5.99999995642122));
#31888=CARTESIAN_POINT('Ctrl Pts',(-0.252217409591645,-15.4992759570407,
3.99993569850462));
#31889=CARTESIAN_POINT('Ctrl Pts',(-0.455085414960348,-15.4946463722799,
2.00006422723889));
#31890=CARTESIAN_POINT('Ctrl Pts',(-0.657803911807544,-15.4860354517744,
8.88178419700125E-15));
#31891=CARTESIAN_POINT('Ctrl Pts',(-0.86052240865474,-15.4774245312688,
-2.00006422723887));
#31892=CARTESIAN_POINT('Ctrl Pts',(-1.06305225241292,-15.4648339377712,
-3.99993569850461));
#31893=CARTESIAN_POINT('Ctrl Pts',(-1.26527609564326,-15.4482709842168,
-5.99999995642121));
#31894=CARTESIAN_POINT('Ctrl Pts',(-1.46754862863696,-15.4317040427731,
-8.00054577305927));
#31895=CARTESIAN_POINT('Ctrl Pts',(-1.66942723837632,-15.4111700275214,
-10.0004173920443));
#31896=CARTESIAN_POINT('Ctrl Pts',(-1.87079645813715,-15.3866864658071,
-11.9999999914697));
#31897=CARTESIAN_POINT('Ctrl Pts',(-4.6784025743345,-14.7770954003634,-12.));
#31898=CARTESIAN_POINT('Ctrl Pts',(-3.90467566848155,-15.0220559863311,
-4.));
#31899=CARTESIAN_POINT('Ctrl Pts',(-3.11167798341368,-15.2061210786984,
4.));
#31900=CARTESIAN_POINT('Ctrl Pts',(-2.30915666147617,-15.3270282387598,
12.));
#31901=CARTESIAN_POINT('Ctrl Pts',(-4.87224514815724,-15.3893621218603,
-12.));
#31902=CARTESIAN_POINT('Ctrl Pts',(-4.06646003173275,-15.6444722812593,
-4.));
#31903=CARTESIAN_POINT('Ctrl Pts',(-3.240605680342,-15.8361638338742,4.));
#31904=CARTESIAN_POINT('Ctrl Pts',(-2.40483309451253,-15.9620806002547,
12.));
#31905=CARTESIAN_POINT('Ctrl Pts',(-5.06608772197997,-16.0016288433572,
-12.));
#31906=CARTESIAN_POINT('Ctrl Pts',(-4.22824439498395,-16.2668885761874,
-4.00000000000001));
#31907=CARTESIAN_POINT('Ctrl Pts',(-3.36953337727031,-16.4662065890499,
4.00000000000001));
#31908=CARTESIAN_POINT('Ctrl Pts',(-2.50050952754889,-16.5971329617496,
12.));
#31909=CARTESIAN_POINT('Ctrl Pts',(-5.2599302958027,-16.6138955648541,-12.));
#31910=CARTESIAN_POINT('Ctrl Pts',(-4.39002875823514,-16.8893048711156,
-4.));
#31911=CARTESIAN_POINT('Ctrl Pts',(-3.49846107419862,-17.0962493442257,
4.));
#31912=CARTESIAN_POINT('Ctrl Pts',(-2.59618596058525,-17.2321853232445,
12.));
#31913=CARTESIAN_POINT('Ctrl Pts',(-4.67840257999253,-14.7770954211018,
-11.9999999914697));
#31914=CARTESIAN_POINT('Ctrl Pts',(-4.48501122377192,-14.8383227908024,
-10.0004173920443));
#31915=CARTESIAN_POINT('Ctrl Pts',(-4.29039030580172,-14.8957624734364,
-8.00054577305927));
#31916=CARTESIAN_POINT('Ctrl Pts',(-4.09465007444454,-14.9493759323877,
-5.99999995642121));
#31917=CARTESIAN_POINT('Ctrl Pts',(-3.89895696043642,-15.0029764858466,
-3.99993569850461));
#31918=CARTESIAN_POINT('Ctrl Pts',(-3.70222996976806,-15.0527293932983,
-2.00006422723888));
#31919=CARTESIAN_POINT('Ctrl Pts',(-3.50458308436497,-15.0986058099674,
-6.66133814775094E-15));
#31920=CARTESIAN_POINT('Ctrl Pts',(-3.30693619896188,-15.1444822266366,
2.00006422723887));
#31921=CARTESIAN_POINT('Ctrl Pts',(-3.10840758407278,-15.1864732938717,
3.99993569850461));
#31922=CARTESIAN_POINT('Ctrl Pts',(-2.90911227356018,-15.2245546989007,
5.99999995642122));
#31923=CARTESIAN_POINT('Ctrl Pts',(-2.70974027110768,-15.2626507582476,
8.00083387021915));
#31924=CARTESIAN_POINT('Ctrl Pts',(-2.50971621033041,-15.2968121341423,
10.0007056240913));
#31925=CARTESIAN_POINT('Ctrl Pts',(-2.30915666586,-15.3270282380994,11.9999999562994));
#31926=CARTESIAN_POINT('Ctrl Pts',(-5.10435222255114,-16.6623507570641,
-10.5713320220547));
#31927=CARTESIAN_POINT('Ctrl Pts',(-4.33577922443239,-16.8977823962929,
-3.52377734068488));
#31928=CARTESIAN_POINT('Ctrl Pts',(-3.55089819699268,-17.0799635066964,
3.52377734068489));
#31929=CARTESIAN_POINT('Ctrl Pts',(-2.7572012668629,-17.2071550680903,10.5713320220547));
#31930=CARTESIAN_POINT('Ctrl Pts',(-2.1033373682508,-17.299259072917,-12.));
#31931=CARTESIAN_POINT('Ctrl Pts',(-1.19755028131709,-17.4093895599857,
-4.));
#31932=CARTESIAN_POINT('Ctrl Pts',(-0.283105004950502,-17.4482326636193,
4.));
#31933=CARTESIAN_POINT('Ctrl Pts',(0.628758543704759,-17.4153109432562,
12.));
#31934=CARTESIAN_POINT('Ctrl Pts',(-2.02582373096845,-16.6617348634049,
-12.));
#31935=CARTESIAN_POINT('Ctrl Pts',(-1.15341733358622,-16.7678067459162,
-4.));
#31936=CARTESIAN_POINT('Ctrl Pts',(-0.272671824331076,-16.8052183767432,
4.));
#31937=CARTESIAN_POINT('Ctrl Pts',(0.605587100820427,-16.7735099102924,
12.));
#31938=CARTESIAN_POINT('Ctrl Pts',(-1.94831009368611,-16.0242106538928,
-12.));
#31939=CARTESIAN_POINT('Ctrl Pts',(-1.10928438585536,-16.1262239318468,
-4.));
#31940=CARTESIAN_POINT('Ctrl Pts',(-0.262238643711649,-16.162204089867,
4.));
#31941=CARTESIAN_POINT('Ctrl Pts',(0.582415657936094,-16.1317088773286,
12.));
#31942=CARTESIAN_POINT('Ctrl Pts',(-1.87079645640376,-15.3866864443807,
-12.));
#31943=CARTESIAN_POINT('Ctrl Pts',(-1.0651514381245,-15.4846411177773,-4.));
#31944=CARTESIAN_POINT('Ctrl Pts',(-0.251805463092223,-15.5191898029909,
4.));
#31945=CARTESIAN_POINT('Ctrl Pts',(0.559244215051762,-15.4899078443647,
12.));
#31946=CARTESIAN_POINT('Ctrl Pts',(-5.10435255326646,-16.6623520957364,
-10.5713320279724));
#31947=CARTESIAN_POINT('Ctrl Pts',(-4.33578260855181,-16.8977961637243,
-3.52377734265748));
#31948=CARTESIAN_POINT('Ctrl Pts',(-3.5509012234375,-17.0799773571509,3.52377734265748));
#31949=CARTESIAN_POINT('Ctrl Pts',(-2.75720155972776,-17.2071564155546,
10.5713320279724));
#31950=CARTESIAN_POINT('Ctrl Pts',(-5.10446210897357,-16.6627197582901,
-10.5713320279724));
#31951=CARTESIAN_POINT('Ctrl Pts',(-4.33587520540538,-16.8981688796597,
-3.52377734265747));
#31952=CARTESIAN_POINT('Ctrl Pts',(-3.55097651134477,-17.0803539511987,
3.52377734265748));
#31953=CARTESIAN_POINT('Ctrl Pts',(-2.75725935384223,-17.2075356754217,
10.5713320279724));
#31954=CARTESIAN_POINT('Ctrl Pts',(-5.10457166468936,-16.6630874208762,
-10.5713320279724));
#31955=CARTESIAN_POINT('Ctrl Pts',(-4.33596780226611,-16.8985415956278,
-3.52377734265748));
#31956=CARTESIAN_POINT('Ctrl Pts',(-3.55105179925777,-17.0807305452794,
3.52377734265749));
#31957=CARTESIAN_POINT('Ctrl Pts',(-2.75731714796086,-17.2079149353218,
10.5713320279724));
#31958=CARTESIAN_POINT('Ctrl Pts',(-5.10468122040586,-16.6634550834647,
-10.5713320279724));
#31959=CARTESIAN_POINT('Ctrl Pts',(-4.33606039912753,-16.8989143115984,
-3.52377734265748));
#31960=CARTESIAN_POINT('Ctrl Pts',(-3.55112708717115,-17.0811071393627,
3.52377734265748));
#31961=CARTESIAN_POINT('Ctrl Pts',(-2.75737494207985,-17.2082941952246,
10.5713320279724));
#31962=CARTESIAN_POINT('Ctrl Pts',(-7.89318567151549,-15.5366023477324,
-12.));
#31963=CARTESIAN_POINT('Ctrl Pts',(-7.07969107489246,-15.94988858305,-4.));
#31964=CARTESIAN_POINT('Ctrl Pts',(-6.23367872045025,-16.2991478653893,
4.));
#31965=CARTESIAN_POINT('Ctrl Pts',(-5.36554738109814,-16.5800872693051,
12.));
#31966=CARTESIAN_POINT('Ctrl Pts',(-7.60230055704008,-14.9640367778145,
-12.));
#31967=CARTESIAN_POINT('Ctrl Pts',(-6.81878542355292,-15.3620923041542,
-3.99999999999999));
#31968=CARTESIAN_POINT('Ctrl Pts',(-6.00395089905301,-15.6984804428827,
3.99999999999999));
#31969=CARTESIAN_POINT('Ctrl Pts',(-5.16781253370865,-15.9690664743998,
12.));
#31970=CARTESIAN_POINT('Ctrl Pts',(-7.31141544256466,-14.3914712078966,
-12.));
#31971=CARTESIAN_POINT('Ctrl Pts',(-6.55787977221338,-14.7742960252583,
-4.00000000000001));
#31972=CARTESIAN_POINT('Ctrl Pts',(-5.77422307765577,-15.0978130203761,
4.00000000000001));
#31973=CARTESIAN_POINT('Ctrl Pts',(-4.97007768631916,-15.3580456794946,
12.));
#31974=CARTESIAN_POINT('Ctrl Pts',(-7.02053032808925,-13.8189056379787,
-12.));
#31975=CARTESIAN_POINT('Ctrl Pts',(-6.29697412087384,-14.1864997463625,
-4.));
#31976=CARTESIAN_POINT('Ctrl Pts',(-5.54449525625854,-14.4971455978694,
4.));
#31977=CARTESIAN_POINT('Ctrl Pts',(-4.77234283892968,-14.7470248845893,
12.));
#31978=CARTESIAN_POINT('Ctrl Pts',(-4.77234284314764,-14.7470248832244,
11.9999999562994));
#31979=CARTESIAN_POINT('Ctrl Pts',(-4.96531284363905,-14.6845771232416,
10.0007056240913));
#31980=CARTESIAN_POINT('Ctrl Pts',(-5.15711253600029,-14.6183238025476,
8.00083387021916));
#31981=CARTESIAN_POINT('Ctrl Pts',(-5.34762862212736,-14.5482943371312,
5.99999995642122));
#31982=CARTESIAN_POINT('Ctrl Pts',(-5.53807142289819,-14.4782918097778,
3.99993569850462));
#31983=CARTESIAN_POINT('Ctrl Pts',(-5.72712157929328,-14.4045564788684,
2.00006422723887));
#31984=CARTESIAN_POINT('Ctrl Pts',(-5.91466954661191,-14.3271310510647,
-2.22044604925031E-15));
#31985=CARTESIAN_POINT('Ctrl Pts',(-6.10221751393055,-14.249705623261,-2.00006422723887));
#31986=CARTESIAN_POINT('Ctrl Pts',(-6.28822707700645,-14.1686050492701,
-3.99993569850461));
#31987=CARTESIAN_POINT('Ctrl Pts',(-6.47259046648839,-14.0838763361911,
-5.9999999564212));
#31988=CARTESIAN_POINT('Ctrl Pts',(-6.6569982454432,-13.9991272228421,-8.00054577305927));
#31989=CARTESIAN_POINT('Ctrl Pts',(-6.83967903847032,-13.9107850091975,
-10.0004173920443));
#31990=CARTESIAN_POINT('Ctrl Pts',(-7.02053033704636,-13.8189056575201,
-11.9999999914697));
#31991=CARTESIAN_POINT('Ctrl Pts',(-9.4503246629373,-12.2858195853618,-12.));
#31992=CARTESIAN_POINT('Ctrl Pts',(-8.8070406537256,-12.7806374276138,-4.));
#31993=CARTESIAN_POINT('Ctrl Pts',(-8.12482055003974,-13.2248232185595,
4.));
#31994=CARTESIAN_POINT('Ctrl Pts',(-7.41204987000498,-13.6129172422203,
12.));
#31995=CARTESIAN_POINT('Ctrl Pts',(-9.84188465099258,-12.7948640406237,
-12.));
#31996=CARTESIAN_POINT('Ctrl Pts',(-9.17194713643085,-13.3101839159077,
-3.99999999999999));
#31997=CARTESIAN_POINT('Ctrl Pts',(-8.4614602688847,-13.7727738769957,3.99999999999998));
#31998=CARTESIAN_POINT('Ctrl Pts',(-7.71915700781015,-14.1769479927898,
12.));
#31999=CARTESIAN_POINT('Ctrl Pts',(-10.2334446390479,-13.3039084958857,
-12.));
#32000=CARTESIAN_POINT('Ctrl Pts',(-9.53685361913611,-13.8397304042016,
-4.00000000000001));
#32001=CARTESIAN_POINT('Ctrl Pts',(-8.79809998772967,-14.3207245354319,
4.00000000000001));
#32002=CARTESIAN_POINT('Ctrl Pts',(-8.02626414561533,-14.7409787433592,
12.));
#32003=CARTESIAN_POINT('Ctrl Pts',(-10.6250046271031,-13.8129529511477,
-12.));
#32004=CARTESIAN_POINT('Ctrl Pts',(-9.90176010184136,-14.3692768924954,
-4.));
#32005=CARTESIAN_POINT('Ctrl Pts',(-9.13473970657464,-14.8686751938681,
4.));
#32006=CARTESIAN_POINT('Ctrl Pts',(-8.3333712834205,-15.3050094939286,12.));
#32007=CARTESIAN_POINT('Ctrl Pts',(-9.45032467534708,-12.2858196029144,
-11.9999999914697));
#32008=CARTESIAN_POINT('Ctrl Pts',(-9.28953723874319,-12.4094982497846,
-10.0004173920443));
#32009=CARTESIAN_POINT('Ctrl Pts',(-9.12629892676312,-12.5300381699545,
-8.00054577305927));
#32010=CARTESIAN_POINT('Ctrl Pts',(-8.96070015868055,-12.6473654436892,
-5.99999995642121));
#32011=CARTESIAN_POINT('Ctrl Pts',(-8.79514125248487,-12.7646644751455,
-3.99993569850461));
#32012=CARTESIAN_POINT('Ctrl Pts',(-8.62729484758191,-12.8787015086849,
-2.00006422723887));
#32013=CARTESIAN_POINT('Ctrl Pts',(-8.45725818645174,-12.9894104549704,
4.4407486176685E-15));
#32014=CARTESIAN_POINT('Ctrl Pts',(-8.28722152532158,-13.1001194012559,
2.00006422723889));
#32015=CARTESIAN_POINT('Ctrl Pts',(-8.11502744172963,-13.2074788825944,
3.9999356985046));
#32016=CARTESIAN_POINT('Ctrl Pts',(-7.94077571668976,-13.311426708555,5.99999995642122));
#32017=CARTESIAN_POINT('Ctrl Pts',(-7.76645693687179,-13.4154145352581,
8.00083387021915));
#32018=CARTESIAN_POINT('Ctrl Pts',(-7.59017968165941,-13.5159279860378,
10.0007056240913));
#32019=CARTESIAN_POINT('Ctrl Pts',(-7.41204987389855,-13.6129172401003,
11.9999999562994));
#32020=CARTESIAN_POINT('Ctrl Pts',(-10.4953817114971,-13.9116967726179,
-10.5713320220547));
#32021=CARTESIAN_POINT('Ctrl Pts',(-9.85368169962205,-14.3957975936737,
-3.52377734068489));
#32022=CARTESIAN_POINT('Ctrl Pts',(-9.17844439943352,-14.8354369602649,
3.52377734068489));
#32023=CARTESIAN_POINT('Ctrl Pts',(-8.47611532710788,-15.2264182697331,
10.5713320220547));
#32024=CARTESIAN_POINT('Ctrl Pts',(-10.4953824801207,-13.9116979174471,
-10.5713320279724));
#32025=CARTESIAN_POINT('Ctrl Pts',(-9.85368958839295,-14.3958093733904,
-3.52377734265748));
#32026=CARTESIAN_POINT('Ctrl Pts',(-9.17845198049581,-14.8354489403297,
3.52377734265748));
#32027=CARTESIAN_POINT('Ctrl Pts',(-8.47611606317077,-15.2264194357697,
10.5713320279724));
#32028=CARTESIAN_POINT('Ctrl Pts',(-10.4956111768096,-13.9120059369772,
-10.5713320279724));
#32029=CARTESIAN_POINT('Ctrl Pts',(-9.85390407733061,-14.3961279418154,
-3.52377734265748));
#32030=CARTESIAN_POINT('Ctrl Pts',(-9.17865153073689,-14.8357770729966,
3.52377734265749));
#32031=CARTESIAN_POINT('Ctrl Pts',(-8.47630008638775,-15.2267560567168,
10.5713320279724));
#32032=CARTESIAN_POINT('Ctrl Pts',(-10.4958398735176,-13.9123139565346,
-10.5713320279724));
#32033=CARTESIAN_POINT('Ctrl Pts',(-9.85411856628614,-14.3964465102686,
-3.52377734265747));
#32034=CARTESIAN_POINT('Ctrl Pts',(-9.17885108099462,-14.8361052056924,
3.52377734265747));
#32035=CARTESIAN_POINT('Ctrl Pts',(-8.47648410961995,-15.2270926776936,
10.5713320279724));
#32036=CARTESIAN_POINT('Ctrl Pts',(-10.4960685702272,-13.9126219760941,
-10.5713320279724));
#32037=CARTESIAN_POINT('Ctrl Pts',(-9.85433305524321,-14.396765078724,-3.52377734265748));
#32038=CARTESIAN_POINT('Ctrl Pts',(-9.17905063125361,-14.8364333383906,
3.52377734265748));
#32039=CARTESIAN_POINT('Ctrl Pts',(-8.4766681328534,-15.2274292986728,10.5713320279724));
#32040=CARTESIAN_POINT('Origin',(2.22044604925031E-15,-4.16333634234434E-16,
-6.));
#32041=CARTESIAN_POINT('Ctrl Pts',(-9.52831491775384,-12.2254330780995,
11.9999999562994));
#32042=CARTESIAN_POINT('Ctrl Pts',(-9.68828901142903,-12.1007517516335,
10.0007056240913));
#32043=CARTESIAN_POINT('Ctrl Pts',(-9.84586179677031,-11.9728946368036,
8.00083387021915));
#32044=CARTESIAN_POINT('Ctrl Pts',(-10.0009368692462,-11.8419281258312,
5.99999995642122));
#32045=CARTESIAN_POINT('Ctrl Pts',(-10.1559522893738,-11.7110119934259,
3.99993569850463));
#32046=CARTESIAN_POINT('Ctrl Pts',(-10.3083823578508,-11.577064485493,2.00006422723886));
#32047=CARTESIAN_POINT('Ctrl Pts',(-10.4581387428691,-11.440163199662,-2.22058953008229E-15));
#32048=CARTESIAN_POINT('Ctrl Pts',(-10.6078951278873,-11.3032619138309,
-2.00006422723889));
#32049=CARTESIAN_POINT('Ctrl Pts',(-10.7549489117653,-11.1634332854871,
-3.9999356985046));
#32050=CARTESIAN_POINT('Ctrl Pts',(-10.8992149018134,-11.0207583461433,
-5.99999995642121));
#32051=CARTESIAN_POINT('Ctrl Pts',(-11.0435156270184,-10.8780490547226,
-8.00054577305927));
#32052=CARTESIAN_POINT('Ctrl Pts',(-11.1849646036129,-10.732554017443,-10.0004173920443));
#32053=CARTESIAN_POINT('Ctrl Pts',(-11.323484645315,-10.5843608816095,-11.9999999914697));
#32054=CARTESIAN_POINT('Ctrl Pts',(-12.7309992917815,-11.9000020835813,
-12.));
#32055=CARTESIAN_POINT('Ctrl Pts',(-12.1079166397235,-12.5665956477133,
-4.));
#32056=CARTESIAN_POINT('Ctrl Pts',(-11.432378782964,-13.1841452847902,4.));
#32057=CARTESIAN_POINT('Ctrl Pts',(-10.7126891046949,-13.7450603746485,
12.));
#32058=CARTESIAN_POINT('Ctrl Pts',(-12.2618277379259,-11.4614550111576,
-12.));
#32059=CARTESIAN_POINT('Ctrl Pts',(-11.6617073568841,-12.1034828101751,
-4.00000000000001));
#32060=CARTESIAN_POINT('Ctrl Pts',(-11.011064886471,-12.6982740827144,4.00000000000001));
#32061=CARTESIAN_POINT('Ctrl Pts',(-10.3178977078823,-13.238517943374,12.));
#32062=CARTESIAN_POINT('Ctrl Pts',(-11.7926561840702,-11.0229079387338,
-12.));
#32063=CARTESIAN_POINT('Ctrl Pts',(-11.2154980740448,-11.6403699726369,
-4.));
#32064=CARTESIAN_POINT('Ctrl Pts',(-10.589750989978,-12.2124028806386,3.99999999999999));
#32065=CARTESIAN_POINT('Ctrl Pts',(-9.92310631106972,-12.7319755120994,
12.));
#32066=CARTESIAN_POINT('Ctrl Pts',(-11.3234846302145,-10.5843608663101,
-12.));
#32067=CARTESIAN_POINT('Ctrl Pts',(-10.7692887912054,-11.1772571350987,
-4.));
#32068=CARTESIAN_POINT('Ctrl Pts',(-10.168437093485,-11.7265316785628,4.));
#32069=CARTESIAN_POINT('Ctrl Pts',(-9.52831491425713,-12.2254330808248,
12.));
#32070=CARTESIAN_POINT('Ctrl Pts',(-14.6205143845238,-9.48308765551918,
-10.5713320279724));
#32071=CARTESIAN_POINT('Ctrl Pts',(-14.1830961789038,-10.1574755131067,
-3.52377734265747));
#32072=CARTESIAN_POINT('Ctrl Pts',(-13.6989459691819,-10.801546433397,3.52377734265748));
#32073=CARTESIAN_POINT('Ctrl Pts',(-13.1726858752452,-11.4091515540133,
10.5713320279724));
#32074=CARTESIAN_POINT('Ctrl Pts',(-14.6208346379921,-9.48329888032005,
-10.5713320279724));
#32075=CARTESIAN_POINT('Ctrl Pts',(-14.1834066893878,-10.1577015099631,
-3.52377734265748));
#32076=CARTESIAN_POINT('Ctrl Pts',(-13.6992457130466,-10.8017865270358,
3.52377734265748));
#32077=CARTESIAN_POINT('Ctrl Pts',(-13.172973931643,-11.4094049345811,10.5713320279724));
#32078=CARTESIAN_POINT('Ctrl Pts',(-14.6211548914877,-9.48351010514003,
-10.5713320279724));
#32079=CARTESIAN_POINT('Ctrl Pts',(-14.1837171998983,-10.1579275068399,
-3.52377734265746));
#32080=CARTESIAN_POINT('Ctrl Pts',(-13.6995454569368,-10.8020266206961,
3.52377734265747));
#32081=CARTESIAN_POINT('Ctrl Pts',(-13.1732619880652,-11.4096583151716,
10.5713320279724));
#32082=CARTESIAN_POINT('Ctrl Pts',(-14.6214751449855,-9.4837213299615,-10.5713320279724));
#32083=CARTESIAN_POINT('Ctrl Pts',(-14.1840277104109,-10.1581535037183,
-3.52377734265747));
#32084=CARTESIAN_POINT('Ctrl Pts',(-13.6998452008291,-10.8022667143581,
3.52377734265748));
#32085=CARTESIAN_POINT('Ctrl Pts',(-13.1735500444894,-11.4099116957638,
10.5713320279724));
#32086=CARTESIAN_POINT('Ctrl Pts',(-14.6205132701638,-9.4830868434418,-10.5713320134286));
#32087=CARTESIAN_POINT('Ctrl Pts',(-14.1830847367669,-10.1574671421628,
-3.52377733780954));
#32088=CARTESIAN_POINT('Ctrl Pts',(-13.6989347480705,-10.8015377684169,
3.52377733780955));
#32089=CARTESIAN_POINT('Ctrl Pts',(-13.1726847854084,-11.4091507093019,
10.5713320134286));
#32090=CARTESIAN_POINT('Ctrl Pts',(-13.082398125252,-8.31269260897955,-12.));
#32091=CARTESIAN_POINT('Ctrl Pts',(-12.6471465580533,-8.99768537300669,
-4.));
#32092=CARTESIAN_POINT('Ctrl Pts',(-12.1579898487504,-9.64841650065859,
4.));
#32093=CARTESIAN_POINT('Ctrl Pts',(-11.6209404740055,-10.2568875210076,
12.));
#32094=CARTESIAN_POINT('Ctrl Pts',(-13.6244476141704,-8.65711652400593,
-12.));
#32095=CARTESIAN_POINT('Ctrl Pts',(-13.1711620529523,-9.37049093290421,
-3.99999999999999));
#32096=CARTESIAN_POINT('Ctrl Pts',(-12.6617378711462,-10.0481841260574,
3.99999999999998));
#32097=CARTESIAN_POINT('Ctrl Pts',(-12.1024366633415,-10.6818662279256,
12.));
#32098=CARTESIAN_POINT('Ctrl Pts',(-14.1664971030888,-9.00154043903231,
-12.));
#32099=CARTESIAN_POINT('Ctrl Pts',(-13.6951775478512,-9.74329649280173,
-4.00000000000001));
#32100=CARTESIAN_POINT('Ctrl Pts',(-13.165485893542,-10.4479517514562,4.00000000000001));
#32101=CARTESIAN_POINT('Ctrl Pts',(-12.5839328526776,-11.1068449348435,
12.));
#32102=CARTESIAN_POINT('Ctrl Pts',(-14.7085465920072,-9.34596435405869,
-12.));
#32103=CARTESIAN_POINT('Ctrl Pts',(-14.2191930427501,-10.1161020526992,
-4.));
#32104=CARTESIAN_POINT('Ctrl Pts',(-13.6692339159378,-10.847719376855,4.));
#32105=CARTESIAN_POINT('Ctrl Pts',(-13.0654290420136,-11.5318236417615,
12.));
#32106=CARTESIAN_POINT('Ctrl Pts',(-13.0823981429167,-8.31269262122918,
-11.9999999914697));
#32107=CARTESIAN_POINT('Ctrl Pts',(-12.9736079637539,-8.48390507515421,
-10.0004173920443));
#32108=CARTESIAN_POINT('Ctrl Pts',(-12.8614412073296,-8.65300633950755,
-8.00054577305927));
#32109=CARTESIAN_POINT('Ctrl Pts',(-12.7459575579299,-8.81989602724713,
-5.9999999564212));
#32110=CARTESIAN_POINT('Ctrl Pts',(-12.630501707023,-8.98674554235783,-3.99993569850462));
#32111=CARTESIAN_POINT('Ctrl Pts',(-12.5117806414659,-9.1513121527328,-2.00006422723887));
#32112=CARTESIAN_POINT('Ctrl Pts',(-12.3898631354148,-9.31350049582264,
-6.66148162858282E-15));
#32113=CARTESIAN_POINT('Ctrl Pts',(-12.2679456293637,-9.47568883891247,
2.00006422723888));
#32114=CARTESIAN_POINT('Ctrl Pts',(-12.1428552248642,-9.63546759644758,
3.99993569850459));
#32115=CARTESIAN_POINT('Ctrl Pts',(-12.0146644150184,-9.79274420142234,
5.99999995642121));
#32116=CARTESIAN_POINT('Ctrl Pts',(-11.8864242753522,-9.95008132888459,
8.00083387021915));
#32117=CARTESIAN_POINT('Ctrl Pts',(-11.7551554642586,-10.1048234489648,
10.0007056240913));
#32118=CARTESIAN_POINT('Ctrl Pts',(-11.6209404769392,-10.2568875176838,
11.9999999562994));
#32119=CARTESIAN_POINT('Origin',(2.22044604925031E-15,-4.16333634234434E-16,
-6.));
#32120=CARTESIAN_POINT('Origin',(2.22044604925031E-15,-4.16333634234434E-16,
-6.));
#32121=CARTESIAN_POINT('Ctrl Pts',(-13.1350315903275,-8.22927361557979,
11.9999999562994));
#32122=CARTESIAN_POINT('Ctrl Pts',(-13.2427145405231,-8.05739713070269,
10.0007056240913));
#32123=CARTESIAN_POINT('Ctrl Pts',(-13.3470548154056,-7.88335767675537,
8.00083387021915));
#32124=CARTESIAN_POINT('Ctrl Pts',(-13.4479845318255,-7.70725061431012,
5.99999995642121));
#32125=CARTESIAN_POINT('Ctrl Pts',(-13.5488754238585,-7.53121129453728,
3.9999356985046));
#32126=CARTESIAN_POINT('Ctrl Pts',(-13.646300088531,-7.35320765589251,2.00006422723887));
#32127=CARTESIAN_POINT('Ctrl Pts',(-13.7402020610468,-7.17334282755303,
-2.22058953191374E-15));
#32128=CARTESIAN_POINT('Ctrl Pts',(-13.8341040335625,-6.99347799921355,
-2.00006422723888));
#32129=CARTESIAN_POINT('Ctrl Pts',(-13.9244651816241,-6.81178671274575,
-3.9999356985046));
#32130=CARTESIAN_POINT('Ctrl Pts',(-14.0112331646994,-6.6283742504801,-5.99999995642121));
#32131=CARTESIAN_POINT('Ctrl Pts',(-14.0980220390429,-6.44491762769787,
-8.00054577305927));
#32132=CARTESIAN_POINT('Ctrl Pts',(-14.1811783650629,-6.25981861555704,
-10.0004173920443));
#32133=CARTESIAN_POINT('Ctrl Pts',(-14.2606595885237,-6.0731859748468,-11.9999999914697));
#32134=CARTESIAN_POINT('Ctrl Pts',(-15.1365412980281,-3.33693222167749,
-12.));
#32135=CARTESIAN_POINT('Ctrl Pts',(-14.9618199354756,-4.12947967072155,
-4.));
#32136=CARTESIAN_POINT('Ctrl Pts',(-14.7247261388817,-4.90826835731623,
4.));
#32137=CARTESIAN_POINT('Ctrl Pts',(-14.4281741500255,-5.66372578922348,
12.));
#32138=CARTESIAN_POINT('Ctrl Pts',(-15.7637011196476,-3.4751929891605,-12.));
#32139=CARTESIAN_POINT('Ctrl Pts',(-15.5817404402384,-4.300578449675,-4.00000000000001));
#32140=CARTESIAN_POINT('Ctrl Pts',(-15.3348230187984,-5.11163507411277,
4.00000000000001));
#32141=CARTESIAN_POINT('Ctrl Pts',(-15.0259838443316,-5.89839374841795,
12.));
#32142=CARTESIAN_POINT('Ctrl Pts',(-16.3908609412671,-3.61345375664351,
-12.));
#32143=CARTESIAN_POINT('Ctrl Pts',(-16.2016609450012,-4.47167722862845,
-4.));
#32144=CARTESIAN_POINT('Ctrl Pts',(-15.9449198987151,-5.3150017909093,3.99999999999999));
#32145=CARTESIAN_POINT('Ctrl Pts',(-15.6237935386376,-6.13306170761243,
12.));
#32146=CARTESIAN_POINT('Ctrl Pts',(-17.0180207628866,-3.75171452412652,
-12.));
#32147=CARTESIAN_POINT('Ctrl Pts',(-16.8215814497639,-4.64277600758191,
-4.));
#32148=CARTESIAN_POINT('Ctrl Pts',(-16.5550167786318,-5.51836850770584,
4.));
#32149=CARTESIAN_POINT('Ctrl Pts',(-16.2216032329437,-6.36772966680691,
12.));
#32150=CARTESIAN_POINT('Ctrl Pts',(-15.1365413188172,-3.33693222714671,
-11.9999999914697));
#32151=CARTESIAN_POINT('Ctrl Pts',(-15.0928700982745,-3.53502773935638,
-10.0004173920443));
#32152=CARTESIAN_POINT('Ctrl Pts',(-15.0453038636357,-3.73229423974341,
-8.00054577305927));
#32153=CARTESIAN_POINT('Ctrl Pts',(-14.9938643653936,-3.92861698211701,
-5.99999995642121));
#32154=CARTESIAN_POINT('Ctrl Pts',(-14.9424372493419,-4.12489246692319,
-3.99993569850461));
#32155=CARTESIAN_POINT('Ctrl Pts',(-14.8871610357731,-4.32013949217793,
-2.00006422723887));
#32156=CARTESIAN_POINT('Ctrl Pts',(-14.8280677353416,-4.51424492425044,
8.88178419516979E-15));
#32157=CARTESIAN_POINT('Ctrl Pts',(-14.7689744349101,-4.70835035632295,
2.00006422723889));
#32158=CARTESIAN_POINT('Ctrl Pts',(-14.7060754584233,-4.90127671381264,
3.9999356985046));
#32159=CARTESIAN_POINT('Ctrl Pts',(-14.6394072673339,-5.09291221808617,
5.9999999564212));
#32160=CARTESIAN_POINT('Ctrl Pts',(-14.5727134212861,-5.28462146668684,
8.00083387021915));
#32161=CARTESIAN_POINT('Ctrl Pts',(-14.5022860102504,-5.47492807263538,
10.0007056240913));
#32162=CARTESIAN_POINT('Ctrl Pts',(-14.4281741516455,-5.66372578509675,
11.9999999562994));
#32163=CARTESIAN_POINT('Ctrl Pts',(-16.9821951536599,-3.91067668393918,
-10.5713320220547));
#32164=CARTESIAN_POINT('Ctrl Pts',(-16.8017984350274,-4.69399624458723,
-3.52377734068488));
#32165=CARTESIAN_POINT('Ctrl Pts',(-16.5671313910066,-5.46481370850019,
3.52377734068489));
#32166=CARTESIAN_POINT('Ctrl Pts',(-16.2804340492558,-6.21577119359523,
10.5713320220547));
#32167=CARTESIAN_POINT('Ctrl Pts',(-16.03326650792,-6.82808594282421,-12.));
#32168=CARTESIAN_POINT('Ctrl Pts',(-15.6757487639857,-7.66758581406302,
-4.));
#32169=CARTESIAN_POINT('Ctrl Pts',(-15.252165240311,-8.478940205584,4.));
#32170=CARTESIAN_POINT('Ctrl Pts',(-14.7677224198127,-9.25217634332294,
12.));
#32171=CARTESIAN_POINT('Ctrl Pts',(-15.4423975283137,-6.57645261709439,
-12.));
#32172=CARTESIAN_POINT('Ctrl Pts',(-15.0980552745046,-7.38501466090712,
-4.00000000000001));
#32173=CARTESIAN_POINT('Ctrl Pts',(-14.6900819425702,-8.16646846160462,
4.));
#32174=CARTESIAN_POINT('Ctrl Pts',(-14.223492142533,-8.91120876866085,12.));
#32175=CARTESIAN_POINT('Ctrl Pts',(-14.8515285487074,-6.32481929136457,
-12.));
#32176=CARTESIAN_POINT('Ctrl Pts',(-14.5203617850235,-7.10244350775121,
-4.));
#32177=CARTESIAN_POINT('Ctrl Pts',(-14.1279986448294,-7.85399671762523,
3.99999999999999));
#32178=CARTESIAN_POINT('Ctrl Pts',(-13.6792618652534,-8.57024119399876,
12.));
#32179=CARTESIAN_POINT('Ctrl Pts',(-14.2606595691012,-6.07318596563475,
-12.));
#32180=CARTESIAN_POINT('Ctrl Pts',(-13.9426682955425,-6.81987235459531,
-4.));
#32181=CARTESIAN_POINT('Ctrl Pts',(-13.5659153470886,-7.54152497364585,
4.));
#32182=CARTESIAN_POINT('Ctrl Pts',(-13.1350315879738,-8.22927361933666,
12.));
#32183=CARTESIAN_POINT('Ctrl Pts',(-16.9821964783418,-3.91067706686746,
-10.5713320279724));
#32184=CARTESIAN_POINT('Ctrl Pts',(-16.8018120500324,-4.69400019756954,
-3.52377734265748));
#32185=CARTESIAN_POINT('Ctrl Pts',(-16.5671448990744,-5.46481801274933,
3.52377734265749));
#32186=CARTESIAN_POINT('Ctrl Pts',(-16.2804353626266,-6.215771613699,10.5713320279725));
#32187=CARTESIAN_POINT('Ctrl Pts',(-16.9825696612994,-3.91076602011706,
-10.5713320279724));
#32188=CARTESIAN_POINT('Ctrl Pts',(-16.8021811299201,-4.69410636430758,
-3.52377734265748));
#32189=CARTESIAN_POINT('Ctrl Pts',(-16.5675086830329,-5.46494110853041,
3.5237773426575));
#32190=CARTESIAN_POINT('Ctrl Pts',(-16.280792708356,-6.21591119245835,10.5713320279725));
#32191=CARTESIAN_POINT('Ctrl Pts',(-16.9829428442892,-3.91085497337525,
-10.5713320279724));
#32192=CARTESIAN_POINT('Ctrl Pts',(-16.8025502098397,-4.69421253105573,
-3.52377734265747));
#32193=CARTESIAN_POINT('Ctrl Pts',(-16.5678724670228,-5.465064204323,3.52377734265748));
#32194=CARTESIAN_POINT('Ctrl Pts',(-16.2811500541162,-6.21605077123067,
10.5713320279725));
#32195=CARTESIAN_POINT('Ctrl Pts',(-16.9833160272816,-3.9109439266341,-10.5713320279724));
#32196=CARTESIAN_POINT('Ctrl Pts',(-16.8029192897619,-4.69431869780458,
-3.52377734265748));
#32197=CARTESIAN_POINT('Ctrl Pts',(-16.5682362510152,-5.46518730011656,
3.52377734265749));
#32198=CARTESIAN_POINT('Ctrl Pts',(-16.2815073998789,-6.21619035000399,
10.5713320279725));
#32199=CARTESIAN_POINT('Ctrl Pts',(-17.401685157391,-0.932601865546468,
-12.));
#32200=CARTESIAN_POINT('Ctrl Pts',(-17.3528542378989,-1.84375196972217,
-4.));
#32201=CARTESIAN_POINT('Ctrl Pts',(-17.2323154716912,-2.75104980175429,
4.));
#32202=CARTESIAN_POINT('Ctrl Pts',(-17.0415504627302,-3.6433432974125,12.));
#32203=CARTESIAN_POINT('Ctrl Pts',(-16.760386271272,-0.898232979305966,
-12.));
#32204=CARTESIAN_POINT('Ctrl Pts',(-16.7133549024554,-1.77580475232522,
-4.00000000000001));
#32205=CARTESIAN_POINT('Ctrl Pts',(-16.5972583138761,-2.64966621978703,
4.00000000000001));
#32206=CARTESIAN_POINT('Ctrl Pts',(-16.413523508407,-3.50907630101261,12.));
#32207=CARTESIAN_POINT('Ctrl Pts',(-16.1190873851531,-0.863864093065465,
-12.));
#32208=CARTESIAN_POINT('Ctrl Pts',(-16.0738555670119,-1.70785753492828,
-4.));
#32209=CARTESIAN_POINT('Ctrl Pts',(-15.962201156061,-2.54828263781977,4.));
#32210=CARTESIAN_POINT('Ctrl Pts',(-15.7854965540837,-3.37480930461271,
12.));
#32211=CARTESIAN_POINT('Ctrl Pts',(-15.4777884990342,-0.829495206824964,
-12.));
#32212=CARTESIAN_POINT('Ctrl Pts',(-15.4343562315683,-1.63991031753134,
-4.));
#32213=CARTESIAN_POINT('Ctrl Pts',(-15.3271439982459,-2.44689905585252,
4.));
#32214=CARTESIAN_POINT('Ctrl Pts',(-15.1574695997605,-3.24054230821282,
12.));
#32215=CARTESIAN_POINT('Ctrl Pts',(-15.1574696006874,-3.24054230387749,
11.9999999562994));
#32216=CARTESIAN_POINT('Ctrl Pts',(-15.1998732543785,-3.04220150129224,
10.0007056240913));
#32217=CARTESIAN_POINT('Ctrl Pts',(-15.2383960417531,-2.84297143492238,
8.00083387021915));
#32218=CARTESIAN_POINT('Ctrl Pts',(-15.2730067887526,-2.64296493179857,
5.99999995642121));
#32219=CARTESIAN_POINT('Ctrl Pts',(-15.3076042221209,-2.44303536468648,
3.9999356985046));
#32220=CARTESIAN_POINT('Ctrl Pts',(-15.3382726305944,-2.24244546120419,
2.00006422723888));
#32221=CARTESIAN_POINT('Ctrl Pts',(-15.3649942268768,-2.04131144317626,
2.22044604925031E-15));
#32222=CARTESIAN_POINT('Ctrl Pts',(-15.3917158231593,-1.84017742514834,
-2.00006422723888));
#32223=CARTESIAN_POINT('Ctrl Pts',(-15.4144854473596,-1.63853813118234,
-3.99993569850461));
#32224=CARTESIAN_POINT('Ctrl Pts',(-15.4332899241442,-1.43651039582365,
-5.99999995642121));
#32225=CARTESIAN_POINT('Ctrl Pts',(-15.4520989285132,-1.23443401791884,
-8.00054577305927));
#32226=CARTESIAN_POINT('Ctrl Pts',(-15.466932723784,-1.03205670355153,-10.0004173920443));
#32227=CARTESIAN_POINT('Ctrl Pts',(-15.477788520436,-0.829495208838559,
-11.9999999914697));
#32228=CARTESIAN_POINT('Ctrl Pts',(-15.3649941987044,2.04131143943342,-12.));
#32229=CARTESIAN_POINT('Ctrl Pts',(-15.4718770157346,1.23680222448176,-4.));
#32230=CARTESIAN_POINT('Ctrl Pts',(-15.5154431428507,0.423889388244509,
4.));
#32231=CARTESIAN_POINT('Ctrl Pts',(-15.4951570863805,-0.387435139568704,
12.));
#32232=CARTESIAN_POINT('Ctrl Pts',(-16.0016196226445,2.12589010856384,-12.));
#32233=CARTESIAN_POINT('Ctrl Pts',(-16.1129309684345,1.2880472643632,-4.));
#32234=CARTESIAN_POINT('Ctrl Pts',(-16.1583021924993,0.441452607469,4.));
#32235=CARTESIAN_POINT('Ctrl Pts',(-16.1371756137918,-0.403487931830612,
12.));
#32236=CARTESIAN_POINT('Ctrl Pts',(-16.6382450465846,2.21046877769426,-12.));
#32237=CARTESIAN_POINT('Ctrl Pts',(-16.7539849211345,1.33929230424465,-4.00000000000001));
#32238=CARTESIAN_POINT('Ctrl Pts',(-16.801161242148,0.459015826693492,4.00000000000001));
#32239=CARTESIAN_POINT('Ctrl Pts',(-16.7791941412031,-0.41954072409252,
12.));
#32240=CARTESIAN_POINT('Ctrl Pts',(-17.2748704705247,2.29504744682469,-12.));
#32241=CARTESIAN_POINT('Ctrl Pts',(-17.3950388738344,1.39053734412609,-4.));
#32242=CARTESIAN_POINT('Ctrl Pts',(-17.4440202917966,0.476579045917982,
4.));
#32243=CARTESIAN_POINT('Ctrl Pts',(-17.4212126686144,-0.435593516354428,
12.));
#32244=CARTESIAN_POINT('Ctrl Pts',(-15.3649942201102,2.04131144140431,-11.9999999914697));
#32245=CARTESIAN_POINT('Ctrl Pts',(-15.3917093519036,1.84022611326084,-10.0004173920443));
#32246=CARTESIAN_POINT('Ctrl Pts',(-15.4144808289508,1.63858762813028,-8.00054577305927));
#32247=CARTESIAN_POINT('Ctrl Pts',(-15.4332898445205,1.43651125126802,-5.99999995642121));
#32248=CARTESIAN_POINT('Ctrl Pts',(-15.4520943325031,1.23448351695164,-3.9999356985046));
#32249=CARTESIAN_POINT('Ctrl Pts',(-15.466930098069,1.03210574960204,-2.00006422723889));
#32250=CARTESIAN_POINT('Ctrl Pts',(-15.4777885274135,0.829495208345887,
-6.66133814775094E-15));
#32251=CARTESIAN_POINT('Ctrl Pts',(-15.4886469567579,0.626884667089732,
2.00006422723887));
#32252=CARTESIAN_POINT('Ctrl Pts',(-15.495525953138,0.424080475648491,3.99993569850462));
#32253=CARTESIAN_POINT('Ctrl Pts',(-15.4984215485681,0.221200142130421,
5.99999995642122));
#32254=CARTESIAN_POINT('Ctrl Pts',(-15.5013182582685,0.0182417370997574,
8.00083387021916));
#32255=CARTESIAN_POINT('Ctrl Pts',(-15.5002268324596,-0.184675569413391,
10.0007056240913));
#32256=CARTESIAN_POINT('Ctrl Pts',(-15.4951570864913,-0.387435135136787,
11.9999999562994));
#32257=CARTESIAN_POINT('Ctrl Pts',(-17.2955736705817,2.13341879826209,-10.5713320220547));
#32258=CARTESIAN_POINT('Ctrl Pts',(-17.3939672736713,1.33563987584167,-3.52377734068488));
#32259=CARTESIAN_POINT('Ctrl Pts',(-17.4370874835488,0.531047536999957,
3.52377734068489));
#32260=CARTESIAN_POINT('Ctrl Pts',(-17.4245226937903,-0.272677936184493,
10.5713320220547));
#32261=CARTESIAN_POINT('Ctrl Pts',(-17.2955750463446,2.1334188914951,-10.5713320279724));
#32262=CARTESIAN_POINT('Ctrl Pts',(-17.3939814195907,1.33564081785934,-3.52377734265747));
#32263=CARTESIAN_POINT('Ctrl Pts',(-17.4371016491204,0.531048112360097,
3.52377734265749));
#32264=CARTESIAN_POINT('Ctrl Pts',(-17.4245240716391,-0.272677881753643,
10.5713320279725));
#32265=CARTESIAN_POINT('Ctrl Pts',(-17.295956147427,2.13346293887238,-10.5713320279724));
#32266=CARTESIAN_POINT('Ctrl Pts',(-17.3943645524084,1.33566728651567,-3.52377734265748));
#32267=CARTESIAN_POINT('Ctrl Pts',(-17.4374855954662,0.531056861604773,
3.52377734265749));
#32268=CARTESIAN_POINT('Ctrl Pts',(-17.4249076055392,-0.272686823446403,
10.5713320279725));
#32269=CARTESIAN_POINT('Ctrl Pts',(-17.2963372485426,2.13350698625262,-10.5713320279724));
#32270=CARTESIAN_POINT('Ctrl Pts',(-17.3947476852595,1.33569375517339,-3.52377734265747));
#32271=CARTESIAN_POINT('Ctrl Pts',(-17.4378695418455,0.531065610849369,
3.52377734265748));
#32272=CARTESIAN_POINT('Ctrl Pts',(-17.4252911394727,-0.272695765140821,
10.5713320279725));
#32273=CARTESIAN_POINT('Ctrl Pts',(-17.2967183496608,2.13355103363312,-10.5713320279724));
#32274=CARTESIAN_POINT('Ctrl Pts',(-17.3951308181133,1.33572022383134,-3.52377734265747));
#32275=CARTESIAN_POINT('Ctrl Pts',(-17.4382534882274,0.531074360093894,
3.52377734265749));
#32276=CARTESIAN_POINT('Ctrl Pts',(-17.4256746734088,-0.272704706835343,
10.5713320279725));
#32277=CARTESIAN_POINT('Origin',(2.22044604925031E-15,-4.16333634234434E-16,
-6.));
#32278=CARTESIAN_POINT('Ctrl Pts',(-15.3516930767777,2.1390462349833,11.9999999562994));
#32279=CARTESIAN_POINT('Ctrl Pts',(-15.3237029275181,2.33992852728641,10.0007056240913));
#32280=CARTESIAN_POINT('Ctrl Pts',(-15.2917618106915,2.540319119752,8.00083387021915));
#32281=CARTESIAN_POINT('Ctrl Pts',(-15.2558790213823,2.74010132749603,5.99999995642122));
#32282=CARTESIAN_POINT('Ctrl Pts',(-15.2200100350179,2.9398066855075,3.9999356985046));
#32283=CARTESIAN_POINT('Ctrl Pts',(-15.1802231246131,3.13878875107565,2.00006422723889));
#32284=CARTESIAN_POINT('Ctrl Pts',(-15.1365413257817,3.33693222779592,-2.22044604925031E-15));
#32285=CARTESIAN_POINT('Ctrl Pts',(-15.0928595269503,3.53507570451619,-2.00006422723887));
#32286=CARTESIAN_POINT('Ctrl Pts',(-15.0452912745672,3.73234233124902,-3.99993569850461));
#32287=CARTESIAN_POINT('Ctrl Pts',(-14.9938641476362,3.92861781320468,-5.99999995642121));
#32288=CARTESIAN_POINT('Ctrl Pts',(-14.9424246385123,4.12494055272707,-8.00054577305927));
#32289=CARTESIAN_POINT('Ctrl Pts',(-14.8871467284008,4.32018647843708,-10.0004173920443));
#32290=CARTESIAN_POINT('Ctrl Pts',(-14.8280677289535,4.51424492140109,-11.9999999914697));
#32291=CARTESIAN_POINT('Ctrl Pts',(-16.67120375536,5.07536776045384,-12.));
#32292=CARTESIAN_POINT('Ctrl Pts',(-16.9369493898684,4.20246557304821,-4.));
#32293=CARTESIAN_POINT('Ctrl Pts',(-17.1339941352951,3.30865780933792,4.));
#32294=CARTESIAN_POINT('Ctrl Pts',(-17.2599160133439,2.40493072018629,12.));
#32295=CARTESIAN_POINT('Ctrl Pts',(-16.0568250729579,4.88832681229368,-12.));
#32296=CARTESIAN_POINT('Ctrl Pts',(-16.312777266322,4.047593417474,-4.));
#32297=CARTESIAN_POINT('Ctrl Pts',(-16.5025603830837,3.18672487304549,4.));
#32298=CARTESIAN_POINT('Ctrl Pts',(-16.6238417013591,2.31630255698833,12.));
#32299=CARTESIAN_POINT('Ctrl Pts',(-15.4424463905558,4.70128586413352,-12.));
#32300=CARTESIAN_POINT('Ctrl Pts',(-15.6886051427755,3.89272126189978,-4.));
#32301=CARTESIAN_POINT('Ctrl Pts',(-15.8711266308723,3.06479193675306,4.));
#32302=CARTESIAN_POINT('Ctrl Pts',(-15.9877673893743,2.22767439379038,12.));
#32303=CARTESIAN_POINT('Ctrl Pts',(-14.8280677081536,4.51424491597336,-12.));
#32304=CARTESIAN_POINT('Ctrl Pts',(-15.0644330192291,3.73784910632557,-4.));
#32305=CARTESIAN_POINT('Ctrl Pts',(-15.2396928786609,2.94285900046063,4.));
#32306=CARTESIAN_POINT('Ctrl Pts',(-15.3516930773895,2.13904623059242,12.));
#32307=CARTESIAN_POINT('Ctrl Pts',(-15.5228520082561,7.92019304563385,-10.5713320279724));
#32308=CARTESIAN_POINT('Ctrl Pts',(-15.8881799221207,7.2041838386953,-3.52377734265748));
#32309=CARTESIAN_POINT('Ctrl Pts',(-16.20388659607,6.46286199768347,3.52377734265748));
#32310=CARTESIAN_POINT('Ctrl Pts',(-16.4669580190248,5.70330482702814,10.5713320279724));
#32311=CARTESIAN_POINT('Ctrl Pts',(-15.5231950610337,7.92036478087257,-10.5713320279724));
#32312=CARTESIAN_POINT('Ctrl Pts',(-15.8885308963815,7.2043397502344,-3.52377734265747));
#32313=CARTESIAN_POINT('Ctrl Pts',(-16.2042443951928,6.46300153666554,3.52377734265747));
#32314=CARTESIAN_POINT('Ctrl Pts',(-16.4673214812322,5.70342760090243,10.5713320279724));
#32315=CARTESIAN_POINT('Ctrl Pts',(-15.5235381138415,7.92053651612543,-10.5713320279724));
#32316=CARTESIAN_POINT('Ctrl Pts',(-15.8888818706732,7.20449566178622,-3.52377734265749));
#32317=CARTESIAN_POINT('Ctrl Pts',(-16.204602194347,6.46314107565896,3.52377734265749));
#32318=CARTESIAN_POINT('Ctrl Pts',(-16.4676849434715,5.70355037478656,10.5713320279724));
#32319=CARTESIAN_POINT('Ctrl Pts',(-15.5238811666517,7.92070825137944,-10.5713320279724));
#32320=CARTESIAN_POINT('Ctrl Pts',(-15.8892328449674,7.20465157333916,-3.52377734265748));
#32321=CARTESIAN_POINT('Ctrl Pts',(-16.2049599935037,6.46328061465322,3.52377734265748));
#32322=CARTESIAN_POINT('Ctrl Pts',(-16.4680484057134,5.7036731486715,10.5713320279724));
#32323=CARTESIAN_POINT('Ctrl Pts',(-15.5228507477965,7.92019248660845,-10.5713320134286));
#32324=CARTESIAN_POINT('Ctrl Pts',(-15.8881669516022,7.20417811498611,-3.52377733780954));
#32325=CARTESIAN_POINT('Ctrl Pts',(-16.2038734814214,6.46285661240599,3.52377733780955));
#32326=CARTESIAN_POINT('Ctrl Pts',(-16.466956742565,5.70330430555751,10.5713320134286));
#32327=CARTESIAN_POINT('Ctrl Pts',(-13.7402020358534,7.17334281440038,-12.));
#32328=CARTESIAN_POINT('Ctrl Pts',(-14.1157973873101,6.45390751815577,-4.));
#32329=CARTESIAN_POINT('Ctrl Pts',(-14.4347687202385,5.70491981764188,4.00000000000001));
#32330=CARTESIAN_POINT('Ctrl Pts',(-14.6931953939549,4.93558590585174,12.));
#32331=CARTESIAN_POINT('Ctrl Pts',(-14.3095066403964,7.47055948439889,-12.));
#32332=CARTESIAN_POINT('Ctrl Pts',(-14.7006642203029,6.72131546876616,-3.99999999999999));
#32333=CARTESIAN_POINT('Ctrl Pts',(-15.0328516506423,5.94129458944341,4.));
#32334=CARTESIAN_POINT('Ctrl Pts',(-15.3019858448814,5.14008448418317,12.));
#32335=CARTESIAN_POINT('Ctrl Pts',(-14.8788112449393,7.76777615439741,-12.));
#32336=CARTESIAN_POINT('Ctrl Pts',(-15.2855310532957,6.98872341937656,-4.00000000000001));
#32337=CARTESIAN_POINT('Ctrl Pts',(-15.6309345810462,6.17766936124494,4.00000000000002));
#32338=CARTESIAN_POINT('Ctrl Pts',(-15.9107762958078,5.3445830625146,12.));
#32339=CARTESIAN_POINT('Ctrl Pts',(-15.4481158494823,8.06499282439592,-12.));
#32340=CARTESIAN_POINT('Ctrl Pts',(-15.8703978862885,7.25613136998696,-4.));
#32341=CARTESIAN_POINT('Ctrl Pts',(-16.2290175114501,6.41404413304647,4.00000000000001));
#32342=CARTESIAN_POINT('Ctrl Pts',(-16.5195667467343,5.54908164084603,12.));
#32343=CARTESIAN_POINT('Ctrl Pts',(-13.7402020552943,7.17334282357369,-11.9999999914697));
#32344=CARTESIAN_POINT('Ctrl Pts',(-13.8340813002562,6.99352153777387,-10.0004173920443));
#32345=CARTESIAN_POINT('Ctrl Pts',(-13.9244439127861,6.81183164507365,-8.00054577305927));
#32346=CARTESIAN_POINT('Ctrl Pts',(-14.0112327972984,6.628375027102,-5.99999995642121));
#32347=CARTESIAN_POINT('Ctrl Pts',(-14.09800079054,6.44496256964577,-3.99993569850462));
#32348=CARTESIAN_POINT('Ctrl Pts',(-14.1811591229608,6.25986380572142,-2.00006422723887));
#32349=CARTESIAN_POINT('Ctrl Pts',(-14.2606595952488,6.07318597677023,-4.44089209839888E-15));
#32350=CARTESIAN_POINT('Ctrl Pts',(-14.3401600675367,5.88650814781904,2.00006422723887));
#32351=CARTESIAN_POINT('Ctrl Pts',(-14.4159873282975,5.69828730098518,3.99993569850462));
#32352=CARTESIAN_POINT('Ctrl Pts',(-14.4880974587037,5.50863250063968,5.99999995642122));
#32353=CARTESIAN_POINT('Ctrl Pts',(-14.5602353382114,5.31890471817276,8.00083387021916));
#32354=CARTESIAN_POINT('Ctrl Pts',(-14.6286115396895,5.12785153300099,10.0007056240913));
#32355=CARTESIAN_POINT('Ctrl Pts',(-14.6931953925432,4.93558591005428,11.9999999562994));
#32356=CARTESIAN_POINT('Origin',(2.22044604925031E-15,-4.16333634234434E-16,
-6.));
#32357=CARTESIAN_POINT('Origin',(2.22044604925031E-15,-4.16333634234434E-16,
-6.));
#32358=CARTESIAN_POINT('Ctrl Pts',(-13.6942758009489,7.26063422894488,11.9999999562994));
#32359=CARTESIAN_POINT('Ctrl Pts',(-13.5992678738299,7.43982864180721,10.0007056240913));
#32360=CARTESIAN_POINT('Ctrl Pts',(-13.500715422892,7.617209697467,8.00083387021915));
#32361=CARTESIAN_POINT('Ctrl Pts',(-13.3986670912385,7.79267092710594,5.99999995642121));
#32362=CARTESIAN_POINT('Ctrl Pts',(-13.2966580142668,7.9680646625034,3.9999356985046));
#32363=CARTESIAN_POINT('Ctrl Pts',(-13.1912146735706,8.14143871638738,2.00006422723888));
#32364=CARTESIAN_POINT('Ctrl Pts',(-13.0823981492392,8.31269262422126,2.22030256658695E-15));
#32365=CARTESIAN_POINT('Ctrl Pts',(-12.9735816249078,8.48394653205514,-2.00006422723887));
#32366=CARTESIAN_POINT('Ctrl Pts',(-12.8614129292112,8.65304722502548,-3.9999356985046));
#32367=CARTESIAN_POINT('Ctrl Pts',(-12.7459570690561,8.81989673373664,-5.99999995642121));
#32368=CARTESIAN_POINT('Ctrl Pts',(-12.630473410406,8.98678641507513,-8.00054577305927));
#32369=CARTESIAN_POINT('Ctrl Pts',(-12.5117511266867,9.15135141196428,-10.0004173920443));
#32370=CARTESIAN_POINT('Ctrl Pts',(-12.3898631303866,9.31350049096029,-11.9999999914697));
#32371=CARTESIAN_POINT('Ctrl Pts',(-10.4581387236936,11.4401631786859,-12.));
#32372=CARTESIAN_POINT('Ctrl Pts',(-11.0571442669941,10.8925763156096,-4.));
#32373=CARTESIAN_POINT('Ctrl Pts',(-11.613048155468,10.2978527213822,4.));
#32374=CARTESIAN_POINT('Ctrl Pts',(-12.1190174885494,9.66330244953633,12.));
#32375=CARTESIAN_POINT('Ctrl Pts',(-10.8914559714904,11.9141691326998,-12.));
#32376=CARTESIAN_POINT('Ctrl Pts',(-11.5152804085056,11.3438938315843,-4.00000000000002));
#32377=CARTESIAN_POINT('Ctrl Pts',(-12.0942173384564,10.7245287597614,4.00000000000001));
#32378=CARTESIAN_POINT('Ctrl Pts',(-12.6211507498191,10.0636868518367,12.));
#32379=CARTESIAN_POINT('Ctrl Pts',(-11.3247732192871,12.3881750867137,-12.));
#32380=CARTESIAN_POINT('Ctrl Pts',(-11.9734165500172,11.795211347559,-3.99999999999999));
#32381=CARTESIAN_POINT('Ctrl Pts',(-12.5753865214448,11.1512047981406,3.99999999999998));
#32382=CARTESIAN_POINT('Ctrl Pts',(-13.1232840110888,10.4640712541372,12.));
#32383=CARTESIAN_POINT('Ctrl Pts',(-11.7580904670839,12.8621810407276,-12.));
#32384=CARTESIAN_POINT('Ctrl Pts',(-12.4315526915288,12.2465288635337,-4.));
#32385=CARTESIAN_POINT('Ctrl Pts',(-13.0565557044332,11.5778808365198,4.));
#32386=CARTESIAN_POINT('Ctrl Pts',(-13.6254172723584,10.8644556564376,12.));
#32387=CARTESIAN_POINT('Ctrl Pts',(-10.4581387388246,11.4401631939552,-11.9999999914697));
#32388=CARTESIAN_POINT('Ctrl Pts',(-10.6078588745025,11.303295051446,-10.0004173920443));
#32389=CARTESIAN_POINT('Ctrl Pts',(-10.7549135578339,11.163468233693,-8.00054577305927));
#32390=CARTESIAN_POINT('Ctrl Pts',(-10.8992142909491,11.0207589502706,-5.99999995642121));
#32391=CARTESIAN_POINT('Ctrl Pts',(-11.0434802889055,10.8780840189234,-3.99993569850461));
#32392=CARTESIAN_POINT('Ctrl Pts',(-11.184931066005,10.7325899011204,-2.00006422723887));
#32393=CARTESIAN_POINT('Ctrl Pts',(-11.3234846509767,10.584360885717,2.2202945954294E-15));
#32394=CARTESIAN_POINT('Ctrl Pts',(-11.4620382359483,10.4361318703137,2.00006422723887));
#32395=CARTESIAN_POINT('Ctrl Pts',(-11.5976678743505,10.2851965800591,3.99993569850461));
#32396=CARTESIAN_POINT('Ctrl Pts',(-11.7302949937737,10.1316424808146,5.99999995642121));
#32397=CARTESIAN_POINT('Ctrl Pts',(-11.8629731501784,9.97802929156078,8.00083387021915));
#32398=CARTESIAN_POINT('Ctrl Pts',(-11.99256979992,9.82188406150686,10.0007056240913));
#32399=CARTESIAN_POINT('Ctrl Pts',(-12.1190174857855,9.66330245300261,11.9999999562994));
#32400=CARTESIAN_POINT('Ctrl Pts',(-11.8778429311088,12.7516740731249,-10.5713320220547));
#32401=CARTESIAN_POINT('Ctrl Pts',(-12.466019210595,12.2037861517057,-3.52377734068488));
#32402=CARTESIAN_POINT('Ctrl Pts',(-13.0162331940139,11.6151497981962,3.52377734068489));
#32403=CARTESIAN_POINT('Ctrl Pts',(-13.5232327823929,10.9913838744951,10.5713320220547));
#32404=CARTESIAN_POINT('Ctrl Pts',(-13.9299291396692,10.4711731300928,-12.));
#32405=CARTESIAN_POINT('Ctrl Pts',(-14.4781984826686,9.74180374592263,-4.));
#32406=CARTESIAN_POINT('Ctrl Pts',(-14.9690602353605,8.96929245803532,4.));
#32407=CARTESIAN_POINT('Ctrl Pts',(-15.3964809635174,8.1631345999333,12.));
#32408=CARTESIAN_POINT('Ctrl Pts',(-13.4165737973453,10.0852822463105,-12.));
#32409=CARTESIAN_POINT('Ctrl Pts',(-13.9446379409184,9.38279208500909,-4.00000000000001));
#32410=CARTESIAN_POINT('Ctrl Pts',(-14.4174101182391,8.63874991513855,4.));
#32411=CARTESIAN_POINT('Ctrl Pts',(-14.8290792433535,7.86230114163155,12.));
#32412=CARTESIAN_POINT('Ctrl Pts',(-12.9032184550213,9.6993913625282,-12.));
#32413=CARTESIAN_POINT('Ctrl Pts',(-13.4110773991682,9.02378042409555,-4.));
#32414=CARTESIAN_POINT('Ctrl Pts',(-13.8657600011178,8.30820737224178,3.99999999999999));
#32415=CARTESIAN_POINT('Ctrl Pts',(-14.2616775231895,7.56146768332979,12.));
#32416=CARTESIAN_POINT('Ctrl Pts',(-12.3898631126974,9.3135004787459,-12.));
#32417=CARTESIAN_POINT('Ctrl Pts',(-12.877516857418,8.66476876318201,-4.));
#32418=CARTESIAN_POINT('Ctrl Pts',(-13.3141098839964,7.977664829345,4.));
#32419=CARTESIAN_POINT('Ctrl Pts',(-13.6942758030256,7.26063422502805,12.));
#32420=CARTESIAN_POINT('Ctrl Pts',(-11.8778439250753,12.7516750288689,-10.5713320279724));
#32421=CARTESIAN_POINT('Ctrl Pts',(-12.4660294414806,12.2037959661548,-3.52377734265748));
#32422=CARTESIAN_POINT('Ctrl Pts',(-13.0162436756369,11.6151593444016,3.52377734265749));
#32423=CARTESIAN_POINT('Ctrl Pts',(-13.5232338028988,10.9913848018556,10.5713320279725));
#32424=CARTESIAN_POINT('Ctrl Pts',(-11.8781075523334,12.7519537381713,-10.5713320279724));
#32425=CARTESIAN_POINT('Ctrl Pts',(-12.4663059245223,12.20406251535,-3.52377734265749));
#32426=CARTESIAN_POINT('Ctrl Pts',(-13.0165321716956,11.6154128426657,3.52377734265749));
#32427=CARTESIAN_POINT('Ctrl Pts',(-13.5235333545211,10.9916244829605,10.5713320279725));
#32428=CARTESIAN_POINT('Ctrl Pts',(-11.878371179615,12.7522324474973,-10.5713320279724));
#32429=CARTESIAN_POINT('Ctrl Pts',(-12.4665824075886,12.2043290645677,-3.52377734265747));
#32430=CARTESIAN_POINT('Ctrl Pts',(-13.0168206677798,11.6156663409513,3.52377734265748));
#32431=CARTESIAN_POINT('Ctrl Pts',(-13.5238329061699,10.9918641640855,10.5713320279725));
#32432=CARTESIAN_POINT('Ctrl Pts',(-11.8786348068985,12.7525111568252,-10.5713320279724));
#32433=CARTESIAN_POINT('Ctrl Pts',(-12.4668588906568,12.2045956137873,-3.52377734265748));
#32434=CARTESIAN_POINT('Ctrl Pts',(-13.0171091638662,11.6159198392386,3.52377734265749));
#32435=CARTESIAN_POINT('Ctrl Pts',(-13.5241324578209,10.9921038452121,10.5713320279725));
#32436=CARTESIAN_POINT('Ctrl Pts',(-9.50849948587548,14.604000482186,-12.));
#32437=CARTESIAN_POINT('Ctrl Pts',(-10.2731631630064,14.1061366133278,-4.));
#32438=CARTESIAN_POINT('Ctrl Pts',(-10.9986367512409,13.5480980636351,4.));
#32439=CARTESIAN_POINT('Ctrl Pts',(-11.6760030816321,12.9367439718926,12.));
#32440=CARTESIAN_POINT('Ctrl Pts',(-9.15808571423197,14.0658037985085,-12.));
#32441=CARTESIAN_POINT('Ctrl Pts',(-9.89456947890246,13.5862875518289,-3.99999999999999));
#32442=CARTESIAN_POINT('Ctrl Pts',(-10.5933074148231,13.0488142230957,4.));
#32443=CARTESIAN_POINT('Ctrl Pts',(-11.2457109746983,12.4599901733872,12.));
#32444=CARTESIAN_POINT('Ctrl Pts',(-8.80767194258845,13.5276071148311,-12.));
#32445=CARTESIAN_POINT('Ctrl Pts',(-9.51597579479849,13.0664384903301,-4.));
#32446=CARTESIAN_POINT('Ctrl Pts',(-10.1879780784053,12.5495303825563,4.00000000000001));
#32447=CARTESIAN_POINT('Ctrl Pts',(-10.8154188677646,11.9832363748819,12.));
#32448=CARTESIAN_POINT('Ctrl Pts',(-8.45725817094493,12.9894104311537,-12.));
#32449=CARTESIAN_POINT('Ctrl Pts',(-9.13738211069452,12.5465894288312,-4.));
#32450=CARTESIAN_POINT('Ctrl Pts',(-9.78264874198741,12.0502465420169,4.));
#32451=CARTESIAN_POINT('Ctrl Pts',(-10.3851267608308,11.5064825763765,12.));
#32452=CARTESIAN_POINT('Ctrl Pts',(-10.3851267575397,11.5064825793468,11.9999999562994));
#32453=CARTESIAN_POINT('Ctrl Pts',(-10.2345604107395,11.6423756219493,10.0007056240913));
#32454=CARTESIAN_POINT('Ctrl Pts',(-10.0812835057528,11.7753523676252,8.00083387021915));
#32455=CARTESIAN_POINT('Ctrl Pts',(-9.92537816662526,11.9053294053327,5.99999995642121));
#32456=CARTESIAN_POINT('Ctrl Pts',(-9.7695327992227,12.0352564450914,3.99993569850461));
#32457=CARTESIAN_POINT('Ctrl Pts',(-9.61115105130114,12.1621110176642,2.00006422723887));
#32458=CARTESIAN_POINT('Ctrl Pts',(-9.45032468026493,12.2858196078884,-2.22030256658673E-15));
#32459=CARTESIAN_POINT('Ctrl Pts',(-9.28949830922872,12.4095281981127,-2.00006422723889));
#32460=CARTESIAN_POINT('Ctrl Pts',(-9.12625837035319,12.5300669180878,-3.99993569850459));
#32461=CARTESIAN_POINT('Ctrl Pts',(-8.9606994576558,12.6473659403674,-5.9999999564212));
#32462=CARTESIAN_POINT('Ctrl Pts',(-8.79510068306996,12.7646932049232,-8.00054577305927));
#32463=CARTESIAN_POINT('Ctrl Pts',(-8.62725368531362,12.878728305646,-10.0004173920443));
#32464=CARTESIAN_POINT('Ctrl Pts',(-8.45725818338971,12.9894104486815,-11.9999999914697));
#32465=CARTESIAN_POINT('Ctrl Pts',(-5.91466953576705,14.3271310247952,-12.));
#32466=CARTESIAN_POINT('Ctrl Pts',(-6.66483636200897,14.0174396520956,-4.));
#32467=CARTESIAN_POINT('Ctrl Pts',(-7.39062259281095,13.648712606804,4.));
#32468=CARTESIAN_POINT('Ctrl Pts',(-8.08310721637551,13.2254821026516,12.));
#32469=CARTESIAN_POINT('Ctrl Pts',(-6.15973497165189,14.9207541491876,-12.));
#32470=CARTESIAN_POINT('Ctrl Pts',(-6.94098383200367,14.5982311802709,-4.));
#32471=CARTESIAN_POINT('Ctrl Pts',(-7.69684192361463,14.2142264844647,4.));
#32472=CARTESIAN_POINT('Ctrl Pts',(-8.41801860598165,13.7734600609591,12.));
#32473=CARTESIAN_POINT('Ctrl Pts',(-6.40480040753672,15.51437727358,-12.));
#32474=CARTESIAN_POINT('Ctrl Pts',(-7.21713130199837,15.1790227084462,-4.00000000000001));
#32475=CARTESIAN_POINT('Ctrl Pts',(-8.00306125441831,14.7797403621254,4.00000000000001));
#32476=CARTESIAN_POINT('Ctrl Pts',(-8.7529299955878,14.3214380192667,12.));
#32477=CARTESIAN_POINT('Ctrl Pts',(-6.64986584342155,16.1080003979724,-12.));
#32478=CARTESIAN_POINT('Ctrl Pts',(-7.49327877199307,15.7598142366215,-4.));
#32479=CARTESIAN_POINT('Ctrl Pts',(-8.30928058522199,15.3452542397861,4.));
#32480=CARTESIAN_POINT('Ctrl Pts',(-9.08784138519395,14.8694159775742,12.));
#32481=CARTESIAN_POINT('Ctrl Pts',(-5.91466954476314,14.3271310443187,-11.9999999914697));
#32482=CARTESIAN_POINT('Ctrl Pts',(-6.10217211316042,14.2497243630455,-10.0004173920443));
#32483=CARTESIAN_POINT('Ctrl Pts',(-6.28818190218765,14.1686257980847,-8.00054577305927));
#32484=CARTESIAN_POINT('Ctrl Pts',(-6.47258968583998,14.0838766949572,-5.99999995642121));
#32485=CARTESIAN_POINT('Ctrl Pts',(-6.65695308001831,13.9991479920971,-3.99993569850461));
#32486=CARTESIAN_POINT('Ctrl Pts',(-6.83963525048718,13.910807258287,-2.00006422723887));
#32487=CARTESIAN_POINT('Ctrl Pts',(-7.02053034096173,13.8189056633163,0.));
#32488=CARTESIAN_POINT('Ctrl Pts',(-7.20142543143627,13.7270040683457,2.00006422723886));
#32489=CARTESIAN_POINT('Ctrl Pts',(-7.38049851140844,13.6315593582429,3.99993569850462));
#32490=CARTESIAN_POINT('Ctrl Pts',(-7.5576458318784,13.5326268506854,5.99999995642121));
#32491=CARTESIAN_POINT('Ctrl Pts',(-7.73486132139669,13.4336562723579,8.00083387021915));
#32492=CARTESIAN_POINT('Ctrl Pts',(-7.91004715080012,13.3312524166245,10.0007056240913));
#32493=CARTESIAN_POINT('Ctrl Pts',(-8.08310721259277,13.2254821049635,11.9999999562994));
#32494=CARTESIAN_POINT('Ctrl Pts',(-6.80019195908459,16.04511557088,-10.5713320220547));
#32495=CARTESIAN_POINT('Ctrl Pts',(-7.54028557404928,15.7314374695154,-3.52377734068489));
#32496=CARTESIAN_POINT('Ctrl Pts',(-8.25864308411527,15.3664844972649,3.52377734068488));
#32497=CARTESIAN_POINT('Ctrl Pts',(-8.94840736668244,14.9537403335486,10.5713320220547));
#32498=CARTESIAN_POINT('Ctrl Pts',(-6.80019256622393,16.0451168089422,-10.5713320279724));
#32499=CARTESIAN_POINT('Ctrl Pts',(-7.54029183119772,15.7314501912497,-3.52377734265748));
#32500=CARTESIAN_POINT('Ctrl Pts',(-8.25864966862456,15.3664970526898,3.52377734265748));
#32501=CARTESIAN_POINT('Ctrl Pts',(-8.94840800846833,14.9537415540161,10.5713320279724));
#32502=CARTESIAN_POINT('Ctrl Pts',(-6.80034497061741,16.0454688758496,-10.5713320279724));
#32503=CARTESIAN_POINT('Ctrl Pts',(-7.54046047507779,15.731795228331,-3.52377734265747));
#32504=CARTESIAN_POINT('Ctrl Pts',(-8.25883406472934,15.3668339346014,3.52377734265747));
#32505=CARTESIAN_POINT('Ctrl Pts',(-8.94860751915147,14.9540692332704,10.5713320279724));
#32506=CARTESIAN_POINT('Ctrl Pts',(-6.80049737502494,16.0458209427872,-10.5713320279724));
#32507=CARTESIAN_POINT('Ctrl Pts',(-7.54062911897336,15.732140265442,-3.52377734265749));
#32508=CARTESIAN_POINT('Ctrl Pts',(-8.2590184608509,15.3671708165418,3.52377734265749));
#32509=CARTESIAN_POINT('Ctrl Pts',(-8.94880702985271,14.9543969125528,10.5713320279724));
#32510=CARTESIAN_POINT('Ctrl Pts',(-6.80064977943358,16.0461730097273,-10.5713320279724));
#32511=CARTESIAN_POINT('Ctrl Pts',(-7.54079776287006,15.7324853025554,-3.52377734265748));
#32512=CARTESIAN_POINT('Ctrl Pts',(-8.25920285697384,15.3675076984845,3.52377734265748));
#32513=CARTESIAN_POINT('Ctrl Pts',(-8.94900654055538,14.9547245918374,10.5713320279724));
#32514=CARTESIAN_POINT('Origin',(2.22044604925031E-15,-4.16333634234434E-16,
-6.));
#32515=CARTESIAN_POINT('Ctrl Pts',(-5.82337815902385,14.3644793130828,11.9999999562994));
#32516=CARTESIAN_POINT('Ctrl Pts',(-5.63541391608915,14.4406802789199,10.0007056240913));
#32517=CARTESIAN_POINT('Ctrl Pts',(-5.44590001392117,14.5132137565555,8.00083387021915));
#32518=CARTESIAN_POINT('Ctrl Pts',(-5.25494215213615,14.5820294533272,5.99999995642121));
#32519=CARTESIAN_POINT('Ctrl Pts',(-5.06405774564414,14.6508186789333,3.9999356985046));
#32520=CARTESIAN_POINT('Ctrl Pts',(-4.87184076676219,14.7158532365687,2.00006422723888));
#32521=CARTESIAN_POINT('Ctrl Pts',(-4.67840258291259,14.7770954274579,2.22044604925031E-15));
#32522=CARTESIAN_POINT('Ctrl Pts',(-4.48496439906298,14.8383376183471,-2.00006422723888));
#32523=CARTESIAN_POINT('Ctrl Pts',(-4.29034236280191,14.895775616736,-3.99993569850461));
#32524=CARTESIAN_POINT('Ctrl Pts',(-4.0946492458228,14.949376159348,-5.99999995642121));
#32525=CARTESIAN_POINT('Ctrl Pts',(-3.89890901149391,15.0029896074497,-8.00054577305927));
#32526=CARTESIAN_POINT('Ctrl Pts',(-3.70218212478788,15.05274049588,-10.0004173920443));
#32527=CARTESIAN_POINT('Ctrl Pts',(-3.50458308363856,15.0986058030105,-11.9999999914697));
#32528=CARTESIAN_POINT('Ctrl Pts',(-3.94020446357842,16.9753698440352,-12.));
#32529=CARTESIAN_POINT('Ctrl Pts',(-4.82903275014493,16.7690612207615,-4.));
#32530=CARTESIAN_POINT('Ctrl Pts',(-5.70161535233114,16.4928030941281,4.));
#32531=CARTESIAN_POINT('Ctrl Pts',(-6.54722690864904,16.1499910948348,12.));
#32532=CARTESIAN_POINT('Ctrl Pts',(-3.794997335032,16.3497818234513,-12.));
#32533=CARTESIAN_POINT('Ctrl Pts',(-4.65106990943784,16.1510762276491,-4.));
#32534=CARTESIAN_POINT('Ctrl Pts',(-5.49149549661271,15.8849989557599,4.));
#32535=CARTESIAN_POINT('Ctrl Pts',(-6.30594399347681,15.5548205003623,12.));
#32536=CARTESIAN_POINT('Ctrl Pts',(-3.64979020648557,15.7241938028673,-12.));
#32537=CARTESIAN_POINT('Ctrl Pts',(-4.47310706873074,15.5330912345367,-4.));
#32538=CARTESIAN_POINT('Ctrl Pts',(-5.28137564089428,15.2771948173917,4.));
#32539=CARTESIAN_POINT('Ctrl Pts',(-6.06466107830459,14.9596499058898,12.));
#32540=CARTESIAN_POINT('Ctrl Pts',(-3.50458307793915,15.0986057822834,-12.));
#32541=CARTESIAN_POINT('Ctrl Pts',(-4.29514422802365,14.9151062414243,-4.));
#32542=CARTESIAN_POINT('Ctrl Pts',(-5.07125578517585,14.6693906790234,4.));
#32543=CARTESIAN_POINT('Ctrl Pts',(-5.82337816313236,14.3644793114172,12.));
#32544=CARTESIAN_POINT('Ctrl Pts',(-0.902337623732298,17.403280701153,-10.5713320279724));
#32545=CARTESIAN_POINT('Ctrl Pts',(-1.70508374321692,17.361659351802,-3.52377734265748));
#32546=CARTESIAN_POINT('Ctrl Pts',(-2.50494062688805,17.2644084310805,3.52377734265748));
#32547=CARTESIAN_POINT('Ctrl Pts',(-3.29427214377962,17.1124563810414,10.5713320279724));
#32548=CARTESIAN_POINT('Ctrl Pts',(-0.902360423041643,17.4036636611926,
-10.5713320279724));
#32549=CARTESIAN_POINT('Ctrl Pts',(-1.70512420699373,17.3620412601975,-3.52377734265747));
#32550=CARTESIAN_POINT('Ctrl Pts',(-2.50499868214617,17.2647880637013,3.52377734265747));
#32551=CARTESIAN_POINT('Ctrl Pts',(-3.29434754958927,17.1128325354835,10.5713320279724));
#32552=CARTESIAN_POINT('Ctrl Pts',(-0.902383222353851,17.4040466212655,
-10.5713320279724));
#32553=CARTESIAN_POINT('Ctrl Pts',(-1.70516467077498,17.3624231686262,-3.52377734265748));
#32554=CARTESIAN_POINT('Ctrl Pts',(-2.50505673741016,17.265167696355,3.52377734265748));
#32555=CARTESIAN_POINT('Ctrl Pts',(-3.29442295540635,17.1132086899581,10.5713320279724));
#32556=CARTESIAN_POINT('Ctrl Pts',(-0.902406021666259,17.4044295813409,
-10.5713320279724));
#32557=CARTESIAN_POINT('Ctrl Pts',(-1.70520513455646,17.3628050770574,-3.52377734265748));
#32558=CARTESIAN_POINT('Ctrl Pts',(-2.50511479267468,17.2655473290114,3.52377734265748));
#32559=CARTESIAN_POINT('Ctrl Pts',(-3.29449836122398,17.1135848444354,10.5713320279724));
#32560=CARTESIAN_POINT('Ctrl Pts',(-0.902337477632694,17.4032793300502,
-10.5713320134286));
#32561=CARTESIAN_POINT('Ctrl Pts',(-1.70508221483526,17.361645257149,-3.52377733780954));
#32562=CARTESIAN_POINT('Ctrl Pts',(-2.50493873335086,17.2643943808229,3.52377733780954));
#32563=CARTESIAN_POINT('Ctrl Pts',(-3.29427195715649,17.1124550148594,10.5713320134286));
#32564=CARTESIAN_POINT('Ctrl Pts',(-0.657803910601428,15.4860354233799,
-12.));
#32565=CARTESIAN_POINT('Ctrl Pts',(-1.46865082925679,15.4515928911625,-4.));
#32566=CARTESIAN_POINT('Ctrl Pts',(-2.2767788714881,15.3533363183005,4.));
#32567=CARTESIAN_POINT('Ctrl Pts',(-3.07225491994942,15.1924734268593,12.));
#32568=CARTESIAN_POINT('Ctrl Pts',(-0.685059026225969,16.1276760084048,
-12.));
#32569=CARTESIAN_POINT('Ctrl Pts',(-1.52950216735065,16.0918064016704,-4.00000000000002));
#32570=CARTESIAN_POINT('Ctrl Pts',(-2.37111377949615,15.9894787155008,4.00000000000002));
#32571=CARTESIAN_POINT('Ctrl Pts',(-3.19954918153982,15.8219507121087,12.));
#32572=CARTESIAN_POINT('Ctrl Pts',(-0.712314141850511,16.7693165934297,
-12.));
#32573=CARTESIAN_POINT('Ctrl Pts',(-1.59035350544452,16.7320199121783,-3.99999999999998));
#32574=CARTESIAN_POINT('Ctrl Pts',(-2.4654486875042,16.6256211127011,3.99999999999999));
#32575=CARTESIAN_POINT('Ctrl Pts',(-3.32684344313022,16.4514279973581,12.));
#32576=CARTESIAN_POINT('Ctrl Pts',(-0.739569257475053,17.4109571784546,
-12.));
#32577=CARTESIAN_POINT('Ctrl Pts',(-1.65120484353838,17.3722334226862,-4.));
#32578=CARTESIAN_POINT('Ctrl Pts',(-2.55978359551225,17.2617635099015,4.));
#32579=CARTESIAN_POINT('Ctrl Pts',(-3.45413770472063,17.0809052826075,12.));
#32580=CARTESIAN_POINT('Ctrl Pts',(-0.657803912377567,15.4860354448028,
-11.9999999914697));
#32581=CARTESIAN_POINT('Ctrl Pts',(-0.860473336502316,15.4774266129281,
-10.0004173920443));
#32582=CARTESIAN_POINT('Ctrl Pts',(-1.06300270545654,15.4648379845811,-8.00054577305927));
#32583=CARTESIAN_POINT('Ctrl Pts',(-1.26527523936852,15.4482710543491,-5.99999995642121));
#32584=CARTESIAN_POINT('Ctrl Pts',(-1.46749908351692,15.4317081120036,-3.99993569850461));
#32585=CARTESIAN_POINT('Ctrl Pts',(-1.66937848149492,15.4111759584542,-2.00006422723887));
#32586=CARTESIAN_POINT('Ctrl Pts',(-1.87079645983396,15.3866864725929,1.8314671836973E-24));
#32587=CARTESIAN_POINT('Ctrl Pts',(-2.072214438173,15.3621969867316,2.00006422723887));
#32588=CARTESIAN_POINT('Ctrl Pts',(-2.2731321034333,15.3337548974327,3.99993569850461));
#32589=CARTESIAN_POINT('Ctrl Pts',(-2.47343304368529,15.301376702062,5.99999995642121));
#32590=CARTESIAN_POINT('Ctrl Pts',(-2.67381106285918,15.2689860470573,8.00083387021915));
#32591=CARTESIAN_POINT('Ctrl Pts',(-2.87345607543091,15.2326749819658,10.0007056240913));
#32592=CARTESIAN_POINT('Ctrl Pts',(-3.07225491560408,15.192473427738,11.9999999562994));
#32593=CARTESIAN_POINT('Origin',(2.22044604925031E-15,-4.16333634234434E-16,
-6.));
#32594=CARTESIAN_POINT('Origin',(2.22044604925031E-15,-4.16333634234434E-16,
-6.));
#32595=CARTESIAN_POINT('Ctrl Pts',(-0.559244210621343,15.4899078445247,
11.9999999562994));
#32596=CARTESIAN_POINT('Ctrl Pts',(-0.356553333306831,15.4972257725099,
10.0007056240913));
#32597=CARTESIAN_POINT('Ctrl Pts',(-0.153660607486406,15.5005673742223,
8.00083387021916));
#32598=CARTESIAN_POINT('Ctrl Pts',(0.0493174405869389,15.499921541416,5.99999995642122));
#32599=CARTESIAN_POINT('Ctrl Pts',(0.252217409591649,15.4992759570407,3.99993569850462));
#32600=CARTESIAN_POINT('Ctrl Pts',(0.455085414960353,15.4946463722799,2.00006422723887));
#32601=CARTESIAN_POINT('Ctrl Pts',(0.657803911807549,15.4860354517744,-2.22030256841817E-15));
#32602=CARTESIAN_POINT('Ctrl Pts',(0.860522408654744,15.4774245312688,-2.00006422723887));
#32603=CARTESIAN_POINT('Ctrl Pts',(1.06305225241292,15.4648339377712,-3.99993569850461));
#32604=CARTESIAN_POINT('Ctrl Pts',(1.26527609564327,15.4482709842168,-5.99999995642121));
#32605=CARTESIAN_POINT('Ctrl Pts',(1.46754862863696,15.4317040427731,-8.00054577305927));
#32606=CARTESIAN_POINT('Ctrl Pts',(1.66942723837633,15.4111700275214,-10.0004173920443));
#32607=CARTESIAN_POINT('Ctrl Pts',(1.87079645813716,15.3866864658071,-11.9999999914697));
#32608=CARTESIAN_POINT('Ctrl Pts',(4.67840257433451,14.7770954003634,-12.));
#32609=CARTESIAN_POINT('Ctrl Pts',(3.90467566848156,15.0220559863311,-4.));
#32610=CARTESIAN_POINT('Ctrl Pts',(3.11167798341369,15.2061210786984,4.));
#32611=CARTESIAN_POINT('Ctrl Pts',(2.30915666147617,15.3270282387598,12.));
#32612=CARTESIAN_POINT('Ctrl Pts',(4.87224514815724,15.3893621218603,-12.));
#32613=CARTESIAN_POINT('Ctrl Pts',(4.06646003173275,15.6444722812593,-4.));
#32614=CARTESIAN_POINT('Ctrl Pts',(3.240605680342,15.8361638338742,4.));
#32615=CARTESIAN_POINT('Ctrl Pts',(2.40483309451253,15.9620806002547,12.));
#32616=CARTESIAN_POINT('Ctrl Pts',(5.06608772197997,16.0016288433572,-12.));
#32617=CARTESIAN_POINT('Ctrl Pts',(4.22824439498395,16.2668885761874,-4.));
#32618=CARTESIAN_POINT('Ctrl Pts',(3.36953337727032,16.4662065890499,4.));
#32619=CARTESIAN_POINT('Ctrl Pts',(2.50050952754889,16.5971329617496,12.));
#32620=CARTESIAN_POINT('Ctrl Pts',(5.25993029580271,16.6138955648541,-12.));
#32621=CARTESIAN_POINT('Ctrl Pts',(4.39002875823515,16.8893048711156,-4.));
#32622=CARTESIAN_POINT('Ctrl Pts',(3.49846107419863,17.0962493442257,4.));
#32623=CARTESIAN_POINT('Ctrl Pts',(2.59618596058525,17.2321853232445,12.));
#32624=CARTESIAN_POINT('Ctrl Pts',(4.67840257999254,14.7770954211018,-11.9999999914697));
#32625=CARTESIAN_POINT('Ctrl Pts',(4.48501122377193,14.8383227908024,-10.0004173920443));
#32626=CARTESIAN_POINT('Ctrl Pts',(4.29039030580173,14.8957624734364,-8.00054577305927));
#32627=CARTESIAN_POINT('Ctrl Pts',(4.09465007444455,14.9493759323877,-5.99999995642121));
#32628=CARTESIAN_POINT('Ctrl Pts',(3.89895696043642,15.0029764858466,-3.99993569850461));
#32629=CARTESIAN_POINT('Ctrl Pts',(3.70222996976807,15.0527293932983,-2.00006422723887));
#32630=CARTESIAN_POINT('Ctrl Pts',(3.50458308436498,15.0986058099674,8.88178419700125E-15));
#32631=CARTESIAN_POINT('Ctrl Pts',(3.30693619896189,15.1444822266365,2.00006422723889));
#32632=CARTESIAN_POINT('Ctrl Pts',(3.10840758407279,15.1864732938717,3.99993569850461));
#32633=CARTESIAN_POINT('Ctrl Pts',(2.90911227356018,15.2245546989007,5.99999995642121));
#32634=CARTESIAN_POINT('Ctrl Pts',(2.70974027110769,15.2626507582476,8.00083387021915));
#32635=CARTESIAN_POINT('Ctrl Pts',(2.50971621033041,15.2968121341423,10.0007056240913));
#32636=CARTESIAN_POINT('Ctrl Pts',(2.30915666586,15.3270282380994,11.9999999562994));
#32637=CARTESIAN_POINT('Ctrl Pts',(5.10435222255114,16.662350757064,-10.5713320220547));
#32638=CARTESIAN_POINT('Ctrl Pts',(4.33577922443239,16.8977823962929,-3.52377734068488));
#32639=CARTESIAN_POINT('Ctrl Pts',(3.55089819699268,17.0799635066964,3.52377734068489));
#32640=CARTESIAN_POINT('Ctrl Pts',(2.75720126686291,17.2071550680903,10.5713320220547));
#32641=CARTESIAN_POINT('Ctrl Pts',(2.1033373682508,17.299259072917,-12.));
#32642=CARTESIAN_POINT('Ctrl Pts',(1.19755028131709,17.4093895599857,-4.));
#32643=CARTESIAN_POINT('Ctrl Pts',(0.283105004950508,17.4482326636193,4.));
#32644=CARTESIAN_POINT('Ctrl Pts',(-0.628758543704754,17.4153109432562,
12.));
#32645=CARTESIAN_POINT('Ctrl Pts',(2.02582373096846,16.6617348634049,-12.));
#32646=CARTESIAN_POINT('Ctrl Pts',(1.15341733358623,16.7678067459162,-4.00000000000002));
#32647=CARTESIAN_POINT('Ctrl Pts',(0.27267182433108,16.8052183767432,4.00000000000002));
#32648=CARTESIAN_POINT('Ctrl Pts',(-0.605587100820421,16.7735099102924,
12.));
#32649=CARTESIAN_POINT('Ctrl Pts',(1.94831009368611,16.0242106538928,-12.));
#32650=CARTESIAN_POINT('Ctrl Pts',(1.10928438585537,16.1262239318468,-3.99999999999998));
#32651=CARTESIAN_POINT('Ctrl Pts',(0.262238643711656,16.162204089867,3.99999999999999));
#32652=CARTESIAN_POINT('Ctrl Pts',(-0.582415657936089,16.1317088773286,
12.));
#32653=CARTESIAN_POINT('Ctrl Pts',(1.87079645640377,15.3866864443807,-12.));
#32654=CARTESIAN_POINT('Ctrl Pts',(1.0651514381245,15.4846411177773,-4.));
#32655=CARTESIAN_POINT('Ctrl Pts',(0.251805463092228,15.5191898029909,4.));
#32656=CARTESIAN_POINT('Ctrl Pts',(-0.559244215051757,15.4899078443647,
12.));
#32657=CARTESIAN_POINT('Ctrl Pts',(5.10435255326647,16.6623520957364,-10.5713320279724));
#32658=CARTESIAN_POINT('Ctrl Pts',(4.33578260855181,16.8977961637243,-3.52377734265748));
#32659=CARTESIAN_POINT('Ctrl Pts',(3.5509012234375,17.0799773571509,3.52377734265749));
#32660=CARTESIAN_POINT('Ctrl Pts',(2.75720155972776,17.2071564155546,10.5713320279724));
#32661=CARTESIAN_POINT('Ctrl Pts',(5.10446210897357,16.6627197582901,-10.5713320279724));
#32662=CARTESIAN_POINT('Ctrl Pts',(4.33587520540538,16.8981688796597,-3.52377734265747));
#32663=CARTESIAN_POINT('Ctrl Pts',(3.55097651134477,17.0803539511987,3.52377734265748));
#32664=CARTESIAN_POINT('Ctrl Pts',(2.75725935384223,17.2075356754217,10.5713320279724));
#32665=CARTESIAN_POINT('Ctrl Pts',(5.10457166468936,16.6630874208762,-10.5713320279724));
#32666=CARTESIAN_POINT('Ctrl Pts',(4.33596780226612,16.8985415956278,-3.52377734265749));
#32667=CARTESIAN_POINT('Ctrl Pts',(3.55105179925777,17.0807305452793,3.5237773426575));
#32668=CARTESIAN_POINT('Ctrl Pts',(2.75731714796087,17.2079149353218,10.5713320279724));
#32669=CARTESIAN_POINT('Ctrl Pts',(5.10468122040587,16.6634550834647,-10.5713320279724));
#32670=CARTESIAN_POINT('Ctrl Pts',(4.33606039912754,16.8989143115984,-3.52377734265748));
#32671=CARTESIAN_POINT('Ctrl Pts',(3.55112708717116,17.0811071393627,3.52377734265749));
#32672=CARTESIAN_POINT('Ctrl Pts',(2.75737494207986,17.2082941952246,10.5713320279724));
#32673=CARTESIAN_POINT('Ctrl Pts',(7.89318567151549,15.5366023477324,-12.));
#32674=CARTESIAN_POINT('Ctrl Pts',(7.07969107489245,15.94988858305,-4.));
#32675=CARTESIAN_POINT('Ctrl Pts',(6.23367872045024,16.2991478653893,4.));
#32676=CARTESIAN_POINT('Ctrl Pts',(5.36554738109813,16.5800872693051,12.));
#32677=CARTESIAN_POINT('Ctrl Pts',(7.60230055704008,14.9640367778145,-12.));
#32678=CARTESIAN_POINT('Ctrl Pts',(6.81878542355292,15.3620923041542,-4.00000000000001));
#32679=CARTESIAN_POINT('Ctrl Pts',(6.00395089905301,15.6984804428827,4.00000000000001));
#32680=CARTESIAN_POINT('Ctrl Pts',(5.16781253370865,15.9690664743998,12.));
#32681=CARTESIAN_POINT('Ctrl Pts',(7.31141544256466,14.3914712078966,-12.));
#32682=CARTESIAN_POINT('Ctrl Pts',(6.55787977221338,14.7742960252583,-4.));
#32683=CARTESIAN_POINT('Ctrl Pts',(5.77422307765577,15.0978130203761,3.99999999999999));
#32684=CARTESIAN_POINT('Ctrl Pts',(4.97007768631916,15.3580456794946,12.));
#32685=CARTESIAN_POINT('Ctrl Pts',(7.02053032808925,13.8189056379787,-12.));
#32686=CARTESIAN_POINT('Ctrl Pts',(6.29697412087384,14.1864997463625,-4.));
#32687=CARTESIAN_POINT('Ctrl Pts',(5.54449525625854,14.4971455978694,4.));
#32688=CARTESIAN_POINT('Ctrl Pts',(4.77234283892968,14.7470248845893,12.));
#32689=CARTESIAN_POINT('Ctrl Pts',(4.77234284314764,14.7470248832244,11.9999999562994));
#32690=CARTESIAN_POINT('Ctrl Pts',(4.96531284363905,14.6845771232416,10.0007056240913));
#32691=CARTESIAN_POINT('Ctrl Pts',(5.15711253600028,14.6183238025476,8.00083387021916));
#32692=CARTESIAN_POINT('Ctrl Pts',(5.34762862212736,14.5482943371312,5.99999995642122));
#32693=CARTESIAN_POINT('Ctrl Pts',(5.53807142289819,14.4782918097778,3.99993569850461));
#32694=CARTESIAN_POINT('Ctrl Pts',(5.72712157929327,14.4045564788684,2.00006422723889));
#32695=CARTESIAN_POINT('Ctrl Pts',(5.91466954661191,14.3271310510647,-2.22058953008253E-15));
#32696=CARTESIAN_POINT('Ctrl Pts',(6.10221751393055,14.249705623261,-2.00006422723888));
#32697=CARTESIAN_POINT('Ctrl Pts',(6.28822707700645,14.1686050492701,-3.9999356985046));
#32698=CARTESIAN_POINT('Ctrl Pts',(6.47259046648839,14.0838763361911,-5.99999995642121));
#32699=CARTESIAN_POINT('Ctrl Pts',(6.6569982454432,13.9991272228421,-8.00054577305927));
#32700=CARTESIAN_POINT('Ctrl Pts',(6.83967903847032,13.9107850091975,-10.0004173920443));
#32701=CARTESIAN_POINT('Ctrl Pts',(7.0205303370464,13.8189056575201,-11.9999999914697));
#32702=CARTESIAN_POINT('Ctrl Pts',(9.4503246629373,12.2858195853618,-12.));
#32703=CARTESIAN_POINT('Ctrl Pts',(8.8070406537256,12.7806374276138,-4.));
#32704=CARTESIAN_POINT('Ctrl Pts',(8.12482055003974,13.2248232185595,4.));
#32705=CARTESIAN_POINT('Ctrl Pts',(7.41204987000498,13.6129172422203,12.));
#32706=CARTESIAN_POINT('Ctrl Pts',(9.84188465099258,12.7948640406238,-12.));
#32707=CARTESIAN_POINT('Ctrl Pts',(9.17194713643085,13.3101839159077,-4.));
#32708=CARTESIAN_POINT('Ctrl Pts',(8.4614602688847,13.7727738769957,4.));
#32709=CARTESIAN_POINT('Ctrl Pts',(7.71915700781016,14.1769479927898,12.));
#32710=CARTESIAN_POINT('Ctrl Pts',(10.2334446390479,13.3039084958857,-12.));
#32711=CARTESIAN_POINT('Ctrl Pts',(9.53685361913611,13.8397304042016,-4.00000000000001));
#32712=CARTESIAN_POINT('Ctrl Pts',(8.79809998772967,14.3207245354319,4.00000000000001));
#32713=CARTESIAN_POINT('Ctrl Pts',(8.02626414561533,14.7409787433592,12.));
#32714=CARTESIAN_POINT('Ctrl Pts',(10.6250046271031,13.8129529511477,-12.));
#32715=CARTESIAN_POINT('Ctrl Pts',(9.90176010184136,14.3692768924954,-4.));
#32716=CARTESIAN_POINT('Ctrl Pts',(9.13473970657463,14.8686751938681,4.));
#32717=CARTESIAN_POINT('Ctrl Pts',(8.3333712834205,15.3050094939286,12.));
#32718=CARTESIAN_POINT('Ctrl Pts',(9.45032467534708,12.2858196029144,-11.9999999914697));
#32719=CARTESIAN_POINT('Ctrl Pts',(9.28953723874319,12.4094982497846,-10.0004173920443));
#32720=CARTESIAN_POINT('Ctrl Pts',(9.12629892676312,12.5300381699545,-8.00054577305927));
#32721=CARTESIAN_POINT('Ctrl Pts',(8.96070015868055,12.6473654436892,-5.99999995642121));
#32722=CARTESIAN_POINT('Ctrl Pts',(8.79514125248487,12.7646644751455,-3.9999356985046));
#32723=CARTESIAN_POINT('Ctrl Pts',(8.62729484758191,12.8787015086849,-2.00006422723888));
#32724=CARTESIAN_POINT('Ctrl Pts',(8.45725818645174,12.9894104549704,-2.22044604925031E-15));
#32725=CARTESIAN_POINT('Ctrl Pts',(8.28722152532158,13.1001194012559,2.00006422723888));
#32726=CARTESIAN_POINT('Ctrl Pts',(8.11502744172963,13.2074788825944,3.9999356985046));
#32727=CARTESIAN_POINT('Ctrl Pts',(7.94077571668976,13.311426708555,5.99999995642122));
#32728=CARTESIAN_POINT('Ctrl Pts',(7.76645693687179,13.4154145352581,8.00083387021915));
#32729=CARTESIAN_POINT('Ctrl Pts',(7.59017968165941,13.5159279860378,10.0007056240913));
#32730=CARTESIAN_POINT('Ctrl Pts',(7.41204987389855,13.6129172401003,11.9999999562994));
#32731=CARTESIAN_POINT('Ctrl Pts',(10.4953817114971,13.9116967726179,-10.5713320220547));
#32732=CARTESIAN_POINT('Ctrl Pts',(9.85368169962204,14.3957975936737,-3.52377734068489));
#32733=CARTESIAN_POINT('Ctrl Pts',(9.17844439943351,14.8354369602649,3.52377734068489));
#32734=CARTESIAN_POINT('Ctrl Pts',(8.47611532710788,15.2264182697331,10.5713320220547));
#32735=CARTESIAN_POINT('Ctrl Pts',(10.4953824801207,13.9116979174471,-10.5713320279724));
#32736=CARTESIAN_POINT('Ctrl Pts',(9.85368958839295,14.3958093733904,-3.52377734265747));
#32737=CARTESIAN_POINT('Ctrl Pts',(9.1784519804958,14.8354489403297,3.52377734265748));
#32738=CARTESIAN_POINT('Ctrl Pts',(8.47611606317077,15.2264194357697,10.5713320279724));
#32739=CARTESIAN_POINT('Ctrl Pts',(10.4956111768049,13.912005936971,-10.5713320279724));
#32740=CARTESIAN_POINT('Ctrl Pts',(9.85390407732624,14.3961279418089,-3.52377734265748));
#32741=CARTESIAN_POINT('Ctrl Pts',(9.17865153073284,14.8357770729899,3.52377734265748));
#32742=CARTESIAN_POINT('Ctrl Pts',(8.47630008638401,15.22675605671,10.5713320279724));
#32743=CARTESIAN_POINT('Ctrl Pts',(10.4958398735083,13.9123139565221,-10.5713320279724));
#32744=CARTESIAN_POINT('Ctrl Pts',(9.85411856627743,14.3964465102557,-3.52377734265747));
#32745=CARTESIAN_POINT('Ctrl Pts',(9.17885108098651,14.8361052056791,3.52377734265748));
#32746=CARTESIAN_POINT('Ctrl Pts',(8.47648410961248,15.22709267768,10.5713320279724));
#32747=CARTESIAN_POINT('Ctrl Pts',(10.4960685702133,13.9126219760754,-10.5713320279724));
#32748=CARTESIAN_POINT('Ctrl Pts',(9.85433305523014,14.3967650787046,-3.52377734265747));
#32749=CARTESIAN_POINT('Ctrl Pts',(9.17905063124145,14.8364333383706,3.52377734265748));
#32750=CARTESIAN_POINT('Ctrl Pts',(8.47666813284218,15.2274292986523,10.5713320279724));
#32751=CARTESIAN_POINT('Origin',(2.22044604925031E-15,-4.16333634234434E-16,
-6.));
#32752=CARTESIAN_POINT('Ctrl Pts',(9.52831491775384,12.2254330780995,11.9999999562994));
#32753=CARTESIAN_POINT('Ctrl Pts',(9.68828901142903,12.1007517516335,10.0007056240913));
#32754=CARTESIAN_POINT('Ctrl Pts',(9.84586179677031,11.9728946368036,8.00083387021915));
#32755=CARTESIAN_POINT('Ctrl Pts',(10.0009368692462,11.8419281258312,5.99999995642121));
#32756=CARTESIAN_POINT('Ctrl Pts',(10.1559522893738,11.7110119934259,3.99993569850462));
#32757=CARTESIAN_POINT('Ctrl Pts',(10.3083823578509,11.5770644854931,2.00006422723886));
#32758=CARTESIAN_POINT('Ctrl Pts',(10.4581387428691,11.440163199662,-6.66133814775096E-15));
#32759=CARTESIAN_POINT('Ctrl Pts',(10.6078951278873,11.3032619138309,-2.0000642272389));
#32760=CARTESIAN_POINT('Ctrl Pts',(10.7549489117653,11.1634332854871,-3.9999356985046));
#32761=CARTESIAN_POINT('Ctrl Pts',(10.8992149018134,11.0207583461433,-5.99999995642121));
#32762=CARTESIAN_POINT('Ctrl Pts',(11.0435156270184,10.8780490547226,-8.00054577305927));
#32763=CARTESIAN_POINT('Ctrl Pts',(11.1849646036129,10.732554017443,-10.0004173920443));
#32764=CARTESIAN_POINT('Ctrl Pts',(11.323484645315,10.5843608816095,-11.9999999914697));
#32765=CARTESIAN_POINT('Ctrl Pts',(12.7309992917815,11.9000020835813,-12.));
#32766=CARTESIAN_POINT('Ctrl Pts',(12.1079166397235,12.5665956477133,-4.));
#32767=CARTESIAN_POINT('Ctrl Pts',(11.432378782964,13.1841452847902,4.));
#32768=CARTESIAN_POINT('Ctrl Pts',(10.7126891046949,13.7450603746485,12.));
#32769=CARTESIAN_POINT('Ctrl Pts',(12.2618277379259,11.4614550111576,-12.));
#32770=CARTESIAN_POINT('Ctrl Pts',(11.6617073568841,12.1034828101751,-3.99999999999999));
#32771=CARTESIAN_POINT('Ctrl Pts',(11.011064886471,12.6982740827144,3.99999999999999));
#32772=CARTESIAN_POINT('Ctrl Pts',(10.3178977078823,13.238517943374,12.));
#32773=CARTESIAN_POINT('Ctrl Pts',(11.7926561840702,11.0229079387338,-12.));
#32774=CARTESIAN_POINT('Ctrl Pts',(11.2154980740448,11.6403699726369,-4.00000000000001));
#32775=CARTESIAN_POINT('Ctrl Pts',(10.589750989978,12.2124028806386,4.00000000000001));
#32776=CARTESIAN_POINT('Ctrl Pts',(9.92310631106972,12.7319755120994,12.));
#32777=CARTESIAN_POINT('Ctrl Pts',(11.3234846302145,10.5843608663101,-12.));
#32778=CARTESIAN_POINT('Ctrl Pts',(10.7692887912054,11.1772571350987,-4.));
#32779=CARTESIAN_POINT('Ctrl Pts',(10.168437093485,11.7265316785628,4.));
#32780=CARTESIAN_POINT('Ctrl Pts',(9.52831491425713,12.2254330808248,12.));
#32781=CARTESIAN_POINT('Ctrl Pts',(14.6205143845238,9.48308765551917,-10.5713320279724));
#32782=CARTESIAN_POINT('Ctrl Pts',(14.1830961789038,10.1574755131067,-3.52377734265748));
#32783=CARTESIAN_POINT('Ctrl Pts',(13.6989459691819,10.801546433397,3.52377734265748));
#32784=CARTESIAN_POINT('Ctrl Pts',(13.1726858752452,11.4091515540133,10.5713320279724));
#32785=CARTESIAN_POINT('Ctrl Pts',(14.6208346379986,9.48329888032434,-10.5713320279724));
#32786=CARTESIAN_POINT('Ctrl Pts',(14.1834066893941,10.1577015099677,-3.52377734265748));
#32787=CARTESIAN_POINT('Ctrl Pts',(13.6992457130527,10.8017865270407,3.52377734265748));
#32788=CARTESIAN_POINT('Ctrl Pts',(13.1729739316488,11.4094049345862,10.5713320279724));
#32789=CARTESIAN_POINT('Ctrl Pts',(14.6211548915007,9.48351010514861,-10.5713320279724));
#32790=CARTESIAN_POINT('Ctrl Pts',(14.1837171999109,10.1579275068491,-3.52377734265747));
#32791=CARTESIAN_POINT('Ctrl Pts',(13.699545456949,10.8020266207058,3.52377734265748));
#32792=CARTESIAN_POINT('Ctrl Pts',(13.1732619880769,11.4096583151819,10.5713320279724));
#32793=CARTESIAN_POINT('Ctrl Pts',(14.621475145005,9.48372132997438,-10.5713320279724));
#32794=CARTESIAN_POINT('Ctrl Pts',(14.1840277104299,10.1581535037321,-3.52377734265748));
#32795=CARTESIAN_POINT('Ctrl Pts',(13.6998452008473,10.8022667143728,3.52377734265748));
#32796=CARTESIAN_POINT('Ctrl Pts',(13.173550044507,11.4099116957793,10.5713320279724));
#32797=CARTESIAN_POINT('Ctrl Pts',(14.6205132701638,9.48308684344182,-10.5713320134285));
#32798=CARTESIAN_POINT('Ctrl Pts',(14.183084736767,10.1574671421628,-3.52377733780948));
#32799=CARTESIAN_POINT('Ctrl Pts',(13.6989347480705,10.8015377684169,3.52377733780958));
#32800=CARTESIAN_POINT('Ctrl Pts',(13.1726847854084,11.4091507093019,10.5713320134286));
#32801=CARTESIAN_POINT('Ctrl Pts',(13.082398125252,8.31269260897954,-12.));
#32802=CARTESIAN_POINT('Ctrl Pts',(12.6471465580533,8.99768537300669,-4.));
#32803=CARTESIAN_POINT('Ctrl Pts',(12.1579898487504,9.64841650065859,4.));
#32804=CARTESIAN_POINT('Ctrl Pts',(11.6209404740055,10.2568875210076,12.));
#32805=CARTESIAN_POINT('Ctrl Pts',(13.6244476141704,8.65711652400593,-12.));
#32806=CARTESIAN_POINT('Ctrl Pts',(13.1711620529523,9.37049093290421,-4.));
#32807=CARTESIAN_POINT('Ctrl Pts',(12.6617378711462,10.0481841260574,3.99999999999999));
#32808=CARTESIAN_POINT('Ctrl Pts',(12.1024366633415,10.6818662279256,12.));
#32809=CARTESIAN_POINT('Ctrl Pts',(14.1664971030888,9.00154043903231,-12.));
#32810=CARTESIAN_POINT('Ctrl Pts',(13.6951775478512,9.74329649280173,-4.00000000000002));
#32811=CARTESIAN_POINT('Ctrl Pts',(13.165485893542,10.4479517514562,4.00000000000001));
#32812=CARTESIAN_POINT('Ctrl Pts',(12.5839328526776,11.1068449348435,12.));
#32813=CARTESIAN_POINT('Ctrl Pts',(14.7085465920072,9.3459643540587,-12.));
#32814=CARTESIAN_POINT('Ctrl Pts',(14.2191930427502,10.1161020526992,-4.));
#32815=CARTESIAN_POINT('Ctrl Pts',(13.6692339159378,10.847719376855,4.));
#32816=CARTESIAN_POINT('Ctrl Pts',(13.0654290420136,11.5318236417615,12.));
#32817=CARTESIAN_POINT('Ctrl Pts',(13.0823981429167,8.31269262122918,-11.9999999914697));
#32818=CARTESIAN_POINT('Ctrl Pts',(12.9736079637539,8.48390507515421,-10.0004173920443));
#32819=CARTESIAN_POINT('Ctrl Pts',(12.8614412073296,8.65300633950756,-8.00054577305927));
#32820=CARTESIAN_POINT('Ctrl Pts',(12.7459575579299,8.81989602724713,-5.99999995642121));
#32821=CARTESIAN_POINT('Ctrl Pts',(12.630501707023,8.98674554235783,-3.99993569850462));
#32822=CARTESIAN_POINT('Ctrl Pts',(12.5117806414659,9.1513121527328,-2.00006422723887));
#32823=CARTESIAN_POINT('Ctrl Pts',(12.3898631354148,9.31350049582264,-1.43482765123828E-19));
#32824=CARTESIAN_POINT('Ctrl Pts',(12.2679456293637,9.47568883891247,2.00006422723888));
#32825=CARTESIAN_POINT('Ctrl Pts',(12.1428552248642,9.63546759644758,3.9999356985046));
#32826=CARTESIAN_POINT('Ctrl Pts',(12.0146644150184,9.79274420142234,5.99999995642121));
#32827=CARTESIAN_POINT('Ctrl Pts',(11.8864242753522,9.95008132888459,8.00083387021915));
#32828=CARTESIAN_POINT('Ctrl Pts',(11.7551554642586,10.1048234489648,10.0007056240913));
#32829=CARTESIAN_POINT('Ctrl Pts',(11.6209404769392,10.2568875176838,11.9999999562994));
#32830=CARTESIAN_POINT('Origin',(2.22044604925031E-15,-4.16333634234434E-16,
-6.));
#32831=CARTESIAN_POINT('Origin',(2.22044604925031E-15,-4.16333634234434E-16,
-6.));
#32832=CARTESIAN_POINT('Ctrl Pts',(13.1350315903275,8.2292736155798,11.9999999562994));
#32833=CARTESIAN_POINT('Ctrl Pts',(13.2427145405231,8.05739713070271,10.0007056240913));
#32834=CARTESIAN_POINT('Ctrl Pts',(13.3470548154056,7.88335767675537,8.00083387021915));
#32835=CARTESIAN_POINT('Ctrl Pts',(13.4479845318255,7.70725061431013,5.99999995642122));
#32836=CARTESIAN_POINT('Ctrl Pts',(13.5488754238585,7.53121129453729,3.99993569850461));
#32837=CARTESIAN_POINT('Ctrl Pts',(13.646300088531,7.35320765589252,2.00006422723887));
#32838=CARTESIAN_POINT('Ctrl Pts',(13.7402020610468,7.17334282755306,-6.66133814775094E-15));
#32839=CARTESIAN_POINT('Ctrl Pts',(13.8341040335626,6.9934779992136,-2.00006422723889));
#32840=CARTESIAN_POINT('Ctrl Pts',(13.9244651816241,6.81178671274576,-3.9999356985046));
#32841=CARTESIAN_POINT('Ctrl Pts',(14.0112331646994,6.62837425048013,-5.99999995642121));
#32842=CARTESIAN_POINT('Ctrl Pts',(14.098022039043,6.44491762769792,-8.00054577305927));
#32843=CARTESIAN_POINT('Ctrl Pts',(14.181178365063,6.25981861555709,-10.0004173920443));
#32844=CARTESIAN_POINT('Ctrl Pts',(14.2606595885237,6.07318597484681,-11.9999999914697));
#32845=CARTESIAN_POINT('Ctrl Pts',(15.1365412980281,3.33693222167749,-12.));
#32846=CARTESIAN_POINT('Ctrl Pts',(14.9618199354756,4.12947967072155,-4.));
#32847=CARTESIAN_POINT('Ctrl Pts',(14.7247261388817,4.90826835731624,4.));
#32848=CARTESIAN_POINT('Ctrl Pts',(14.4281741500255,5.66372578922348,12.));
#32849=CARTESIAN_POINT('Ctrl Pts',(15.7637011196476,3.4751929891605,-12.));
#32850=CARTESIAN_POINT('Ctrl Pts',(15.5817404402384,4.300578449675,-3.99999999999999));
#32851=CARTESIAN_POINT('Ctrl Pts',(15.3348230187984,5.11163507411277,3.99999999999999));
#32852=CARTESIAN_POINT('Ctrl Pts',(15.0259838443316,5.89839374841796,12.));
#32853=CARTESIAN_POINT('Ctrl Pts',(16.3908609412671,3.61345375664351,-12.));
#32854=CARTESIAN_POINT('Ctrl Pts',(16.2016609450012,4.47167722862846,-4.00000000000001));
#32855=CARTESIAN_POINT('Ctrl Pts',(15.9449198987151,5.31500179090931,4.00000000000001));
#32856=CARTESIAN_POINT('Ctrl Pts',(15.6237935386377,6.13306170761243,12.));
#32857=CARTESIAN_POINT('Ctrl Pts',(17.0180207628866,3.75171452412652,-12.));
#32858=CARTESIAN_POINT('Ctrl Pts',(16.8215814497639,4.64277600758191,-4.));
#32859=CARTESIAN_POINT('Ctrl Pts',(16.5550167786318,5.51836850770584,4.));
#32860=CARTESIAN_POINT('Ctrl Pts',(16.2216032329437,6.36772966680691,12.));
#32861=CARTESIAN_POINT('Ctrl Pts',(15.1365413188172,3.33693222714671,-11.9999999914697));
#32862=CARTESIAN_POINT('Ctrl Pts',(15.0928700982745,3.53502773935638,-10.0004173920443));
#32863=CARTESIAN_POINT('Ctrl Pts',(15.0453038636357,3.73229423974341,-8.00054577305927));
#32864=CARTESIAN_POINT('Ctrl Pts',(14.9938643653936,3.92861698211701,-5.99999995642121));
#32865=CARTESIAN_POINT('Ctrl Pts',(14.9424372493419,4.12489246692319,-3.99993569850461));
#32866=CARTESIAN_POINT('Ctrl Pts',(14.8871610357731,4.32013949217793,-2.00006422723889));
#32867=CARTESIAN_POINT('Ctrl Pts',(14.8280677353416,4.51424492425044,-6.66133814775094E-15));
#32868=CARTESIAN_POINT('Ctrl Pts',(14.7689744349101,4.70835035632295,2.00006422723887));
#32869=CARTESIAN_POINT('Ctrl Pts',(14.7060754584233,4.90127671381265,3.9999356985046));
#32870=CARTESIAN_POINT('Ctrl Pts',(14.6394072673339,5.09291221808618,5.99999995642121));
#32871=CARTESIAN_POINT('Ctrl Pts',(14.5727134212861,5.28462146668684,8.00083387021915));
#32872=CARTESIAN_POINT('Ctrl Pts',(14.5022860102504,5.47492807263538,10.0007056240913));
#32873=CARTESIAN_POINT('Ctrl Pts',(14.4281741516455,5.66372578509675,11.9999999562994));
#32874=CARTESIAN_POINT('Ctrl Pts',(16.9821951536599,3.91067668393918,-10.5713320220547));
#32875=CARTESIAN_POINT('Ctrl Pts',(16.8017984350274,4.69399624458723,-3.52377734068488));
#32876=CARTESIAN_POINT('Ctrl Pts',(16.5671313910066,5.46481370850019,3.52377734068489));
#32877=CARTESIAN_POINT('Ctrl Pts',(16.2804340492558,6.21577119359523,10.5713320220547));
#32878=CARTESIAN_POINT('Ctrl Pts',(16.03326650792,6.82808594282421,-12.));
#32879=CARTESIAN_POINT('Ctrl Pts',(15.6757487639857,7.66758581406302,-4.));
#32880=CARTESIAN_POINT('Ctrl Pts',(15.252165240311,8.478940205584,4.));
#32881=CARTESIAN_POINT('Ctrl Pts',(14.7677224198127,9.25217634332295,12.));
#32882=CARTESIAN_POINT('Ctrl Pts',(15.4423975283137,6.5764526170944,-12.));
#32883=CARTESIAN_POINT('Ctrl Pts',(15.0980552745046,7.38501466090712,-4.00000000000002));
#32884=CARTESIAN_POINT('Ctrl Pts',(14.6900819425702,8.16646846160462,4.00000000000002));
#32885=CARTESIAN_POINT('Ctrl Pts',(14.223492142533,8.91120876866085,12.));
#32886=CARTESIAN_POINT('Ctrl Pts',(14.8515285487075,6.32481929136458,-12.));
#32887=CARTESIAN_POINT('Ctrl Pts',(14.5203617850236,7.10244350775122,-3.99999999999999));
#32888=CARTESIAN_POINT('Ctrl Pts',(14.1279986448294,7.85399671762524,3.99999999999999));
#32889=CARTESIAN_POINT('Ctrl Pts',(13.6792618652534,8.57024119399876,12.));
#32890=CARTESIAN_POINT('Ctrl Pts',(14.2606595691012,6.07318596563476,-12.));
#32891=CARTESIAN_POINT('Ctrl Pts',(13.9426682955425,6.81987235459531,-4.));
#32892=CARTESIAN_POINT('Ctrl Pts',(13.5659153470886,7.54152497364586,4.));
#32893=CARTESIAN_POINT('Ctrl Pts',(13.1350315879738,8.22927361933667,12.));
#32894=CARTESIAN_POINT('Ctrl Pts',(16.9821964783418,3.91067706686746,-10.5713320279724));
#32895=CARTESIAN_POINT('Ctrl Pts',(16.8018120500324,4.69400019756955,-3.52377734265747));
#32896=CARTESIAN_POINT('Ctrl Pts',(16.5671448990744,5.46481801274934,3.52377734265748));
#32897=CARTESIAN_POINT('Ctrl Pts',(16.2804353626266,6.215771613699,10.5713320279724));
#32898=CARTESIAN_POINT('Ctrl Pts',(16.982569661307,3.91076602011887,-10.5713320279724));
#32899=CARTESIAN_POINT('Ctrl Pts',(16.8021811299277,4.69410636430973,-3.52377734265748));
#32900=CARTESIAN_POINT('Ctrl Pts',(16.5675086830403,5.46494110853292,3.52377734265749));
#32901=CARTESIAN_POINT('Ctrl Pts',(16.2807927083633,6.21591119246119,10.5713320279724));
#32902=CARTESIAN_POINT('Ctrl Pts',(16.9829428443044,3.91085497337887,-10.5713320279724));
#32903=CARTESIAN_POINT('Ctrl Pts',(16.8025502098547,4.69421253106005,-3.52377734265747));
#32904=CARTESIAN_POINT('Ctrl Pts',(16.5678724670376,5.46506420432801,3.52377734265747));
#32905=CARTESIAN_POINT('Ctrl Pts',(16.2811500541308,6.21605077123634,10.5713320279724));
#32906=CARTESIAN_POINT('Ctrl Pts',(16.9833160273043,3.91094392663953,-10.5713320279724));
#32907=CARTESIAN_POINT('Ctrl Pts',(16.8029192897844,4.69431869781105,-3.52377734265747));
#32908=CARTESIAN_POINT('Ctrl Pts',(16.5682362510374,5.46518730012407,3.52377734265748));
#32909=CARTESIAN_POINT('Ctrl Pts',(16.2815073999007,6.2161903500125,10.5713320279724));
#32910=CARTESIAN_POINT('Ctrl Pts',(17.401685157391,0.93260186554647,-12.));
#32911=CARTESIAN_POINT('Ctrl Pts',(17.3528542378989,1.84375196972217,-4.));
#32912=CARTESIAN_POINT('Ctrl Pts',(17.2323154716912,2.75104980175429,4.));
#32913=CARTESIAN_POINT('Ctrl Pts',(17.0415504627302,3.64334329741251,12.));
#32914=CARTESIAN_POINT('Ctrl Pts',(16.760386271272,0.898232979305968,-12.));
#32915=CARTESIAN_POINT('Ctrl Pts',(16.7133549024554,1.77580475232523,-3.99999999999999));
#32916=CARTESIAN_POINT('Ctrl Pts',(16.5972583138761,2.64966621978703,4.));
#32917=CARTESIAN_POINT('Ctrl Pts',(16.413523508407,3.50907630101261,12.));
#32918=CARTESIAN_POINT('Ctrl Pts',(16.1190873851531,0.863864093065467,-12.));
#32919=CARTESIAN_POINT('Ctrl Pts',(16.0738555670119,1.70785753492828,-4.00000000000001));
#32920=CARTESIAN_POINT('Ctrl Pts',(15.962201156061,2.54828263781977,4.00000000000001));
#32921=CARTESIAN_POINT('Ctrl Pts',(15.7854965540837,3.37480930461272,12.));
#32922=CARTESIAN_POINT('Ctrl Pts',(15.4777884990342,0.829495206824966,-12.));
#32923=CARTESIAN_POINT('Ctrl Pts',(15.4343562315684,1.63991031753134,-4.));
#32924=CARTESIAN_POINT('Ctrl Pts',(15.3271439982459,2.44689905585252,4.));
#32925=CARTESIAN_POINT('Ctrl Pts',(15.1574695997605,3.24054230821282,12.));
#32926=CARTESIAN_POINT('Ctrl Pts',(15.1574696006874,3.24054230387749,11.9999999562994));
#32927=CARTESIAN_POINT('Ctrl Pts',(15.1998732543785,3.04220150129224,10.0007056240913));
#32928=CARTESIAN_POINT('Ctrl Pts',(15.2383960417531,2.84297143492237,8.00083387021915));
#32929=CARTESIAN_POINT('Ctrl Pts',(15.2730067887526,2.64296493179857,5.99999995642122));
#32930=CARTESIAN_POINT('Ctrl Pts',(15.3076042221209,2.44303536468648,3.99993569850461));
#32931=CARTESIAN_POINT('Ctrl Pts',(15.3382726305943,2.24244546120418,2.00006422723887));
#32932=CARTESIAN_POINT('Ctrl Pts',(15.3649942268768,2.04131144317626,-2.22044604741885E-15));
#32933=CARTESIAN_POINT('Ctrl Pts',(15.3917158231593,1.84017742514833,-2.00006422723887));
#32934=CARTESIAN_POINT('Ctrl Pts',(15.4144854473596,1.63853813118233,-3.99993569850461));
#32935=CARTESIAN_POINT('Ctrl Pts',(15.4332899241442,1.43651039582365,-5.99999995642121));
#32936=CARTESIAN_POINT('Ctrl Pts',(15.4520989285132,1.23443401791883,-8.00054577305927));
#32937=CARTESIAN_POINT('Ctrl Pts',(15.466932723784,1.03205670355153,-10.0004173920443));
#32938=CARTESIAN_POINT('Ctrl Pts',(15.4777885204361,0.829495208838567,-11.9999999914697));
#32939=CARTESIAN_POINT('Ctrl Pts',(15.3649941987044,-2.04131143943342,-12.));
#32940=CARTESIAN_POINT('Ctrl Pts',(15.4718770157346,-1.23680222448176,-4.));
#32941=CARTESIAN_POINT('Ctrl Pts',(15.5154431428507,-0.423889388244508,
4.));
#32942=CARTESIAN_POINT('Ctrl Pts',(15.4951570863805,0.387435139568705,12.));
#32943=CARTESIAN_POINT('Ctrl Pts',(16.0016196226445,-2.12589010856384,-12.));
#32944=CARTESIAN_POINT('Ctrl Pts',(16.1129309684345,-1.2880472643632,-3.99999999999999));
#32945=CARTESIAN_POINT('Ctrl Pts',(16.1583021924993,-0.441452607468999,
3.99999999999999));
#32946=CARTESIAN_POINT('Ctrl Pts',(16.1371756137918,0.403487931830613,12.));
#32947=CARTESIAN_POINT('Ctrl Pts',(16.6382450465846,-2.21046877769426,-12.));
#32948=CARTESIAN_POINT('Ctrl Pts',(16.7539849211345,-1.33929230424465,-4.00000000000001));
#32949=CARTESIAN_POINT('Ctrl Pts',(16.801161242148,-0.459015826693489,4.00000000000001));
#32950=CARTESIAN_POINT('Ctrl Pts',(16.7791941412031,0.419540724092521,12.));
#32951=CARTESIAN_POINT('Ctrl Pts',(17.2748704705247,-2.29504744682469,-12.));
#32952=CARTESIAN_POINT('Ctrl Pts',(17.3950388738344,-1.39053734412609,-4.));
#32953=CARTESIAN_POINT('Ctrl Pts',(17.4440202917966,-0.47657904591798,4.));
#32954=CARTESIAN_POINT('Ctrl Pts',(17.4212126686144,0.435593516354429,12.));
#32955=CARTESIAN_POINT('Ctrl Pts',(17.2955736705817,-2.13341879826209,-10.5713320220547));
#32956=CARTESIAN_POINT('Ctrl Pts',(17.3939672736713,-1.33563987584167,-3.52377734068488));
#32957=CARTESIAN_POINT('Ctrl Pts',(17.4370874835488,-0.531047536999956,
3.52377734068489));
#32958=CARTESIAN_POINT('Ctrl Pts',(17.4245226937903,0.272677936184493,10.5713320220547));
#32959=CARTESIAN_POINT('Ctrl Pts',(17.2955750463447,-2.1334188914951,-10.5713320279724));
#32960=CARTESIAN_POINT('Ctrl Pts',(17.3939814195907,-1.33564081785934,-3.52377734265747));
#32961=CARTESIAN_POINT('Ctrl Pts',(17.4371016491204,-0.531048112360096,
3.52377734265748));
#32962=CARTESIAN_POINT('Ctrl Pts',(17.4245240716391,0.272677881753644,10.5713320279724));
#32963=CARTESIAN_POINT('Ctrl Pts',(17.295956147427,-2.13346293887238,-10.5713320279724));
#32964=CARTESIAN_POINT('Ctrl Pts',(17.3943645524084,-1.33566728651567,-3.52377734265748));
#32965=CARTESIAN_POINT('Ctrl Pts',(17.4374855954662,-0.531056861604771,
3.52377734265749));
#32966=CARTESIAN_POINT('Ctrl Pts',(17.4249076055392,0.272686823446403,10.5713320279724));
#32967=CARTESIAN_POINT('Ctrl Pts',(17.2963372485426,-2.13350698625262,-10.5713320279724));
#32968=CARTESIAN_POINT('Ctrl Pts',(17.3947476852595,-1.33569375517339,-3.52377734265746));
#32969=CARTESIAN_POINT('Ctrl Pts',(17.4378695418455,-0.531065610849369,
3.52377734265747));
#32970=CARTESIAN_POINT('Ctrl Pts',(17.4252911394727,0.27269576514082,10.5713320279724));
#32971=CARTESIAN_POINT('Ctrl Pts',(17.2967183496608,-2.13355103363312,-10.5713320279724));
#32972=CARTESIAN_POINT('Ctrl Pts',(17.3951308181133,-1.33572022383133,-3.52377734265747));
#32973=CARTESIAN_POINT('Ctrl Pts',(17.4382534882275,-0.531074360093895,
3.52377734265748));
#32974=CARTESIAN_POINT('Ctrl Pts',(17.4256746734088,0.272704706835342,10.5713320279724));
#32975=CARTESIAN_POINT('Origin',(2.22044604925031E-15,-4.16333634234434E-16,
-6.));
#88463=UNCERTAINTY_MEASURE_WITH_UNIT(LENGTH_MEASURE(0.01),#88484,
'DISTANCE_ACCURACY_VALUE',
'Maximum model space distance between geometric entities at asserted c
onnectivities');
#88472=UNCERTAINTY_MEASURE_WITH_UNIT(LENGTH_MEASURE(0.01),#88484,
'DISTANCE_ACCURACY_VALUE',
'Maximum model space distance between geometric entities at asserted c
onnectivities');
#88474=(
GEOMETRIC_REPRESENTATION_CONTEXT(3)
GLOBAL_UNCERTAINTY_ASSIGNED_CONTEXT((#88463))
GLOBAL_UNIT_ASSIGNED_CONTEXT((#88484,#88486,#88487))
REPRESENTATION_CONTEXT('','3D')
);
#88483=(
GEOMETRIC_REPRESENTATION_CONTEXT(3)
GLOBAL_UNCERTAINTY_ASSIGNED_CONTEXT((#88472))
GLOBAL_UNIT_ASSIGNED_CONTEXT((#88484,#88486,#88487))
REPRESENTATION_CONTEXT('','3D')
);
#88484=(
LENGTH_UNIT()
NAMED_UNIT(*)
SI_UNIT(.MILLI.,.METRE.)
);
#88486=(
NAMED_UNIT(*)
PLANE_ANGLE_UNIT()
SI_UNIT($,.RADIAN.)
);
#88487=(
NAMED_UNIT(*)
SI_UNIT($,.STERADIAN.)
SOLID_ANGLE_UNIT()
);
#88489=SHAPE_DEFINITION_REPRESENTATION(#88499,#88520);
#88499=PRODUCT_DEFINITION_SHAPE('',$,#88531);
#88520=SHAPE_REPRESENTATION('',(#13128),#88474);
#88529=PRODUCT_DEFINITION_CONTEXT('part definition',#88561,'design');
#88531=PRODUCT_DEFINITION('Wormgear','Wormgear',#88541,#88529);
#88541=PRODUCT_DEFINITION_FORMATION('',$,#88564);
#88561=APPLICATION_CONTEXT(
'Core Data for Automotive Mechanical Design Process');
#88562=PRODUCT_CONTEXT('part definition',#88561,'mechanical');
#88564=PRODUCT('Wormgear','Wormgear',$,(#88562));
#88574=PRESENTATION_STYLE_ASSIGNMENT((#88576));
#88576=SURFACE_STYLE_USAGE(.BOTH.,#88578);
#88578=SURFACE_SIDE_STYLE('',(#88580));
#88580=SURFACE_STYLE_FILL_AREA(#88582);
#88582=FILL_AREA_STYLE('Opaque(160,160,160)',(#88584));
#88584=FILL_AREA_STYLE_COLOUR('Opaque(160,160,160)',#88586);
#88586=COLOUR_RGB('Opaque(160,160,160)', 0.66274510, 0.83137255, 0.94901961);
ENDSEC;
END-ISO-10303-21;
